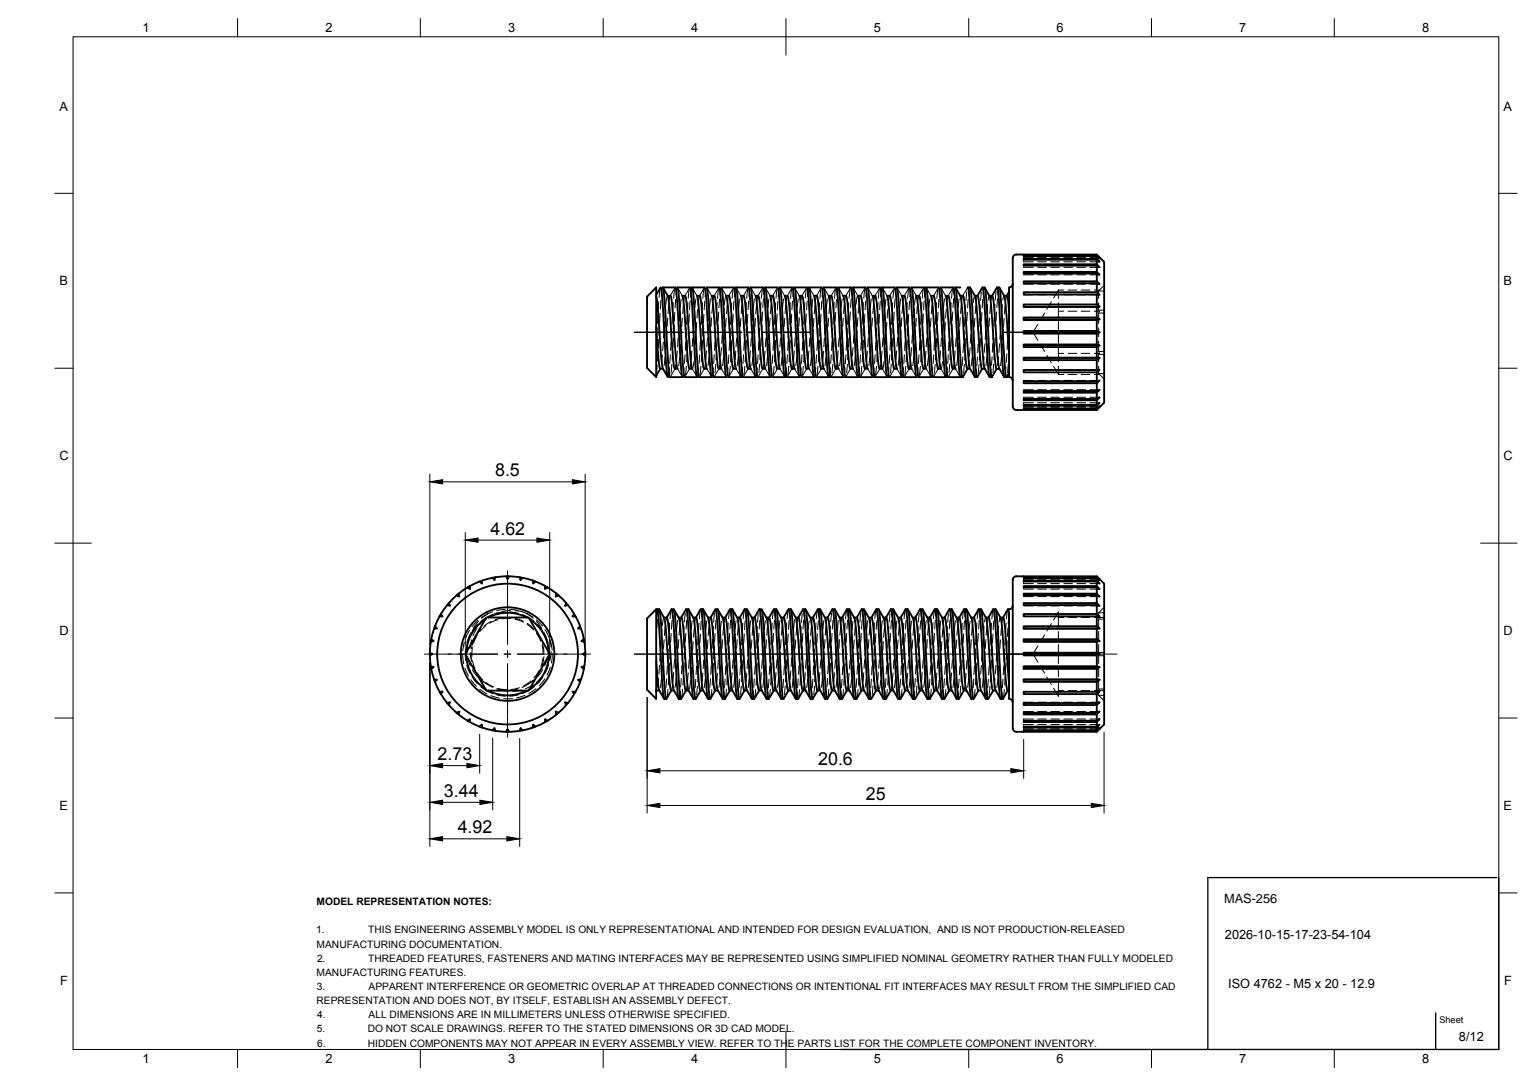
ISO-10303-21;
HEADER;
/* Generated by software containing ST-Developer
 * from STEP Tools, Inc. (www.steptools.com) 
 */

FILE_DESCRIPTION(
/* description */ (''),
/* implementation_level */ '2;1');

FILE_NAME(
/* name */ 'ISO 4762 - M5 x 20 - 12.9.step',
/* time_stamp */ '2026-10-14T18:40:07-07:00',
/* author */ (''),
/* organization */ (''),
/* preprocessor_version */ 'ST-DEVELOPER v20.2',
/* originating_system */ 'Autodesk Translation Framework v15.15.0.0',
/* authorisation */ '');

FILE_SCHEMA (('AUTOMOTIVE_DESIGN { 1 0 10303 214 3 1 1 }'));
ENDSEC;

DATA;
#10=MECHANICAL_DESIGN_GEOMETRIC_PRESENTATION_REPRESENTATION('',(#837),#81040);
#260=(
BOUNDED_CURVE()
B_SPLINE_CURVE(2,(#42262,#42263,#42264),.UNSPECIFIED.,.F.,.F.)
B_SPLINE_CURVE_WITH_KNOTS((3,3),(0.,0.0216285523885327),.UNSPECIFIED.)
CURVE()
GEOMETRIC_REPRESENTATION_ITEM()
RATIONAL_B_SPLINE_CURVE((1.,1.000549833114,1.00070303138813))
REPRESENTATION_ITEM('')
);
#261=(
BOUNDED_CURVE()
B_SPLINE_CURVE(2,(#42268,#42269,#42270),.UNSPECIFIED.,.F.,.F.)
B_SPLINE_CURVE_WITH_KNOTS((3,3),(0.0383363983196538,0.0599649507081082),
 .UNSPECIFIED.)
CURVE()
GEOMETRIC_REPRESENTATION_ITEM()
RATIONAL_B_SPLINE_CURVE((1.00070303139789,1.00054983312164,1.))
REPRESENTATION_ITEM('')
);
#262=(
BOUNDED_CURVE()
B_SPLINE_CURVE(2,(#42563,#42564,#42565),.UNSPECIFIED.,.F.,.F.)
B_SPLINE_CURVE_WITH_KNOTS((3,3),(0.,0.0216285523885616),.UNSPECIFIED.)
CURVE()
GEOMETRIC_REPRESENTATION_ITEM()
RATIONAL_B_SPLINE_CURVE((1.,1.00054983311705,1.00070303139203))
REPRESENTATION_ITEM('')
);
#263=(
BOUNDED_CURVE()
B_SPLINE_CURVE(2,(#42567,#42568,#42569),.UNSPECIFIED.,.F.,.F.)
B_SPLINE_CURVE_WITH_KNOTS((3,3),(0.0383363983195465,0.0599649507081086),
 .UNSPECIFIED.)
CURVE()
GEOMETRIC_REPRESENTATION_ITEM()
RATIONAL_B_SPLINE_CURVE((1.00070303139079,1.00054983311608,1.))
REPRESENTATION_ITEM('')
);
#264=(
BOUNDED_CURVE()
B_SPLINE_CURVE(2,(#42574,#42575,#42576),.UNSPECIFIED.,.F.,.F.)
B_SPLINE_CURVE_WITH_KNOTS((3,3),(0.0383363983195738,0.0599649507081061),
 .UNSPECIFIED.)
CURVE()
GEOMETRIC_REPRESENTATION_ITEM()
RATIONAL_B_SPLINE_CURVE((1.00070303139411,1.00054983311868,1.))
REPRESENTATION_ITEM('')
);
#265=(
BOUNDED_CURVE()
B_SPLINE_CURVE(2,(#42578,#42579,#42580),.UNSPECIFIED.,.F.,.F.)
B_SPLINE_CURVE_WITH_KNOTS((3,3),(0.,0.0216285523884906),.UNSPECIFIED.)
CURVE()
GEOMETRIC_REPRESENTATION_ITEM()
RATIONAL_B_SPLINE_CURVE((1.,1.00054983311838,1.00070303139373))
REPRESENTATION_ITEM('')
);
#266=(
BOUNDED_CURVE()
B_SPLINE_CURVE(2,(#42581,#42582,#42583),.UNSPECIFIED.,.F.,.F.)
B_SPLINE_CURVE_WITH_KNOTS((3,3),(0.0383363983195406,0.0599649507081063),
 .UNSPECIFIED.)
CURVE()
GEOMETRIC_REPRESENTATION_ITEM()
RATIONAL_B_SPLINE_CURVE((1.00070303138964,1.00054983311518,1.))
REPRESENTATION_ITEM('')
);
#267=(
BOUNDED_CURVE()
B_SPLINE_CURVE(2,(#42585,#42586,#42587),.UNSPECIFIED.,.F.,.F.)
B_SPLINE_CURVE_WITH_KNOTS((3,3),(0.,0.0216285523884772),.UNSPECIFIED.)
CURVE()
GEOMETRIC_REPRESENTATION_ITEM()
RATIONAL_B_SPLINE_CURVE((1.,1.00054983312122,1.00070303139736))
REPRESENTATION_ITEM('')
);
#268=(
BOUNDED_CURVE()
B_SPLINE_CURVE(2,(#42588,#42589,#42590),.UNSPECIFIED.,.F.,.F.)
B_SPLINE_CURVE_WITH_KNOTS((3,3),(0.0383363983195954,0.0599649507081057),
 .UNSPECIFIED.)
CURVE()
GEOMETRIC_REPRESENTATION_ITEM()
RATIONAL_B_SPLINE_CURVE((1.00070303139538,1.00054983311967,1.))
REPRESENTATION_ITEM('')
);
#269=(
BOUNDED_CURVE()
B_SPLINE_CURVE(2,(#42592,#42593,#42594),.UNSPECIFIED.,.F.,.F.)
B_SPLINE_CURVE_WITH_KNOTS((3,3),(0.,0.0216285523885691),.UNSPECIFIED.)
CURVE()
GEOMETRIC_REPRESENTATION_ITEM()
RATIONAL_B_SPLINE_CURVE((1.,1.00054983311357,1.00070303138758))
REPRESENTATION_ITEM('')
);
#270=(
BOUNDED_CURVE()
B_SPLINE_CURVE(2,(#42595,#42596,#42597),.UNSPECIFIED.,.F.,.F.)
B_SPLINE_CURVE_WITH_KNOTS((3,3),(0.0383363983195734,0.0599649507081057),
 .UNSPECIFIED.)
CURVE()
GEOMETRIC_REPRESENTATION_ITEM()
RATIONAL_B_SPLINE_CURVE((1.00070303138924,1.00054983311487,1.))
REPRESENTATION_ITEM('')
);
#271=(
BOUNDED_CURVE()
B_SPLINE_CURVE(2,(#42599,#42600,#42601),.UNSPECIFIED.,.F.,.F.)
B_SPLINE_CURVE_WITH_KNOTS((3,3),(0.,0.021628552388544),.UNSPECIFIED.)
CURVE()
GEOMETRIC_REPRESENTATION_ITEM()
RATIONAL_B_SPLINE_CURVE((1.,1.00054983311579,1.00070303139042))
REPRESENTATION_ITEM('')
);
#272=(
BOUNDED_CURVE()
B_SPLINE_CURVE(2,(#42602,#42603,#42604),.UNSPECIFIED.,.F.,.F.)
B_SPLINE_CURVE_WITH_KNOTS((3,3),(0.0383363983195219,0.0599649507081056),
 .UNSPECIFIED.)
CURVE()
GEOMETRIC_REPRESENTATION_ITEM()
RATIONAL_B_SPLINE_CURVE((1.00070303138672,1.0005498331129,1.))
REPRESENTATION_ITEM('')
);
#273=(
BOUNDED_CURVE()
B_SPLINE_CURVE(2,(#42606,#42607,#42608),.UNSPECIFIED.,.F.,.F.)
B_SPLINE_CURVE_WITH_KNOTS((3,3),(0.,0.0216285523886276),.UNSPECIFIED.)
CURVE()
GEOMETRIC_REPRESENTATION_ITEM()
RATIONAL_B_SPLINE_CURVE((1.,1.00054983311002,1.00070303138303))
REPRESENTATION_ITEM('')
);
#274=(
BOUNDED_CURVE()
B_SPLINE_CURVE(2,(#42609,#42610,#42611),.UNSPECIFIED.,.F.,.F.)
B_SPLINE_CURVE_WITH_KNOTS((3,3),(0.0383363983195948,0.0599649507081057),
 .UNSPECIFIED.)
CURVE()
GEOMETRIC_REPRESENTATION_ITEM()
RATIONAL_B_SPLINE_CURVE((1.00070303139332,1.00054983311806,1.))
REPRESENTATION_ITEM('')
);
#275=(
BOUNDED_CURVE()
B_SPLINE_CURVE(2,(#42613,#42614,#42615),.UNSPECIFIED.,.F.,.F.)
B_SPLINE_CURVE_WITH_KNOTS((3,3),(0.,0.0216285523885387),.UNSPECIFIED.)
CURVE()
GEOMETRIC_REPRESENTATION_ITEM()
RATIONAL_B_SPLINE_CURVE((1.,1.00054983311459,1.00070303138888))
REPRESENTATION_ITEM('')
);
#276=(
BOUNDED_CURVE()
B_SPLINE_CURVE(2,(#42616,#42617,#42618),.UNSPECIFIED.,.F.,.F.)
B_SPLINE_CURVE_WITH_KNOTS((3,3),(0.0383363983195453,0.0599649507081048),
 .UNSPECIFIED.)
CURVE()
GEOMETRIC_REPRESENTATION_ITEM()
RATIONAL_B_SPLINE_CURVE((1.00070303138923,1.00054983311486,1.))
REPRESENTATION_ITEM('')
);
#277=(
BOUNDED_CURVE()
B_SPLINE_CURVE(2,(#42620,#42621,#42622),.UNSPECIFIED.,.F.,.F.)
B_SPLINE_CURVE_WITH_KNOTS((3,3),(0.,0.0216285523885327),.UNSPECIFIED.)
CURVE()
GEOMETRIC_REPRESENTATION_ITEM()
RATIONAL_B_SPLINE_CURVE((1.,1.000549833118,1.00070303139324))
REPRESENTATION_ITEM('')
);
#278=(
BOUNDED_CURVE()
B_SPLINE_CURVE(2,(#42623,#42624,#42625),.UNSPECIFIED.,.F.,.F.)
B_SPLINE_CURVE_WITH_KNOTS((3,3),(0.038336398319501,0.0599649507081059),
 .UNSPECIFIED.)
CURVE()
GEOMETRIC_REPRESENTATION_ITEM()
RATIONAL_B_SPLINE_CURVE((1.00070303138577,1.00054983311216,1.))
REPRESENTATION_ITEM('')
);
#279=(
BOUNDED_CURVE()
B_SPLINE_CURVE(2,(#42627,#42628,#42629),.UNSPECIFIED.,.F.,.F.)
B_SPLINE_CURVE_WITH_KNOTS((3,3),(0.,0.0216285523885216),.UNSPECIFIED.)
CURVE()
GEOMETRIC_REPRESENTATION_ITEM()
RATIONAL_B_SPLINE_CURVE((1.,1.0005498331148,1.00070303138915))
REPRESENTATION_ITEM('')
);
#280=(
BOUNDED_CURVE()
B_SPLINE_CURVE(2,(#42630,#42631,#42632),.UNSPECIFIED.,.F.,.F.)
B_SPLINE_CURVE_WITH_KNOTS((3,3),(0.0383363983195421,0.0599649507081054),
 .UNSPECIFIED.)
CURVE()
GEOMETRIC_REPRESENTATION_ITEM()
RATIONAL_B_SPLINE_CURVE((1.00070303139029,1.00054983311569,1.))
REPRESENTATION_ITEM('')
);
#281=(
BOUNDED_CURVE()
B_SPLINE_CURVE(2,(#42634,#42635,#42636),.UNSPECIFIED.,.F.,.F.)
B_SPLINE_CURVE_WITH_KNOTS((3,3),(0.,0.0216285523885795),.UNSPECIFIED.)
CURVE()
GEOMETRIC_REPRESENTATION_ITEM()
RATIONAL_B_SPLINE_CURVE((1.,1.0005498331127,1.00070303138646))
REPRESENTATION_ITEM('')
);
#282=(
BOUNDED_CURVE()
B_SPLINE_CURVE(2,(#42637,#42638,#42639),.UNSPECIFIED.,.F.,.F.)
B_SPLINE_CURVE_WITH_KNOTS((3,3),(0.0383363983195796,0.0599649507081049),
 .UNSPECIFIED.)
CURVE()
GEOMETRIC_REPRESENTATION_ITEM()
RATIONAL_B_SPLINE_CURVE((1.00070303139298,1.00054983311779,1.))
REPRESENTATION_ITEM('')
);
#283=(
BOUNDED_CURVE()
B_SPLINE_CURVE(2,(#42641,#42642,#42643),.UNSPECIFIED.,.F.,.F.)
B_SPLINE_CURVE_WITH_KNOTS((3,3),(0.,0.0216285523885516),.UNSPECIFIED.)
CURVE()
GEOMETRIC_REPRESENTATION_ITEM()
RATIONAL_B_SPLINE_CURVE((1.,1.00054983311626,1.00070303139102))
REPRESENTATION_ITEM('')
);
#284=(
BOUNDED_CURVE()
B_SPLINE_CURVE(2,(#42644,#42645,#42646),.UNSPECIFIED.,.F.,.F.)
B_SPLINE_CURVE_WITH_KNOTS((3,3),(0.0383363983195596,0.059964950708105),
 .UNSPECIFIED.)
CURVE()
GEOMETRIC_REPRESENTATION_ITEM()
RATIONAL_B_SPLINE_CURVE((1.00070303138868,1.00054983311444,1.))
REPRESENTATION_ITEM('')
);
#285=(
BOUNDED_CURVE()
B_SPLINE_CURVE(2,(#42648,#42649,#42650),.UNSPECIFIED.,.F.,.F.)
B_SPLINE_CURVE_WITH_KNOTS((3,3),(0.,0.0216285523885783),.UNSPECIFIED.)
CURVE()
GEOMETRIC_REPRESENTATION_ITEM()
RATIONAL_B_SPLINE_CURVE((1.,1.00054983311312,1.000703031387))
REPRESENTATION_ITEM('')
);
#286=(
BOUNDED_CURVE()
B_SPLINE_CURVE(2,(#42651,#42652,#42653),.UNSPECIFIED.,.F.,.F.)
B_SPLINE_CURVE_WITH_KNOTS((3,3),(0.0383363983195159,0.0599649507081054),
 .UNSPECIFIED.)
CURVE()
GEOMETRIC_REPRESENTATION_ITEM()
RATIONAL_B_SPLINE_CURVE((1.00070303138659,1.0005498331128,1.))
REPRESENTATION_ITEM('')
);
#287=(
BOUNDED_CURVE()
B_SPLINE_CURVE(2,(#42655,#42656,#42657),.UNSPECIFIED.,.F.,.F.)
B_SPLINE_CURVE_WITH_KNOTS((3,3),(0.,0.0216285523885604),.UNSPECIFIED.)
CURVE()
GEOMETRIC_REPRESENTATION_ITEM()
RATIONAL_B_SPLINE_CURVE((1.,1.00054983311293,1.00070303138676))
REPRESENTATION_ITEM('')
);
#288=(
BOUNDED_CURVE()
B_SPLINE_CURVE(2,(#42658,#42659,#42660),.UNSPECIFIED.,.F.,.F.)
B_SPLINE_CURVE_WITH_KNOTS((3,3),(0.0383363983195082,0.0599649507081046),
 .UNSPECIFIED.)
CURVE()
GEOMETRIC_REPRESENTATION_ITEM()
RATIONAL_B_SPLINE_CURVE((1.00070303138548,1.00054983311193,1.))
REPRESENTATION_ITEM('')
);
#289=(
BOUNDED_CURVE()
B_SPLINE_CURVE(2,(#42662,#42663,#42664),.UNSPECIFIED.,.F.,.F.)
B_SPLINE_CURVE_WITH_KNOTS((3,3),(0.,0.0216285523886338),.UNSPECIFIED.)
CURVE()
GEOMETRIC_REPRESENTATION_ITEM()
RATIONAL_B_SPLINE_CURVE((1.,1.00054983310968,1.00070303138259))
REPRESENTATION_ITEM('')
);
#290=(
BOUNDED_CURVE()
B_SPLINE_CURVE(2,(#42665,#42666,#42667),.UNSPECIFIED.,.F.,.F.)
B_SPLINE_CURVE_WITH_KNOTS((3,3),(0.0383363983196053,0.0599649507081053),
 .UNSPECIFIED.)
CURVE()
GEOMETRIC_REPRESENTATION_ITEM()
RATIONAL_B_SPLINE_CURVE((1.00070303139687,1.00054983312084,1.))
REPRESENTATION_ITEM('')
);
#291=(
BOUNDED_CURVE()
B_SPLINE_CURVE(2,(#42669,#42670,#42671),.UNSPECIFIED.,.F.,.F.)
B_SPLINE_CURVE_WITH_KNOTS((3,3),(0.,0.0216285523885115),.UNSPECIFIED.)
CURVE()
GEOMETRIC_REPRESENTATION_ITEM()
RATIONAL_B_SPLINE_CURVE((1.,1.00054983312007,1.00070303139589))
REPRESENTATION_ITEM('')
);
#292=(
BOUNDED_CURVE()
B_SPLINE_CURVE(2,(#42672,#42673,#42674),.UNSPECIFIED.,.F.,.F.)
B_SPLINE_CURVE_WITH_KNOTS((3,3),(0.0383363983195966,0.0599649507081041),
 .UNSPECIFIED.)
CURVE()
GEOMETRIC_REPRESENTATION_ITEM()
RATIONAL_B_SPLINE_CURVE((1.00070303139314,1.00054983311792,1.))
REPRESENTATION_ITEM('')
);
#293=(
BOUNDED_CURVE()
B_SPLINE_CURVE(2,(#42676,#42677,#42678),.UNSPECIFIED.,.F.,.F.)
B_SPLINE_CURVE_WITH_KNOTS((3,3),(0.,0.0216285523885745),.UNSPECIFIED.)
CURVE()
GEOMETRIC_REPRESENTATION_ITEM()
RATIONAL_B_SPLINE_CURVE((1.,1.00054983311169,1.00070303138517))
REPRESENTATION_ITEM('')
);
#294=(
BOUNDED_CURVE()
B_SPLINE_CURVE(2,(#42679,#42680,#42681),.UNSPECIFIED.,.F.,.F.)
B_SPLINE_CURVE_WITH_KNOTS((3,3),(0.0383363983195842,0.0599649507081042),
 .UNSPECIFIED.)
CURVE()
GEOMETRIC_REPRESENTATION_ITEM()
RATIONAL_B_SPLINE_CURVE((1.00070303139113,1.00054983311635,1.))
REPRESENTATION_ITEM('')
);
#295=(
BOUNDED_CURVE()
B_SPLINE_CURVE(2,(#42683,#42684,#42685),.UNSPECIFIED.,.F.,.F.)
B_SPLINE_CURVE_WITH_KNOTS((3,3),(0.,0.0216285523885027),.UNSPECIFIED.)
CURVE()
GEOMETRIC_REPRESENTATION_ITEM()
RATIONAL_B_SPLINE_CURVE((1.,1.00054983311917,1.00070303139474))
REPRESENTATION_ITEM('')
);
#296=(
BOUNDED_CURVE()
B_SPLINE_CURVE(2,(#42686,#42687,#42688),.UNSPECIFIED.,.F.,.F.)
B_SPLINE_CURVE_WITH_KNOTS((3,3),(0.0383363983195908,0.0599649507081052),
 .UNSPECIFIED.)
CURVE()
GEOMETRIC_REPRESENTATION_ITEM()
RATIONAL_B_SPLINE_CURVE((1.00070303139353,1.00054983311823,1.))
REPRESENTATION_ITEM('')
);
#297=(
BOUNDED_CURVE()
B_SPLINE_CURVE(2,(#42690,#42691,#42692),.UNSPECIFIED.,.F.,.F.)
B_SPLINE_CURVE_WITH_KNOTS((3,3),(0.,0.0216285523885997),.UNSPECIFIED.)
CURVE()
GEOMETRIC_REPRESENTATION_ITEM()
RATIONAL_B_SPLINE_CURVE((1.,1.00054983311374,1.00070303138779))
REPRESENTATION_ITEM('')
);
#298=(
BOUNDED_CURVE()
B_SPLINE_CURVE(2,(#42693,#42694,#42695),.UNSPECIFIED.,.F.,.F.)
B_SPLINE_CURVE_WITH_KNOTS((3,3),(0.0383363983195373,0.0599649507081046),
 .UNSPECIFIED.)
CURVE()
GEOMETRIC_REPRESENTATION_ITEM()
RATIONAL_B_SPLINE_CURVE((1.00070303138796,1.00054983311387,1.))
REPRESENTATION_ITEM('')
);
#299=(
BOUNDED_CURVE()
B_SPLINE_CURVE(2,(#42697,#42698,#42699),.UNSPECIFIED.,.F.,.F.)
B_SPLINE_CURVE_WITH_KNOTS((3,3),(0.,0.0216285523885614),.UNSPECIFIED.)
CURVE()
GEOMETRIC_REPRESENTATION_ITEM()
RATIONAL_B_SPLINE_CURVE((1.,1.00054983311414,1.00070303138831))
REPRESENTATION_ITEM('')
);
#300=(
BOUNDED_CURVE()
B_SPLINE_CURVE(2,(#42700,#42701,#42702),.UNSPECIFIED.,.F.,.F.)
B_SPLINE_CURVE_WITH_KNOTS((3,3),(0.0383363983195286,0.0599649507081044),
 .UNSPECIFIED.)
CURVE()
GEOMETRIC_REPRESENTATION_ITEM()
RATIONAL_B_SPLINE_CURVE((1.00070303139035,1.00054983311574,1.))
REPRESENTATION_ITEM('')
);
#301=(
BOUNDED_CURVE()
B_SPLINE_CURVE(2,(#42704,#42705,#42706),.UNSPECIFIED.,.F.,.F.)
B_SPLINE_CURVE_WITH_KNOTS((3,3),(0.,0.0216285523885108),.UNSPECIFIED.)
CURVE()
GEOMETRIC_REPRESENTATION_ITEM()
RATIONAL_B_SPLINE_CURVE((1.,1.00054983311702,1.00070303139198))
REPRESENTATION_ITEM('')
);
#302=(
BOUNDED_CURVE()
B_SPLINE_CURVE(2,(#42707,#42708,#42709),.UNSPECIFIED.,.F.,.F.)
B_SPLINE_CURVE_WITH_KNOTS((3,3),(0.0383363983195893,0.0599649507081084),
 .UNSPECIFIED.)
CURVE()
GEOMETRIC_REPRESENTATION_ITEM()
RATIONAL_B_SPLINE_CURVE((1.00070303139496,1.00054983311935,1.))
REPRESENTATION_ITEM('')
);
#303=(
BOUNDED_CURVE()
B_SPLINE_CURVE(2,(#42711,#42712,#42713),.UNSPECIFIED.,.F.,.F.)
B_SPLINE_CURVE_WITH_KNOTS((3,3),(0.,0.021628552388581),.UNSPECIFIED.)
CURVE()
GEOMETRIC_REPRESENTATION_ITEM()
RATIONAL_B_SPLINE_CURVE((1.,1.00054983311652,1.00070303139135))
REPRESENTATION_ITEM('')
);
#304=(
BOUNDED_CURVE()
B_SPLINE_CURVE(2,(#42714,#42715,#42716),.UNSPECIFIED.,.F.,.F.)
B_SPLINE_CURVE_WITH_KNOTS((3,3),(0.0383363983195303,0.059964950708108),
 .UNSPECIFIED.)
CURVE()
GEOMETRIC_REPRESENTATION_ITEM()
RATIONAL_B_SPLINE_CURVE((1.00070303138822,1.00054983311407,1.))
REPRESENTATION_ITEM('')
);
#305=(
BOUNDED_CURVE()
B_SPLINE_CURVE(2,(#42718,#42719,#42720),.UNSPECIFIED.,.F.,.F.)
B_SPLINE_CURVE_WITH_KNOTS((3,3),(0.,0.0216285523886002),.UNSPECIFIED.)
CURVE()
GEOMETRIC_REPRESENTATION_ITEM()
RATIONAL_B_SPLINE_CURVE((1.,1.00054983311286,1.00070303138666))
REPRESENTATION_ITEM('')
);
#306=(
BOUNDED_CURVE()
B_SPLINE_CURVE(2,(#42721,#42722,#42723),.UNSPECIFIED.,.F.,.F.)
B_SPLINE_CURVE_WITH_KNOTS((3,3),(0.0383363983195208,0.059964950708108),
 .UNSPECIFIED.)
CURVE()
GEOMETRIC_REPRESENTATION_ITEM()
RATIONAL_B_SPLINE_CURVE((1.00070303138903,1.00054983311471,1.))
REPRESENTATION_ITEM('')
);
#307=(
BOUNDED_CURVE()
B_SPLINE_CURVE(2,(#42725,#42726,#42727),.UNSPECIFIED.,.F.,.F.)
B_SPLINE_CURVE_WITH_KNOTS((3,3),(0.,0.0216285523885397),.UNSPECIFIED.)
CURVE()
GEOMETRIC_REPRESENTATION_ITEM()
RATIONAL_B_SPLINE_CURVE((1.,1.00054983311497,1.00070303138936))
REPRESENTATION_ITEM('')
);
#308=(
BOUNDED_CURVE()
B_SPLINE_CURVE(2,(#42728,#42729,#42730),.UNSPECIFIED.,.F.,.F.)
B_SPLINE_CURVE_WITH_KNOTS((3,3),(0.0383363983195002,0.0599649507081073),
 .UNSPECIFIED.)
CURVE()
GEOMETRIC_REPRESENTATION_ITEM()
RATIONAL_B_SPLINE_CURVE((1.00070303138446,1.00054983311114,1.))
REPRESENTATION_ITEM('')
);
#309=(
BOUNDED_CURVE()
B_SPLINE_CURVE(2,(#42732,#42733,#42734),.UNSPECIFIED.,.F.,.F.)
B_SPLINE_CURVE_WITH_KNOTS((3,3),(0.,0.0216285523885717),.UNSPECIFIED.)
CURVE()
GEOMETRIC_REPRESENTATION_ITEM()
RATIONAL_B_SPLINE_CURVE((1.,1.00054983311286,1.00070303138667))
REPRESENTATION_ITEM('')
);
#310=(
BOUNDED_CURVE()
B_SPLINE_CURVE(2,(#42735,#42736,#42737),.UNSPECIFIED.,.F.,.F.)
B_SPLINE_CURVE_WITH_KNOTS((3,3),(0.0383363983195212,0.0599649507081082),
 .UNSPECIFIED.)
CURVE()
GEOMETRIC_REPRESENTATION_ITEM()
RATIONAL_B_SPLINE_CURVE((1.00070303138591,1.00054983311226,1.))
REPRESENTATION_ITEM('')
);
#311=(
BOUNDED_CURVE()
B_SPLINE_CURVE(2,(#42739,#42740,#42741),.UNSPECIFIED.,.F.,.F.)
B_SPLINE_CURVE_WITH_KNOTS((3,3),(0.,0.0216285523885764),.UNSPECIFIED.)
CURVE()
GEOMETRIC_REPRESENTATION_ITEM()
RATIONAL_B_SPLINE_CURVE((1.,1.0005498331135,1.00070303138749))
REPRESENTATION_ITEM('')
);
#312=(
BOUNDED_CURVE()
B_SPLINE_CURVE(2,(#42742,#42743,#42744),.UNSPECIFIED.,.F.,.F.)
B_SPLINE_CURVE_WITH_KNOTS((3,3),(0.0383363983195505,0.059964950708108),
 .UNSPECIFIED.)
CURVE()
GEOMETRIC_REPRESENTATION_ITEM()
RATIONAL_B_SPLINE_CURVE((1.00070303138856,1.00054983311434,1.))
REPRESENTATION_ITEM('')
);
#313=(
BOUNDED_CURVE()
B_SPLINE_CURVE(2,(#42746,#42747,#42748),.UNSPECIFIED.,.F.,.F.)
B_SPLINE_CURVE_WITH_KNOTS((3,3),(0.,0.0216285523885379),.UNSPECIFIED.)
CURVE()
GEOMETRIC_REPRESENTATION_ITEM()
RATIONAL_B_SPLINE_CURVE((1.,1.00054983311513,1.00070303138957))
REPRESENTATION_ITEM('')
);
#314=(
BOUNDED_CURVE()
B_SPLINE_CURVE(2,(#42749,#42750,#42751),.UNSPECIFIED.,.F.,.F.)
B_SPLINE_CURVE_WITH_KNOTS((3,3),(0.0383363983195525,0.0599649507081075),
 .UNSPECIFIED.)
CURVE()
GEOMETRIC_REPRESENTATION_ITEM()
RATIONAL_B_SPLINE_CURVE((1.00070303138821,1.00054983311407,1.))
REPRESENTATION_ITEM('')
);
#315=(
BOUNDED_CURVE()
B_SPLINE_CURVE(2,(#42753,#42754,#42755),.UNSPECIFIED.,.F.,.F.)
B_SPLINE_CURVE_WITH_KNOTS((3,3),(0.,0.0216285523885421),.UNSPECIFIED.)
CURVE()
GEOMETRIC_REPRESENTATION_ITEM()
RATIONAL_B_SPLINE_CURVE((1.,1.00054983311399,1.00070303138812))
REPRESENTATION_ITEM('')
);
#316=(
BOUNDED_CURVE()
B_SPLINE_CURVE(2,(#42756,#42757,#42758),.UNSPECIFIED.,.F.,.F.)
B_SPLINE_CURVE_WITH_KNOTS((3,3),(0.0383363983195263,0.0599649507081077),
 .UNSPECIFIED.)
CURVE()
GEOMETRIC_REPRESENTATION_ITEM()
RATIONAL_B_SPLINE_CURVE((1.00070303138823,1.00054983311409,1.))
REPRESENTATION_ITEM('')
);
#317=(
BOUNDED_CURVE()
B_SPLINE_CURVE(2,(#42760,#42761,#42762),.UNSPECIFIED.,.F.,.F.)
B_SPLINE_CURVE_WITH_KNOTS((3,3),(0.,0.0216285523886281),.UNSPECIFIED.)
CURVE()
GEOMETRIC_REPRESENTATION_ITEM()
RATIONAL_B_SPLINE_CURVE((1.,1.00054983311262,1.00070303138635))
REPRESENTATION_ITEM('')
);
#318=(
BOUNDED_CURVE()
B_SPLINE_CURVE(2,(#42763,#42764,#42765),.UNSPECIFIED.,.F.,.F.)
B_SPLINE_CURVE_WITH_KNOTS((3,3),(0.0383363983195607,0.0599649507081075),
 .UNSPECIFIED.)
CURVE()
GEOMETRIC_REPRESENTATION_ITEM()
RATIONAL_B_SPLINE_CURVE((1.00070303139002,1.00054983311548,1.))
REPRESENTATION_ITEM('')
);
#319=(
BOUNDED_CURVE()
B_SPLINE_CURVE(2,(#42767,#42768,#42769),.UNSPECIFIED.,.F.,.F.)
B_SPLINE_CURVE_WITH_KNOTS((3,3),(0.,0.0216285523885411),.UNSPECIFIED.)
CURVE()
GEOMETRIC_REPRESENTATION_ITEM()
RATIONAL_B_SPLINE_CURVE((1.,1.00054983311589,1.00070303139054))
REPRESENTATION_ITEM('')
);
#320=(
BOUNDED_CURVE()
B_SPLINE_CURVE(2,(#42770,#42771,#42772),.UNSPECIFIED.,.F.,.F.)
B_SPLINE_CURVE_WITH_KNOTS((3,3),(0.0383363983195253,0.0599649507081071),
 .UNSPECIFIED.)
CURVE()
GEOMETRIC_REPRESENTATION_ITEM()
RATIONAL_B_SPLINE_CURVE((1.0007030313902,1.00054983311562,1.))
REPRESENTATION_ITEM('')
);
#321=(
BOUNDED_CURVE()
B_SPLINE_CURVE(2,(#42774,#42775,#42776),.UNSPECIFIED.,.F.,.F.)
B_SPLINE_CURVE_WITH_KNOTS((3,3),(0.,0.0216285523886145),.UNSPECIFIED.)
CURVE()
GEOMETRIC_REPRESENTATION_ITEM()
RATIONAL_B_SPLINE_CURVE((1.,1.00054983311291,1.00070303138673))
REPRESENTATION_ITEM('')
);
#322=(
BOUNDED_CURVE()
B_SPLINE_CURVE(2,(#42777,#42778,#42779),.UNSPECIFIED.,.F.,.F.)
B_SPLINE_CURVE_WITH_KNOTS((3,3),(0.0383363983195111,0.0599649507081069),
 .UNSPECIFIED.)
CURVE()
GEOMETRIC_REPRESENTATION_ITEM()
RATIONAL_B_SPLINE_CURVE((1.00070303138553,1.00054983311197,1.))
REPRESENTATION_ITEM('')
);
#323=(
BOUNDED_CURVE()
B_SPLINE_CURVE(2,(#42781,#42782,#42783),.UNSPECIFIED.,.F.,.F.)
B_SPLINE_CURVE_WITH_KNOTS((3,3),(0.,0.0216285523885865),.UNSPECIFIED.)
CURVE()
GEOMETRIC_REPRESENTATION_ITEM()
RATIONAL_B_SPLINE_CURVE((1.,1.00054983311348,1.00070303138746))
REPRESENTATION_ITEM('')
);
#324=(
BOUNDED_CURVE()
B_SPLINE_CURVE(2,(#42784,#42785,#42786),.UNSPECIFIED.,.F.,.F.)
B_SPLINE_CURVE_WITH_KNOTS((3,3),(0.0383363983194927,0.0599649507081069),
 .UNSPECIFIED.)
CURVE()
GEOMETRIC_REPRESENTATION_ITEM()
RATIONAL_B_SPLINE_CURVE((1.00070303138451,1.00054983311118,1.))
REPRESENTATION_ITEM('')
);
#325=(
BOUNDED_CURVE()
B_SPLINE_CURVE(2,(#42788,#42789,#42790),.UNSPECIFIED.,.F.,.F.)
B_SPLINE_CURVE_WITH_KNOTS((3,3),(0.,0.0216285523884905),.UNSPECIFIED.)
CURVE()
GEOMETRIC_REPRESENTATION_ITEM()
RATIONAL_B_SPLINE_CURVE((1.,1.00054983311838,1.00070303139373))
REPRESENTATION_ITEM('')
);
#326=(
BOUNDED_CURVE()
B_SPLINE_CURVE(2,(#42791,#42792,#42793),.UNSPECIFIED.,.F.,.F.)
B_SPLINE_CURVE_WITH_KNOTS((3,3),(0.0383363983196131,0.0599649507081062),
 .UNSPECIFIED.)
CURVE()
GEOMETRIC_REPRESENTATION_ITEM()
RATIONAL_B_SPLINE_CURVE((1.00070303139756,1.00054983312138,1.))
REPRESENTATION_ITEM('')
);
#327=(
BOUNDED_CURVE()
B_SPLINE_CURVE(2,(#42795,#42796,#42797),.UNSPECIFIED.,.F.,.F.)
B_SPLINE_CURVE_WITH_KNOTS((3,3),(0.,0.0216285523886255),.UNSPECIFIED.)
CURVE()
GEOMETRIC_REPRESENTATION_ITEM()
RATIONAL_B_SPLINE_CURVE((1.,1.00054983311094,1.00070303138421))
REPRESENTATION_ITEM('')
);
#328=(
BOUNDED_CURVE()
B_SPLINE_CURVE(2,(#42798,#42799,#42800),.UNSPECIFIED.,.F.,.F.)
B_SPLINE_CURVE_WITH_KNOTS((3,3),(0.0383363983195603,0.0599649507081068),
 .UNSPECIFIED.)
CURVE()
GEOMETRIC_REPRESENTATION_ITEM()
RATIONAL_B_SPLINE_CURVE((1.0007030313936,1.00054983311828,1.))
REPRESENTATION_ITEM('')
);
#329=(
BOUNDED_CURVE()
B_SPLINE_CURVE(2,(#42802,#42803,#42804),.UNSPECIFIED.,.F.,.F.)
B_SPLINE_CURVE_WITH_KNOTS((3,3),(0.,0.021628552388625),.UNSPECIFIED.)
CURVE()
GEOMETRIC_REPRESENTATION_ITEM()
RATIONAL_B_SPLINE_CURVE((1.,1.00054983311264,1.00070303138639))
REPRESENTATION_ITEM('')
);
#330=(
BOUNDED_CURVE()
B_SPLINE_CURVE(2,(#42805,#42806,#42807),.UNSPECIFIED.,.F.,.F.)
B_SPLINE_CURVE_WITH_KNOTS((3,3),(0.0383363983195806,0.059964950708106),
 .UNSPECIFIED.)
CURVE()
GEOMETRIC_REPRESENTATION_ITEM()
RATIONAL_B_SPLINE_CURVE((1.00070303139255,1.00054983311746,1.))
REPRESENTATION_ITEM('')
);
#331=(
BOUNDED_CURVE()
B_SPLINE_CURVE(2,(#42808,#42809,#42810),.UNSPECIFIED.,.F.,.F.)
B_SPLINE_CURVE_WITH_KNOTS((3,3),(0.,0.0216285523884755),.UNSPECIFIED.)
CURVE()
GEOMETRIC_REPRESENTATION_ITEM()
RATIONAL_B_SPLINE_CURVE((1.,1.00054983312103,1.00070303139712))
REPRESENTATION_ITEM('')
);
#332=(
BOUNDED_CURVE()
B_SPLINE_CURVE(2,(#43060,#43061,#43062),.UNSPECIFIED.,.F.,.F.)
B_SPLINE_CURVE_WITH_KNOTS((3,3),(0.,0.0124050518656677),.UNSPECIFIED.)
CURVE()
GEOMETRIC_REPRESENTATION_ITEM()
RATIONAL_B_SPLINE_CURVE((1.,1.00128973373368,1.00206600698525))
REPRESENTATION_ITEM('')
);
#333=(
BOUNDED_CURVE()
B_SPLINE_CURVE(2,(#43066,#43067,#43068),.UNSPECIFIED.,.F.,.F.)
B_SPLINE_CURVE_WITH_KNOTS((3,3),(0.0499141116010052,0.0623191634666637),
 .UNSPECIFIED.)
CURVE()
GEOMETRIC_REPRESENTATION_ITEM()
RATIONAL_B_SPLINE_CURVE((1.00206600698578,1.00128973373401,1.))
REPRESENTATION_ITEM('')
);
#334=(
BOUNDED_CURVE()
B_SPLINE_CURVE(2,(#43070,#43071,#43072),.UNSPECIFIED.,.F.,.F.)
B_SPLINE_CURVE_WITH_KNOTS((3,3),(0.,0.0124050518656597),.UNSPECIFIED.)
CURVE()
GEOMETRIC_REPRESENTATION_ITEM()
RATIONAL_B_SPLINE_CURVE((1.,1.00128973373396,1.00206600698569))
REPRESENTATION_ITEM('')
);
#335=(
BOUNDED_CURVE()
B_SPLINE_CURVE(2,(#43076,#43077,#43078),.UNSPECIFIED.,.F.,.F.)
B_SPLINE_CURVE_WITH_KNOTS((3,3),(0.049914111601003,0.0623191634666626),
 .UNSPECIFIED.)
CURVE()
GEOMETRIC_REPRESENTATION_ITEM()
RATIONAL_B_SPLINE_CURVE((1.00206600698569,1.00128973373396,1.))
REPRESENTATION_ITEM('')
);
#336=(
BOUNDED_CURVE()
B_SPLINE_CURVE(2,(#43080,#43081,#43082),.UNSPECIFIED.,.F.,.F.)
B_SPLINE_CURVE_WITH_KNOTS((3,3),(0.,0.0124050518656559),.UNSPECIFIED.)
CURVE()
GEOMETRIC_REPRESENTATION_ITEM()
RATIONAL_B_SPLINE_CURVE((1.,1.00128973373402,1.0020660069858))
REPRESENTATION_ITEM('')
);
#337=(
BOUNDED_CURVE()
B_SPLINE_CURVE(2,(#43086,#43087,#43088),.UNSPECIFIED.,.F.,.F.)
B_SPLINE_CURVE_WITH_KNOTS((3,3),(0.0499141116009975,0.062319163466664),
 .UNSPECIFIED.)
CURVE()
GEOMETRIC_REPRESENTATION_ITEM()
RATIONAL_B_SPLINE_CURVE((1.00206600698527,1.0012897337337,1.))
REPRESENTATION_ITEM('')
);
#338=(
BOUNDED_CURVE()
B_SPLINE_CURVE(2,(#43090,#43091,#43092),.UNSPECIFIED.,.F.,.F.)
B_SPLINE_CURVE_WITH_KNOTS((3,3),(0.,0.0124050518656685),.UNSPECIFIED.)
CURVE()
GEOMETRIC_REPRESENTATION_ITEM()
RATIONAL_B_SPLINE_CURVE((1.,1.00128973373364,1.00206600698518))
REPRESENTATION_ITEM('')
);
#339=(
BOUNDED_CURVE()
B_SPLINE_CURVE(2,(#43096,#43097,#43098),.UNSPECIFIED.,.F.,.F.)
B_SPLINE_CURVE_WITH_KNOTS((3,3),(0.049914111600997,0.0623191634666649),
 .UNSPECIFIED.)
CURVE()
GEOMETRIC_REPRESENTATION_ITEM()
RATIONAL_B_SPLINE_CURVE((1.00206600698519,1.00128973373364,1.))
REPRESENTATION_ITEM('')
);
#340=(
BOUNDED_CURVE()
B_SPLINE_CURVE(2,(#43100,#43101,#43102),.UNSPECIFIED.,.F.,.F.)
B_SPLINE_CURVE_WITH_KNOTS((3,3),(0.,0.0124050518656616),.UNSPECIFIED.)
CURVE()
GEOMETRIC_REPRESENTATION_ITEM()
RATIONAL_B_SPLINE_CURVE((1.,1.0012897337338,1.00206600698545))
REPRESENTATION_ITEM('')
);
#341=(
BOUNDED_CURVE()
B_SPLINE_CURVE(2,(#43106,#43107,#43108),.UNSPECIFIED.,.F.,.F.)
B_SPLINE_CURVE_WITH_KNOTS((3,3),(0.049914111601002,0.0623191634666634),
 .UNSPECIFIED.)
CURVE()
GEOMETRIC_REPRESENTATION_ITEM()
RATIONAL_B_SPLINE_CURVE((1.00206600698545,1.0012897337338,1.))
REPRESENTATION_ITEM('')
);
#342=(
BOUNDED_CURVE()
B_SPLINE_CURVE(2,(#43110,#43111,#43112),.UNSPECIFIED.,.F.,.F.)
B_SPLINE_CURVE_WITH_KNOTS((3,3),(0.,0.0124050518656481),.UNSPECIFIED.)
CURVE()
GEOMETRIC_REPRESENTATION_ITEM()
RATIONAL_B_SPLINE_CURVE((1.,1.00128973373427,1.0020660069862))
REPRESENTATION_ITEM('')
);
#343=(
BOUNDED_CURVE()
B_SPLINE_CURVE(2,(#43115,#43116,#43117),.UNSPECIFIED.,.F.,.F.)
B_SPLINE_CURVE_WITH_KNOTS((3,3),(0.0499141116009961,0.0623191634666644),
 .UNSPECIFIED.)
CURVE()
GEOMETRIC_REPRESENTATION_ITEM()
RATIONAL_B_SPLINE_CURVE((1.0020660069852,1.00128973373365,1.))
REPRESENTATION_ITEM('')
);
#360=TOROIDAL_SURFACE('',#16122,2.6505,0.2);
#361=TOROIDAL_SURFACE('',#16315,4.05,0.2);
#364=B_SPLINE_SURFACE_WITH_KNOTS('',3,3,((#40791,#40792,#40793,#40794,#40795,
#40796,#40797,#40798,#40799,#40800,#40801,#40802,#40803,#40804,#40805,#40806,
#40807,#40808,#40809,#40810,#40811,#40812,#40813,#40814,#40815,#40816,#40817,
#40818,#40819,#40820,#40821,#40822,#40823,#40824,#40825,#40826,#40827,#40828,
#40829,#40830,#40831,#40832,#40833,#40834,#40835,#40836,#40837,#40838,#40839,
#40840,#40841,#40842,#40843,#40844,#40845,#40846,#40847,#40848,#40849,#40850,
#40851,#40852,#40853,#40854,#40855,#40856,#40857,#40858,#40859,#40860,#40861,
#40862,#40863,#40864,#40865,#40866,#40867,#40868,#40869,#40870,#40871,#40872,
#40873,#40874,#40875,#40876,#40877,#40878,#40879,#40880,#40881,#40882,#40883,
#40884,#40885,#40886,#40887,#40888,#40889,#40890,#40891,#40892,#40893,#40894,
#40895,#40896,#40897,#40898,#40899,#40900,#40901,#40902,#40903,#40904,#40905,
#40906,#40907,#40908,#40909,#40910,#40911,#40912,#40913,#40914,#40915,#40916,
#40917,#40918,#40919,#40920,#40921,#40922,#40923,#40924,#40925,#40926,#40927,
#40928,#40929,#40930,#40931,#40932,#40933,#40934,#40935,#40936,#40937,#40938,
#40939,#40940,#40941,#40942,#40943,#40944,#40945,#40946,#40947),(#40948,
#40949,#40950,#40951,#40952,#40953,#40954,#40955,#40956,#40957,#40958,#40959,
#40960,#40961,#40962,#40963,#40964,#40965,#40966,#40967,#40968,#40969,#40970,
#40971,#40972,#40973,#40974,#40975,#40976,#40977,#40978,#40979,#40980,#40981,
#40982,#40983,#40984,#40985,#40986,#40987,#40988,#40989,#40990,#40991,#40992,
#40993,#40994,#40995,#40996,#40997,#40998,#40999,#41000,#41001,#41002,#41003,
#41004,#41005,#41006,#41007,#41008,#41009,#41010,#41011,#41012,#41013,#41014,
#41015,#41016,#41017,#41018,#41019,#41020,#41021,#41022,#41023,#41024,#41025,
#41026,#41027,#41028,#41029,#41030,#41031,#41032,#41033,#41034,#41035,#41036,
#41037,#41038,#41039,#41040,#41041,#41042,#41043,#41044,#41045,#41046,#41047,
#41048,#41049,#41050,#41051,#41052,#41053,#41054,#41055,#41056,#41057,#41058,
#41059,#41060,#41061,#41062,#41063,#41064,#41065,#41066,#41067,#41068,#41069,
#41070,#41071,#41072,#41073,#41074,#41075,#41076,#41077,#41078,#41079,#41080,
#41081,#41082,#41083,#41084,#41085,#41086,#41087,#41088,#41089,#41090,#41091,
#41092,#41093,#41094,#41095,#41096,#41097,#41098,#41099,#41100,#41101,#41102,
#41103,#41104),(#41105,#41106,#41107,#41108,#41109,#41110,#41111,#41112,
#41113,#41114,#41115,#41116,#41117,#41118,#41119,#41120,#41121,#41122,#41123,
#41124,#41125,#41126,#41127,#41128,#41129,#41130,#41131,#41132,#41133,#41134,
#41135,#41136,#41137,#41138,#41139,#41140,#41141,#41142,#41143,#41144,#41145,
#41146,#41147,#41148,#41149,#41150,#41151,#41152,#41153,#41154,#41155,#41156,
#41157,#41158,#41159,#41160,#41161,#41162,#41163,#41164,#41165,#41166,#41167,
#41168,#41169,#41170,#41171,#41172,#41173,#41174,#41175,#41176,#41177,#41178,
#41179,#41180,#41181,#41182,#41183,#41184,#41185,#41186,#41187,#41188,#41189,
#41190,#41191,#41192,#41193,#41194,#41195,#41196,#41197,#41198,#41199,#41200,
#41201,#41202,#41203,#41204,#41205,#41206,#41207,#41208,#41209,#41210,#41211,
#41212,#41213,#41214,#41215,#41216,#41217,#41218,#41219,#41220,#41221,#41222,
#41223,#41224,#41225,#41226,#41227,#41228,#41229,#41230,#41231,#41232,#41233,
#41234,#41235,#41236,#41237,#41238,#41239,#41240,#41241,#41242,#41243,#41244,
#41245,#41246,#41247,#41248,#41249,#41250,#41251,#41252,#41253,#41254,#41255,
#41256,#41257,#41258,#41259,#41260,#41261),(#41262,#41263,#41264,#41265,
#41266,#41267,#41268,#41269,#41270,#41271,#41272,#41273,#41274,#41275,#41276,
#41277,#41278,#41279,#41280,#41281,#41282,#41283,#41284,#41285,#41286,#41287,
#41288,#41289,#41290,#41291,#41292,#41293,#41294,#41295,#41296,#41297,#41298,
#41299,#41300,#41301,#41302,#41303,#41304,#41305,#41306,#41307,#41308,#41309,
#41310,#41311,#41312,#41313,#41314,#41315,#41316,#41317,#41318,#41319,#41320,
#41321,#41322,#41323,#41324,#41325,#41326,#41327,#41328,#41329,#41330,#41331,
#41332,#41333,#41334,#41335,#41336,#41337,#41338,#41339,#41340,#41341,#41342,
#41343,#41344,#41345,#41346,#41347,#41348,#41349,#41350,#41351,#41352,#41353,
#41354,#41355,#41356,#41357,#41358,#41359,#41360,#41361,#41362,#41363,#41364,
#41365,#41366,#41367,#41368,#41369,#41370,#41371,#41372,#41373,#41374,#41375,
#41376,#41377,#41378,#41379,#41380,#41381,#41382,#41383,#41384,#41385,#41386,
#41387,#41388,#41389,#41390,#41391,#41392,#41393,#41394,#41395,#41396,#41397,
#41398,#41399,#41400,#41401,#41402,#41403,#41404,#41405,#41406,#41407,#41408,
#41409,#41410,#41411,#41412,#41413,#41414,#41415,#41416,#41417,#41418)),
 .UNSPECIFIED.,.F.,.F.,.F.,(4,4),(4,1,1,1,1,1,1,1,1,1,1,1,1,1,1,1,1,1,1,
1,1,1,1,1,1,1,1,1,1,1,1,1,1,1,1,1,1,1,1,1,1,1,1,1,1,1,1,1,1,1,1,1,1,1,1,
1,1,1,1,1,1,1,1,1,1,1,1,1,1,1,1,1,1,1,1,1,1,1,1,1,1,1,1,1,1,1,1,1,1,1,1,
1,1,1,1,1,1,1,1,1,1,1,1,1,1,1,1,1,1,1,1,1,1,1,1,1,1,1,1,1,1,1,1,1,1,1,1,
1,1,1,1,1,1,1,1,1,1,1,1,1,1,1,1,1,1,1,1,1,1,1,1,1,1,1,4),(-0.000414828532079457,
0.0529939397069977),(8.30815772716272,9.30587489071033,10.3035920542579,
11.3013092178055,12.2990263813532,13.2967435449008,14.2944607084484,15.292177871996,
16.2898950355436,17.2876121990912,18.2853293626388,19.2830465261864,20.280763689734,
21.2784808532816,22.2761980168293,23.2739151803769,24.2716323439245,25.2693495074721,
26.2670666710197,27.2647838345673,28.2625009981149,29.2602181616625,30.2579353252101,
31.2556524887577,32.2533696523054,33.251086815853,34.2488039794006,35.2465211429482,
36.2442383064958,37.2419554700434,38.239672633591,39.2373897971386,40.2351069606862,
41.2328241242338,42.2305412877814,43.2282584513291,44.2259756148767,45.2236927784243,
46.2214099419719,47.2191271055195,48.2168442690671,49.2145614326147,50.2122785961623,
51.2099957597099,52.2077129232575,53.2054300868052,54.2031472503528,55.2008644139004,
56.198581577448,57.1962987409956,58.1940159045432,59.1917330680908,60.1894502316384,
61.187167395186,62.1848845587336,63.1826017222812,64.1803188858289,65.1780360493765,
66.1757532129241,67.1734703764717,68.1711875400193,69.1689047035669,70.1666218671145,
71.1643390306621,72.1620561942097,73.1597733577573,74.157490521305,75.1552076848526,
76.1529248484002,77.1506420119478,78.1483591754954,79.146076339043,80.1437935025906,
81.1415106661382,82.1392278296858,83.1369449932334,84.1346621567811,85.1323793203287,
86.1300964838763,87.1278136474239,88.1255308109715,89.1232479745191,90.1209651380667,
91.1186823016143,92.1163994651619,93.1141166287095,94.1118337922572,95.1095509558048,
96.1072681193524,97.1049852829,98.1027024464476,99.1004196099952,100.098136773543,
101.09585393709,102.093571100638,103.091288264186,104.089005427733,105.086722591281,
106.084439754828,107.082156918376,108.079874081924,109.077591245471,110.075308409019,
111.073025572567,112.070742736114,113.068459899662,114.066177063209,115.063894226757,
116.061611390305,117.059328553852,118.0570457174,119.054762880947,120.052480044495,
121.050197208043,122.04791437159,123.045631535138,124.043348698685,125.041065862233,
126.038783025781,127.036500189328,128.034217352876,129.031934516423,130.029651679971,
131.027368843519,132.025086007066,133.022803170614,134.020520334162,135.018237497709,
136.015954661257,137.013671824804,138.011388988352,139.0091061519,140.006823315447,
141.004540478995,142.002257642542,142.99997480609,143.997691969638,144.995409133185,
145.993126296733,146.99084346028,147.988560623828,148.986277787376,149.983994950923,
150.981712114471,151.979429278019,152.977146441566,153.974863605114,154.972580768661,
155.970297932209,156.968015095757,157.965732259304,158.963449422852,159.961166586399,
160.958883749947,161.957015742027),.UNSPECIFIED.);
#365=B_SPLINE_SURFACE_WITH_KNOTS('',3,3,((#41606,#41607,#41608,#41609,#41610,
#41611,#41612,#41613,#41614,#41615,#41616,#41617,#41618,#41619,#41620,#41621,
#41622,#41623,#41624,#41625,#41626,#41627,#41628,#41629,#41630,#41631,#41632,
#41633,#41634,#41635,#41636,#41637,#41638,#41639,#41640,#41641,#41642,#41643,
#41644,#41645,#41646,#41647,#41648,#41649,#41650,#41651,#41652,#41653,#41654,
#41655,#41656,#41657,#41658,#41659,#41660,#41661,#41662,#41663,#41664,#41665,
#41666,#41667,#41668,#41669,#41670,#41671,#41672,#41673,#41674,#41675,#41676,
#41677,#41678,#41679,#41680,#41681,#41682,#41683,#41684,#41685,#41686,#41687,
#41688,#41689,#41690,#41691,#41692,#41693,#41694,#41695,#41696,#41697,#41698,
#41699,#41700,#41701,#41702,#41703,#41704,#41705,#41706,#41707,#41708,#41709,
#41710,#41711,#41712,#41713,#41714,#41715,#41716,#41717,#41718,#41719,#41720,
#41721,#41722,#41723,#41724,#41725,#41726,#41727,#41728,#41729,#41730,#41731,
#41732,#41733,#41734,#41735,#41736,#41737,#41738,#41739,#41740,#41741,#41742,
#41743,#41744,#41745,#41746,#41747,#41748,#41749,#41750,#41751,#41752,#41753,
#41754,#41755,#41756,#41757,#41758,#41759,#41760,#41761,#41762),(#41763,
#41764,#41765,#41766,#41767,#41768,#41769,#41770,#41771,#41772,#41773,#41774,
#41775,#41776,#41777,#41778,#41779,#41780,#41781,#41782,#41783,#41784,#41785,
#41786,#41787,#41788,#41789,#41790,#41791,#41792,#41793,#41794,#41795,#41796,
#41797,#41798,#41799,#41800,#41801,#41802,#41803,#41804,#41805,#41806,#41807,
#41808,#41809,#41810,#41811,#41812,#41813,#41814,#41815,#41816,#41817,#41818,
#41819,#41820,#41821,#41822,#41823,#41824,#41825,#41826,#41827,#41828,#41829,
#41830,#41831,#41832,#41833,#41834,#41835,#41836,#41837,#41838,#41839,#41840,
#41841,#41842,#41843,#41844,#41845,#41846,#41847,#41848,#41849,#41850,#41851,
#41852,#41853,#41854,#41855,#41856,#41857,#41858,#41859,#41860,#41861,#41862,
#41863,#41864,#41865,#41866,#41867,#41868,#41869,#41870,#41871,#41872,#41873,
#41874,#41875,#41876,#41877,#41878,#41879,#41880,#41881,#41882,#41883,#41884,
#41885,#41886,#41887,#41888,#41889,#41890,#41891,#41892,#41893,#41894,#41895,
#41896,#41897,#41898,#41899,#41900,#41901,#41902,#41903,#41904,#41905,#41906,
#41907,#41908,#41909,#41910,#41911,#41912,#41913,#41914,#41915,#41916,#41917,
#41918,#41919),(#41920,#41921,#41922,#41923,#41924,#41925,#41926,#41927,
#41928,#41929,#41930,#41931,#41932,#41933,#41934,#41935,#41936,#41937,#41938,
#41939,#41940,#41941,#41942,#41943,#41944,#41945,#41946,#41947,#41948,#41949,
#41950,#41951,#41952,#41953,#41954,#41955,#41956,#41957,#41958,#41959,#41960,
#41961,#41962,#41963,#41964,#41965,#41966,#41967,#41968,#41969,#41970,#41971,
#41972,#41973,#41974,#41975,#41976,#41977,#41978,#41979,#41980,#41981,#41982,
#41983,#41984,#41985,#41986,#41987,#41988,#41989,#41990,#41991,#41992,#41993,
#41994,#41995,#41996,#41997,#41998,#41999,#42000,#42001,#42002,#42003,#42004,
#42005,#42006,#42007,#42008,#42009,#42010,#42011,#42012,#42013,#42014,#42015,
#42016,#42017,#42018,#42019,#42020,#42021,#42022,#42023,#42024,#42025,#42026,
#42027,#42028,#42029,#42030,#42031,#42032,#42033,#42034,#42035,#42036,#42037,
#42038,#42039,#42040,#42041,#42042,#42043,#42044,#42045,#42046,#42047,#42048,
#42049,#42050,#42051,#42052,#42053,#42054,#42055,#42056,#42057,#42058,#42059,
#42060,#42061,#42062,#42063,#42064,#42065,#42066,#42067,#42068,#42069,#42070,
#42071,#42072,#42073,#42074,#42075,#42076),(#42077,#42078,#42079,#42080,
#42081,#42082,#42083,#42084,#42085,#42086,#42087,#42088,#42089,#42090,#42091,
#42092,#42093,#42094,#42095,#42096,#42097,#42098,#42099,#42100,#42101,#42102,
#42103,#42104,#42105,#42106,#42107,#42108,#42109,#42110,#42111,#42112,#42113,
#42114,#42115,#42116,#42117,#42118,#42119,#42120,#42121,#42122,#42123,#42124,
#42125,#42126,#42127,#42128,#42129,#42130,#42131,#42132,#42133,#42134,#42135,
#42136,#42137,#42138,#42139,#42140,#42141,#42142,#42143,#42144,#42145,#42146,
#42147,#42148,#42149,#42150,#42151,#42152,#42153,#42154,#42155,#42156,#42157,
#42158,#42159,#42160,#42161,#42162,#42163,#42164,#42165,#42166,#42167,#42168,
#42169,#42170,#42171,#42172,#42173,#42174,#42175,#42176,#42177,#42178,#42179,
#42180,#42181,#42182,#42183,#42184,#42185,#42186,#42187,#42188,#42189,#42190,
#42191,#42192,#42193,#42194,#42195,#42196,#42197,#42198,#42199,#42200,#42201,
#42202,#42203,#42204,#42205,#42206,#42207,#42208,#42209,#42210,#42211,#42212,
#42213,#42214,#42215,#42216,#42217,#42218,#42219,#42220,#42221,#42222,#42223,
#42224,#42225,#42226,#42227,#42228,#42229,#42230,#42231,#42232,#42233)),
 .UNSPECIFIED.,.F.,.F.,.F.,(4,4),(4,1,1,1,1,1,1,1,1,1,1,1,1,1,1,1,1,1,1,
1,1,1,1,1,1,1,1,1,1,1,1,1,1,1,1,1,1,1,1,1,1,1,1,1,1,1,1,1,1,1,1,1,1,1,1,
1,1,1,1,1,1,1,1,1,1,1,1,1,1,1,1,1,1,1,1,1,1,1,1,1,1,1,1,1,1,1,1,1,1,1,1,
1,1,1,1,1,1,1,1,1,1,1,1,1,1,1,1,1,1,1,1,1,1,1,1,1,1,1,1,1,1,1,1,1,1,1,1,
1,1,1,1,1,1,1,1,1,1,1,1,1,1,1,1,1,1,1,1,1,1,1,1,1,1,1,4),(-0.000352467397055627,
0.053040310820889),(11.6159783635572,12.6141103608891,13.6118275244367,
14.6095446879844,15.607261851532,16.6049790150796,17.6026961786272,18.6004133421748,
19.5981305057224,20.59584766927,21.5935648328176,22.5912819963652,23.5889991599128,
24.5867163234605,25.5844334870081,26.5821506505557,27.5798678141033,28.5775849776509,
29.5753021411985,30.5730193047461,31.5707364682937,32.5684536318413,33.5661707953889,
34.5638879589366,35.5616051224842,36.5593222860318,37.5570394495794,38.554756613127,
39.5524737766746,40.5501909402222,41.5479081037698,42.5456252673174,43.543342430865,
44.5410595944127,45.5387767579603,46.5364939215079,47.5342110850555,48.5319282486031,
49.5296454121507,50.5273625756983,51.5250797392459,52.5227969027935,53.5205140663411,
54.5182312298887,55.5159483934364,56.513665556984,57.5113827205316,58.5090998840792,
59.5068170476268,60.5045342111744,61.502251374722,62.4999685382696,63.4976857018172,
64.4954028653649,65.4931200289125,66.4908371924601,67.4885543560077,68.4862715195553,
69.4839886831029,70.4817058466505,71.4794230101981,72.4771401737457,73.4748573372933,
74.4725745008409,75.4702916643886,76.4680088279362,77.4657259914838,78.4634431550314,
79.461160318579,80.4588774821266,81.4565946456742,82.4543118092218,83.4520289727694,
84.449746136317,85.4474632998647,86.4451804634123,87.4428976269599,88.4406147905075,
89.4383319540551,90.4360491176027,91.4337662811503,92.4314834446979,93.4292006082455,
94.4269177717931,95.4246349353407,96.4223520988884,97.420069262436,98.4177864259836,
99.4155035895312,100.413220753079,101.410937916626,102.408655080174,103.406372243722,
104.404089407269,105.401806570817,106.399523734364,107.397240897912,108.39495806146,
109.392675225007,110.390392388555,111.388109552103,112.38582671565,113.383543879198,
114.381261042745,115.378978206293,116.376695369841,117.374412533388,118.372129696936,
119.369846860483,120.367564024031,121.365281187579,122.362998351126,123.360715514674,
124.358432678221,125.356149841769,126.353867005317,127.351584168864,128.349301332412,
129.34701849596,130.344735659507,131.342452823055,132.340169986602,133.33788715015,
134.335604313698,135.333321477245,136.331038640793,137.32875580434,138.326472967888,
139.324190131436,140.321907294983,141.319624458531,142.317341622078,143.315058785626,
144.312775949174,145.310493112721,146.308210276269,147.305927439816,148.303644603364,
149.301361766912,150.299078930459,151.296796094007,152.294513257555,153.292230421102,
154.28994758465,155.287664748197,156.285381911745,157.283099075293,158.28081623884,
159.278533402388,160.276250565935,161.273967729483,162.271684893031,163.269402056578,
164.267119220126,165.264836383673),.UNSPECIFIED.);
#408=B_SPLINE_CURVE_WITH_KNOTS('',3,(#23040,#23041,#23042,#23043,#23044,
#23045,#23046,#23047,#23048,#23049,#23050,#23051,#23052,#23053,#23054,#23055,
#23056,#23057,#23058,#23059,#23060,#23061,#23062,#23063,#23064,#23065,#23066,
#23067,#23068,#23069,#23070,#23071,#23072,#23073,#23074,#23075,#23076,#23077,
#23078,#23079,#23080,#23081,#23082,#23083,#23084,#23085,#23086,#23087,#23088,
#23089,#23090,#23091,#23092,#23093,#23094,#23095,#23096,#23097,#23098,#23099,
#23100,#23101,#23102,#23103,#23104,#23105,#23106,#23107,#23108,#23109,#23110,
#23111,#23112,#23113,#23114,#23115,#23116,#23117,#23118,#23119,#23120,#23121,
#23122,#23123,#23124,#23125,#23126,#23127,#23128,#23129,#23130,#23131,#23132,
#23133,#23134,#23135,#23136,#23137,#23138,#23139,#23140,#23141,#23142,#23143,
#23144,#23145,#23146,#23147,#23148,#23149,#23150,#23151,#23152,#23153,#23154,
#23155,#23156,#23157,#23158,#23159,#23160,#23161,#23162,#23163,#23164,#23165,
#23166,#23167,#23168,#23169,#23170,#23171,#23172,#23173,#23174,#23175,#23176,
#23177,#23178,#23179,#23180,#23181,#23182,#23183,#23184,#23185,#23186,#23187,
#23188,#23189,#23190,#23191,#23192,#23193,#23194,#23195,#23196,#23197),
 .UNSPECIFIED.,.F.,.F.,(4,2,2,2,2,2,2,2,2,2,2,2,2,2,2,2,2,2,2,2,2,2,2,2,
2,2,2,2,2,2,2,2,2,2,2,2,2,2,2,2,2,2,2,2,2,2,2,2,2,2,2,2,2,2,2,2,2,2,2,2,
2,2,2,2,2,2,2,2,2,2,2,2,2,2,2,2,2,2,4),(-0.736675210638058,-0.733821596808743,
-0.694292033914328,-0.689636306082269,-0.686738441869285,-0.684478224512377,
-0.68197459732431,-0.677843159020972,-0.662315926433236,-0.609673816667036,
-0.60542480610492,-0.590249017300808,-0.587646734993429,-0.58603249381003,
-0.584775927897407,-0.583320803513858,-0.580700810859027,-0.567619048230907,
-0.498749414458695,-0.490687875993121,-0.487355526501576,-0.485269466399629,
-0.482983111861107,-0.47981466001079,-0.472190340759041,-0.461503343415649,
-0.402687458406344,-0.390008334220899,-0.387544858158691,-0.385977168728162,
-0.38472244088543,-0.383223865036566,-0.380442637090082,-0.364403892819621,
-0.310894446169308,-0.293090695693202,-0.288631625129639,-0.286024966281755,
-0.283770737027648,-0.281009047858853,-0.27569948623136,-0.268986738050613,
-0.253669224173961,-0.215639415702403,-0.191097914207698,-0.187984675517241,
-0.186403617887784,-0.185150735660367,-0.185140371720751,-0.185130377235419,
-0.185120735762252,-0.185111431649632,-0.185102450266112,-0.185093777770031,
-0.185085401014474,-0.185077307521438,-0.185069485549634,-0.185061923946848,
-0.185054612044751,-0.185047539936342,-0.1850406980958,-0.185032579111707,
-0.185024517471098,-0.185016512188063,-0.185008562278368,-0.185000666664865,
-0.184992824418986,-0.183459446820892,-0.180515474988828,-0.161220776772221,
-0.119046916699663,-0.0967044542819805,-0.0923424843568188,-0.0895154180428306,
-0.087237298885081,-0.0846349927311359,-0.0801453807302738,-0.0602832274206637,
-0.00330615950253142),.UNSPECIFIED.);
#409=B_SPLINE_CURVE_WITH_KNOTS('',3,(#23200,#23201,#23202,#23203,#23204,
#23205,#23206,#23207,#23208,#23209,#23210,#23211,#23212,#23213,#23214,#23215,
#23216,#23217,#23218,#23219,#23220,#23221,#23222,#23223,#23224,#23225,#23226,
#23227,#23228,#23229,#23230,#23231,#23232,#23233,#23234,#23235,#23236,#23237,
#23238,#23239,#23240,#23241,#23242,#23243,#23244,#23245,#23246,#23247,#23248,
#23249,#23250,#23251,#23252,#23253,#23254,#23255,#23256,#23257,#23258,#23259,
#23260,#23261,#23262,#23263,#23264,#23265,#23266,#23267,#23268,#23269,#23270,
#23271,#23272,#23273,#23274,#23275),.UNSPECIFIED.,.F.,.F.,(4,3,3,3,3,3,
3,3,3,3,3,3,3,3,3,3,3,3,3,3,3,3,3,3,3,4),(11.6163931973415,11.7237492295633,
11.835044370979,11.9423196466468,12.049596139851,12.156902775469,12.2642685060456,
12.371800331433,12.4794284226994,12.5872559860832,12.6141103608891,12.7180831030621,
12.8218829433769,12.9255411761381,13.0291226045906,13.1326641607794,13.2362027194087,
13.3398462288228,13.4435459699825,13.5474312704339,13.6118275244367,13.7169098947458,
13.8218092643123,13.9266035018259,14.0313222763496,14.054777935193),
 .UNSPECIFIED.);
#410=B_SPLINE_CURVE_WITH_KNOTS('',3,(#23280,#23281,#23282,#23283,#23284,
#23285,#23286,#23287,#23288,#23289,#23290,#23291,#23292,#23293,#23294,#23295,
#23296,#23297,#23298,#23299,#23300,#23301,#23302,#23303,#23304,#23305,#23306,
#23307,#23308,#23309,#23310,#23311,#23312,#23313,#23314,#23315,#23316,#23317,
#23318,#23319,#23320,#23321,#23322,#23323,#23324,#23325,#23326,#23327,#23328,
#23329,#23330,#23331,#23332,#23333,#23334,#23335,#23336,#23337,#23338,#23339,
#23340,#23341,#23342,#23343,#23344,#23345,#23346,#23347,#23348,#23349,#23350,
#23351,#23352,#23353,#23354,#23355,#23356,#23357,#23358,#23359,#23360,#23361,
#23362,#23363,#23364,#23365,#23366,#23367,#23368,#23369,#23370,#23371,#23372,
#23373,#23374,#23375,#23376,#23377,#23378,#23379,#23380,#23381,#23382,#23383,
#23384,#23385,#23386,#23387,#23388,#23389,#23390,#23391,#23392,#23393,#23394,
#23395,#23396,#23397,#23398,#23399,#23400,#23401,#23402,#23403,#23404,#23405,
#23406,#23407,#23408,#23409,#23410,#23411,#23412,#23413,#23414,#23415,#23416,
#23417,#23418,#23419,#23420,#23421,#23422,#23423,#23424,#23425,#23426,#23427,
#23428,#23429,#23430,#23431,#23432,#23433,#23434,#23435,#23436,#23437,#23438,
#23439,#23440,#23441,#23442,#23443,#23444,#23445,#23446,#23447,#23448,#23449,
#23450,#23451,#23452,#23453,#23454,#23455,#23456,#23457,#23458,#23459,#23460,
#23461,#23462,#23463,#23464,#23465,#23466,#23467,#23468,#23469,#23470,#23471,
#23472,#23473,#23474,#23475,#23476,#23477,#23478,#23479,#23480,#23481,#23482,
#23483,#23484,#23485,#23486,#23487,#23488,#23489,#23490,#23491,#23492,#23493,
#23494,#23495,#23496,#23497,#23498,#23499,#23500,#23501),.UNSPECIFIED.,
 .F.,.F.,(4,2,2,2,2,2,2,2,2,2,2,2,2,2,2,2,2,2,2,2,2,2,2,2,2,2,2,2,2,2,2,
2,2,2,2,2,2,2,2,2,2,2,2,2,2,2,2,2,2,2,2,2,2,2,2,2,2,2,2,2,2,2,2,2,2,2,2,
2,2,2,2,2,2,2,2,2,2,2,2,2,2,2,2,2,2,2,2,2,2,2,2,2,2,2,2,2,2,2,2,2,2,2,2,
2,2,2,2,2,2,2,4),(-1.99319254965038,-1.98653737002634,-1.98379876219187,
-1.98231127336989,-1.98105390575671,-1.97946774020603,-1.97695764114924,
-1.96358609747753,-1.95947365261895,-1.91009979267965,-1.88997447752518,
-1.8855124399241,-1.88293983892923,-1.88069627497894,-1.87792368335606,
-1.87366964594137,-1.85263256574772,-1.80271668913237,-1.79220829787831,
-1.7878977864728,-1.78462777973597,-1.78303063756752,-1.78177262317214,
-1.78029379898174,-1.77766847778042,-1.76624504842418,-1.72805574524784,
-1.69152579643256,-1.68645760565609,-1.68375522131271,-1.68173376564286,
-1.67918575318431,-1.67483532908617,-1.65877935779111,-1.6037048732393,
-1.58756341620945,-1.5847825791044,-1.583286052845,-1.58202929210908,-1.58045430170204,
-1.57798093406084,-1.56527370394193,-1.55688098194784,-1.50556565384859,
-1.49022978933833,-1.48612066592295,-1.48362540409227,-1.48136947813647,
-1.47847265369504,-1.47380975113612,-1.44015465221223,-1.41430436279017,
-1.3907709908021,-1.38618570486933,-1.38435473181944,-1.383063591166,-1.38186692765178,
-1.38018734647392,-1.37572966665698,-1.33404109191877,-1.29299639046651,
-1.28762830059024,-1.28486300891597,-1.28261920610225,-1.28003953442239,
-1.27566305997605,-1.25870238180554,-1.20068310336964,-1.18819100667183,
-1.18559107374171,-1.18413335063411,-1.18287330707974,-1.18124711843356,
-1.17860182329707,-1.16243375888946,-1.10376929772002,-1.09093020651619,
-1.08691406550062,-1.08444070426442,-1.08218190750236,-1.07924926338534,
-1.07302093646664,-1.03972953816717,-1.0098835930594,-1.00216406863422,
-0.988916655393418,-0.986414427156384,-0.984831290152103,-0.983574602856247,
-0.982085784279071,-0.979340969979418,-0.964033763220833,-0.917227233395081,
-0.892981609427976,-0.888570353940284,-0.885748892048188,-0.883500284903431,
-0.880958973937785,-0.876643557614502,-0.858725039011845,-0.8120316403843,
-0.810317698066935,-0.80146037094138,-0.789266527434246,-0.786821851193486,
-0.785254625932403,-0.783995157677338,-0.782484136198523,-0.779651271266861,
-0.762365581868955,-0.736675210638058),.UNSPECIFIED.);
#411=B_SPLINE_CURVE_WITH_KNOTS('',3,(#23503,#23504,#23505,#23506,#23507,
#23508,#23509,#23510,#23511,#23512,#23513,#23514,#23515,#23516,#23517,#23518,
#23519,#23520,#23521,#23522,#23523,#23524,#23525,#23526,#23527,#23528,#23529,
#23530,#23531,#23532,#23533,#23534,#23535,#23536,#23537,#23538,#23539,#23540,
#23541,#23542,#23543,#23544,#23545,#23546,#23547,#23548,#23549,#23550,#23551,
#23552,#23553,#23554),.UNSPECIFIED.,.F.,.F.,(4,3,3,3,3,3,3,3,3,3,3,3,3,
3,3,3,3,4),(14.054777935193,14.1594700099767,14.2641741224379,14.3689912503651,
14.4738754371146,14.5789317449399,14.6095446879844,14.7146790594763,14.8196597064566,
14.9245217842077,15.0293208169872,15.1340920802013,15.2388708079724,15.3437622025241,
15.4487162544608,15.5538525389373,15.607261851532,15.707963267949),
 .UNSPECIFIED.);
#412=B_SPLINE_CURVE_WITH_KNOTS('',3,(#23555,#23556,#23557,#23558,#23559,
#23560,#23561,#23562,#23563,#23564,#23565,#23566,#23567,#23568,#23569,#23570,
#23571,#23572,#23573,#23574,#23575,#23576,#23577,#23578,#23579,#23580,#23581,
#23582,#23583,#23584,#23585,#23586,#23587,#23588,#23589,#23590,#23591,#23592,
#23593,#23594,#23595,#23596,#23597,#23598,#23599,#23600,#23601,#23602,#23603,
#23604,#23605,#23606,#23607,#23608,#23609,#23610,#23611,#23612,#23613,#23614,
#23615,#23616,#23617,#23618,#23619,#23620,#23621,#23622,#23623,#23624,#23625,
#23626,#23627,#23628,#23629,#23630,#23631,#23632,#23633,#23634,#23635,#23636,
#23637,#23638,#23639,#23640,#23641,#23642,#23643,#23644,#23645,#23646,#23647,
#23648,#23649,#23650,#23651,#23652,#23653,#23654,#23655,#23656,#23657,#23658,
#23659,#23660,#23661,#23662,#23663,#23664,#23665,#23666,#23667,#23668,#23669,
#23670,#23671,#23672,#23673,#23674,#23675,#23676,#23677,#23678,#23679,#23680,
#23681,#23682,#23683,#23684,#23685,#23686,#23687,#23688,#23689,#23690,#23691,
#23692,#23693,#23694,#23695,#23696,#23697,#23698,#23699,#23700,#23701,#23702,
#23703,#23704,#23705,#23706,#23707,#23708,#23709,#23710,#23711,#23712,#23713,
#23714),.UNSPECIFIED.,.F.,.F.,(4,2,2,2,2,2,2,2,2,2,2,2,2,2,2,2,2,2,2,2,
2,2,2,2,2,2,2,2,2,2,2,2,2,2,2,2,2,2,2,2,2,2,2,2,2,2,2,2,2,2,2,2,2,2,2,2,
2,2,2,2,2,2,2,2,2,2,2,2,2,2,2,2,2,2,2,2,2,2,2,4),(-2.51428340140175,-2.5075761767229,
-2.45683770840886,-2.44694558480235,-2.43976138139802,-2.43666717087808,
-2.43439424280313,-2.43229232245576,-2.42942596561606,-2.42222426557208,
-2.37875002873089,-2.35254832993181,-2.34360277058353,-2.33975515706998,
-2.33763316598838,-2.33579391733833,-2.33452171846559,-2.33334371170081,
-2.33142428110962,-2.32662747627728,-2.29536552386702,-2.26894776642379,
-2.24547788033084,-2.23934453969068,-2.23642506127349,-2.23416264487136,
-2.23167141480239,-2.22759445232846,-2.21427158911533,-2.1564453148252,
-2.14010421221288,-2.13730832658454,-2.13580526270536,-2.13454558661861,
-2.13296942338265,-2.12990975131705,-2.10887285789977,-2.05788040819895,
-2.04275310843614,-2.03866156407082,-2.03616971049145,-2.03391216218611,
-2.03100666744326,-2.02631629293022,-1.98971337666585,-1.95395538417286,
-1.94029352616069,-1.93762888225658,-1.93615744135929,-1.93489938813596,
-1.93329387424094,-1.93071738003684,-1.9161173043658,-1.8943178333712,-1.86074202471722,
-1.84349754275835,-1.83923594398317,-1.83670871473161,-1.83446173565513,
-1.83162783997351,-1.82716877083037,-1.8015579920678,-1.76511576577924,
-1.74342876761541,-1.73902692727964,-1.73722685757312,-1.73594237209019,
-1.73457089489806,-1.7323601738389,-1.72554131716868,-1.68365381660965,
-1.66232755257428,-1.64407877699645,-1.63974031220367,-1.63719430830286,
-1.63494695966009,-1.63213425033871,-1.62775052475623,-1.60421127678611,
-1.58825468741526),.UNSPECIFIED.);
#413=B_SPLINE_CURVE_WITH_KNOTS('',3,(#23720,#23721,#23722,#23723,#23724,
#23725,#23726,#23727,#23728,#23729,#23730,#23731,#23732,#23733,#23734,#23735,
#23736,#23737,#23738,#23739,#23740,#23741,#23742,#23743,#23744,#23745,#23746,
#23747,#23748,#23749,#23750,#23751,#23752,#23753,#23754,#23755,#23756,#23757,
#23758,#23759,#23760,#23761,#23762,#23763,#23764,#23765,#23766,#23767,#23768,
#23769,#23770,#23771,#23772,#23773,#23774,#23775,#23776,#23777,#23778,#23779,
#23780,#23781,#23782,#23783,#23784,#23785,#23786,#23787,#23788,#23789,#23790,
#23791,#23792,#23793,#23794,#23795,#23796,#23797,#23798,#23799,#23800,#23801,
#23802,#23803,#23804,#23805,#23806,#23807,#23808,#23809,#23810,#23811,#23812,
#23813,#23814,#23815,#23816,#23817,#23818,#23819,#23820,#23821,#23822,#23823,
#23824,#23825,#23826,#23827,#23828,#23829,#23830,#23831,#23832,#23833,#23834,
#23835,#23836,#23837,#23838,#23839,#23840,#23841,#23842,#23843,#23844,#23845,
#23846,#23847,#23848,#23849,#23850,#23851,#23852,#23853,#23854,#23855,#23856,
#23857,#23858,#23859,#23860,#23861,#23862,#23863,#23864,#23865,#23866,#23867,
#23868,#23869,#23870,#23871,#23872,#23873,#23874,#23875,#23876,#23877,#23878,
#23879),.UNSPECIFIED.,.F.,.F.,(4,2,2,2,2,2,2,2,2,2,2,2,2,2,2,2,2,2,2,2,
2,2,2,2,2,2,2,2,2,2,2,2,2,2,2,2,2,2,2,2,2,2,2,2,2,2,2,2,2,2,2,2,2,2,2,2,
2,2,2,2,2,2,2,2,2,2,2,2,2,2,2,2,2,2,2,2,2,2,2,4),(-0.926471073029744,-0.901398759294761,
-0.863449560271604,-0.8587761697636,-0.856877258545011,-0.85570281277469,
-0.854390777529996,-0.852453661213017,-0.847162662369924,-0.839085288849207,
-0.785971877562881,-0.777057598575648,-0.763193976411606,-0.75906279309083,
-0.75656269366143,-0.75430788109391,-0.751420113184561,-0.745434473064014,
-0.701439480574167,-0.663919966451118,-0.65922739160026,-0.657325276204849,
-0.656150248169787,-0.654838926037188,-0.652905234628083,-0.647638216958983,
-0.639610055216725,-0.58732950151616,-0.578277266020182,-0.563770046930224,
-0.559571489157056,-0.557056546905337,-0.555029930440796,-0.552279559627591,
-0.546982047577972,-0.540281886959943,-0.524985634153146,-0.487492707266087,
-0.462041993179969,-0.458914167666053,-0.45732445647121,-0.456066807200957,
-0.45458193471129,-0.451855905147516,-0.436961198923767,-0.393353239812336,
-0.365760600957839,-0.361234075326173,-0.358378298953241,-0.356127120693537,
-0.353608895514417,-0.349395326665183,-0.332804041632327,-0.269379222595975,
-0.261094679575136,-0.258714976427778,-0.257305711512071,-0.256034303932594,
-0.254320957608614,-0.250434290240936,-0.245054712240226,-0.230482217332864,
-0.180040824463748,-0.164788409045415,-0.160515653588025,-0.157984118036114,
-0.155959670457389,-0.153814290875608,-0.149684335246355,-0.132747892627418,
-0.104663709423388,-0.0651145466777724,-0.0605245248097448,-0.0586393776065246,
-0.0573507265026836,-0.0560085391993869,-0.0539314083632888,-0.0514996293803942,
-0.046843274153505,-0.000589973186885262),.UNSPECIFIED.);
#414=B_SPLINE_CURVE_WITH_KNOTS('',3,(#23880,#23881,#23882,#23883,#23884,
#23885,#23886,#23887,#23888,#23889,#23890,#23891,#23892,#23893,#23894,#23895,
#23896,#23897,#23898,#23899,#23900,#23901,#23902,#23903,#23904,#23905,#23906,
#23907,#23908,#23909,#23910,#23911,#23912,#23913,#23914,#23915,#23916,#23917,
#23918,#23919,#23920,#23921,#23922,#23923,#23924,#23925,#23926,#23927,#23928,
#23929,#23930,#23931,#23932,#23933,#23934,#23935,#23936,#23937,#23938,#23939),
 .UNSPECIFIED.,.F.,.F.,(4,2,2,2,2,2,2,2,2,2,2,2,2,2,2,2,2,2,2,2,2,2,2,2,
2,2,2,2,2,4),(-2.32386902743845,-2.30024041246414,-2.28982706294607,-2.28626771725673,
-2.28379755546917,-2.28169323369155,-2.27944215589424,-2.27658444578319,
-2.27205069880471,-2.24420995510776,-2.22185146770358,-2.20084557525772,
-2.18598778828631,-2.18325338576836,-2.18176690229588,-2.18050966000605,
-2.17892272561299,-2.17580707699489,-2.15134499037956,-2.1195743325545,
-2.1000265239033,-2.08816509482076,-2.0844248315671,-2.08231862587725,-2.0800700710637,
-2.07723710407267,-2.07278513444405,-2.04741796436327,-2.00170747490439,
-1.99319254965038),.UNSPECIFIED.);
#415=B_SPLINE_CURVE_WITH_KNOTS('',3,(#23940,#23941,#23942,#23943,#23944,
#23945,#23946,#23947,#23948,#23949,#23950,#23951,#23952,#23953,#23954,#23955,
#23956,#23957,#23958,#23959,#23960,#23961,#23962,#23963,#23964,#23965,#23966,
#23967,#23968,#23969,#23970,#23971,#23972,#23973,#23974,#23975,#23976,#23977,
#23978,#23979,#23980,#23981,#23982,#23983,#23984,#23985,#23986,#23987,#23988,
#23989,#23990,#23991,#23992,#23993,#23994,#23995,#23996,#23997,#23998,#23999,
#24000,#24001,#24002,#24003,#24004,#24005,#24006,#24007,#24008,#24009,#24010,
#24011,#24012,#24013,#24014,#24015,#24016,#24017,#24018,#24019,#24020,#24021,
#24022,#24023,#24024,#24025,#24026,#24027,#24028,#24029,#24030,#24031,#24032,
#24033,#24034,#24035,#24036,#24037,#24038,#24039,#24040,#24041,#24042,#24043,
#24044,#24045,#24046,#24047,#24048,#24049,#24050,#24051,#24052,#24053,#24054,
#24055,#24056,#24057,#24058,#24059,#24060,#24061,#24062,#24063,#24064,#24065,
#24066,#24067,#24068,#24069,#24070,#24071,#24072,#24073,#24074,#24075,#24076,
#24077,#24078,#24079,#24080,#24081,#24082,#24083,#24084,#24085,#24086,#24087,
#24088,#24089,#24090,#24091,#24092,#24093,#24094,#24095,#24096,#24097,#24098,
#24099,#24100,#24101,#24102,#24103,#24104,#24105,#24106,#24107,#24108,#24109,
#24110,#24111,#24112,#24113,#24114,#24115,#24116,#24117,#24118,#24119,#24120,
#24121,#24122,#24123,#24124,#24125,#24126,#24127,#24128,#24129,#24130,#24131,
#24132,#24133,#24134,#24135,#24136,#24137,#24138,#24139,#24140,#24141,#24142,
#24143,#24144,#24145,#24146,#24147,#24148,#24149,#24150,#24151),
 .UNSPECIFIED.,.F.,.F.,(4,2,2,2,2,2,2,2,2,2,2,2,2,2,2,2,2,2,2,2,2,2,2,2,
2,2,2,2,2,2,2,2,2,2,2,2,2,2,2,2,2,2,2,2,2,2,2,2,2,2,2,2,2,2,2,2,2,2,2,2,
2,2,2,2,2,2,2,2,2,2,2,2,2,2,2,2,2,2,2,2,2,2,2,2,2,2,2,2,2,2,2,2,2,2,2,2,
2,2,2,2,2,2,2,2,2,4),(-1.58825468741526,-1.55677506762686,-1.54139479875759,
-1.53864569877202,-1.53715547627514,-1.53589789844193,-1.53431399719557,
-1.53181158703341,-1.51858553333341,-1.46036439035829,-1.44421639674659,
-1.44003904369588,-1.43752901255672,-1.4352766705218,-1.43240780443973,
-1.42783719397291,-1.39873623119091,-1.35645497139845,-1.34174254908841,
-1.33902537677097,-1.33754258912259,-1.33628509220085,-1.33469355133465,
-1.33155601228223,-1.30476527817291,-1.25760534437154,-1.24442306199696,
-1.24036672110512,-1.23788355567592,-1.23562557886839,-1.23270783868223,
-1.22656355135345,-1.2029636011212,-1.17666026239359,-1.1454594412336,-1.14066498106173,
-1.13874619950042,-1.13756839240883,-1.13626106863574,-1.13434584666061,
-1.12920515949249,-1.099335148626,-1.04964048219559,-1.04338318364314,-1.04003650932242,
-1.03793804377308,-1.03563519696388,-1.0324382829047,-1.02471587082062,
-1.01386799284532,-0.952496209407458,-0.942316435553413,-0.939786839112411,
-0.938329715197559,-0.937080962753366,-0.935459307712926,-0.932064270962055,
-0.902850075623865,-0.851083944835811,-0.843539045504256,-0.840604468987905,
-0.838475751765444,-0.836195552509475,-0.833129397117509,-0.826177351757518,
-0.796164195035236,-0.765251952016309,-0.743697803607661,-0.740614769775796,
-0.739034717233685,-0.737777777429725,-0.736285594195263,-0.733524951392105,
-0.717856561959718,-0.667803722517626,-0.646912657506546,-0.642668709759187,
-0.639899310754679,-0.63765612011023,-0.63508152058239,-0.630609816994546,
-0.610327666667982,-0.559925052734969,-0.543811958200507,-0.541167496046246,
-0.539540907412971,-0.53828042250701,-0.536822407231302,-0.534220187814012,
-0.521681642425395,-0.462957025843696,-0.446684494953387,-0.442359922472271,
-0.439792878570727,-0.437548984029459,-0.434769297797808,-0.429327067146504,
-0.39206335072283,-0.3510844558689,-0.343160369793844,-0.340819935367345,
-0.339419677534822,-0.3381459957407,-0.33641512250523,-0.332427443485893,
-0.331363008767816),.UNSPECIFIED.);
#416=B_SPLINE_CURVE_WITH_KNOTS('',3,(#24156,#24157,#24158,#24159,#24160,
#24161,#24162,#24163,#24164,#24165,#24166,#24167,#24168,#24169,#24170,#24171,
#24172,#24173,#24174,#24175,#24176,#24177,#24178,#24179,#24180,#24181,#24182,
#24183,#24184,#24185,#24186,#24187,#24188,#24189,#24190,#24191,#24192,#24193,
#24194,#24195,#24196,#24197,#24198,#24199,#24200,#24201,#24202,#24203,#24204,
#24205,#24206,#24207,#24208,#24209,#24210,#24211,#24212,#24213,#24214,#24215,
#24216,#24217,#24218,#24219,#24220,#24221,#24222,#24223,#24224,#24225,#24226,
#24227,#24228,#24229,#24230,#24231,#24232,#24233,#24234,#24235,#24236,#24237,
#24238,#24239,#24240,#24241,#24242,#24243,#24244,#24245,#24246,#24247,#24248,
#24249,#24250,#24251,#24252,#24253,#24254,#24255,#24256,#24257,#24258,#24259,
#24260,#24261,#24262,#24263,#24264,#24265,#24266,#24267,#24268,#24269,#24270,
#24271,#24272,#24273,#24274,#24275,#24276,#24277,#24278,#24279,#24280,#24281,
#24282,#24283,#24284,#24285,#24286,#24287,#24288,#24289,#24290,#24291,#24292,
#24293,#24294,#24295,#24296,#24297,#24298,#24299,#24300,#24301,#24302,#24303,
#24304,#24305,#24306,#24307,#24308,#24309,#24310,#24311,#24312,#24313,#24314,
#24315,#24316,#24317,#24318,#24319,#24320,#24321,#24322,#24323,#24324,#24325,
#24326,#24327,#24328,#24329,#24330,#24331,#24332,#24333,#24334,#24335,#24336,
#24337,#24338,#24339,#24340,#24341,#24342,#24343,#24344,#24345,#24346,#24347,
#24348,#24349,#24350,#24351,#24352,#24353,#24354,#24355,#24356,#24357,#24358,
#24359,#24360,#24361,#24362,#24363,#24364,#24365,#24366,#24367,#24368,#24369,
#24370,#24371),.UNSPECIFIED.,.F.,.F.,(4,2,2,2,2,2,2,2,2,2,2,2,2,2,2,2,2,
2,2,2,2,2,2,2,2,2,2,2,2,2,2,2,2,2,2,2,2,2,2,2,2,2,2,2,2,2,2,2,2,2,2,2,2,
2,2,2,2,2,2,2,2,2,2,2,2,2,2,2,2,2,2,2,2,2,2,2,2,2,2,2,2,2,2,2,2,2,2,2,2,
2,2,2,2,2,2,2,2,2,2,2,2,2,2,2,2,2,2,4),(-2.18288930522275,-2.17834301383946,
-2.16020040172271,-2.15587072988079,-2.15332731439035,-2.1510806879597,
-2.14826681747001,-2.14387730153829,-2.1201523076371,-2.07288484499641,
-2.05752614137735,-2.05477918087068,-2.05328996736556,-2.05203287237048,
-2.05044923516515,-2.04794710130817,-2.03471863569996,-1.97652329525705,
-1.96038039200939,-1.95620379391468,-1.95369409432431,-1.9514419666657,
-1.94857325213857,-1.94400261283041,-1.91487487853451,-1.87265683400618,
-1.85795633725304,-1.85523983324506,-1.85375720853212,-1.85249967531851,
-1.85090784074904,-1.84776905670891,-1.82053844454068,-1.80702176300512,
-1.762770457098,-1.75754620130744,-1.75481133108086,-1.75278677223426,-1.75026235437542,
-1.74601912725718,-1.73107638943766,-1.72277035561684,-1.67406462991704,
-1.6585415000374,-1.65578724851468,-1.65429647179162,-1.65303948404066,
-1.65145778811473,-1.64836688534275,-1.61499255657007,-1.6073174439316,
-1.56316058746397,-1.55800618092379,-1.55528573064452,-1.55326253842361,
-1.55072773351432,-1.54643765807058,-1.53099284876732,-1.52359312990677,
-1.47079345239254,-1.46273356700672,-1.45745170533687,-1.4555160347539,
-1.45420441800844,-1.45302991697515,-1.45113012579219,-1.44645060936936,
-1.40879652980982,-1.37789096259205,-1.36733124129625,-1.35976588672558,
-1.35659469999181,-1.35429635296919,-1.35219233198252,-1.34935546633975,
-1.34239240660485,-1.29454086604358,-1.26039285948415,-1.25710430676926,
-1.25550345953941,-1.2542450605592,-1.2527686867682,-1.25008208414243,-1.23599879538802,
-1.20020177073284,-1.16420873192039,-1.15953052808974,-1.15662915048781,
-1.15437271942564,-1.15187998748226,-1.14778215559761,-1.13257488419503,
-1.08167177164236,-1.06058446385204,-1.05751334261323,-1.055935687434,-1.05467867073207,
-1.05318402170262,-1.05041255344463,-1.03449880251862,-0.981965032847736,
-0.963518796284954,-0.959029969321492,-0.956424982584346,-0.954183684597177,
-0.951452370623684,-0.946247010678033,-0.926471073029744),.UNSPECIFIED.);
#417=B_SPLINE_CURVE_WITH_KNOTS('',3,(#24373,#24374,#24375,#24376,#24377,
#24378,#24379,#24380,#24381,#24382,#24383,#24384,#24385,#24386,#24387,#24388,
#24389,#24390,#24391,#24392,#24393,#24394,#24395,#24396,#24397,#24398,#24399,
#24400,#24401,#24402,#24403,#24404,#24405,#24406,#24407,#24408,#24409,#24410,
#24411,#24412,#24413,#24414,#24415,#24416,#24417,#24418,#24419,#24420,#24421,
#24422,#24423,#24424,#24425,#24426,#24427,#24428,#24429,#24430,#24431,#24432),
 .UNSPECIFIED.,.F.,.F.,(4,2,2,2,2,2,2,2,2,2,2,2,2,2,2,2,2,2,2,2,2,2,2,2,
2,2,2,2,2,4),(-0.331363008767816,-0.314613325869936,-0.263867340288622,
-0.247176462282809,-0.242822084074471,-0.240248181884976,-0.238004959710724,
-0.235289894837674,-0.230105687478555,-0.223506425722653,-0.208541152356611,
-0.174691666715924,-0.145069412420928,-0.141929844389683,-0.140337806477531,
-0.139080220156367,-0.137597676101777,-0.13488172883738,-0.120193948897179,
-0.102666300485983,-0.0745907170427717,-0.0667114523857546,-0.0479811673334748,
-0.0434728312697193,-0.0408636002469527,-0.0386228621979387,-0.0364783822061139,
-0.0338123195932177,-0.0297771153707352,-0.000589579587611316),
 .UNSPECIFIED.);
#418=B_SPLINE_CURVE_WITH_KNOTS('',3,(#24433,#24434,#24435,#24436,#24437,
#24438,#24439,#24440,#24441,#24442,#24443,#24444,#24445,#24446,#24447,#24448,
#24449,#24450,#24451,#24452,#24453,#24454,#24455,#24456,#24457,#24458,#24459,
#24460,#24461,#24462,#24463,#24464,#24465,#24466,#24467,#24468,#24469,#24470,
#24471,#24472,#24473,#24474,#24475,#24476,#24477,#24478,#24479,#24480,#24481,
#24482,#24483,#24484,#24485,#24486,#24487,#24488,#24489,#24490,#24491,#24492,
#24493,#24494,#24495,#24496,#24497,#24498,#24499,#24500,#24501,#24502,#24503,
#24504,#24505,#24506,#24507,#24508,#24509,#24510,#24511,#24512,#24513,#24514,
#24515,#24516,#24517,#24518,#24519,#24520,#24521,#24522,#24523,#24524,#24525,
#24526,#24527,#24528,#24529,#24530,#24531,#24532,#24533,#24534,#24535,#24536,
#24537,#24538,#24539,#24540,#24541,#24542,#24543,#24544,#24545,#24546,#24547,
#24548,#24549,#24550,#24551,#24552,#24553,#24554,#24555,#24556,#24557,#24558,
#24559,#24560,#24561,#24562,#24563,#24564,#24565,#24566,#24567,#24568,#24569,
#24570,#24571,#24572,#24573,#24574,#24575,#24576,#24577,#24578,#24579,#24580,
#24581,#24582,#24583,#24584,#24585,#24586,#24587,#24588,#24589,#24590,#24591,
#24592),.UNSPECIFIED.,.F.,.F.,(4,2,2,2,2,2,2,2,2,2,2,2,2,2,2,2,2,2,2,2,
2,2,2,2,2,2,2,2,2,2,2,2,2,2,2,2,2,2,2,2,2,2,2,2,2,2,2,2,2,2,2,2,2,2,2,2,
2,2,2,2,2,2,2,2,2,2,2,2,2,2,2,2,2,2,2,2,2,2,2,4),(-2.51358401917516,-2.46703860870495,
-2.46051812019456,-2.45601462776875,-2.45419725742886,-2.45290914450858,
-2.45171041740422,-2.45002073159288,-2.44548318021959,-2.40464700529405,
-2.37779981793696,-2.36090169562812,-2.35677388468954,-2.35462965872032,
-2.35238935779344,-2.3497816367392,-2.34527840742169,-2.32661282921734,
-2.29323509950433,-2.26204653145543,-2.25680265662964,-2.25487274654001,
-2.25356258071575,-2.25238753313668,-2.25048344397783,-2.24577632722571,
-2.20858866072298,-2.17736326057625,-2.16674123678549,-2.15914203105175,
-2.15596576186363,-2.15366699020086,-2.15156482532594,-2.14873385523847,
-2.14180236408896,-2.09357101040751,-2.06252505115547,-2.05729207703341,
-2.05536366441566,-2.05405375605734,-2.05287836137734,-2.05097263444841,
-2.04625610368035,-2.00958269215844,-2.00827377236082,-1.96357062935181,
-1.95836210175496,-1.95563066737396,-1.95360665753113,-1.95108035445126,
-1.94682777536967,-1.93178326394824,-1.92412774371613,-1.87492927438097,
-1.85935091895692,-1.85659442034959,-1.85510325700639,-1.85384644525813,
-1.85226563405835,-1.84917842462162,-1.82743592732228,-1.7933232899625,
-1.7734818379219,-1.76145754600471,-1.75767679399282,-1.75525400601117,
-1.75297560363687,-1.74997200248425,-1.74318546755197,-1.69190450788205,
-1.66983204042916,-1.66282779437516,-1.65807321130845,-1.65621599499858,
-1.65492022064735,-1.65373063107379,-1.65174984896922,-1.64657571147666,
-1.60316397744653,-1.58790776972358),.UNSPECIFIED.);
#419=B_SPLINE_CURVE_WITH_KNOTS('',3,(#24598,#24599,#24600,#24601,#24602,
#24603,#24604,#24605,#24606,#24607,#24608,#24609,#24610,#24611,#24612,#24613,
#24614,#24615,#24616,#24617,#24618,#24619,#24620,#24621,#24622,#24623,#24624,
#24625,#24626,#24627,#24628,#24629,#24630,#24631,#24632,#24633,#24634,#24635,
#24636,#24637,#24638,#24639,#24640,#24641,#24642,#24643,#24644,#24645,#24646,
#24647,#24648,#24649,#24650,#24651,#24652,#24653,#24654,#24655,#24656,#24657,
#24658,#24659,#24660,#24661,#24662,#24663,#24664,#24665,#24666,#24667,#24668,
#24669,#24670,#24671,#24672,#24673,#24674,#24675,#24676,#24677,#24678,#24679,
#24680,#24681,#24682,#24683,#24684,#24685,#24686,#24687,#24688,#24689,#24690,
#24691,#24692,#24693,#24694,#24695,#24696,#24697,#24698,#24699,#24700,#24701,
#24702,#24703,#24704,#24705,#24706,#24707,#24708,#24709,#24710,#24711,#24712,
#24713,#24714,#24715,#24716,#24717,#24718,#24719,#24720,#24721,#24722,#24723,
#24724,#24725,#24726,#24727,#24728,#24729,#24730,#24731,#24732,#24733,#24734,
#24735,#24736,#24737,#24738,#24739,#24740,#24741,#24742,#24743,#24744,#24745,
#24746,#24747,#24748,#24749,#24750,#24751,#24752,#24753,#24754,#24755,#24756,
#24757,#24758,#24759,#24760,#24761,#24762,#24763,#24764,#24765,#24766,#24767,
#24768,#24769,#24770,#24771,#24772,#24773,#24774,#24775,#24776,#24777,#24778,
#24779,#24780,#24781,#24782,#24783,#24784,#24785,#24786,#24787,#24788,#24789,
#24790,#24791,#24792,#24793,#24794,#24795,#24796,#24797,#24798,#24799),
 .UNSPECIFIED.,.F.,.F.,(4,2,2,2,2,2,2,2,2,2,2,2,2,2,2,2,2,2,2,2,2,2,2,2,
2,2,2,2,2,2,2,2,2,2,2,2,2,2,2,2,2,2,2,2,2,2,2,2,2,2,2,2,2,2,2,2,2,2,2,2,
2,2,2,2,2,2,2,2,2,2,2,2,2,2,2,2,2,2,2,2,2,2,2,2,2,2,2,2,2,2,2,2,2,2,2,2,
2,2,2,2,4),(-0.926590849584021,-0.895705628617206,-0.849097035878392,-0.84205238580067,
-0.839201487858656,-0.837093933251416,-0.834798394542621,-0.831643261401205,
-0.824174518738562,-0.813788802669523,-0.7837535010908,-0.777232071165272,
-0.774946725784697,-0.756916936181162,-0.742064214596665,-0.739479374222173,
-0.737870647314892,-0.736611704772934,-0.735141235364103,-0.732481715790049,
-0.718919058633716,-0.685782092130831,-0.646498652233088,-0.641855846977377,
-0.638965158103643,-0.636710135130437,-0.634211917532468,-0.630088762293131,
-0.614588451309749,-0.562036459205467,-0.557273586525968,-0.542536259699213,
-0.539956820168759,-0.53834966162718,-0.537090765311508,-0.535618981590008,
-0.532953677846819,-0.519284180896549,-0.483463864555616,-0.479834864333695,
-0.447003099826601,-0.442349011651426,-0.43945481891684,-0.437199219675766,
-0.434702563613216,-0.430587084483246,-0.415178318239458,-0.363324761820432,
-0.356756312954078,-0.342930448248988,-0.340396089552481,-0.338802484965043,
-0.337544493127627,-0.336062417776771,-0.333349724848171,-0.318740074634343,
-0.287948673622923,-0.247447086897912,-0.242803199030523,-0.239911966447855,
-0.237656599298613,-0.2376061950838,-0.237560501009073,-0.237519066148853,
-0.237481482031868,-0.237447381287586,-0.237416432763583,-0.237388337869124,
-0.237362827247346,-0.237339657852027,-0.237318610250785,-0.237299486247105,
-0.237272793681814,-0.237246662466461,-0.237221077810542,-0.237196025360201,
-0.237171491207558,-0.237147461813345,-0.237123924063153,-0.234481204273956,
-0.229639135778107,-0.223576755855529,-0.172049741676069,-0.143982609666729,
-0.140842202158548,-0.139249695289737,-0.137991710515435,-0.136508637639563,
-0.13379154507168,-0.1190922253451,-0.0836875128642156,-0.0677007568617229,
-0.0578862961661651,-0.045709236361506,-0.0417684314047173,-0.0393099850987222,
-0.0370436444585214,-0.0348306661534586,-0.0319439022230871,-0.0273777962145406,
-0.000589178997369609),.UNSPECIFIED.);
#420=B_SPLINE_CURVE_WITH_KNOTS('',3,(#24800,#24801,#24802,#24803,#24804,
#24805,#24806,#24807,#24808,#24809,#24810,#24811,#24812,#24813,#24814,#24815,
#24816,#24817,#24818,#24819,#24820,#24821,#24822,#24823,#24824,#24825,#24826,
#24827,#24828,#24829,#24830,#24831,#24832,#24833,#24834,#24835,#24836,#24837,
#24838,#24839,#24840,#24841,#24842,#24843,#24844,#24845,#24846,#24847,#24848,
#24849,#24850,#24851,#24852,#24853),.UNSPECIFIED.,.F.,.F.,(4,2,2,2,2,2,
2,2,2,2,2,2,2,2,2,2,2,2,2,2,2,2,2,2,2,2,4),(-2.51327171715581,-2.48216238508032,
-2.45919088034406,-2.45466062409862,-2.45283886646618,-2.4515498705018,
-2.45035209269732,-2.44866616191491,-2.44415559962663,-2.40283336804128,
-2.37572130933742,-2.35946289330924,-2.35538592518744,-2.35324585131935,
-2.35102717896767,-2.34841220047479,-2.34387768404516,-2.32476294411026,
-2.27290024661368,-2.25704996916575,-2.25428163299295,-2.25278787855367,
-2.25153113879486,-2.24995323829489,-2.24687991493532,-2.22570759015456,
-2.18288930522275),.UNSPECIFIED.);
#421=B_SPLINE_CURVE_WITH_KNOTS('',3,(#24854,#24855,#24856,#24857,#24858,
#24859,#24860,#24861,#24862,#24863,#24864,#24865,#24866,#24867,#24868,#24869,
#24870,#24871,#24872,#24873,#24874,#24875,#24876,#24877,#24878,#24879,#24880,
#24881,#24882,#24883,#24884,#24885,#24886,#24887,#24888,#24889,#24890,#24891,
#24892,#24893,#24894,#24895,#24896,#24897,#24898,#24899,#24900,#24901,#24902,
#24903,#24904,#24905,#24906,#24907,#24908,#24909,#24910,#24911,#24912,#24913,
#24914,#24915,#24916,#24917,#24918,#24919,#24920,#24921,#24922,#24923,#24924,
#24925,#24926,#24927,#24928,#24929,#24930,#24931,#24932,#24933,#24934,#24935,
#24936,#24937,#24938,#24939,#24940,#24941,#24942,#24943,#24944,#24945,#24946,
#24947,#24948,#24949,#24950,#24951,#24952,#24953,#24954,#24955,#24956,#24957,
#24958,#24959,#24960,#24961,#24962,#24963,#24964,#24965,#24966,#24967,#24968,
#24969,#24970,#24971,#24972,#24973,#24974,#24975,#24976,#24977,#24978,#24979,
#24980,#24981,#24982,#24983,#24984,#24985,#24986,#24987,#24988,#24989,#24990,
#24991,#24992,#24993,#24994,#24995,#24996,#24997,#24998,#24999,#25000,#25001,
#25002,#25003,#25004,#25005,#25006,#25007,#25008,#25009,#25010,#25011,#25012,
#25013,#25014,#25015,#25016,#25017,#25018,#25019,#25020,#25021,#25022,#25023,
#25024,#25025,#25026,#25027,#25028,#25029,#25030,#25031,#25032,#25033,#25034,
#25035,#25036,#25037,#25038,#25039,#25040,#25041,#25042,#25043,#25044,#25045,
#25046,#25047,#25048,#25049,#25050,#25051,#25052,#25053,#25054,#25055,#25056,
#25057,#25058,#25059,#25060,#25061,#25062,#25063,#25064,#25065,#25066,#25067,
#25068,#25069,#25070,#25071,#25072,#25073,#25074,#25075),.UNSPECIFIED.,
 .F.,.F.,(4,2,2,2,2,2,2,2,2,2,2,2,2,2,2,2,2,2,2,2,2,2,2,2,2,2,2,2,2,2,2,
2,2,2,2,2,2,2,2,2,2,2,2,2,2,2,2,2,2,2,2,2,2,2,2,2,2,2,2,2,2,2,2,2,2,2,2,
2,2,2,2,2,2,2,2,2,2,2,2,2,2,2,2,2,2,2,2,2,2,2,2,2,2,2,2,2,2,2,2,2,2,2,2,
2,2,2,2,2,2,2,4),(-1.58790776972358,-1.56433038537726,-1.55922552834473,
-1.55651550855986,-1.55429663836922,-1.55168292212814,-1.54715436724346,
-1.52813037922064,-1.47614614877465,-1.46028109451036,-1.45751195575631,
-1.45601797405431,-1.45476117260214,-1.45318338617889,-1.4501108637531,
-1.42896988838759,-1.37803958926502,-1.36805226866343,-1.36080496724478,
-1.3576876652133,-1.35539902472085,-1.35328333181485,-1.35039917994523,
-1.34315648021733,-1.30169838395921,-1.27269464144579,-1.26449670339422,
-1.25914786400453,-1.25720279984552,-1.25601998818139,-1.25471780634858,
-1.25282809331194,-1.24786016457302,-1.24043607544603,-1.21609426764117,
-1.16831833072192,-1.16135110661376,-1.15851372473321,-1.15640974861023,
-1.15411187187234,-1.15094212745578,-1.14338416094597,-1.13283645927949,
-1.10199248833042,-1.06418610726124,-1.05951055055522,-1.05761151373998,
-1.05643722499709,-1.05512561058081,-1.05318956827674,-1.04790434174775,
-1.03983840816093,-0.986921597734203,-0.979849263367743,-0.96424914910678,
-0.959944356115374,-0.957406397205592,-0.955383753702977,-0.952667993201792,
-0.947535709764712,-0.906442000049919,-0.864311606286453,-0.859854417102353,
-0.858175525700282,-0.856979535409336,-0.855688908569718,-0.853859037279309,
-0.849278918784948,-0.825798522273947,-0.799834300346273,-0.766250011593278,
-0.761588242008963,-0.758691938877223,-0.756436334221659,-0.753941347516222,
-0.74983251145566,-0.73449664720544,-0.683187480161499,-0.674762776190746,
-0.662035645267422,-0.659561113628769,-0.657985800836894,-0.656729035787356,
-0.655232800303313,-0.652453434985366,-0.636347181587834,-0.581669316826979,
-0.565263035664434,-0.560927233560201,-0.558357533134028,-0.556113792558436,
-0.553337497964581,-0.547912321027593,-0.504863377490104,-0.465348547109447,
-0.460756767152621,-0.458871617368697,-0.457583207893888,-0.456241511823363,
-0.454165620251658,-0.447820358056242,-0.437464068155186,-0.389527692327158,
-0.366507039381414,-0.362143755338416,-0.35933772025724,-0.357091582241529,
-0.354542529520285,-0.35018792614072,-0.331697579609663,-0.331164696783045),
 .UNSPECIFIED.);
#422=B_SPLINE_CURVE_WITH_KNOTS('',3,(#25080,#25081,#25082,#25083,#25084,
#25085,#25086,#25087,#25088,#25089,#25090,#25091,#25092,#25093,#25094,#25095,
#25096,#25097,#25098,#25099,#25100,#25101,#25102,#25103,#25104,#25105,#25106,
#25107,#25108,#25109,#25110,#25111,#25112,#25113,#25114,#25115,#25116,#25117,
#25118,#25119,#25120,#25121,#25122,#25123,#25124,#25125,#25126,#25127,#25128,
#25129,#25130,#25131,#25132,#25133,#25134,#25135,#25136,#25137,#25138,#25139,
#25140,#25141,#25142,#25143,#25144,#25145,#25146,#25147,#25148,#25149,#25150,
#25151,#25152,#25153,#25154,#25155,#25156,#25157,#25158,#25159,#25160,#25161,
#25162,#25163,#25164,#25165,#25166,#25167,#25168,#25169,#25170,#25171,#25172,
#25173,#25174,#25175,#25176,#25177,#25178,#25179,#25180,#25181,#25182,#25183,
#25184,#25185,#25186,#25187,#25188,#25189,#25190,#25191,#25192,#25193,#25194,
#25195,#25196,#25197,#25198,#25199,#25200,#25201,#25202,#25203,#25204,#25205,
#25206,#25207,#25208,#25209,#25210,#25211,#25212,#25213,#25214,#25215,#25216,
#25217,#25218,#25219,#25220,#25221,#25222,#25223,#25224,#25225,#25226,#25227,
#25228,#25229,#25230,#25231,#25232,#25233,#25234,#25235,#25236,#25237,#25238,
#25239,#25240,#25241,#25242,#25243,#25244,#25245,#25246,#25247,#25248,#25249,
#25250,#25251,#25252,#25253,#25254,#25255,#25256,#25257,#25258,#25259,#25260,
#25261,#25262,#25263,#25264,#25265,#25266,#25267,#25268,#25269,#25270,#25271,
#25272,#25273,#25274,#25275,#25276,#25277,#25278,#25279,#25280,#25281,#25282,
#25283,#25284,#25285,#25286,#25287,#25288,#25289,#25290,#25291,#25292,#25293),
 .UNSPECIFIED.,.F.,.F.,(4,2,2,2,2,2,2,2,2,2,2,2,2,2,2,2,2,2,2,2,2,2,2,2,
2,2,2,2,2,2,2,2,2,2,2,2,2,2,2,2,2,2,2,2,2,2,2,2,2,2,2,2,2,2,2,2,2,2,2,2,
2,2,2,2,2,2,2,2,2,2,2,2,2,2,2,2,2,2,2,2,2,2,2,2,2,2,2,2,2,2,2,2,2,2,2,2,
2,2,2,2,2,2,2,2,2,2,4),(-2.18303470285366,-2.15323070742354,-2.13838275441974,
-2.13565920080161,-2.13417502276345,-2.13291756089068,-2.13132758505621,
-2.12819774145529,-2.09732430128089,-2.05947037596656,-2.04158971387745,
-2.03727871475553,-2.03473931492364,-2.03249198606179,-2.02967158806749,
-2.02526089969832,-2.00098170680169,-1.95423868863094,-1.9389419007886,
-1.93619761165177,-1.93470892585,-1.93345172481894,-1.93186725469224,-1.92936251419912,
-1.91608774371415,-1.8579349067261,-1.84179569422143,-1.83761925732135,
-1.83510951416174,-1.83285725855118,-1.8299882590998,-1.82541692029795,
-1.79627084060417,-1.75406610782806,-1.73936708878227,-1.73665055484494,
-1.73516787905997,-1.73391028142891,-1.73231833842737,-1.72917926022242,
-1.70187761255867,-1.68842486591373,-1.65811051600642,-1.64766888773947,
-1.64016876818698,-1.63700858717922,-1.6347123316985,-1.6326061581937,-1.62976022503272,
-1.62274365673674,-1.57566490710204,-1.54073000057352,-1.5375055302525,
-1.53591745204772,-1.53465999739472,-1.53317406646495,-1.5305178873319,
-1.51865850714293,-1.45907989559261,-1.44280473715374,-1.43861714468706,
-1.43610491853278,-1.4338530992537,-1.43098830552653,-1.42643100233579,
-1.39778419182389,-1.35512210007525,-1.34035792101552,-1.33763825993884,
-1.33615489535833,-1.33489733058598,-1.33330621547456,-1.33017111859939,
-1.30379552089089,-1.25734096698368,-1.24325615154456,-1.23910203776784,
-1.23659716011384,-1.23434383637724,-1.23146598879311,-1.22552999347426,
-1.18770298528498,-1.14331160636109,-1.13908645869486,-1.13744080414567,
-1.13625357555316,-1.13495547125603,-1.13308668699463,-1.12825750268597,
-1.12110796042993,-1.09826765738807,-1.04825527587019,-1.04134067265296,
-1.03858686777589,-1.03629453433488,-1.03393894020954,-1.0304741371515,
-1.0209779822248,-1.0067028198717,-0.950036471996001,-0.940858628873664,
-0.938389628295971,-0.936960772696591,-0.935821787841959,-0.934218751633752,
-0.930919155436449,-0.926590849584021),.UNSPECIFIED.);
#423=B_SPLINE_CURVE_WITH_KNOTS('',3,(#25295,#25296,#25297,#25298,#25299,
#25300,#25301,#25302,#25303,#25304,#25305,#25306,#25307,#25308,#25309,#25310,
#25311,#25312,#25313,#25314,#25315,#25316,#25317,#25318,#25319,#25320,#25321,
#25322,#25323,#25324,#25325,#25326,#25327,#25328,#25329,#25330,#25331,#25332,
#25333,#25334,#25335,#25336,#25337,#25338,#25339,#25340,#25341,#25342,#25343,
#25344,#25345,#25346),.UNSPECIFIED.,.F.,.F.,(4,2,2,2,2,2,2,2,2,2,2,2,2,
2,2,2,2,2,2,2,2,2,2,2,2,4),(-0.331164696783045,-0.284340024328848,-0.263458405458446,
-0.260394021052475,-0.258817921732811,-0.25756113203129,-0.256065580756608,
-0.253289371421596,-0.237388738728392,-0.184912682781884,-0.166395205030571,
-0.161901670623027,-0.159295798848285,-0.157054846381753,-0.154909335325312,
-0.150771729368069,-0.13373600435653,-0.106159192349091,-0.0661893748728856,
-0.061617829780471,-0.0597360883543101,-0.0584483707546459,-0.0571057808163933,
-0.0550256913502012,-0.0486456322016143,-0.00058995120662514),
 .UNSPECIFIED.);
#424=B_SPLINE_CURVE_WITH_KNOTS('',3,(#25347,#25348,#25349,#25350,#25351,
#25352,#25353,#25354,#25355,#25356,#25357,#25358,#25359,#25360,#25361,#25362,
#25363,#25364,#25365,#25366,#25367,#25368,#25369,#25370,#25371,#25372,#25373,
#25374,#25375,#25376,#25377,#25378,#25379,#25380,#25381,#25382,#25383,#25384,
#25385,#25386,#25387,#25388,#25389,#25390,#25391,#25392,#25393,#25394,#25395,
#25396,#25397,#25398,#25399,#25400,#25401,#25402,#25403,#25404,#25405,#25406,
#25407,#25408,#25409,#25410,#25411,#25412,#25413,#25414,#25415,#25416,#25417,
#25418,#25419,#25420,#25421,#25422,#25423,#25424,#25425,#25426,#25427,#25428,
#25429,#25430,#25431,#25432,#25433,#25434,#25435,#25436,#25437,#25438,#25439,
#25440,#25441,#25442,#25443,#25444,#25445,#25446,#25447,#25448,#25449,#25450,
#25451,#25452,#25453,#25454,#25455,#25456,#25457,#25458,#25459,#25460,#25461,
#25462,#25463,#25464,#25465,#25466,#25467,#25468,#25469,#25470,#25471,#25472,
#25473,#25474,#25475,#25476,#25477,#25478,#25479,#25480,#25481,#25482,#25483,
#25484,#25485,#25486,#25487,#25488,#25489,#25490,#25491,#25492,#25493,#25494,
#25495,#25496,#25497,#25498,#25499,#25500,#25501,#25502,#25503,#25504,#25505,
#25506),.UNSPECIFIED.,.F.,.F.,(4,2,2,2,2,2,2,2,2,2,2,2,2,2,2,2,2,2,2,2,
2,2,2,2,2,2,2,2,2,2,2,2,2,2,2,2,2,2,2,2,2,2,2,2,2,2,2,2,2,2,2,2,2,2,2,2,
2,2,2,2,2,2,2,2,2,2,2,2,2,2,2,2,2,2,2,2,2,2,2,4),(-2.51410445116209,-2.48115962050804,
-2.4775909854511,-2.47511710807547,-2.47301244678002,-2.47076222930669,
-2.46791145153916,-2.46340035413433,-2.43629515448796,-2.41345917543091,
-2.3918711866273,-2.37725269550936,-2.37452995355423,-2.37304602537111,
-2.37178866658817,-2.37019871104166,-2.36706860085179,-2.34130238490027,
-2.28778461265617,-2.28158674873041,-2.27666077349263,-2.27399903801622,
-2.27197657063979,-2.26943915158629,-2.26513604710984,-2.24955080300122,
-2.2424050734882,-2.20341756298698,-2.18046744818344,-2.17593920896639,
-2.1741178163007,-2.17282892763191,-2.17163114411436,-2.16994507729867,
-2.16543325549935,-2.12410635948414,-2.08265470442655,-2.07733252077868,
-2.07457767069645,-2.07255116461594,-2.07004071453089,-2.06585997657549,
-2.05151614598836,-2.04212252185987,-1.99373447131584,-1.98334167469653,
-1.97698131906251,-1.97490385701313,-1.97356201090889,-1.97227418791932,
-1.97039103713779,-1.96580976647041,-1.92614628363177,-1.88300627035365,
-1.87775431228586,-1.87501386675412,-1.87298888623818,-1.87046871175628,
-1.86624407825216,-1.85147730278375,-1.84284309777178,-1.79042690555159,
-1.78238945657257,-1.7771186455345,-1.77518472927491,-1.77387361724298,
-1.77269906382288,-1.77079827600718,-1.76611178981052,-1.72855070920642,
-1.6844844865033,-1.67858935215021,-1.67571960484346,-1.67346737213277,
-1.67095829089961,-1.66678447810119,-1.652509791412,-1.64298838599048,-1.59084016524227,
-1.58799807313078),.UNSPECIFIED.);
#425=B_SPLINE_CURVE_WITH_KNOTS('',3,(#25512,#25513,#25514,#25515,#25516,
#25517,#25518,#25519,#25520),.UNSPECIFIED.,.F.,.F.,(4,1,1,1,1,1,4),(47.1238898038469,
47.2191271055195,48.2168442690671,49.2145614326147,50.2122785961623,51.2099957597099,
51.753505798748),.UNSPECIFIED.);
#426=B_SPLINE_CURVE_WITH_KNOTS('',3,(#25521,#25522,#25523,#25524,#25525,
#25526,#25527,#25528,#25529,#25530,#25531,#25532,#25533,#25534,#25535,#25536,
#25537,#25538,#25539,#25540,#25541,#25542,#25543,#25544,#25545,#25546,#25547,
#25548,#25549,#25550,#25551,#25552,#25553,#25554,#25555,#25556,#25557,#25558,
#25559,#25560,#25561,#25562,#25563,#25564,#25565,#25566,#25567,#25568,#25569,
#25570,#25571,#25572,#25573,#25574),.UNSPECIFIED.,.F.,.F.,(4,2,2,2,2,2,
2,2,2,2,2,2,2,2,2,2,2,2,2,2,2,2,2,2,2,2,4),(-2.51382926221767,-2.45903949326626,
-2.44068235929343,-2.43633727043439,-2.4337903419711,-2.43154397812033,
-2.42873488528968,-2.42436142953249,-2.40107333404785,-2.35338312683811,
-2.34304546170578,-2.33878344098341,-2.33559364184831,-2.33400554447704,
-2.33278162207138,-2.33133353937978,-2.32884275385845,-2.31910991204386,
-2.25731393916809,-2.24084993657796,-2.23664717385184,-2.23413165225028,
-2.23188053067103,-2.22902160968702,-2.22448363042851,-2.19649575545307,
-2.18303470285366),.UNSPECIFIED.);
#427=B_SPLINE_CURVE_WITH_KNOTS('',3,(#25575,#25576,#25577,#25578,#25579,
#25580,#25581,#25582,#25583,#25584,#25585,#25586,#25587,#25588,#25589,#25590,
#25591,#25592,#25593,#25594,#25595,#25596,#25597,#25598,#25599,#25600,#25601,
#25602,#25603,#25604,#25605,#25606,#25607,#25608,#25609,#25610,#25611,#25612,
#25613,#25614,#25615,#25616,#25617,#25618,#25619,#25620,#25621,#25622,#25623,
#25624,#25625,#25626,#25627,#25628,#25629,#25630,#25631,#25632,#25633,#25634,
#25635,#25636,#25637,#25638,#25639,#25640,#25641,#25642,#25643,#25644,#25645,
#25646,#25647,#25648,#25649,#25650,#25651,#25652,#25653,#25654,#25655,#25656,
#25657,#25658,#25659,#25660,#25661,#25662,#25663,#25664,#25665,#25666,#25667,
#25668,#25669,#25670,#25671,#25672,#25673,#25674,#25675,#25676,#25677,#25678,
#25679,#25680,#25681,#25682,#25683,#25684,#25685,#25686,#25687,#25688,#25689,
#25690,#25691,#25692,#25693,#25694,#25695,#25696,#25697,#25698,#25699,#25700,
#25701,#25702,#25703,#25704,#25705,#25706,#25707,#25708,#25709,#25710,#25711,
#25712,#25713,#25714,#25715,#25716,#25717,#25718,#25719,#25720,#25721,#25722,
#25723,#25724,#25725,#25726,#25727,#25728,#25729,#25730,#25731,#25732,#25733,
#25734,#25735,#25736,#25737,#25738,#25739,#25740,#25741,#25742,#25743,#25744,
#25745,#25746,#25747,#25748,#25749,#25750,#25751,#25752,#25753,#25754,#25755,
#25756,#25757,#25758,#25759,#25760,#25761,#25762,#25763,#25764,#25765,#25766,
#25767,#25768,#25769,#25770,#25771,#25772,#25773,#25774,#25775,#25776,#25777,
#25778,#25779,#25780,#25781,#25782,#25783,#25784,#25785,#25786,#25787,#25788,
#25789,#25790,#25791,#25792,#25793,#25794),.UNSPECIFIED.,.F.,.F.,(4,2,2,
2,2,2,2,2,2,2,2,2,2,2,2,2,2,2,2,2,2,2,2,2,2,2,2,2,2,2,2,2,2,2,2,2,2,2,2,
2,2,2,2,2,2,2,2,2,2,2,2,2,2,2,2,2,2,2,2,2,2,2,2,2,2,2,2,2,2,2,2,2,2,2,2,
2,2,2,2,2,2,2,2,2,2,2,2,2,2,2,2,2,2,2,2,2,2,2,2,2,2,2,2,2,2,2,2,2,2,4),
(-1.58799807313078,-1.58281854779097,-1.57755537961493,-1.5756224874594,
-1.57431153510487,-1.57313671950623,-1.57123475362205,-1.56654160087626,
-1.52906351136109,-1.49802699439358,-1.48199304797864,-1.47782511396363,
-1.47531717555945,-1.47306445112747,-1.47019199152731,-1.46560938630689,
-1.43669924933499,-1.39428106696778,-1.37954944304334,-1.37683123410999,
-1.37534815887241,-1.37409054249698,-1.3724990119409,-1.36936207201397,
-1.34274183254778,-1.28674100229136,-1.27993345901643,-1.27689317464382,
-1.27461735267793,-1.2721882306633,-1.26837862871245,-1.25723710660705,
-1.23894332830876,-1.21377157079921,-1.20269944921508,-1.20183196487044,
-1.1806593824426,-1.17758610323861,-1.17600826057003,-1.174751591428,-1.17325796937191,
-1.17049004405378,-1.15464591426987,-1.10283366266568,-1.08368075910792,
-1.0791439567425,-1.07652848512044,-1.07430988584095,-1.07160236463613,
-1.06650883198453,-1.02845631994496,-0.98703199366014,-0.979653981653059,
-0.977375689492475,-0.975989358952021,-0.974710736414749,-0.972948252382905,
-0.968776938777643,-0.949308591445746,-0.898213513488314,-0.883458187345647,
-0.879234678108117,-0.876714705181225,-0.874689625715152,-0.871948694274047,
-0.866694631378739,-0.823439680357804,-0.783858298084751,-0.779271076918284,
-0.777386865775199,-0.776098786118058,-0.774757126591892,-0.772680757375622,
-0.766329880626308,-0.755960188204414,-0.707840955538581,-0.697561859977648,
-0.683732683711984,-0.679605829781044,-0.677107111653054,-0.674852757496159,
-0.671964490956605,-0.665973890678441,-0.62125639897922,-0.584495431343864,
-0.579779286833981,-0.577873528946357,-0.576698059128757,-0.575388009606254,
-0.57345929734738,-0.568224880184591,-0.537165905962623,-0.488987914889991,
-0.482052090544821,-0.479220220913931,-0.477117698220485,-0.474818838034934,
-0.471643015508458,-0.464047682685806,-0.453431819894759,-0.42224030535768,
-0.384950837732984,-0.380245214903167,-0.378341230681134,-0.377166096588368,
-0.375855686179772,-0.373925163426813,-0.368678008366101,-0.360689937409051,
-0.331376765677369),.UNSPECIFIED.);
#428=B_SPLINE_CURVE_WITH_KNOTS('',3,(#25800,#25801,#25802,#25803,#25804,
#25805,#25806,#25807,#25808,#25809,#25810,#25811,#25812,#25813,#25814,#25815,
#25816,#25817,#25818,#25819,#25820,#25821,#25822,#25823,#25824,#25825,#25826,
#25827,#25828,#25829,#25830,#25831,#25832,#25833,#25834,#25835,#25836,#25837,
#25838,#25839,#25840,#25841,#25842,#25843,#25844,#25845,#25846,#25847,#25848,
#25849,#25850,#25851,#25852,#25853,#25854,#25855,#25856,#25857,#25858,#25859,
#25860,#25861,#25862,#25863,#25864,#25865,#25866,#25867,#25868,#25869,#25870,
#25871,#25872,#25873,#25874,#25875,#25876,#25877,#25878,#25879,#25880,#25881,
#25882,#25883,#25884,#25885,#25886,#25887,#25888,#25889,#25890,#25891,#25892,
#25893,#25894,#25895,#25896,#25897,#25898,#25899,#25900,#25901,#25902,#25903,
#25904,#25905,#25906,#25907,#25908,#25909,#25910,#25911,#25912,#25913,#25914,
#25915,#25916,#25917,#25918,#25919,#25920,#25921,#25922,#25923,#25924,#25925,
#25926,#25927,#25928,#25929,#25930,#25931,#25932,#25933,#25934,#25935,#25936,
#25937,#25938,#25939,#25940,#25941,#25942,#25943,#25944,#25945,#25946,#25947,
#25948,#25949,#25950,#25951,#25952,#25953),.UNSPECIFIED.,.F.,.F.,(4,2,2,
2,2,2,2,2,2,2,2,2,2,2,2,2,2,2,2,2,2,2,2,2,2,2,2,2,2,2,2,2,2,2,2,2,2,2,2,
2,2,2,2,2,2,2,2,2,2,2,2,2,2,2,2,2,2,2,2,2,2,2,2,2,2,2,2,2,2,2,2,2,2,2,2,
2,4),(-0.926782221294469,-0.896569100631809,-0.867447118673057,-0.862876094611461,
-0.860006951553309,-0.857754387215146,-0.855244096965053,-0.851066274682072,
-0.834916065147125,-0.776686390209619,-0.763443585714247,-0.760940167704961,
-0.759355947067707,-0.758098536432829,-0.756609114835076,-0.753862217391411,
-0.738514391918759,-0.691339421288076,-0.667534478572589,-0.663141365188601,
-0.660325983629374,-0.658078676370874,-0.655535052155691,-0.651206417428453,
-0.6330909157989,-0.585626792600053,-0.564456624116818,-0.561382686323562,
-0.559804384165768,-0.558547278484847,-0.557053027733001,-0.554283624801016,
-0.53842083286486,-0.486429462491141,-0.467451549432601,-0.46292553704893,
-0.460311979787076,-0.458092471214793,-0.455380709575718,-0.450269616839376,
-0.411074460894452,-0.366679149602077,-0.362463768482037,-0.360819511930875,
-0.359632481435553,-0.358333666825421,-0.356462303850262,-0.351617877119955,
-0.344438872658291,-0.32144410179083,-0.271648037273247,-0.264711303041573,
-0.261953609145812,-0.25965992714859,-0.257304879895282,-0.253844487590635,
-0.244586799371763,-0.23069623817164,-0.182930715482505,-0.179584128800173,
-0.164918984744038,-0.162342767911905,-0.160736473467934,-0.159477499261556,
-0.158004749467612,-0.155523551248057,-0.143761124602971,-0.116923019618865,
-0.0726531924634352,-0.0654919159067642,-0.0626209873586662,-0.0605082243338179,
-0.0582162528217251,-0.0550827265177684,-0.0516124903134288,-0.0403488636777721,
-0.000589815695671829),.UNSPECIFIED.);
#429=B_SPLINE_CURVE_WITH_KNOTS('',3,(#25954,#25955,#25956,#25957,#25958,
#25959),.UNSPECIFIED.,.F.,.F.,(4,1,1,4),(51.753505798748,52.2077129232575,
53.2054300868052,53.4070751110265),.UNSPECIFIED.);
#430=B_SPLINE_CURVE_WITH_KNOTS('',3,(#25961,#25962,#25963,#25964,#25965,
#25966,#25967,#25968,#25969,#25970,#25971,#25972,#25973,#25974,#25975,#25976,
#25977,#25978,#25979,#25980,#25981,#25982,#25983,#25984,#25985,#25986,#25987,
#25988,#25989,#25990,#25991,#25992,#25993,#25994,#25995,#25996,#25997,#25998,
#25999,#26000,#26001,#26002,#26003,#26004,#26005,#26006,#26007,#26008,#26009,
#26010,#26011,#26012,#26013,#26014,#26015,#26016,#26017,#26018,#26019,#26020,
#26021,#26022,#26023,#26024,#26025,#26026,#26027,#26028,#26029,#26030,#26031,
#26032),.UNSPECIFIED.,.F.,.F.,(4,2,2,2,2,2,2,2,2,2,2,2,2,2,2,2,2,2,2,2,
2,2,2,2,2,2,2,2,2,2,2,2,2,2,2,4),(-0.331376765677369,-0.309063892239683,
-0.285958208367855,-0.281592278087566,-0.278785677343909,-0.276539819396871,
-0.273991872497997,-0.269641116675965,-0.251198764775781,-0.210921638042901,
-0.183051994460163,-0.179916331687803,-0.178325200630787,-0.177067771202634,
-0.177060482826282,-0.177053263815713,-0.177046112922922,-0.177039028893918,
-0.177032010767957,-0.177025057373861,-0.177018167626151,-0.177011340628512,
-0.175534301229271,-0.172876503285918,-0.169474827828848,-0.16198886748036,
-0.137296419888448,-0.0900392263524134,-0.0830363294569277,-0.0801930047857767,
-0.0780877085930016,-0.0757913910703241,-0.0726292855006604,-0.0651159049661456,
-0.0546487482589572,-0.000590208984640202),.UNSPECIFIED.);
#431=B_SPLINE_CURVE_WITH_KNOTS('',3,(#26033,#26034,#26035,#26036,#26037,
#26038,#26039,#26040,#26041,#26042,#26043,#26044,#26045,#26046,#26047,#26048,
#26049,#26050,#26051,#26052,#26053,#26054,#26055,#26056,#26057,#26058,#26059,
#26060,#26061,#26062,#26063,#26064,#26065,#26066,#26067,#26068,#26069,#26070,
#26071,#26072,#26073,#26074,#26075,#26076,#26077,#26078,#26079,#26080,#26081,
#26082,#26083,#26084,#26085,#26086,#26087,#26088,#26089,#26090,#26091,#26092,
#26093,#26094,#26095,#26096,#26097,#26098,#26099,#26100,#26101,#26102,#26103,
#26104,#26105,#26106,#26107,#26108,#26109,#26110,#26111,#26112,#26113,#26114,
#26115,#26116,#26117,#26118,#26119,#26120,#26121,#26122,#26123,#26124,#26125,
#26126,#26127,#26128,#26129,#26130,#26131,#26132,#26133,#26134,#26135,#26136,
#26137,#26138,#26139,#26140,#26141,#26142,#26143,#26144,#26145,#26146,#26147,
#26148,#26149,#26150,#26151,#26152,#26153,#26154,#26155,#26156,#26157,#26158,
#26159,#26160,#26161,#26162,#26163,#26164,#26165,#26166,#26167,#26168,#26169,
#26170,#26171,#26172,#26173,#26174,#26175,#26176,#26177,#26178,#26179,#26180,
#26181,#26182,#26183,#26184,#26185,#26186,#26187,#26188,#26189,#26190,#26191,
#26192,#26193,#26194,#26195,#26196,#26197,#26198,#26199,#26200,#26201,#26202,
#26203,#26204,#26205,#26206,#26207,#26208,#26209,#26210,#26211,#26212,#26213,
#26214,#26215,#26216,#26217,#26218,#26219,#26220,#26221,#26222,#26223,#26224,
#26225,#26226,#26227,#26228,#26229,#26230,#26231,#26232,#26233,#26234,#26235,
#26236,#26237,#26238,#26239,#26240,#26241,#26242,#26243,#26244,#26245,#26246,
#26247,#26248,#26249,#26250,#26251,#26252,#26253,#26254,#26255,#26256,#26257,
#26258,#26259,#26260,#26261,#26262),.UNSPECIFIED.,.F.,.F.,(4,2,2,2,2,2,
2,2,2,2,2,2,2,2,2,2,2,2,2,2,2,2,2,2,2,2,2,2,2,2,2,2,2,2,2,2,2,2,2,2,2,2,
2,2,2,2,2,2,2,2,2,2,2,2,2,2,2,2,2,2,2,2,2,2,2,2,2,2,2,2,2,2,2,2,2,2,2,2,
2,2,2,2,2,2,2,2,2,2,2,2,2,2,2,2,2,2,2,2,2,2,2,2,2,2,2,2,2,2,2,2,2,2,2,2,
4),(-2.51346753526968,-2.49656179228236,-2.49424723594855,-2.49273616890078,
-2.49153253300303,-2.4904003041141,-2.48891890748557,-2.48628092833495,
-2.47467461223247,-2.46438953224031,-2.41344210935815,-2.40349461615151,
-2.39627032435406,-2.39315773071129,-2.39087061291293,-2.38875496529178,
-2.38586876956187,-2.37860980224731,-2.34044838303393,-2.30883856078443,
-2.3002571234992,-2.29651339291565,-2.29361521200013,-2.29210067622909,
-2.29209676840992,-2.29209284763182,-2.29208891390529,-2.29208496724888,
-2.292081007472,-2.29207703453806,-2.29207304832167,-2.29206904876174,-2.2920650358846,
-2.29206100947057,-2.29205696947747,-2.29205291583333,-2.29204884855905,
-2.29204476735244,-2.29204067231708,-2.29203656334953,-2.29203244024959,
-2.29202830317416,-2.29202415190499,-2.29201998627501,-2.2920158061623,
-2.29201161171023,-2.29200735585989,-2.29200303220012,-2.29199863949181,
-2.29199417644603,-2.29198964205109,-2.29198503500484,-2.29198035405605,
-2.29072396623304,-2.28914406122872,-2.28605971234948,-2.25313701549437,
-2.22819669415689,-2.20033728864931,-2.19550277604362,-2.19285044322371,
-2.19083341211432,-2.18824620332314,-2.18383126039513,-2.16634169349974,
-2.11751650752112,-2.10362146207841,-2.09841081189956,-2.0946197886711,
-2.09292436995261,-2.09165624682317,-2.09023965806498,-2.08782411721593,
-2.07918227157483,-2.06467469556245,-2.03652651853766,-2.00123953520626,
-1.99619631574526,-1.99349966870737,-1.99128187958603,-1.98865784365498,
-1.98408208799893,-1.9643599454585,-1.9131083739074,-1.89731800110081,-1.89455263350775,
-1.89305970821891,-1.89180321516825,-1.89022508306611,-1.88714975356278,
-1.86590431340644,-1.81848083834169,-1.8004494510167,-1.79612832339647,
-1.79358712837836,-1.7913407632741,-1.78852497205372,-1.78412811281269,
-1.7601943684581,-1.71311724953864,-1.69778110606826,-1.69503556125834,
-1.69354684698124,-1.69229002049101,-1.69070655582423,-1.68760642285652,
-1.66434293455431,-1.62354861643047,-1.60893761960786,-1.60244718966934,
-1.59728205236897,-1.59455970113808,-1.59231958379201,-1.58970895658841,
-1.58797213626332),.UNSPECIFIED.);
#432=B_SPLINE_CURVE_WITH_KNOTS('',3,(#26267,#26268,#26269,#26270,#26271,
#26272,#26273,#26274,#26275,#26276,#26277,#26278,#26279,#26280,#26281,#26282,
#26283,#26284,#26285,#26286,#26287,#26288,#26289,#26290,#26291,#26292,#26293,
#26294,#26295,#26296,#26297,#26298,#26299,#26300,#26301,#26302,#26303,#26304,
#26305,#26306,#26307,#26308,#26309,#26310,#26311,#26312,#26313,#26314,#26315,
#26316,#26317,#26318,#26319,#26320,#26321,#26322,#26323,#26324,#26325,#26326,
#26327,#26328,#26329,#26330,#26331,#26332,#26333,#26334,#26335,#26336,#26337,
#26338,#26339,#26340,#26341,#26342,#26343,#26344,#26345,#26346,#26347,#26348,
#26349,#26350,#26351,#26352,#26353,#26354,#26355,#26356,#26357,#26358,#26359,
#26360,#26361,#26362,#26363,#26364,#26365,#26366,#26367,#26368,#26369,#26370,
#26371,#26372,#26373,#26374,#26375,#26376,#26377,#26378,#26379,#26380,#26381,
#26382,#26383,#26384,#26385,#26386,#26387,#26388,#26389,#26390,#26391,#26392,
#26393,#26394,#26395,#26396,#26397,#26398,#26399,#26400,#26401,#26402,#26403,
#26404,#26405,#26406,#26407,#26408,#26409,#26410,#26411,#26412,#26413,#26414,
#26415,#26416,#26417,#26418,#26419,#26420,#26421,#26422,#26423,#26424,#26425,
#26426,#26427,#26428,#26429,#26430,#26431,#26432,#26433,#26434,#26435,#26436,
#26437,#26438,#26439,#26440,#26441,#26442,#26443,#26444,#26445,#26446,#26447,
#26448,#26449,#26450,#26451,#26452,#26453,#26454,#26455,#26456,#26457,#26458,
#26459,#26460,#26461,#26462,#26463,#26464,#26465,#26466,#26467,#26468,#26469,
#26470,#26471,#26472,#26473,#26474,#26475,#26476,#26477,#26478,#26479,#26480,
#26481,#26482,#26483,#26484,#26485,#26486),.UNSPECIFIED.,.F.,.F.,(4,2,2,
2,2,2,2,2,2,2,2,2,2,2,2,2,2,2,2,2,2,2,2,2,2,2,2,2,2,2,2,2,2,2,2,2,2,2,2,
2,2,2,2,2,2,2,2,2,2,2,2,2,2,2,2,2,2,2,2,2,2,2,2,2,2,2,2,2,2,2,2,2,2,2,2,
2,2,2,2,2,2,2,2,2,2,2,2,2,2,2,2,2,2,2,2,2,2,2,2,2,2,2,2,2,2,2,2,2,2,4),
(-2.18319200174337,-2.16359838216707,-2.1584116001934,-2.15648969410656,
-2.15518100271013,-2.15400424566726,-2.15209168910771,-2.14733515781527,
-2.1117026065375,-2.06598685646796,-2.05998912749124,-2.05709937449685,
-2.05484471035047,-2.05234651101395,-2.04822250514987,-2.03442145243029,
-2.02543629577283,-1.97610993079422,-1.96051859735302,-1.95776130709681,
-1.95626985859612,-1.95501288431121,-1.95343193894711,-1.95093872828567,
-1.93786949853894,-1.93007531197245,-1.87860936625802,-1.86846603671781,
-1.86113158605661,-1.85799942688707,-1.85570820926452,-1.85359596284519,
-1.85072546270073,-1.84356386857095,-1.79931583588026,-1.76201427868664,
-1.75863540324206,-1.75701699140117,-1.75575730520372,-1.75429383070465,
-1.75173592666085,-1.74120938965973,-1.68599124027133,-1.67182058774856,
-1.66237510029339,-1.65891752477938,-1.65656353706547,-1.65427022678671,
-1.65151217240877,-1.64457021923226,-1.59480995628112,-1.56498014999898,
-1.55984312005975,-1.55792842001342,-1.55662118878533,-1.55544310789001,
-1.55352343947155,-1.54872459774506,-1.51607767614575,-1.48675320837772,
-1.47243778484153,-1.4629208941717,-1.45945320627041,-1.45709700459764,
-1.45480511416044,-1.45205307667352,-1.44514971648253,-1.39499021934369,
-1.37221643280129,-1.36507931473656,-1.36025683228186,-1.35838905648669,
-1.35709114121835,-1.35590368006945,-1.35425717660693,-1.35002685272821,
-1.3057114569128,-1.27140333647857,-1.26302142366455,-1.25971968882476,
-1.25739687609636,-1.25504560822842,-1.25160198491647,-1.24225736039381,
-1.22828929603157,-1.17569161707384,-1.16249594593501,-1.1599952910368,
-1.1584119989668,-1.15715476730923,-1.15566490053829,-1.15291547138757,
-1.13750586590118,-1.08979268683339,-1.06655946222934,-1.06218820417152,
-1.05937965125502,-1.05713317268694,-1.05458552700571,-1.05023776279689,
-1.03184699280381,-0.991802722515877,-0.963657384518453,-0.96051761509897,
-0.958925407794182,-0.957667647150966,-0.956184823873192,-0.953468151099108,
-0.938770136960093,-0.926782221294469),.UNSPECIFIED.);
#433=B_SPLINE_CURVE_WITH_KNOTS('',3,(#26487,#26488,#26489,#26490,#26491,
#26492,#26493,#26494,#26495,#26496,#26497,#26498,#26499,#26500,#26501,#26502,
#26503,#26504,#26505,#26506,#26507,#26508,#26509,#26510,#26511,#26512,#26513,
#26514,#26515,#26516,#26517,#26518,#26519,#26520,#26521,#26522,#26523,#26524,
#26525,#26526,#26527,#26528,#26529,#26530,#26531,#26532,#26533,#26534,#26535,
#26536,#26537,#26538,#26539,#26540,#26541,#26542,#26543,#26544,#26545,#26546,
#26547,#26548,#26549,#26550,#26551,#26552,#26553,#26554,#26555,#26556,#26557,
#26558,#26559,#26560,#26561,#26562,#26563,#26564,#26565,#26566,#26567,#26568,
#26569,#26570,#26571,#26572,#26573,#26574,#26575,#26576,#26577,#26578,#26579,
#26580,#26581,#26582,#26583,#26584,#26585,#26586,#26587,#26588,#26589,#26590,
#26591,#26592,#26593,#26594,#26595,#26596,#26597,#26598,#26599,#26600,#26601,
#26602,#26603,#26604,#26605,#26606,#26607,#26608,#26609,#26610,#26611,#26612,
#26613,#26614,#26615,#26616,#26617,#26618,#26619,#26620,#26621,#26622,#26623,
#26624,#26625,#26626,#26627,#26628,#26629,#26630,#26631,#26632,#26633,#26634,
#26635,#26636,#26637,#26638,#26639,#26640,#26641,#26642,#26643,#26644,#26645,
#26646,#26647,#26648,#26649,#26650,#26651,#26652,#26653,#26654,#26655,#26656,
#26657,#26658,#26659,#26660,#26661,#26662,#26663,#26664,#26665,#26666,#26667,
#26668,#26669,#26670,#26671,#26672,#26673,#26674,#26675,#26676,#26677,#26678,
#26679,#26680,#26681,#26682,#26683,#26684,#26685,#26686,#26687,#26688,#26689,
#26690,#26691,#26692,#26693,#26694,#26695,#26696),.UNSPECIFIED.,.F.,.F.,
(4,2,2,2,2,2,2,2,2,2,2,2,2,2,2,2,2,2,2,2,2,2,2,2,2,2,2,2,2,2,2,2,2,2,2,
2,2,2,2,2,2,2,2,2,2,2,2,2,2,2,2,2,2,2,2,2,2,2,2,2,2,2,2,2,2,2,2,2,2,2,2,
2,2,2,2,2,2,2,2,2,2,2,2,2,2,2,2,2,2,2,2,2,2,2,2,2,2,2,2,2,2,2,2,2,4),(-1.58797213626332,
-1.5851929007491,-1.5663422844173,-1.51419113504517,-1.49831169608799,-1.49554225745563,
-1.49404834616904,-1.49279174156747,-1.49121437593086,-1.48814317787937,
-1.46703177656211,-1.41614769494923,-1.40097955905269,-1.39688603160707,
-1.39439474632506,-1.39213887207933,-1.38923716471809,-1.38455625656101,
-1.34767100094664,-1.31220497116264,-1.29859999805051,-1.2959386080392,
-1.29446795206325,-1.29320937908204,-1.29160184711831,-1.28902033922292,
-1.27422728704706,-1.2704075810326,-1.25750066205839,-1.20583112652477,
-1.19976368995687,-1.19646809061598,-1.19417002883725,-1.19182259665336,
-1.18839578697113,-1.17916635650738,-1.12562321929112,-1.09988575134419,
-1.09675565798519,-1.09516571459432,-1.09390836805184,-1.09242444874957,
-1.08970172541419,-1.07486675030426,-1.03169035384809,-1.00362467498763,
-0.999084627258315,-0.996225166722573,-0.993974121173912,-0.991459211339525,
-0.98725874516619,-0.970822265571422,-0.909425777807314,-0.899269227848342,
-0.896741808908697,-0.895285306637434,-0.894036620311793,-0.892414479487631,
-0.889016543084278,-0.859688219414146,-0.806342908280219,-0.79989390930073,
-0.796904624741144,-0.794628474582261,-0.792199789842373,-0.788392523505356,
-0.776131794161726,-0.755719113906674,-0.723641362493661,-0.717161664297247,
-0.710306326389501,-0.699775968838783,-0.697217776842032,-0.695754280985651,
-0.694494670686153,-0.692876520728066,-0.689498760586868,-0.65523219478018,
-0.607696342518147,-0.600711970852484,-0.597871687747316,-0.595767030877307,
-0.59346984196221,-0.590303667014539,-0.582766833567633,-0.572257412688759,
-0.5416056563801,-0.52126461190133,-0.514076782525264,-0.500608793142929,
-0.498093774263695,-0.496506300997038,-0.495249084389736,-0.493763178101448,
-0.491031291730914,-0.476000215818838,-0.431365170330414,-0.404886988352848,
-0.400388542027565,-0.397541633132385,-0.395291889687219,-0.39276946027005,
-0.388534951295831,-0.371669015387297,-0.331262636501411),.UNSPECIFIED.);
#434=B_SPLINE_CURVE_WITH_KNOTS('',3,(#26702,#26703,#26704,#26705,#26706,
#26707,#26708,#26709,#26710),.UNSPECIFIED.,.F.,.F.,(4,1,1,1,1,1,4),(65.9734457253857,
66.1757532129241,67.1734703764717,68.1711875400193,69.1689047035669,70.1666218671145,
70.6036277493768),.UNSPECIFIED.);
#435=B_SPLINE_CURVE_WITH_KNOTS('',3,(#26711,#26712,#26713,#26714,#26715,
#26716,#26717,#26718,#26719,#26720,#26721,#26722,#26723,#26724,#26725,#26726,
#26727,#26728,#26729,#26730,#26731,#26732,#26733,#26734,#26735,#26736,#26737,
#26738,#26739,#26740,#26741,#26742,#26743,#26744,#26745,#26746,#26747,#26748,
#26749,#26750,#26751,#26752,#26753,#26754,#26755,#26756,#26757,#26758,#26759,
#26760,#26761,#26762,#26763,#26764,#26765,#26766),.UNSPECIFIED.,.F.,.F.,
(4,2,2,2,2,2,2,2,2,2,2,2,2,2,2,2,2,2,2,2,2,2,2,2,2,2,2,4),(-2.51394155306699,
-2.466637600994,-2.4617427397929,-2.45762045848769,-2.45512266136964,-2.45286794636516,
-2.44997755319159,-2.44533497805284,-2.40601539242209,-2.38392710713627,
-2.36049431156025,-2.35724775535317,-2.35593199396106,-2.3546288135796,
-2.35344713167725,-2.35150779911278,-2.34659141335136,-2.30853132004468,
-2.27817622236129,-2.26772679171622,-2.2602956332158,-2.25710544234426,
-2.25480391126825,-2.25270422506788,-2.24988409942968,-2.2430165150615,
-2.19405343286759,-2.18319200174337),.UNSPECIFIED.);
#436=B_SPLINE_CURVE_WITH_KNOTS('',3,(#26768,#26769,#26770,#26771,#26772,
#26773,#26774,#26775,#26776,#26777,#26778,#26779,#26780,#26781,#26782,#26783,
#26784,#26785,#26786,#26787,#26788,#26789,#26790,#26791,#26792,#26793,#26794,
#26795,#26796,#26797,#26798,#26799,#26800,#26801,#26802,#26803,#26804,#26805,
#26806,#26807,#26808,#26809,#26810,#26811,#26812,#26813,#26814,#26815,#26816,
#26817,#26818,#26819,#26820,#26821,#26822,#26823,#26824,#26825,#26826,#26827,
#26828,#26829,#26830,#26831,#26832,#26833,#26834,#26835,#26836,#26837,#26838,
#26839,#26840,#26841,#26842,#26843,#26844,#26845,#26846,#26847,#26848,#26849,
#26850,#26851,#26852,#26853,#26854,#26855,#26856,#26857,#26858,#26859),
 .UNSPECIFIED.,.F.,.F.,(4,2,2,2,2,2,2,2,2,2,2,2,2,2,2,2,2,2,2,2,2,2,2,2,
2,2,2,2,2,2,2,2,2,2,2,2,2,2,2,2,2,2,2,2,2,4),(-0.331262636501411,-0.312537078033625,
-0.300832996363419,-0.298187411773189,-0.296703916745071,-0.295446313583396,
-0.293855270118835,-0.290615749906918,-0.286356679162698,-0.276030209491528,
-0.228465125088051,-0.205056141648706,-0.200292075512775,-0.197657880779281,
-0.195582052980325,-0.195490067650667,-0.195407293701803,-0.195331674364844,
-0.195261724972701,-0.195196335329914,-0.195134650617439,-0.195075995992206,
-0.195019826822999,-0.194965694784247,-0.194913223937621,-0.194862093538244,
-0.194812025352817,-0.194762774111738,-0.19471412011704,-0.194665863532038,
-0.191834663234259,-0.185628295894901,-0.161570327181278,-0.120953101159568,
-0.116450037651974,-0.101616979484438,-0.099033135339379,-0.0974247572295934,
-0.096165915090873,-0.0946953889985359,-0.0920353584835478,-0.0784614972025078,
-0.0467598687421659,-0.00940609176814624,-0.00362882690152282,-0.000621359024833994),
 .UNSPECIFIED.);
#437=B_SPLINE_CURVE_WITH_KNOTS('',3,(#26860,#26861,#26862,#26863,#26864,
#26865,#26866,#26867,#26868),.UNSPECIFIED.,.F.,.F.,(4,1,1,1,1,1,4),(65.9734457253857,
66.4908371924601,67.4885543560077,68.4862715195553,69.4839886831029,70.4817058466505,
70.6039745846252),.UNSPECIFIED.);
#438=B_SPLINE_CURVE_WITH_KNOTS('',3,(#26874,#26875,#26876,#26877,#26878,
#26879,#26880,#26881,#26882,#26883,#26884,#26885,#26886,#26887,#26888,#26889,
#26890,#26891,#26892,#26893,#26894,#26895,#26896,#26897,#26898,#26899,#26900,
#26901,#26902,#26903,#26904,#26905,#26906,#26907,#26908,#26909,#26910,#26911,
#26912,#26913,#26914,#26915,#26916,#26917,#26918,#26919,#26920,#26921,#26922,
#26923,#26924,#26925,#26926,#26927,#26928,#26929,#26930,#26931,#26932,#26933,
#26934,#26935,#26936,#26937,#26938,#26939,#26940,#26941,#26942,#26943,#26944,
#26945,#26946,#26947,#26948,#26949,#26950,#26951,#26952,#26953,#26954,#26955,
#26956,#26957,#26958,#26959,#26960,#26961,#26962,#26963,#26964,#26965,#26966,
#26967,#26968,#26969,#26970,#26971,#26972,#26973,#26974,#26975,#26976,#26977,
#26978,#26979,#26980,#26981,#26982,#26983,#26984,#26985,#26986,#26987,#26988,
#26989,#26990,#26991,#26992,#26993,#26994,#26995,#26996,#26997,#26998,#26999,
#27000,#27001,#27002,#27003,#27004,#27005,#27006,#27007,#27008,#27009,#27010,
#27011,#27012),.UNSPECIFIED.,.F.,.F.,(4,3,3,3,3,3,3,3,3,3,3,3,3,3,3,3,3,
3,3,3,3,3,3,3,3,3,3,3,3,3,3,3,3,3,3,3,3,3,3,3,3,3,3,3,3,3,4),(72.2566313142932,
72.3602645627545,72.4637412961988,72.567131952733,72.670473758299,72.7738038687084,
72.8772298862312,72.9807049395385,73.0843641198611,73.1597733577573,73.2647320310558,
73.3695332432659,73.474211236588,73.5788234142111,73.6834053394952,73.7879925318276,
73.8926903737461,73.9974494450646,74.1023905972613,74.157490521305,74.2624491946034,
74.3672504068134,74.4719284001355,74.5765405777585,74.6811225030425,74.7857096953747,
74.8904075372932,74.9951666086117,75.1001077608083,75.1552076848526,75.2601663581511,
75.3649675703609,75.469645563683,75.5742577413061,75.6788396665902,75.783426858922,
75.8881247008404,75.9928837721588,76.0978249243555,76.1529248484002,76.2578569199746,
76.3626439379309,76.4673216974341,76.5719713509118,76.6765579426452,76.7812391269951,
76.8859203113449),.UNSPECIFIED.);
#439=B_SPLINE_CURVE_WITH_KNOTS('',3,(#27013,#27014,#27015,#27016,#27017,
#27018),.UNSPECIFIED.,.F.,.F.,(4,1,1,4),(70.6036277493768,71.1643390306621,
72.1620561942097,72.2566310325653),.UNSPECIFIED.);
#440=B_SPLINE_CURVE_WITH_KNOTS('',3,(#27020,#27021,#27022,#27023,#27024),
 .UNSPECIFIED.,.F.,.F.,(4,1,4),(70.6039745846252,71.4794230101981,72.2566298138773),
 .UNSPECIFIED.);
#441=B_SPLINE_CURVE_WITH_KNOTS('',3,(#27025,#27026,#27027,#27028,#27029,
#27030,#27031,#27032,#27033,#27034,#27035,#27036,#27037,#27038,#27039,#27040,
#27041,#27042,#27043,#27044,#27045,#27046,#27047,#27048,#27049,#27050,#27051,
#27052,#27053,#27054,#27055,#27056,#27057,#27058,#27059,#27060,#27061,#27062,
#27063,#27064,#27065,#27066,#27067,#27068,#27069,#27070,#27071,#27072,#27073,
#27074,#27075,#27076,#27077,#27078,#27079,#27080,#27081,#27082,#27083,#27084,
#27085,#27086,#27087,#27088,#27089,#27090,#27091,#27092,#27093,#27094,#27095,
#27096,#27097,#27098,#27099,#27100,#27101,#27102,#27103,#27104,#27105,#27106,
#27107,#27108,#27109,#27110,#27111,#27112,#27113,#27114,#27115,#27116,#27117,
#27118,#27119,#27120,#27121,#27122,#27123,#27124,#27125,#27126,#27127,#27128,
#27129,#27130,#27131,#27132,#27133,#27134,#27135,#27136,#27137,#27138,#27139,
#27140,#27141,#27142,#27143,#27144,#27145,#27146,#27147,#27148,#27149,#27150,
#27151,#27152,#27153,#27154,#27155,#27156,#27157,#27158,#27159,#27160,#27161,
#27162,#27163,#27164,#27165,#27166,#27167,#27168,#27169,#27170,#27171,#27172,
#27173,#27174,#27175,#27176,#27177,#27178,#27179,#27180,#27181,#27182,#27183,
#27184,#27185,#27186,#27187,#27188,#27189,#27190),.UNSPECIFIED.,.F.,.F.,
(4,2,2,2,2,2,2,2,2,2,2,2,2,2,2,2,2,2,2,2,2,2,2,2,2,2,2,2,2,2,2,2,2,2,2,
2,2,2,2,2,2,2,2,2,2,2,2,2,2,2,2,2,2,2,2,2,2,2,2,2,2,2,2,2,2,2,2,2,2,2,2,
2,2,2,2,2,2,2,2,2,2,2,4),(-2.51330016705752,-2.47991256274182,-2.47529421864695,
-2.4728770419069,-2.47132370811844,-2.4698596046738,-2.46860064517186,-2.4669848530403,
-2.46437511981821,-2.44905909909445,-2.43145075979571,-2.40980862070163,
-2.38441020802264,-2.37554419845501,-2.37294406094825,-2.37043126395865,
-2.36818048880956,-2.36531915807952,-2.36077166539362,-2.33242979206749,
-2.29028115258029,-2.27985543836915,-2.27556886743201,-2.27238212011941,
-2.27076428981524,-2.26951646673672,-2.26805808971772,-2.26552097690678,
-2.25524029574819,-2.19403330477267,-2.18319928172661,-2.17548453064293,
-2.17228976555339,-2.16998810430565,-2.16789046670598,-2.16454458651877,
-2.15828727472907,-2.10862815690352,-2.07872439634806,-2.07358234294318,
-2.07166740114468,-2.07036050990824,-2.06918313579971,-2.06726539847066,
-2.0624752654823,-2.03120494517,-2.00474676260167,-1.98139779817127,-1.97528812501293,
-1.97237746645103,-1.97012089964132,-1.96763517933785,-1.96356529556603,
-1.95025468714898,-1.94074376402126,-1.89135754142829,-1.87576111808876,
-1.8730042864536,-1.87151325004914,-1.87025672840254,-1.86867651365306,
-1.86559114622134,-1.84390124485284,-1.80799875526818,-1.78930432285737,
-1.78162123549416,-1.77571718100365,-1.77284603762069,-1.77059403159059,
-1.76808656862234,-1.76391866536552,-1.74969554545172,-1.74008836109247,
-1.69176924791012,-1.68138250321778,-1.67502498943512,-1.67294800552402,
-1.67160635405697,-1.67031862047412,-1.66843544979252,-1.66385338009683,
-1.62422138514652,-1.58784062522319),.UNSPECIFIED.);
#442=B_SPLINE_CURVE_WITH_KNOTS('',3,(#27196,#27197,#27198,#27199,#27200,
#27201,#27202,#27203,#27204,#27205,#27206,#27207,#27208,#27209,#27210,#27211,
#27212,#27213,#27214,#27215,#27216,#27217,#27218,#27219,#27220,#27221,#27222,
#27223,#27224,#27225,#27226,#27227,#27228,#27229,#27230,#27231,#27232,#27233,
#27234,#27235,#27236,#27237,#27238,#27239,#27240,#27241,#27242,#27243,#27244,
#27245,#27246,#27247,#27248,#27249,#27250,#27251,#27252,#27253,#27254,#27255,
#27256,#27257,#27258,#27259,#27260,#27261,#27262,#27263,#27264,#27265,#27266,
#27267,#27268,#27269,#27270,#27271,#27272,#27273,#27274,#27275,#27276,#27277,
#27278,#27279,#27280,#27281,#27282,#27283,#27284,#27285,#27286,#27287,#27288,
#27289,#27290,#27291,#27292,#27293,#27294,#27295,#27296,#27297,#27298,#27299,
#27300,#27301,#27302,#27303,#27304,#27305,#27306,#27307,#27308,#27309,#27310,
#27311,#27312,#27313,#27314,#27315,#27316,#27317,#27318,#27319,#27320,#27321,
#27322,#27323,#27324,#27325,#27326,#27327,#27328,#27329,#27330,#27331,#27332,
#27333,#27334,#27335,#27336,#27337,#27338,#27339,#27340,#27341,#27342,#27343,
#27344,#27345,#27346,#27347,#27348,#27349,#27350,#27351,#27352,#27353,#27354,
#27355,#27356,#27357,#27358,#27359,#27360,#27361,#27362,#27363,#27364,#27365,
#27366,#27367),.UNSPECIFIED.,.F.,.F.,(4,2,2,2,2,2,2,2,2,2,2,2,2,2,2,2,2,
2,2,2,2,2,2,2,2,2,2,2,2,2,2,2,2,2,2,2,2,2,2,2,2,2,2,2,2,2,2,2,2,2,2,2,2,
2,2,2,2,2,2,2,2,2,2,2,2,2,2,2,2,2,2,2,2,2,2,2,2,2,2,2,2,2,2,2,2,4),(-0.926807318156856,
-0.925373376894712,-0.922713571027084,-0.921082197429211,-0.919820983452259,
-0.918365503869921,-0.915775850211289,-0.90345491509868,-0.874298322310961,
-0.833079534301998,-0.825834080675445,-0.822948939119945,-0.820832544766051,
-0.818543164258394,-0.815424891538882,-0.80817547098942,-0.798184089328335,
-0.747211001922924,-0.726077872881513,-0.723004874505717,-0.721426667831066,
-0.720169431854571,-0.718674782275535,-0.715903998226448,-0.700014398287469,
-0.647755460227258,-0.6290304993301,-0.624521689505782,-0.621911878994728,
-0.619670455078301,-0.61694400867495,-0.611763386103654,-0.566763233892935,
-0.528911052604525,-0.524235744475249,-0.522336329847796,-0.521161656910474,
-0.519849451286753,-0.517912226725937,-0.512621818685951,-0.504546114369096,
-0.451475453742175,-0.443037867787702,-0.428727097014748,-0.424548478078506,
-0.422037670582143,-0.419784616041472,-0.416914813247638,-0.41102309633798,
-0.369520376990956,-0.329162402132365,-0.324603233221116,-0.322909765846531,
-0.32170959020882,-0.320421249380948,-0.318605707999499,-0.314117460590152,
-0.291589075693152,-0.282497019545978,-0.233799987062063,-0.226907837373905,
-0.22408277986961,-0.221981296203417,-0.219725598053063,-0.21664096372067,
-0.213179056558184,-0.207203429930074,-0.1942258004651,-0.147710486661316,
-0.139797729375172,-0.126759667223844,-0.124267477631899,-0.122686546961463,
-0.121429143446021,-0.119936657983165,-0.117176084710195,-0.101525116676944,
-0.0480775700168125,-0.0330517577391862,-0.0268002465373971,-0.0238929708442883,
-0.0216289297483238,-0.019528173283468,-0.0171074106056456,-0.0136712472908266,
-0.000589101730667486),.UNSPECIFIED.);
#443=B_SPLINE_CURVE_WITH_KNOTS('',3,(#27368,#27369,#27370,#27371,#27372,
#27373,#27374,#27375,#27376,#27377,#27378,#27379,#27380,#27381,#27382,#27383,
#27384,#27385,#27386,#27387,#27388,#27389,#27390,#27391,#27392,#27393,#27394,
#27395,#27396,#27397,#27398,#27399,#27400,#27401,#27402,#27403,#27404,#27405,
#27406,#27407,#27408,#27409,#27410,#27411,#27412,#27413,#27414,#27415,#27416,
#27417,#27418,#27419),.UNSPECIFIED.,.F.,.F.,(4,3,3,3,3,3,3,3,3,3,3,3,3,
3,3,3,3,4),(76.8859203113449,76.9906794404996,77.095620626684,77.1506420119478,
77.2556006852461,77.3604018974561,77.4650798907783,77.5696920684015,77.6742739936856,
77.7788611860176,77.8835590279362,77.9883180992548,78.0932592514514,78.1483591754954,
78.2655869204099,78.382405937241,78.4985506711647,78.5398163393789),
 .UNSPECIFIED.);
#444=B_SPLINE_CURVE_WITH_KNOTS('',3,(#27420,#27421,#27422,#27423,#27424,
#27425,#27426,#27427,#27428,#27429,#27430,#27431,#27432,#27433,#27434,#27435,
#27436,#27437,#27438,#27439,#27440,#27441,#27442,#27443,#27444,#27445,#27446,
#27447,#27448,#27449,#27450,#27451,#27452,#27453,#27454,#27455,#27456,#27457,
#27458,#27459,#27460,#27461,#27462,#27463,#27464,#27465,#27466,#27467,#27468,
#27469,#27470,#27471,#27472,#27473,#27474,#27475,#27476,#27477,#27478,#27479,
#27480,#27481,#27482,#27483,#27484,#27485,#27486,#27487,#27488,#27489,#27490,
#27491,#27492,#27493,#27494,#27495,#27496,#27497,#27498,#27499,#27500,#27501,
#27502,#27503,#27504,#27505,#27506,#27507,#27508,#27509,#27510,#27511,#27512,
#27513,#27514,#27515,#27516,#27517,#27518,#27519,#27520,#27521,#27522,#27523,
#27524,#27525,#27526,#27527,#27528,#27529,#27530,#27531,#27532,#27533,#27534,
#27535,#27536,#27537,#27538,#27539,#27540,#27541,#27542,#27543,#27544,#27545,
#27546,#27547,#27548,#27549,#27550,#27551,#27552,#27553,#27554,#27555,#27556,
#27557,#27558,#27559,#27560,#27561,#27562,#27563,#27564,#27565,#27566,#27567,
#27568,#27569,#27570,#27571,#27572,#27573,#27574,#27575,#27576,#27577,#27578,
#27579,#27580,#27581,#27582,#27583,#27584,#27585,#27586,#27587,#27588,#27589,
#27590,#27591,#27592,#27593,#27594,#27595,#27596,#27597,#27598,#27599,#27600,
#27601,#27602,#27603,#27604,#27605,#27606,#27607,#27608,#27609,#27610,#27611,
#27612,#27613,#27614,#27615,#27616,#27617,#27618,#27619,#27620,#27621,#27622,
#27623,#27624,#27625,#27626,#27627,#27628,#27629,#27630,#27631,#27632,#27633,
#27634,#27635,#27636,#27637,#27638,#27639,#27640,#27641,#27642,#27643),
 .UNSPECIFIED.,.F.,.F.,(4,2,2,2,2,2,2,2,2,2,2,2,2,2,2,2,2,2,2,2,2,2,2,2,
2,2,2,2,2,2,2,2,2,2,2,2,2,2,2,2,2,2,2,2,2,2,2,2,2,2,2,2,2,2,2,2,2,2,2,2,
2,2,2,2,2,2,2,2,2,2,2,2,2,2,2,2,2,2,2,2,2,2,2,2,2,2,2,2,2,2,2,2,2,2,2,2,
2,2,2,2,2,2,2,2,2,2,2,2,2,2,2,4),(-1.58784062522319,-1.58221103954342,-1.57624379253658,
-1.57336030004944,-1.57110678889273,-1.5686060511992,-1.56446898299355,
-1.55054031333842,-1.5403996123742,-1.48844940522033,-1.48044057016584,
-1.47518385362657,-1.47325207147764,-1.47194149333888,-1.47076672597767,
-1.4688643037845,-1.46416735823224,-1.42685748453031,-1.39571037012948,
-1.3796441492217,-1.37547399866116,-1.37296582418165,-1.3707135833922,-1.36784269676348,
-1.36326452976911,-1.3338661568848,-1.28269358222039,-1.27823077797614,
-1.27487063935757,-1.2732559658949,-1.27199671755082,-1.27053092911233,
-1.26796255187546,-1.25730409551706,-1.23402934605179,-1.18466678326279,
-1.17768802828592,-1.17492424917217,-1.1726295664007,-1.17027763960127,
-1.16682955455234,-1.15745100760379,-1.14341407555502,-1.09000305083113,
-1.07762655782137,-1.07517309973763,-1.07360431720513,-1.07234799098609,
-1.07084660405032,-1.06804254251476,-1.05131907054971,-1.02219495066418,
-0.9823059764507,-0.977656020347348,-0.974763331421145,-0.972508259456574,
-0.970011535578737,-0.965894451670222,-0.950461926067842,-0.898434063152091,
-0.892358085407629,-0.878254646857698,-0.875706396014921,-0.874108733593552,
-0.872850670815167,-0.871372190868561,-0.868675453697037,-0.854386645095842,
-0.83379807270375,-0.785706357108745,-0.77876249055942,-0.775929036702919,
-0.773825952992545,-0.771527079904415,-0.768352342853144,-0.760764958496427,
-0.750163951228377,-0.71905093550358,-0.681637270713771,-0.676937307973491,
-0.67503413336087,-0.673859046308614,-0.672548249224625,-0.670616392034461,
-0.665360920851439,-0.657356160705935,-0.605467264792169,-0.595107241660825,
-0.581320178577621,-0.577197514745334,-0.574699536054711,-0.572444695775254,
-0.569554203330038,-0.563553117135836,-0.519029241755175,-0.482077028959812,
-0.477362993831511,-0.475457459290951,-0.474281934789479,-0.472971637895728,
-0.471042237212878,-0.465803971318245,-0.434699629213652,-0.386567694011509,
-0.379627406296936,-0.376794578242346,-0.374691656841344,-0.372392666182983,
-0.369217224770673,-0.361625527917048,-0.351016654667816,-0.331163854026367),
 .UNSPECIFIED.);
#445=B_SPLINE_CURVE_WITH_KNOTS('',3,(#27648,#27649,#27650,#27651,#27652,
#27653,#27654,#27655,#27656,#27657,#27658,#27659,#27660,#27661,#27662,#27663,
#27664,#27665,#27666,#27667,#27668,#27669,#27670,#27671,#27672,#27673,#27674,
#27675,#27676,#27677,#27678,#27679,#27680,#27681,#27682,#27683,#27684,#27685,
#27686,#27687,#27688,#27689,#27690,#27691,#27692,#27693,#27694,#27695,#27696,
#27697,#27698,#27699,#27700,#27701,#27702,#27703,#27704,#27705,#27706,#27707,
#27708,#27709,#27710,#27711,#27712,#27713,#27714,#27715,#27716,#27717,#27718,
#27719,#27720,#27721,#27722,#27723,#27724,#27725,#27726,#27727,#27728,#27729,
#27730,#27731,#27732,#27733,#27734,#27735,#27736,#27737,#27738,#27739,#27740,
#27741,#27742,#27743,#27744,#27745,#27746,#27747,#27748,#27749,#27750,#27751,
#27752,#27753,#27754,#27755,#27756,#27757,#27758,#27759,#27760,#27761,#27762,
#27763,#27764,#27765,#27766,#27767,#27768,#27769,#27770,#27771,#27772,#27773,
#27774,#27775,#27776,#27777,#27778,#27779,#27780,#27781,#27782,#27783,#27784,
#27785,#27786,#27787,#27788,#27789,#27790,#27791,#27792,#27793,#27794,#27795,
#27796,#27797,#27798,#27799,#27800,#27801,#27802,#27803,#27804,#27805,#27806,
#27807,#27808,#27809,#27810,#27811,#27812,#27813,#27814,#27815,#27816,#27817,
#27818,#27819,#27820,#27821,#27822,#27823,#27824,#27825,#27826,#27827,#27828,
#27829,#27830,#27831,#27832,#27833,#27834,#27835,#27836,#27837,#27838,#27839,
#27840,#27841,#27842,#27843,#27844,#27845,#27846,#27847,#27848,#27849,#27850,
#27851),.UNSPECIFIED.,.F.,.F.,(4,2,2,2,2,2,2,2,2,2,2,2,2,2,2,2,2,2,2,2,
2,2,2,2,2,2,2,2,2,2,2,2,2,2,2,2,2,2,2,2,2,2,2,2,2,2,2,2,2,2,2,2,2,2,2,2,
2,2,2,2,2,2,2,2,2,2,2,2,2,2,2,2,2,2,2,2,2,2,2,2,2,2,2,2,2,2,2,2,2,2,2,2,
2,2,2,2,2,2,2,2,2,4),(-2.18351281682041,-2.18101681610237,-2.1372290852562,
-2.12230855412162,-2.11958131522797,-2.11809621566542,-2.11683862965526,
-2.11524933235074,-2.11212331065142,-2.08108951867406,-2.04334702308628,
-2.02549204063445,-2.02118247014029,-2.01864315334134,-2.01639543379035,
-2.01357392767378,-2.00916030230868,-1.98481735473266,-1.94652470527624,
-1.92531954767722,-1.9209651494158,-1.91917173531293,-1.91788759929618,
-1.91668201002598,-1.9146197520273,-1.90890717017128,-1.86602816708059,
-1.82738618997019,-1.82228356652633,-1.81957374242647,-1.81735452457443,
-1.81473979965965,-1.81020797347806,-1.79114276621091,-1.73921311664175,
-1.723353900045,-1.720584705783,-1.7190905623037,-1.7178335390829,-1.71625533803371,
-1.71318159035454,-1.69201279303018,-1.64100155323564,-1.63108288676515,
-1.62387392809614,-1.62076290641904,-1.61847505178503,-1.61635738373742,
-1.61290670811308,-1.6042227764439,-1.54679198967744,-1.5313036791489,-1.52570400233818,
-1.5216955570262,-1.51996082054256,-1.51868632399239,-1.51728732222685,
-1.51495338261783,-1.5070907376698,-1.44322790731788,-1.42660968236939,
-1.42239416762734,-1.41987559198117,-1.41762460781561,-1.41476976814698,
-1.41024606415742,-1.38274738846111,-1.33902026916804,-1.32410781823506,
-1.32138092997059,-1.31989589425515,-1.31863828554251,-1.3170488618652,
-1.31452805404872,-1.30095653388421,-1.294006931938,-1.25769731442286,-1.22865277151619,
-1.22408373627076,-1.22121511994126,-1.2189625206458,-1.21645172735011,
-1.21227197191485,-1.19609988066308,-1.13765288145582,-1.12462434190597,
-1.12213286299651,-1.12055223188168,-1.11929496323575,-1.11780251585233,
-1.1150416935152,-1.0993801385356,-1.04939480462388,-1.02844500712769,-1.02419649919778,
-1.02142533428652,-1.0191815040607,-1.016607034876,-1.0121377570243,-0.991906648634121,
-0.941860362376527,-0.926807318156856),.UNSPECIFIED.);
#446=B_SPLINE_CURVE_WITH_KNOTS('',3,(#27853,#27854,#27855,#27856,#27857,
#27858,#27859,#27860,#27861,#27862,#27863,#27864,#27865,#27866,#27867,#27868,
#27869,#27870,#27871,#27872,#27873,#27874,#27875,#27876,#27877,#27878,#27879,
#27880,#27881,#27882,#27883,#27884,#27885,#27886,#27887,#27888,#27889,#27890,
#27891,#27892,#27893,#27894,#27895,#27896,#27897,#27898,#27899,#27900,#27901,
#27902,#27903,#27904,#27905,#27906,#27907,#27908,#27909,#27910),
 .UNSPECIFIED.,.F.,.F.,(4,2,2,2,2,2,2,2,2,2,2,2,2,2,2,2,2,2,2,2,2,2,2,2,
2,2,2,2,4),(-0.331163854026367,-0.319863441156325,-0.282506835646621,-0.277805204671239,
-0.275901757877679,-0.274726626002702,-0.273415898471444,-0.271484352001104,
-0.26623100329555,-0.258230573221689,-0.206412150061396,-0.183470942609572,
-0.179123961518021,-0.176322980558378,-0.174077374758578,-0.171620148404089,
-0.167481878800948,-0.162478015590372,-0.152386304442785,-0.125059925231917,
-0.0825698578329224,-0.0781441494796792,-0.0764693740893651,-0.0752744619194422,
-0.0739829355785006,-0.0721483906077727,-0.0675390301218784,-0.0437529782176269,
-0.000590121595483474),.UNSPECIFIED.);
#447=B_SPLINE_CURVE_WITH_KNOTS('',3,(#27911,#27912,#27913,#27914,#27915,
#27916,#27917,#27918,#27919,#27920,#27921,#27922,#27923,#27924,#27925,#27926,
#27927,#27928,#27929,#27930,#27931,#27932,#27933,#27934,#27935,#27936,#27937,
#27938,#27939,#27940,#27941,#27942,#27943,#27944,#27945,#27946,#27947,#27948,
#27949,#27950,#27951,#27952,#27953,#27954,#27955,#27956,#27957,#27958,#27959,
#27960,#27961,#27962,#27963,#27964,#27965,#27966,#27967,#27968,#27969,#27970,
#27971,#27972,#27973,#27974,#27975,#27976,#27977,#27978,#27979,#27980,#27981,
#27982,#27983,#27984,#27985,#27986,#27987,#27988,#27989,#27990,#27991,#27992,
#27993,#27994,#27995,#27996,#27997,#27998,#27999,#28000,#28001,#28002,#28003,
#28004,#28005,#28006,#28007,#28008,#28009,#28010,#28011,#28012,#28013,#28014,
#28015,#28016,#28017,#28018,#28019,#28020,#28021,#28022,#28023,#28024,#28025,
#28026,#28027,#28028,#28029,#28030,#28031,#28032,#28033,#28034,#28035,#28036,
#28037,#28038,#28039,#28040,#28041,#28042,#28043,#28044,#28045,#28046,#28047,
#28048,#28049,#28050,#28051,#28052,#28053,#28054,#28055,#28056,#28057,#28058,
#28059,#28060,#28061,#28062,#28063,#28064,#28065,#28066,#28067,#28068,#28069,
#28070,#28071,#28072,#28073,#28074,#28075,#28076,#28077,#28078,#28079,#28080,
#28081,#28082,#28083,#28084,#28085,#28086,#28087,#28088,#28089,#28090,#28091,
#28092),.UNSPECIFIED.,.F.,.F.,(4,2,2,2,2,2,2,2,2,2,2,2,2,2,2,2,2,2,2,2,
2,2,2,2,2,2,2,2,2,2,2,2,2,2,2,2,2,2,2,2,2,2,2,2,2,2,2,2,2,2,2,2,2,2,2,2,
2,2,2,2,2,2,2,2,2,2,2,2,2,2,2,2,2,2,2,2,2,2,2,2,2,2,2,2,2,2,2,2,2,2,4),
(-2.51353945094856,-2.50220186507432,-2.49527542065432,-2.4923592038255,
-2.4901372269883,-2.48799464166275,-2.48587512033717,-2.48240866365923,
-2.47361280374915,-2.45880492184982,-2.40618900205649,-2.39313758226095,
-2.3905069447287,-2.38904325567487,-2.38778433848214,-2.38616819344917,
-2.38355710255715,-2.36822767398951,-2.31716309211462,-2.30372540991668,
-2.2976034428148,-2.29271602857679,-2.29006856305797,-2.29004487329658,
-2.2900206881505,-2.28999599511909,-2.28997078131414,-2.28994503347818,
-2.28991873800238,-2.28789976666376,-2.28529951635349,-2.28082673225287,
-2.26259338861597,-2.20983409160828,-2.1939004978952,-2.19112940705993,
-2.18963541990004,-2.18837923418689,-2.18680300330163,-2.1837357838108,
-2.16272443384726,-2.11187846482913,-2.09661162278341,-2.09251027500257,
-2.0900177539398,-2.08776303461586,-2.08486599196874,-2.08019913913287,
-2.04067387747045,-2.00775269183138,-1.99423646712642,-1.99158039115654,
-1.99011116142325,-1.98885286758129,-1.98724447781428,-1.98465927006454,
-1.96977723397764,-1.9657112920977,-1.92484159572174,-1.90074633741755,
-1.89453602685366,-1.89160633467944,-1.88934741998761,-1.88687152921894,
-1.88284584064097,-1.86992814297236,-1.86106762445878,-1.81066778903153,
-1.79496500775627,-1.7922036682246,-1.79071171582063,-1.78945532751888,
-1.78787642461829,-1.78538884343792,-1.77240851787872,-1.7644681380549,
-1.71798280984101,-1.69832496422443,-1.6938938206752,-1.69132871223749,
-1.68908556850196,-1.68630559324293,-1.68202529533571,-1.66054121399684,
-1.61108208154023,-1.59547781481612,-1.59272064160989,-1.59122953241725,
-1.58997301610867,-1.58839289240738,-1.58779384257567),.UNSPECIFIED.);
#448=B_SPLINE_CURVE_WITH_KNOTS('',3,(#28098,#28099,#28100,#28101,#28102,
#28103,#28104,#28105,#28106,#28107,#28108,#28109,#28110,#28111,#28112,#28113,
#28114,#28115,#28116,#28117,#28118,#28119,#28120,#28121,#28122,#28123,#28124,
#28125,#28126,#28127,#28128,#28129,#28130,#28131,#28132,#28133,#28134,#28135,
#28136,#28137,#28138,#28139,#28140,#28141,#28142,#28143,#28144,#28145,#28146,
#28147,#28148,#28149,#28150,#28151,#28152,#28153,#28154,#28155,#28156,#28157,
#28158,#28159,#28160,#28161,#28162,#28163,#28164,#28165,#28166,#28167,#28168,
#28169,#28170,#28171,#28172,#28173,#28174,#28175,#28176,#28177,#28178,#28179,
#28180,#28181,#28182,#28183,#28184,#28185,#28186,#28187,#28188,#28189,#28190,
#28191,#28192,#28193,#28194,#28195,#28196,#28197,#28198,#28199,#28200,#28201,
#28202,#28203,#28204,#28205,#28206,#28207,#28208,#28209,#28210,#28211,#28212,
#28213,#28214,#28215,#28216,#28217,#28218,#28219,#28220,#28221,#28222,#28223,
#28224,#28225,#28226,#28227,#28228,#28229,#28230,#28231,#28232,#28233,#28234,
#28235,#28236,#28237,#28238,#28239,#28240,#28241,#28242,#28243,#28244,#28245,
#28246,#28247,#28248,#28249,#28250,#28251,#28252,#28253,#28254,#28255,#28256,
#28257,#28258,#28259,#28260,#28261,#28262,#28263,#28264,#28265,#28266,#28267),
 .UNSPECIFIED.,.F.,.F.,(4,2,2,2,2,2,2,2,2,2,2,2,2,2,2,2,2,2,2,2,2,2,2,2,
2,2,2,2,2,2,2,2,2,2,2,2,2,2,2,2,2,2,2,2,2,2,2,2,2,2,2,2,2,2,2,2,2,2,2,2,
2,2,2,2,2,2,2,2,2,2,2,2,2,2,2,2,2,2,2,2,2,2,2,2,4),(-0.926452780362809,
-0.909637390829123,-0.905229033347337,-0.902409538782332,-0.900162569554983,
-0.897623191808063,-0.893311291056809,-0.875413314360576,-0.828683561839237,
-0.826602189992789,-0.819658396293833,-0.806054498526084,-0.803532363268601,
-0.801942752075319,-0.800685424975685,-0.799201217319981,-0.796477140805644,
-0.781612357380261,-0.738205760173885,-0.71041582483058,-0.705884297560961,
-0.703027417811861,-0.700776653718294,-0.698260229705421,-0.69405286355535,
-0.67752947311056,-0.614988949722869,-0.605919794125388,-0.603461365362065,
-0.602034923473083,-0.600895576046197,-0.599289021167143,-0.595971085594238,
-0.562732826372065,-0.513945411207184,-0.507061002043918,-0.504237813121291,
-0.502137243919294,-0.499836115548513,-0.496649028056098,-0.488986935526028,
-0.478249535149239,-0.418807071527379,-0.4067760496548,-0.404108058120974,
-0.402619354801629,-0.401361957695237,-0.399777010521043,-0.396568755446391,
-0.392362061495167,-0.382219182975904,-0.336833320660837,-0.311146559031905,
-0.306682433989072,-0.303845509941163,-0.301596223973575,-0.29906647174904,
-0.294800719127599,-0.277538402984045,-0.243906241970156,-0.210539914062049,
-0.205761662800579,-0.203876827853335,-0.202607846560628,-0.20131699883905,
-0.199985948362352,-0.198115467943968,-0.185932207224183,-0.157374934046016,
-0.11539442927958,-0.108162898220615,-0.105280301336457,-0.103164725556191,
-0.100875228828571,-0.0977550038494009,-0.0904928011869399,-0.0804782340822814,
-0.0295372784663833,-0.0132637756828869,-0.00675812967874559,-0.00463040526874976,
-0.00325817851213518,-0.00205816246604583,-0.00108891780732919,-0.000589454289888855),
 .UNSPECIFIED.);
#449=B_SPLINE_CURVE_WITH_KNOTS('',3,(#28268,#28269,#28270,#28271,#28272,
#28273,#28274,#28275,#28276,#28277,#28278,#28279,#28280,#28281,#28282,#28283,
#28284,#28285,#28286,#28287,#28288,#28289,#28290,#28291,#28292,#28293,#28294,
#28295,#28296,#28297,#28298,#28299,#28300,#28301,#28302,#28303,#28304,#28305,
#28306,#28307,#28308,#28309,#28310,#28311,#28312,#28313,#28314,#28315,#28316,
#28317,#28318,#28319,#28320,#28321,#28322,#28323,#28324,#28325),
 .UNSPECIFIED.,.F.,.F.,(4,2,2,2,2,2,2,2,2,2,2,2,2,2,2,2,2,2,2,2,2,2,2,2,
2,2,2,2,4),(-2.51424347129331,-2.51298909616975,-2.50974297696382,-2.49086577269954,
-2.43953947552916,-2.42420230201702,-2.42009286305575,-2.41759741122848,
-2.41534131430693,-2.41244427175551,-2.40778102725624,-2.36861356833193,
-2.34088994770667,-2.32822021179079,-2.32332203447788,-2.31970836324781,
-2.3180661535042,-2.31684531340443,-2.31546990813453,-2.31321238005377,
-2.30562425205202,-2.24145067854674,-2.22481168872888,-2.22059456534028,
-2.21807565631282,-2.21582476734007,-2.21297058292729,-2.2084489828068,
-2.18351281682041),.UNSPECIFIED.);
#450=B_SPLINE_CURVE_WITH_KNOTS('',3,(#28326,#28327,#28328,#28329,#28330,
#28331,#28332,#28333,#28334,#28335,#28336,#28337,#28338,#28339,#28340,#28341,
#28342,#28343,#28344,#28345,#28346,#28347,#28348,#28349,#28350,#28351,#28352,
#28353,#28354,#28355,#28356,#28357,#28358,#28359,#28360,#28361,#28362,#28363,
#28364,#28365,#28366,#28367,#28368,#28369,#28370,#28371,#28372,#28373,#28374,
#28375,#28376,#28377,#28378,#28379,#28380,#28381,#28382,#28383,#28384,#28385,
#28386,#28387,#28388,#28389,#28390,#28391,#28392,#28393,#28394,#28395,#28396,
#28397,#28398,#28399,#28400,#28401,#28402,#28403,#28404,#28405,#28406,#28407,
#28408,#28409,#28410,#28411,#28412,#28413,#28414,#28415,#28416,#28417,#28418,
#28419,#28420,#28421,#28422,#28423,#28424,#28425,#28426,#28427,#28428,#28429,
#28430,#28431,#28432,#28433,#28434,#28435,#28436,#28437,#28438,#28439,#28440,
#28441,#28442,#28443,#28444,#28445,#28446,#28447,#28448,#28449,#28450,#28451,
#28452,#28453,#28454,#28455,#28456,#28457,#28458,#28459,#28460,#28461,#28462,
#28463,#28464,#28465,#28466,#28467,#28468,#28469,#28470,#28471,#28472,#28473,
#28474,#28475,#28476,#28477,#28478,#28479,#28480,#28481,#28482,#28483,#28484,
#28485,#28486,#28487,#28488,#28489,#28490,#28491,#28492,#28493,#28494,#28495,
#28496,#28497,#28498,#28499,#28500,#28501,#28502,#28503,#28504,#28505,#28506,
#28507,#28508,#28509,#28510,#28511,#28512,#28513,#28514,#28515,#28516,#28517,
#28518,#28519,#28520,#28521,#28522,#28523,#28524,#28525,#28526,#28527),
 .UNSPECIFIED.,.F.,.F.,(4,2,2,2,2,2,2,2,2,2,2,2,2,2,2,2,2,2,2,2,2,2,2,2,
2,2,2,2,2,2,2,2,2,2,2,2,2,2,2,2,2,2,2,2,2,2,2,2,2,2,2,2,2,2,2,2,2,2,2,2,
2,2,2,2,2,2,2,2,2,2,2,2,2,2,2,2,2,2,2,2,2,2,2,2,2,2,2,2,2,2,2,2,2,2,2,2,
2,2,2,2,4),(-1.58779384257567,-1.58530794947241,-1.56363531377009,-1.5277173334975,
-1.502108239085,-1.4956983741498,-1.49273101241254,-1.49046665410613,-1.48800798875912,
-1.48406165264793,-1.47182624559535,-1.42947772403734,-1.39953940009233,
-1.39439420386491,-1.39247864574392,-1.39117150395504,-1.38999403421244,
-1.38807638593596,-1.38328768519082,-1.35003123001768,-1.3163578787736,
-1.2990850221524,-1.29481979239473,-1.29229086757762,-1.2900426420838,-1.28720749980552,
-1.28274703433158,-1.25712946427265,-1.2309016158967,-1.19974792762863,
-1.19495386378932,-1.19303530967686,-1.19185766863045,-1.19055070335237,
-1.18863604401668,-1.1834970163045,-1.15363841567152,-1.10395251088246,
-1.0976974001608,-1.09435182250629,-1.09225401353284,-1.08995186341681,
-1.08675587422493,-1.07903550863753,-1.06819045349403,-1.00684065986656,
-0.996653163768813,-0.994123460804956,-0.992666602774408,-0.991418250122011,
-0.989797372338245,-0.986404993373701,-0.957262671062231,-0.905738153423709,
-0.897985897829439,-0.894690400011276,-0.892392346577639,-0.890044870833402,
-0.886617901687495,-0.87738745063311,-0.823843874675645,-0.798107568135285,
-0.794977466447497,-0.793387515135325,-0.792130160400013,-0.790646229167718,
-0.787923478132749,-0.773088200049362,-0.729910036825996,-0.70184577967035,
-0.69730574949192,-0.694446284358185,-0.692195225413299,-0.689680290444027,
-0.685479758113578,-0.669042693550401,-0.607639976093929,-0.597488851031956,
-0.594961878846494,-0.593505473381675,-0.592256763100708,-0.590634452145934,
-0.587235670757584,-0.557876756830801,-0.504570747755453,-0.498116529623879,
-0.495126226002401,-0.49284989523288,-0.490421592138919,-0.486616126413661,
-0.474371876822789,-0.453999217792585,-0.422879830155066,-0.398939084188236,
-0.395825093693884,-0.394238486223362,-0.392981235825957,-0.391494444456293,
-0.388758746054412,-0.373647931397671,-0.331223639443211),.UNSPECIFIED.);
#451=B_SPLINE_CURVE_WITH_KNOTS('',3,(#28532,#28533,#28534,#28535,#28536,
#28537,#28538,#28539,#28540,#28541,#28542,#28543,#28544,#28545,#28546,#28547,
#28548,#28549,#28550,#28551,#28552,#28553,#28554,#28555,#28556,#28557,#28558,
#28559,#28560,#28561,#28562,#28563,#28564,#28565,#28566,#28567,#28568,#28569,
#28570,#28571,#28572,#28573,#28574,#28575,#28576,#28577,#28578,#28579,#28580,
#28581,#28582,#28583,#28584,#28585,#28586,#28587,#28588,#28589,#28590,#28591,
#28592,#28593,#28594,#28595,#28596,#28597,#28598,#28599,#28600,#28601,#28602,
#28603,#28604,#28605,#28606,#28607,#28608,#28609,#28610,#28611,#28612,#28613,
#28614,#28615,#28616,#28617,#28618,#28619,#28620,#28621,#28622,#28623,#28624,
#28625,#28626,#28627,#28628,#28629,#28630,#28631,#28632,#28633,#28634,#28635,
#28636,#28637,#28638,#28639,#28640,#28641,#28642,#28643,#28644,#28645,#28646,
#28647,#28648,#28649,#28650,#28651,#28652,#28653,#28654,#28655,#28656,#28657,
#28658,#28659,#28660,#28661,#28662,#28663,#28664,#28665,#28666,#28667,#28668,
#28669,#28670,#28671,#28672,#28673,#28674,#28675,#28676,#28677,#28678,#28679,
#28680,#28681,#28682,#28683,#28684,#28685,#28686,#28687,#28688,#28689,#28690,
#28691,#28692,#28693,#28694,#28695,#28696,#28697,#28698,#28699,#28700,#28701,
#28702,#28703,#28704,#28705,#28706,#28707,#28708,#28709,#28710,#28711,#28712,
#28713,#28714,#28715,#28716,#28717,#28718,#28719,#28720,#28721,#28722,#28723,
#28724,#28725,#28726,#28727,#28728,#28729,#28730,#28731,#28732,#28733),
 .UNSPECIFIED.,.F.,.F.,(4,2,2,2,2,2,2,2,2,2,2,2,2,2,2,2,2,2,2,2,2,2,2,2,
2,2,2,2,2,2,2,2,2,2,2,2,2,2,2,2,2,2,2,2,2,2,2,2,2,2,2,2,2,2,2,2,2,2,2,2,
2,2,2,2,2,2,2,2,2,2,2,2,2,2,2,2,2,2,2,2,2,2,2,2,2,2,2,2,2,2,2,2,2,2,2,2,
2,2,2,2,4),(-2.18264003139251,-2.14598451708076,-2.10816324425232,-2.10222939614988,
-2.0993523865971,-2.09709962472545,-2.09459527428191,-2.09044181082173,
-2.07635722326331,-2.06768237234159,-2.01458815009102,-2.00651223311199,
-2.00122290088457,-1.99928645620989,-1.9979749021351,-1.99680090168871,
-1.99490274494027,-1.99023136912594,-1.95231774782686,-1.90753000941557,
-1.90231067993299,-1.89957704643358,-1.89733637115704,-1.8947349626996,
-1.89025938272062,-1.87198742392528,-1.81926721632703,-1.8033360604423,
-1.80056442705413,-1.79907002736022,-1.797813416199,-1.79623652430868,-1.79316762776359,
-1.7721257845726,-1.72130604146506,-1.70604383032626,-1.70194202418997,
-1.69944887860977,-1.69719336477275,-1.69429497280168,-1.68962524999063,
-1.65465448426018,-1.62954044403999,-1.60654603379918,-1.60201364758044,
-1.60019159491186,-1.59890258516541,-1.59770495083073,-1.59601943672233,
-1.59151154759564,-1.55015084884505,-1.50844831044497,-1.50331178188857,
-1.50059537565022,-1.49857291477652,-1.49603605541585,-1.49173523329185,
-1.47617214165339,-1.42057980179783,-1.40439869897935,-1.40161658903259,
-1.40011994170544,-1.39886344698385,-1.39728922798726,-1.39423284770309,
-1.37359207520142,-1.32240919203572,-1.30709484263055,-1.30298844807667,
-1.30049427226178,-1.29823895994862,-1.29534240983719,-1.29067890181161,
-1.25678765109242,-1.2202430768001,-1.20510121321782,-1.20250176290395,
-1.20088882445463,-1.19962978186435,-1.19816288368014,-1.19551894024778,
-1.18223748360061,-1.15043463924379,-1.10948361271134,-1.10486482500918,
-1.10198167533799,-1.09972796941844,-1.09722653510611,-1.09308717663254,
-1.07738987906207,-1.04744044205406,-1.00837454542915,-1.00375780977525,
-1.00186871928028,-1.00057971673414,-0.99923944727864,-0.997169282320156,
-0.990868671238765,-0.980612478789826,-0.933876250565931,-0.926452780362809),
 .UNSPECIFIED.);
#452=B_SPLINE_CURVE_WITH_KNOTS('',3,(#28735,#28736,#28737,#28738,#28739,
#28740,#28741,#28742,#28743,#28744,#28745,#28746,#28747,#28748,#28749,#28750,
#28751,#28752,#28753,#28754,#28755,#28756,#28757,#28758,#28759,#28760,#28761,
#28762,#28763,#28764,#28765,#28766,#28767,#28768,#28769,#28770,#28771,#28772,
#28773,#28774,#28775,#28776,#28777,#28778,#28779,#28780,#28781,#28782,#28783,
#28784,#28785,#28786,#28787,#28788,#28789,#28790,#28791,#28792,#28793,#28794,
#28795,#28796,#28797,#28798,#28799,#28800,#28801,#28802,#28803,#28804,#28805,
#28806,#28807,#28808,#28809,#28810,#28811,#28812,#28813,#28814,#28815,#28816,
#28817,#28818),.UNSPECIFIED.,.F.,.F.,(4,2,2,2,2,2,2,2,2,2,2,2,2,2,2,2,2,
2,2,2,2,2,2,2,2,2,2,2,2,2,2,2,2,2,2,2,2,2,2,2,2,4),(-0.331223639443211,
-0.328400283237573,-0.318230345971041,-0.301571799019314,-0.297219577159239,
-0.294646191467861,-0.29240295333943,-0.289632073593904,-0.284232991031098,
-0.277370440987669,-0.261533147621455,-0.221660235473837,-0.19938299995667,
-0.196293789654357,-0.194712475032134,-0.193490616217635,-0.193482886691718,
-0.193475217914417,-0.193467608531236,-0.1934600574321,-0.193452563300397,
-0.193445124781644,-0.19343774067915,-0.193430409979487,-0.19342313169482,
-0.193415904542959,-0.193408727497731,-0.1919276918568,-0.190320685315479,
-0.187773706910874,-0.18280122812995,-0.169845147164471,-0.128787708133948,
-0.103050212938598,-0.0985848410198022,-0.0957478779548156,-0.0934990459870276,
-0.0909703220249327,-0.0867075750181842,-0.0694766656570718,-0.0373212317703668,
-0.000589895100449732),.UNSPECIFIED.);
#453=B_SPLINE_CURVE_WITH_KNOTS('',3,(#28819,#28820,#28821,#28822,#28823,
#28824,#28825,#28826,#28827,#28828,#28829,#28830,#28831,#28832,#28833,#28834,
#28835,#28836,#28837,#28838,#28839,#28840,#28841,#28842,#28843,#28844,#28845,
#28846,#28847,#28848,#28849,#28850,#28851,#28852,#28853,#28854,#28855,#28856,
#28857,#28858,#28859,#28860,#28861,#28862,#28863,#28864,#28865,#28866,#28867,
#28868,#28869,#28870,#28871,#28872,#28873,#28874,#28875,#28876,#28877,#28878,
#28879,#28880,#28881,#28882,#28883,#28884,#28885,#28886,#28887,#28888,#28889,
#28890,#28891,#28892,#28893,#28894,#28895,#28896,#28897,#28898,#28899,#28900,
#28901,#28902,#28903,#28904,#28905,#28906,#28907,#28908,#28909,#28910,#28911,
#28912,#28913,#28914,#28915,#28916,#28917,#28918,#28919,#28920,#28921,#28922,
#28923,#28924,#28925,#28926,#28927,#28928,#28929,#28930,#28931,#28932,#28933,
#28934,#28935,#28936,#28937,#28938,#28939,#28940,#28941,#28942,#28943,#28944,
#28945,#28946,#28947,#28948,#28949,#28950,#28951,#28952,#28953,#28954,#28955,
#28956,#28957,#28958,#28959,#28960,#28961,#28962,#28963,#28964,#28965,#28966,
#28967,#28968,#28969,#28970,#28971,#28972,#28973,#28974,#28975,#28976,#28977,
#28978,#28979,#28980,#28981,#28982,#28983,#28984,#28985,#28986),
 .UNSPECIFIED.,.F.,.F.,(4,2,2,2,2,2,2,2,2,2,2,2,2,2,2,2,2,2,2,2,2,2,2,2,
2,2,2,2,2,2,2,2,2,2,2,2,2,2,2,2,2,2,2,2,2,2,2,2,2,2,2,2,2,2,2,2,2,2,2,2,
2,2,2,2,2,2,2,2,2,2,2,2,2,2,2,2,2,2,2,2,2,2,2,4),(-2.51455855929107,-2.51267182880103,
-2.51070992938911,-2.50944404317543,-2.50824341760209,-2.50686998312504,
-2.5046508170838,-2.49776268037399,-2.48328141238618,-2.43134975919785,
-2.41592979517343,-2.41181344669691,-2.40931665937358,-2.40706120102442,
-2.40416755859932,-2.399515090484,-2.35967307239754,-2.33087137330689,-2.31934138430718,
-2.31474724717373,-2.31233861907934,-2.31078850070573,-2.30934995365382,
-2.30813825193173,-2.3065556437761,-2.30346104587939,-2.27105233106817,
-2.23432188999498,-2.21671480519106,-2.212423325102,-2.20988796821129,-2.20763964562131,
-2.20481190507332,-2.20037783686281,-2.17550534314661,-2.12929179002068,
-2.11907402644167,-2.11279029264204,-2.1107217758433,-2.10938159027269,
-2.1080918321381,-2.10620037573726,-2.10157158395456,-2.06272787620119,
-2.01882008688869,-2.01355659330931,-2.01081321545647,-2.0087873446844,
-2.00626769959418,-2.00204787052256,-1.9873360563847,-1.93617665552517,
-1.9166595416907,-1.91248251071885,-1.91071870976273,-1.90943955011861,
-1.9080530718869,-1.90577541100855,-1.89840660830998,-1.85698225723775,
-1.83578842024898,-1.81760633237194,-1.81327287723171,-1.81072815510037,
-1.80848093849328,-1.80566708304984,-1.80127907173016,-1.77762856658772,
-1.73981116668979,-1.71684754745087,-1.71284628666751,-1.71111281516262,
-1.70983852640525,-1.7084390022998,-1.70610267362239,-1.6982184297288,-1.63435668719908,
-1.61773550055021,-1.61351972240989,-1.61100110385319,-1.60875015954643,
-1.60589548422185,-1.60137228783183,-1.58839498599662),.UNSPECIFIED.);
#454=B_SPLINE_CURVE_WITH_KNOTS('',3,(#28992,#28993,#28994,#28995,#28996,
#28997,#28998,#28999,#29000,#29001,#29002,#29003,#29004,#29005,#29006,#29007,
#29008,#29009,#29010,#29011,#29012,#29013,#29014,#29015,#29016,#29017,#29018,
#29019,#29020,#29021,#29022,#29023,#29024,#29025,#29026,#29027,#29028,#29029,
#29030,#29031,#29032,#29033,#29034,#29035,#29036,#29037,#29038,#29039,#29040,
#29041,#29042,#29043,#29044,#29045,#29046,#29047,#29048,#29049,#29050,#29051,
#29052,#29053,#29054,#29055,#29056,#29057,#29058,#29059,#29060,#29061,#29062,
#29063,#29064,#29065,#29066,#29067,#29068,#29069,#29070,#29071,#29072,#29073,
#29074,#29075,#29076,#29077,#29078,#29079,#29080,#29081,#29082,#29083,#29084,
#29085,#29086,#29087,#29088,#29089,#29090,#29091,#29092,#29093,#29094,#29095,
#29096,#29097,#29098,#29099,#29100,#29101,#29102,#29103,#29104,#29105,#29106,
#29107,#29108,#29109,#29110,#29111,#29112,#29113,#29114,#29115,#29116,#29117,
#29118,#29119,#29120,#29121,#29122,#29123,#29124,#29125,#29126,#29127,#29128,
#29129,#29130,#29131,#29132,#29133,#29134,#29135,#29136,#29137,#29138,#29139,
#29140,#29141,#29142,#29143,#29144,#29145,#29146,#29147,#29148,#29149,#29150,
#29151,#29152,#29153,#29154,#29155),.UNSPECIFIED.,.F.,.F.,(4,2,2,2,2,2,
2,2,2,2,2,2,2,2,2,2,2,2,2,2,2,2,2,2,2,2,2,2,2,2,2,2,2,2,2,2,2,2,2,2,2,2,
2,2,2,2,2,2,2,2,2,2,2,2,2,2,2,2,2,2,2,2,2,2,2,2,2,2,2,2,2,2,2,2,2,2,2,2,
2,2,2,4),(-0.92677959358465,-0.913956461130793,-0.887738891672986,-0.88460392692942,
-0.883012622282303,-0.88175477462299,-0.880270911707597,-0.877549931281789,
-0.862766394361419,-0.819969429023721,-0.79148963880891,-0.786936396563254,
-0.784072428199227,-0.78182019700041,-0.779306410335309,-0.775113611790413,
-0.758784126405556,-0.698657199786042,-0.687281807858335,-0.684659282558548,
-0.683180723310601,-0.681922185656012,-0.680323380708066,-0.67704636708009,
-0.672724771099001,-0.62415063732743,-0.592032702904539,-0.587387979671654,
-0.584496297058608,-0.582240621835037,-0.579741807221744,-0.575617958157782,
-0.560118639868694,-0.507592837897413,-0.502745404443118,-0.488037317593654,
-0.485458757510819,-0.48385163229742,-0.482592422724597,-0.481119879474698,
-0.478452219407395,-0.464748199372748,-0.428746998202478,-0.392514894443486,
-0.387837323526096,-0.384935697135191,-0.38267868134251,-0.380184906170556,
-0.37608444400125,-0.360856403997985,-0.30994950409805,-0.288863758069141,
-0.285791990872181,-0.284213929083897,-0.282956548399099,-0.281461419176586,
-0.278688936006906,-0.262765672654064,-0.210164493371885,-0.191771762761121,
-0.187280697736259,-0.184674739580836,-0.182516231652231,-0.182476324449123,
-0.182438033032951,-0.182401247586332,-0.182365867957033,-0.18233180268593,
-0.182298968078676,-0.179559949958377,-0.176588839186943,-0.171819231333473,
-0.162389840194946,-0.115810719314727,-0.089364706251363,-0.0862274145327824,
-0.0846353913761449,-0.0833772170991153,-0.081893251484031,-0.0791728076642042,
-0.0644110085413288,-0.000590038431533063),.UNSPECIFIED.);
#455=B_SPLINE_CURVE_WITH_KNOTS('',3,(#29156,#29157,#29158,#29159,#29160,
#29161,#29162,#29163,#29164,#29165,#29166,#29167,#29168,#29169,#29170,#29171,
#29172,#29173,#29174,#29175,#29176,#29177,#29178,#29179,#29180,#29181,#29182,
#29183,#29184,#29185,#29186,#29187,#29188,#29189,#29190,#29191,#29192,#29193,
#29194,#29195,#29196,#29197,#29198,#29199,#29200,#29201,#29202,#29203,#29204,
#29205,#29206,#29207,#29208,#29209,#29210,#29211,#29212,#29213,#29214,#29215,
#29216,#29217,#29218,#29219,#29220,#29221,#29222,#29223,#29224,#29225),
 .UNSPECIFIED.,.F.,.F.,(4,2,2,2,2,2,2,2,2,2,2,2,2,2,2,2,2,2,2,2,2,2,2,2,
2,2,2,2,2,2,2,2,2,2,4),(-2.51322710726194,-2.50306881125958,-2.500318325518,
-2.49815032271898,-2.4959489582546,-2.49342563129446,-2.48918475967013,
-2.47519140971142,-2.41681275051123,-2.40166680893969,-2.3989300207045,
-2.39744323970873,-2.39618634741625,-2.39460061606263,-2.39148957656057,
-2.36733357237162,-2.32989726596998,-2.31379660224984,-2.30685603765565,
-2.30301464286754,-2.29965910347358,-2.29735087919383,-2.29505941343393,
-2.29230722082498,-2.28539985991157,-2.23532504570624,-2.21251159976598,
-2.20536789146102,-2.20054240368459,-2.1986744984044,-2.19737683100111,
-2.19618986191896,-2.19454439272652,-2.1903186976033,-2.18264003139251),
 .UNSPECIFIED.);
#456=B_SPLINE_CURVE_WITH_KNOTS('',3,(#29226,#29227,#29228,#29229,#29230,
#29231,#29232,#29233,#29234,#29235,#29236,#29237,#29238,#29239,#29240,#29241,
#29242,#29243,#29244,#29245,#29246,#29247,#29248,#29249,#29250,#29251,#29252,
#29253,#29254,#29255,#29256,#29257,#29258,#29259,#29260,#29261,#29262,#29263,
#29264,#29265,#29266,#29267,#29268,#29269,#29270,#29271,#29272,#29273,#29274,
#29275,#29276,#29277,#29278,#29279,#29280,#29281,#29282,#29283,#29284,#29285,
#29286,#29287,#29288,#29289,#29290,#29291,#29292,#29293,#29294,#29295,#29296,
#29297,#29298,#29299,#29300,#29301,#29302,#29303,#29304,#29305,#29306,#29307,
#29308,#29309,#29310,#29311,#29312,#29313,#29314,#29315,#29316,#29317,#29318,
#29319,#29320,#29321,#29322,#29323,#29324,#29325,#29326,#29327,#29328,#29329,
#29330,#29331,#29332,#29333,#29334,#29335,#29336,#29337,#29338,#29339,#29340,
#29341,#29342,#29343,#29344,#29345,#29346,#29347,#29348,#29349,#29350,#29351,
#29352,#29353,#29354,#29355,#29356,#29357,#29358,#29359,#29360,#29361,#29362,
#29363,#29364,#29365,#29366,#29367,#29368,#29369,#29370,#29371,#29372,#29373,
#29374,#29375,#29376,#29377,#29378,#29379,#29380,#29381,#29382,#29383,#29384,
#29385,#29386,#29387,#29388,#29389,#29390,#29391,#29392,#29393,#29394,#29395,
#29396,#29397,#29398,#29399,#29400,#29401,#29402,#29403,#29404,#29405,#29406,
#29407,#29408,#29409,#29410,#29411,#29412,#29413,#29414,#29415,#29416,#29417,
#29418,#29419,#29420,#29421,#29422,#29423,#29424,#29425,#29426,#29427,#29428,
#29429,#29430,#29431),.UNSPECIFIED.,.F.,.F.,(4,2,2,2,2,2,2,2,2,2,2,2,2,
2,2,2,2,2,2,2,2,2,2,2,2,2,2,2,2,2,2,2,2,2,2,2,2,2,2,2,2,2,2,2,2,2,2,2,2,
2,2,2,2,2,2,2,2,2,2,2,2,2,2,2,2,2,2,2,2,2,2,2,2,2,2,2,2,2,2,2,2,2,2,2,2,
2,2,2,2,2,2,2,2,2,2,2,2,2,2,2,2,2,4),(-1.58839498599662,-1.57389679594943,
-1.53012524666282,-1.51520503035608,-1.51247775967064,-1.51099264995324,
-1.50973506747913,-1.50814581829002,-1.50562556430176,-1.49206516637976,
-1.48508584688019,-1.43335240337203,-1.42318373105345,-1.41583489023955,
-1.41270008424995,-1.41040822700298,-1.40829630140824,-1.40542764008709,
-1.39827798178308,-1.35366871659575,-1.31743508525211,-1.3135487905047,
-1.31183575689162,-1.31056465268956,-1.30915580048413,-1.30677702832592,
-1.29849796658949,-1.25782231538263,-1.25419345451046,-1.22028973431126,
-1.21562517441884,-1.21272792532229,-1.21047206546839,-1.20797728645389,
-1.20386992457662,-1.18855331909787,-1.13738865577281,-1.11664590076547,
-1.11358558436978,-1.11201027469046,-1.11075341699938,-1.10925695855602,
-1.10647688108613,-1.0903574930049,-1.03553479667585,-1.01925934847971,
-1.01493416233628,-1.01236678209581,-1.01012261103052,-1.00734260511122,
-1.00189982430362,-0.964635404703312,-0.923660173673593,-0.915723316973921,
-0.913381301371229,-0.911980585637987,-0.910706838537789,-0.908976374686079,
-0.904991790424494,-0.88720698795585,-0.844130026595071,-0.820569568567948,
-0.816185610615111,-0.813373101539888,-0.811126170030985,-0.808580924010213,
-0.804244487974513,-0.786017809540127,-0.764732584541424,-0.723010575005474,
-0.715967458056545,-0.713728838222886,-0.712351086200415,-0.711068255573755,
-0.709282598561758,-0.704975328454701,-0.68423109950062,-0.624017932979638,
-0.617203246173567,-0.614465329367151,-0.612176940933543,-0.609815841503152,
-0.606324959288843,-0.596640907909793,-0.581981948412719,-0.551236680492311,
-0.520479501240534,-0.515690744058459,-0.513772684182183,-0.512594840768582,
-0.511287165012195,-0.5093706262964,-0.504221547627114,-0.474249737280712,
-0.424678480154916,-0.417717637722567,-0.414956446843606,-0.412662192114699,
-0.410308947906355,-0.406855666865491,-0.397442401063055,-0.3833359825281,
-0.331428972207689),.UNSPECIFIED.);
#457=B_SPLINE_CURVE_WITH_KNOTS('',3,(#29436,#29437,#29438,#29439,#29440,
#29441,#29442,#29443,#29444,#29445,#29446,#29447,#29448,#29449,#29450,#29451,
#29452,#29453,#29454,#29455,#29456,#29457,#29458,#29459,#29460,#29461,#29462,
#29463,#29464,#29465,#29466,#29467,#29468,#29469,#29470,#29471,#29472,#29473,
#29474,#29475,#29476,#29477,#29478,#29479,#29480,#29481,#29482,#29483,#29484,
#29485,#29486,#29487,#29488,#29489,#29490,#29491,#29492,#29493,#29494,#29495,
#29496,#29497,#29498,#29499,#29500,#29501,#29502,#29503,#29504,#29505,#29506,
#29507,#29508,#29509,#29510,#29511,#29512,#29513,#29514,#29515,#29516,#29517,
#29518,#29519,#29520,#29521,#29522,#29523,#29524,#29525,#29526,#29527,#29528,
#29529,#29530,#29531,#29532,#29533,#29534,#29535,#29536,#29537,#29538,#29539,
#29540,#29541,#29542,#29543,#29544,#29545,#29546,#29547,#29548,#29549,#29550,
#29551,#29552,#29553,#29554,#29555,#29556,#29557,#29558,#29559,#29560,#29561,
#29562,#29563,#29564,#29565,#29566,#29567,#29568,#29569,#29570,#29571,#29572,
#29573,#29574,#29575,#29576,#29577,#29578,#29579,#29580,#29581,#29582,#29583,
#29584,#29585,#29586,#29587,#29588,#29589,#29590,#29591,#29592,#29593,#29594,
#29595,#29596,#29597,#29598,#29599,#29600,#29601,#29602,#29603,#29604,#29605,
#29606,#29607,#29608,#29609,#29610,#29611,#29612,#29613,#29614,#29615,#29616,
#29617,#29618,#29619,#29620,#29621,#29622,#29623,#29624,#29625,#29626,#29627,
#29628,#29629,#29630,#29631,#29632,#29633,#29634,#29635,#29636,#29637,#29638,
#29639,#29640,#29641,#29642,#29643,#29644,#29645,#29646,#29647,#29648,#29649,
#29650,#29651),.UNSPECIFIED.,.F.,.F.,(4,2,2,2,2,2,2,2,2,2,2,2,2,2,2,2,2,
2,2,2,2,2,2,2,2,2,2,2,2,2,2,2,2,2,2,2,2,2,2,2,2,2,2,2,2,2,2,2,2,2,2,2,2,
2,2,2,2,2,2,2,2,2,2,2,2,2,2,2,2,2,2,2,2,2,2,2,2,2,2,2,2,2,2,2,2,2,2,2,2,
2,2,2,2,2,2,2,2,2,2,2,2,2,2,2,2,2,2,4),(-2.18327158177654,-2.18237473463362,
-2.1798643145631,-2.17761231538485,-2.17474482746901,-2.1701782813769,-2.14119715670792,
-2.09884498927307,-2.08412528277437,-2.08140785580374,-2.07992502811304,
-2.07866750515955,-2.07707591611306,-2.07393831137517,-2.04707624538335,
-2.01093049290248,-1.99572431302921,-1.98905151351183,-1.9837710798474,
-1.9810245526589,-1.97899869223382,-1.97648204385171,-1.97227433396359,
-1.957673757243,-1.94954653254484,-1.89650001839176,-1.88842577944554,-1.88313696289202,
-1.88120032976807,-1.87988853525725,-1.87871423424549,-1.87681543313071,
-1.87214168097356,-1.83434134530135,-1.78938220949677,-1.78418661432689,
-1.78145753919213,-1.77921661409665,-1.77661040136295,-1.7721153282108,
-1.75357539473028,-1.70111512496838,-1.68520588740849,-1.68243472274365,
-1.68094022540139,-1.67968332464732,-1.67810580755332,-1.6750349335161,
-1.65394829732468,-1.60305970955705,-1.58787946106536,-1.58378424760483,
-1.58129220698214,-1.57903581742817,-1.57613367572018,-1.57145251493047,
-1.53446495148284,-1.49946601313129,-1.48553350804964,-1.48285462501969,
-1.48137997219493,-1.4801214786333,-1.47851851655293,-1.47595282504375,
-1.46149580455587,-1.45617430555503,-1.40387978146931,-1.388414579538,-1.38429462681168,
-1.38179719136077,-1.37954212907725,-1.37665035336343,-1.37200364225382,
-1.33262458000192,-1.2995395597515,-1.28598744316519,-1.28332849442826,
-1.28185818415954,-1.2805992736605,-1.27899046539558,-1.27640527788,-1.26154228164339,
-1.2576224943358,-1.2187346028497,-1.19060414772441,-1.18606172708297,-1.18320127153122,
-1.18094974656275,-1.17843461100669,-1.1742344872179,-1.15780836471621,
-1.0965292632248,-1.08627150875081,-1.08373530750034,-1.08227662295387,
-1.08102796737465,-1.07940830558278,-1.07602408042783,-1.04721034938435,
-0.996823319807449,-0.9879960720525,-0.984523368248433,-0.982401526806259,
-0.980116372271241,-0.977021824067564,-0.969908843914664,-0.960159636101433,
-0.92677959358465),.UNSPECIFIED.);
#458=B_SPLINE_CURVE_WITH_KNOTS('',3,(#29653,#29654,#29655,#29656,#29657,
#29658,#29659,#29660,#29661,#29662,#29663,#29664,#29665,#29666,#29667,#29668,
#29669,#29670,#29671,#29672,#29673,#29674,#29675,#29676,#29677,#29678,#29679,
#29680,#29681,#29682,#29683,#29684,#29685,#29686,#29687,#29688,#29689,#29690,
#29691,#29692,#29693,#29694,#29695,#29696,#29697,#29698,#29699,#29700,#29701,
#29702,#29703,#29704,#29705,#29706,#29707,#29708,#29709,#29710,#29711,#29712,
#29713,#29714,#29715,#29716,#29717,#29718,#29719,#29720),.UNSPECIFIED.,
 .F.,.F.,(4,2,2,2,2,2,2,2,2,2,2,2,2,2,2,2,2,2,2,2,2,2,2,2,2,2,2,2,2,2,2,
2,2,4),(-0.331428972207689,-0.329069592277333,-0.31754448082226,-0.314911286889619,
-0.313430515309816,-0.312172530874924,-0.310577569749016,-0.307318810788601,
-0.272108301779798,-0.225394121966846,-0.218355992557429,-0.215506219692164,
-0.213398962200356,-0.21114907560631,-0.208088514010398,-0.20466469999614,
-0.198783566725625,-0.160678346912252,-0.12099775587246,-0.116413804600362,
-0.114529870692238,-0.113241624547243,-0.111899440938968,-0.10982164988372,
-0.103461667375636,-0.0930722481795077,-0.0320180274467594,-0.0203029537165471,
-0.0164251417768983,-0.0139809767253367,-0.011820034564099,-0.00961711351532164,
-0.00560281701044909,-0.000589238754991204),.UNSPECIFIED.);
#459=B_SPLINE_CURVE_WITH_KNOTS('',3,(#29721,#29722,#29723,#29724,#29725,
#29726,#29727,#29728,#29729,#29730,#29731,#29732,#29733,#29734,#29735,#29736,
#29737,#29738,#29739,#29740,#29741,#29742,#29743,#29744,#29745,#29746,#29747,
#29748,#29749,#29750,#29751,#29752,#29753,#29754,#29755,#29756,#29757,#29758,
#29759,#29760,#29761,#29762,#29763,#29764,#29765,#29766,#29767,#29768,#29769,
#29770,#29771,#29772,#29773,#29774,#29775,#29776,#29777,#29778,#29779,#29780,
#29781,#29782,#29783,#29784,#29785,#29786,#29787,#29788,#29789,#29790,#29791,
#29792,#29793,#29794,#29795,#29796,#29797,#29798,#29799,#29800,#29801,#29802,
#29803,#29804,#29805,#29806,#29807,#29808,#29809,#29810,#29811,#29812,#29813,
#29814,#29815,#29816,#29817,#29818,#29819,#29820,#29821,#29822,#29823,#29824,
#29825,#29826,#29827,#29828,#29829,#29830,#29831,#29832,#29833,#29834,#29835,
#29836,#29837,#29838,#29839,#29840,#29841,#29842,#29843,#29844,#29845,#29846,
#29847,#29848,#29849,#29850,#29851,#29852,#29853,#29854,#29855,#29856,#29857,
#29858,#29859,#29860,#29861,#29862,#29863,#29864,#29865,#29866,#29867,#29868,
#29869,#29870,#29871,#29872,#29873,#29874,#29875,#29876,#29877,#29878,#29879,
#29880,#29881,#29882,#29883,#29884,#29885,#29886,#29887,#29888,#29889,#29890,
#29891,#29892,#29893,#29894,#29895,#29896,#29897,#29898,#29899,#29900,#29901,
#29902,#29903,#29904,#29905,#29906,#29907,#29908,#29909,#29910),
 .UNSPECIFIED.,.F.,.F.,(4,2,2,2,2,2,2,2,2,2,2,2,2,2,2,2,2,2,2,2,2,2,2,2,
2,2,2,2,2,2,2,2,2,2,2,2,2,2,2,2,2,2,2,2,2,2,2,2,2,2,2,2,2,2,2,2,2,2,2,2,
2,2,2,2,2,2,2,2,2,2,2,2,2,2,2,2,2,2,2,2,2,2,2,2,2,2,2,2,2,2,2,2,2,2,4),
(-2.51385800421912,-2.44636517931643,-2.431612280618,-2.42889332475062,
-2.42741020504889,-2.42615277103915,-2.42456175169058,-2.42142665686335,
-2.39504305790227,-2.34861391700199,-2.33910351988365,-2.33430548895331,
-2.33132315755465,-2.32857636760943,-2.32854220446278,-2.32850690336214,
-2.32847038404083,-2.32843255880197,-2.32839333146543,-2.32835259642427,
-2.32831023743384,-2.3282661261745,-2.32822012052279,-2.32817206277085,
-2.32812177731026,-2.32809325676061,-2.32805762578005,-2.32801285630427,
-2.32795619200621,-2.32788379186356,-2.32779013116768,-2.32559208321247,
-2.32272021037873,-2.3181389885118,-2.28886693672711,-2.24676880078385,
-2.23208397823921,-2.22936822641916,-2.22788578304132,-2.22662827238712,
-2.22503632728358,-2.22189693076285,-2.19439071927247,-2.15792878071183,
-2.14329755799621,-2.1368005931387,-2.13163115886668,-2.12890766716624,
-2.12666718396756,-2.12405678205579,-2.1195427478348,-2.10072813596257,
-2.09399861600692,-2.05216146011603,-2.03454642543843,-2.03058191621004,
-2.02885519540958,-2.0275822319552,-2.02635660388504,-2.02419252284182,
-2.01773514987145,-1.95224143081994,-1.94120671222611,-1.9333823437529,
-1.93016920728132,-1.92786370886945,-1.92576895023238,-1.92244140505524,
-1.91625461428461,-1.86576513105235,-1.83362518615939,-1.83050911421993,
-1.82894304034653,-1.82780852984964,-1.82635534807342,-1.8238416015201,
-1.81384137755083,-1.75232256766172,-1.73588031383969,-1.73167986356789,
-1.72916519412771,-1.72691450722465,-1.7240556984035,-1.71951703761676,
-1.69148772476889,-1.64825210442742,-1.63340831816123,-1.63068535834978,
-1.62920150167953,-1.627944318572,-1.62635473168511,-1.62383237486457,-1.61021973740491,
-1.60334132476312,-1.58784363167967),.UNSPECIFIED.);
#460=B_SPLINE_CURVE_WITH_KNOTS('',3,(#29916,#29917,#29918,#29919,#29920,
#29921,#29922,#29923,#29924,#29925,#29926,#29927,#29928,#29929,#29930,#29931,
#29932,#29933,#29934,#29935,#29936,#29937,#29938,#29939,#29940,#29941,#29942,
#29943,#29944,#29945,#29946,#29947,#29948,#29949,#29950,#29951,#29952,#29953,
#29954,#29955,#29956,#29957,#29958,#29959,#29960,#29961,#29962,#29963,#29964,
#29965,#29966,#29967,#29968,#29969,#29970,#29971,#29972,#29973,#29974,#29975,
#29976,#29977,#29978,#29979,#29980,#29981,#29982,#29983,#29984,#29985,#29986,
#29987,#29988,#29989,#29990,#29991,#29992,#29993,#29994,#29995,#29996,#29997,
#29998,#29999,#30000,#30001,#30002,#30003,#30004,#30005,#30006,#30007,#30008,
#30009,#30010,#30011,#30012,#30013,#30014,#30015,#30016,#30017,#30018,#30019,
#30020,#30021,#30022,#30023,#30024,#30025,#30026,#30027,#30028,#30029,#30030,
#30031,#30032,#30033,#30034,#30035,#30036,#30037,#30038,#30039,#30040,#30041,
#30042,#30043,#30044,#30045,#30046,#30047,#30048,#30049,#30050,#30051,#30052,
#30053,#30054,#30055,#30056,#30057,#30058,#30059,#30060,#30061,#30062,#30063,
#30064,#30065,#30066,#30067,#30068,#30069,#30070,#30071,#30072,#30073),
 .UNSPECIFIED.,.F.,.F.,(4,2,2,2,2,2,2,2,2,2,2,2,2,2,2,2,2,2,2,2,2,2,2,2,
2,2,2,2,2,2,2,2,2,2,2,2,2,2,2,2,2,2,2,2,2,2,2,2,2,2,2,2,2,2,2,2,2,2,2,2,
2,2,2,2,2,2,2,2,2,2,2,2,2,2,2,2,2,2,4),(-0.926655402496498,-0.923325713363623,
-0.875292521762498,-0.868346533299104,-0.865512679640234,-0.863409460980203,
-0.861110593662156,-0.857936137348705,-0.850350669588792,-0.839753052092,
-0.80865427827618,-0.771245861527511,-0.766547068349882,-0.764644066482668,
-0.763468989606336,-0.76215809480017,-0.760225876991041,-0.754968056358794,
-0.74695836949584,-0.694972907930171,-0.684978571269381,-0.670996910459284,
-0.666853556032092,-0.664350981166793,-0.662097059452066,-0.659214757552757,
-0.653256188746563,-0.612550460754442,-0.571486359006606,-0.56695796555454,
-0.565269281098544,-0.564070607723434,-0.562781806314694,-0.560962224650154,
-0.556446943285244,-0.533636464436129,-0.510487308828706,-0.473380312573813,
-0.468700165707988,-0.465798253733345,-0.463541815998277,-0.461049491659218,
-0.456953285347575,-0.441763515642257,-0.390850431239601,-0.36975580306435,
-0.366684518508422,-0.365106856799941,-0.363849876085606,-0.362355318467321,
-0.359584148064584,-0.343675898136389,-0.291197077674096,-0.272699618055052,
-0.268207304685064,-0.265601569733216,-0.263360387709269,-0.260630165087058,
-0.255429819582491,-0.248883755018148,-0.23409264982936,-0.182540404821751,
-0.169618780281208,-0.167133463660783,-0.165554781913349,-0.16429772163908,
-0.163102679175141,-0.160860067986025,-0.152482104862663,-0.13694380760027,
-0.115306868483614,-0.0741973780390122,-0.0695757179166427,-0.0666911871463561,
-0.0644366553561687,-0.0619345645218826,-0.0577947266259297,-0.0528738525793985,
-0.000589974190451465),.UNSPECIFIED.);
#461=B_SPLINE_CURVE_WITH_KNOTS('',3,(#30074,#30075,#30076,#30077,#30078,
#30079,#30080,#30081,#30082,#30083,#30084,#30085,#30086,#30087,#30088,#30089,
#30090,#30091,#30092,#30093,#30094,#30095,#30096,#30097,#30098,#30099,#30100,
#30101,#30102,#30103,#30104,#30105,#30106,#30107,#30108,#30109,#30110,#30111,
#30112,#30113,#30114,#30115,#30116,#30117,#30118,#30119,#30120,#30121,#30122,
#30123,#30124,#30125,#30126,#30127,#30128,#30129,#30130,#30131,#30132,#30133,
#30134,#30135,#30136,#30137,#30138,#30139,#30140,#30141,#30142,#30143,#30144,
#30145,#30146,#30147,#30148,#30149,#30150,#30151,#30152,#30153,#30154,#30155,
#30156,#30157,#30158,#30159,#30160,#30161,#30162,#30163,#30164,#30165,#30166,
#30167,#30168,#30169,#30170,#30171,#30172,#30173,#30174,#30175,#30176,#30177,
#30178,#30179,#30180,#30181,#30182,#30183,#30184,#30185,#30186,#30187),
 .UNSPECIFIED.,.F.,.F.,(4,2,2,2,2,2,2,2,2,2,2,2,2,2,2,2,2,2,2,2,2,2,2,2,
2,2,2,2,2,2,2,2,2,2,2,2,2,2,2,2,2,2,2,2,2,2,2,2,2,2,2,2,2,2,2,2,4),(-2.5136943146703,
-2.48380750396871,-2.48159185501007,-2.48012132498352,-2.47892808420488,
-2.47767089825701,-2.47608450433997,-2.47297130089924,-2.44869524354049,
-2.43335605149126,-2.39114991208164,-2.38382693609609,-2.38069679813858,
-2.37840599846826,-2.37629339513071,-2.37342127026519,-2.36624967973667,
-2.32226479000931,-2.28769438669882,-2.28397482608036,-2.28110157668122,
-2.27958653808802,-2.27958267230492,-2.27957879377167,-2.27957490225234,
-2.27957099774637,-2.27956708041037,-2.27956315007698,-2.27955920645746,
-2.27955524962164,-2.2795512794122,-2.27954729589535,-2.2795432988887,-2.27953928829381,
-2.27953526406274,-2.2795312261854,-2.27952717450785,-2.2795231090035,-2.27951902952133,
-2.27951493603563,-2.27951082802332,-2.2795067058843,-2.27950256948525,
-2.27949841863929,-2.27949425329322,-2.27949007323984,-2.27948587865382,
-2.27948160529282,-2.27947726300606,-2.27947285048055,-2.27821609677091,
-2.27663886446651,-2.27415779496651,-2.261334242407,-2.2027368319213,-2.18655457165281,
-2.18327158177654),.UNSPECIFIED.);
#462=B_SPLINE_CURVE_WITH_KNOTS('',3,(#30188,#30189,#30190,#30191,#30192,
#30193,#30194,#30195,#30196,#30197,#30198,#30199,#30200,#30201,#30202,#30203,
#30204,#30205,#30206,#30207,#30208,#30209,#30210,#30211,#30212,#30213,#30214,
#30215,#30216,#30217,#30218,#30219,#30220,#30221,#30222,#30223,#30224,#30225,
#30226,#30227,#30228,#30229,#30230,#30231,#30232,#30233,#30234,#30235,#30236,
#30237,#30238,#30239,#30240,#30241,#30242,#30243,#30244,#30245,#30246,#30247,
#30248,#30249,#30250,#30251,#30252,#30253,#30254,#30255,#30256,#30257,#30258,
#30259,#30260,#30261,#30262,#30263,#30264,#30265,#30266,#30267,#30268,#30269,
#30270,#30271,#30272,#30273,#30274,#30275,#30276,#30277,#30278,#30279,#30280,
#30281,#30282,#30283,#30284,#30285,#30286,#30287,#30288,#30289,#30290,#30291,
#30292,#30293,#30294,#30295,#30296,#30297,#30298,#30299,#30300,#30301,#30302,
#30303,#30304,#30305,#30306,#30307,#30308,#30309,#30310,#30311,#30312,#30313,
#30314,#30315,#30316,#30317,#30318,#30319,#30320,#30321,#30322,#30323,#30324,
#30325,#30326,#30327,#30328,#30329,#30330,#30331,#30332,#30333,#30334,#30335,
#30336,#30337,#30338,#30339,#30340,#30341,#30342,#30343,#30344,#30345,#30346,
#30347,#30348,#30349,#30350,#30351,#30352,#30353,#30354,#30355,#30356,#30357,
#30358,#30359,#30360,#30361,#30362,#30363,#30364,#30365,#30366,#30367,#30368,
#30369,#30370,#30371,#30372,#30373,#30374,#30375,#30376,#30377,#30378,#30379,
#30380,#30381,#30382,#30383,#30384,#30385,#30386,#30387,#30388,#30389,#30390,
#30391,#30392,#30393,#30394,#30395),.UNSPECIFIED.,.F.,.F.,(4,2,2,2,2,2,
2,2,2,2,2,2,2,2,2,2,2,2,2,2,2,2,2,2,2,2,2,2,2,2,2,2,2,2,2,2,2,2,2,2,2,2,
2,2,2,2,2,2,2,2,2,2,2,2,2,2,2,2,2,2,2,2,2,2,2,2,2,2,2,2,2,2,2,2,2,2,2,2,
2,2,2,2,2,2,2,2,2,2,2,2,2,2,2,2,2,2,2,2,2,2,2,2,2,4),(-1.58784363167967,
-1.55653980649131,-1.53682627591046,-1.53239112152884,-1.52982491184867,
-1.52758152976368,-1.52480219787095,-1.5205246686636,-1.4991362545965,-1.4495755190104,
-1.43395890214868,-1.43120089727338,-1.42970948290601,-1.42845279554363,
-1.4268725656368,-1.42378773388125,-1.40213419884548,-1.36619124270863,
-1.34057587306419,-1.33416475951176,-1.33119691501943,-1.32893222794554,
-1.32647324435256,-1.32252648248045,-1.31029044259186,-1.25706652143903,
-1.25621897288139,-1.2350281280096,-1.23195418944306,-1.2303761830444,-1.22911947666921,
-1.22762592046895,-1.22485840672266,-1.2090251233432,-1.15732730437855,
-1.13806118812672,-1.1335162372456,-1.13089886856031,-1.12868029723667,
-1.12597482324312,-1.12089126147169,-1.08347584283976,-1.04337702507936,
-1.03435336219944,-1.0318995445329,-1.03047424955446,-1.02920787039768,
-1.02752769853864,-1.02382166632852,-0.992139621717132,-0.942218023775984,
-0.935292937536694,-0.932537678671096,-0.930245188132086,-0.927890516315309,
-0.924429104431877,-0.914955356384526,-0.900725485187351,-0.84475086213516,
-0.834904872657207,-0.832404181503658,-0.830953864441757,-0.829818732357317,
-0.828248138572338,-0.825110504955073,-0.821021047967029,-0.77728167038638,
-0.739952702858024,-0.735273637980358,-0.73237221966898,-0.730116066076078,
-0.727623960439035,-0.723527910733295,-0.708336824255992,-0.657429690776177,
-0.636313026745115,-0.633241211270951,-0.631663541276157,-0.630406700922518,
-0.628912510370345,-0.626142571117113,-0.610258665634811,-0.558049427505137,
-0.539273879825064,-0.534762426406683,-0.532152499129624,-0.529911820416523,
-0.527187340481007,-0.52201373775495,-0.47680791018961,-0.439162346565744,
-0.434478173968208,-0.432577618931206,-0.431402995563107,-0.430091594735694,
-0.428156892725011,-0.422881651416646,-0.41483641160278,-0.362276266293727,
-0.354099082601777,-0.339103189566385,-0.334854231083463,-0.332328427301319,
-0.331109356375104),.UNSPECIFIED.);
#463=B_SPLINE_CURVE_WITH_KNOTS('',3,(#30400,#30401,#30402,#30403,#30404,
#30405,#30406,#30407,#30408,#30409,#30410,#30411,#30412,#30413,#30414,#30415,
#30416,#30417,#30418,#30419,#30420,#30421,#30422,#30423,#30424,#30425,#30426,
#30427,#30428,#30429,#30430,#30431,#30432,#30433,#30434,#30435,#30436,#30437,
#30438,#30439,#30440,#30441,#30442,#30443,#30444,#30445,#30446,#30447,#30448,
#30449,#30450,#30451,#30452,#30453,#30454,#30455,#30456,#30457,#30458,#30459,
#30460,#30461,#30462,#30463,#30464,#30465,#30466,#30467,#30468,#30469,#30470,
#30471,#30472,#30473,#30474,#30475,#30476,#30477,#30478,#30479,#30480,#30481,
#30482,#30483,#30484,#30485,#30486,#30487,#30488,#30489,#30490,#30491,#30492,
#30493,#30494,#30495,#30496,#30497,#30498,#30499,#30500,#30501,#30502,#30503,
#30504,#30505,#30506,#30507,#30508,#30509,#30510,#30511,#30512,#30513,#30514,
#30515,#30516,#30517,#30518,#30519,#30520,#30521,#30522,#30523,#30524,#30525,
#30526,#30527,#30528,#30529,#30530,#30531,#30532,#30533,#30534,#30535,#30536,
#30537,#30538,#30539,#30540,#30541,#30542,#30543,#30544,#30545,#30546,#30547,
#30548,#30549,#30550,#30551,#30552,#30553,#30554,#30555,#30556,#30557,#30558,
#30559,#30560,#30561,#30562,#30563,#30564,#30565,#30566,#30567,#30568,#30569,
#30570,#30571,#30572,#30573,#30574,#30575,#30576,#30577,#30578,#30579,#30580,
#30581,#30582,#30583,#30584,#30585,#30586,#30587,#30588,#30589,#30590,#30591,
#30592,#30593,#30594,#30595,#30596,#30597,#30598,#30599,#30600,#30601,#30602,
#30603,#30604,#30605,#30606,#30607,#30608,#30609,#30610,#30611,#30612,#30613,
#30614,#30615,#30616,#30617,#30618,#30619,#30620,#30621),.UNSPECIFIED.,
 .F.,.F.,(4,2,2,2,2,2,2,2,2,2,2,2,2,2,2,2,2,2,2,2,2,2,2,2,2,2,2,2,2,2,2,
2,2,2,2,2,2,2,2,2,2,2,2,2,2,2,2,2,2,2,2,2,2,2,2,2,2,2,2,2,2,2,2,2,2,2,2,
2,2,2,2,2,2,2,2,2,2,2,2,2,2,2,2,2,2,2,2,2,2,2,2,2,2,2,2,2,2,2,2,2,2,2,2,
2,2,2,2,2,2,2,4),(-2.18313823310106,-2.17650014074798,-2.16849956335008,
-2.16324663360991,-2.16131510569996,-2.16000435347047,-2.1588291534518,
-2.15692548973529,-2.15222274298792,-2.11487023056838,-2.08376576596208,
-2.0731669056622,-2.06558003609966,-2.06240529074588,-2.06010631427114,
-2.05800305845717,-2.05516924953659,-2.04822388216365,-2.00013839462087,
-1.96898236395335,-1.96374033751326,-1.96181030409453,-1.96049980788447,
-1.95932426178314,-1.957418964536,-1.9527068278182,-1.91570222526175,-1.87000896481567,
-1.86480345652993,-1.86207220397753,-1.85983102407378,-1.85722625106635,
-1.85273798025903,-1.83429862184862,-1.78172974525158,-1.76580949915184,
-1.76303771422548,-1.76154301824036,-1.7602860308786,-1.75870850659651,
-1.75563791355718,-1.73456528107433,-1.68369541475719,-1.66848094942072,
-1.66438252302699,-1.66188965770112,-1.65963325176594,-1.6567321110341,
-1.65205466644138,-1.61615542557009,-1.58024314816059,-1.56613753979821,
-1.5634497122733,-1.56197306179936,-1.56071466483217,-1.55911413597651,
-1.55655670877066,-1.54227070067467,-1.49018592542974,-1.46967833143249,
-1.46519267704807,-1.46261485308224,-1.46037166749937,-1.45760587903819,
-1.45337417161085,-1.43267580750312,-1.38240894350438,-1.37187447011469,
-1.36755647697839,-1.36428196163704,-1.36268385445326,-1.36142561557265,
-1.35994710565132,-1.35732397881196,-1.34593489590491,-1.29158172521746,
-1.27747394335548,-1.26805908156956,-1.26460544793684,-1.26225200778468,
-1.25995758854654,-1.25719621503331,-1.25023503729521,-1.22014279652187,
-1.18744383121592,-1.18147278862045,-1.16731804592522,-1.16476720102792,
-1.16316872289635,-1.16191055240079,-1.16043254288782,-1.15773815192072,
-1.14349749066547,-1.1230353616999,-1.07476600581412,-1.06783840326462,
-1.06500769531284,-1.06290523220257,-1.06060564806382,-1.05742736527376,
-1.04981897316048,-1.03917966466301,-1.00786834948704,-0.970762749794328,
-0.966051433093671,-0.964146324132916,-0.962970851662352,-0.961660393374075,
-0.959730346751497,-0.954487792326,-0.926655402496498),.UNSPECIFIED.);
#464=B_SPLINE_CURVE_WITH_KNOTS('',3,(#30623,#30624,#30625,#30626,#30627,
#30628,#30629,#30630,#30631,#30632,#30633,#30634,#30635,#30636,#30637,#30638,
#30639,#30640,#30641,#30642,#30643,#30644,#30645,#30646,#30647,#30648,#30649,
#30650,#30651,#30652,#30653,#30654,#30655,#30656,#30657,#30658,#30659,#30660,
#30661,#30662,#30663,#30664,#30665,#30666,#30667,#30668,#30669,#30670,#30671,
#30672,#30673,#30674,#30675,#30676,#30677,#30678,#30679,#30680,#30681,#30682,
#30683,#30684,#30685,#30686,#30687,#30688),.UNSPECIFIED.,.F.,.F.,(4,2,2,
2,2,2,2,2,2,2,2,2,2,2,2,2,2,2,2,2,2,2,2,2,2,2,2,2,2,2,2,2,4),(-0.331109356375104,
-0.330303897401218,-0.327570551246305,-0.322354305808374,-0.278470603079092,
-0.23948808912336,-0.23486645263933,-0.232976334313686,-0.231686962383251,
-0.230512412367563,-0.228725244679188,-0.224022011686405,-0.217062588272462,
-0.195224533200124,-0.14360464029413,-0.136858870570049,-0.133862335986385,
-0.131584959885326,-0.129159100344137,-0.125364891990015,-0.113222369558161,
-0.0848579885321056,-0.0607828913531212,-0.0560868797785358,-0.0521097054833987,
-0.037208406203165,-0.0346213853586508,-0.0330120986818491,-0.0317532478928443,
-0.0305638137843062,-0.0291095057448026,-0.026933433543985,-0.000589134625819604),
 .UNSPECIFIED.);
#465=B_SPLINE_CURVE_WITH_KNOTS('',3,(#30689,#30690,#30691,#30692,#30693,
#30694,#30695,#30696,#30697,#30698,#30699,#30700,#30701,#30702,#30703,#30704,
#30705,#30706,#30707,#30708,#30709,#30710,#30711,#30712,#30713,#30714,#30715,
#30716,#30717,#30718,#30719,#30720,#30721,#30722,#30723,#30724,#30725,#30726,
#30727,#30728,#30729,#30730,#30731,#30732,#30733,#30734,#30735,#30736,#30737,
#30738,#30739,#30740,#30741,#30742,#30743,#30744,#30745,#30746,#30747,#30748,
#30749,#30750,#30751,#30752,#30753,#30754,#30755,#30756,#30757,#30758,#30759,
#30760,#30761,#30762,#30763,#30764,#30765,#30766,#30767,#30768,#30769,#30770,
#30771,#30772,#30773,#30774,#30775,#30776,#30777,#30778,#30779,#30780,#30781,
#30782,#30783,#30784,#30785,#30786,#30787,#30788,#30789,#30790,#30791,#30792,
#30793,#30794,#30795,#30796,#30797,#30798,#30799,#30800,#30801,#30802,#30803,
#30804,#30805,#30806,#30807,#30808,#30809,#30810,#30811,#30812,#30813,#30814,
#30815,#30816,#30817,#30818,#30819,#30820,#30821,#30822,#30823,#30824,#30825,
#30826,#30827,#30828,#30829,#30830,#30831,#30832,#30833,#30834,#30835,#30836,
#30837,#30838,#30839,#30840,#30841,#30842),.UNSPECIFIED.,.F.,.F.,(4,2,2,
2,2,2,2,2,2,2,2,2,2,2,2,2,2,2,2,2,2,2,2,2,2,2,2,2,2,2,2,2,2,2,2,2,2,2,2,
2,2,2,2,2,2,2,2,2,2,2,2,2,2,2,2,2,2,2,2,2,2,2,2,2,2,2,2,2,2,2,2,2,2,2,2,
2,4),(-2.51375681360086,-2.45794213146706,-2.45071965764826,-2.44760757250335,
-2.44532072587026,-2.44320525687753,-2.44031919318414,-2.43305996673879,
-2.39470503687006,-2.37296163661332,-2.35801217863793,-2.34984917919882,
-2.34760362946983,-2.34641337301195,-2.34515585191424,-2.34355624402572,
-2.34099993793383,-2.32671139850862,-2.32106395787574,-2.27386825927659,
-2.25409208787252,-2.24965391941919,-2.24708754296824,-2.24484495058458,
-2.24206780788502,-2.23779593935463,-2.21649416166766,-2.16305184237234,
-2.15495619772662,-2.14965759124721,-2.14772017971664,-2.14640869992296,
-2.14523533076961,-2.14333926789419,-2.13867843596651,-2.10024950972278,
-2.05591925371147,-2.05072604681632,-2.04799832590834,-2.04597526168391,
-2.04344780178337,-2.03918762058278,-2.02404691056754,-2.01609730897087,
-1.96348548779911,-1.95543802649353,-1.95016278811696,-1.94822863453562,
-1.9469177773227,-1.94574376699351,-1.94384444309316,-1.939164485079,-1.90154490452413,
-1.856382454607,-1.85121484610332,-1.84849235200069,-1.84625270765591,-1.84364330378483,
-1.83913104721527,-1.82032471937217,-1.76814426432835,-1.75226448396576,
-1.74949550249777,-1.74800189206388,-1.74674557266302,-1.74516860558605,
-1.74209830147497,-1.72099784261568,-1.67013420248603,-1.65495626934021,
-1.65086249948869,-1.64837151860129,-1.64611621211735,-1.64321564406959,
-1.63853741526135,-1.60240793685852,-1.58789531626404),.UNSPECIFIED.);
#466=B_SPLINE_CURVE_WITH_KNOTS('',3,(#30848,#30849,#30850,#30851,#30852,
#30853,#30854,#30855,#30856,#30857,#30858,#30859,#30860,#30861,#30862,#30863,
#30864,#30865,#30866,#30867,#30868,#30869,#30870,#30871,#30872,#30873,#30874,
#30875,#30876,#30877,#30878,#30879,#30880,#30881,#30882,#30883,#30884,#30885,
#30886,#30887,#30888,#30889,#30890,#30891,#30892,#30893,#30894,#30895,#30896,
#30897,#30898,#30899,#30900,#30901,#30902,#30903,#30904,#30905,#30906,#30907,
#30908,#30909,#30910,#30911,#30912,#30913,#30914,#30915,#30916,#30917,#30918,
#30919,#30920,#30921,#30922,#30923,#30924,#30925,#30926,#30927,#30928,#30929,
#30930,#30931,#30932,#30933,#30934,#30935,#30936,#30937,#30938,#30939,#30940,
#30941,#30942,#30943,#30944,#30945,#30946,#30947,#30948,#30949,#30950,#30951,
#30952,#30953,#30954,#30955,#30956,#30957,#30958,#30959,#30960,#30961,#30962,
#30963,#30964,#30965,#30966,#30967,#30968,#30969,#30970,#30971,#30972,#30973,
#30974,#30975,#30976,#30977,#30978,#30979,#30980,#30981,#30982,#30983,#30984,
#30985,#30986,#30987,#30988,#30989,#30990,#30991,#30992,#30993,#30994,#30995,
#30996,#30997,#30998,#30999,#31000,#31001,#31002,#31003,#31004,#31005,#31006,
#31007),.UNSPECIFIED.,.F.,.F.,(4,2,2,2,2,2,2,2,2,2,2,2,2,2,2,2,2,2,2,2,
2,2,2,2,2,2,2,2,2,2,2,2,2,2,2,2,2,2,2,2,2,2,2,2,2,2,2,2,2,2,2,2,2,2,2,2,
2,2,2,2,2,2,2,2,2,2,2,2,2,2,2,2,2,2,2,2,2,2,2,4),(-0.926487082041935,-0.919519046294147,
-0.853132654091859,-0.850806128732264,-0.846777685742755,-0.845165205788428,
-0.843986415478232,-0.842679504961684,-0.840767190191302,-0.835647875483367,
-0.806046589922917,-0.756015259050599,-0.749101116906417,-0.746347187231973,
-0.744054631341706,-0.74169868715226,-0.738233142163533,-0.728733503487495,
-0.714451857078804,-0.685274123450052,-0.652362504504582,-0.647567338036432,
-0.64564813668675,-0.644470029801406,-0.643162466602563,-0.641246764996082,
-0.63610391052732,-0.606208788186661,-0.556561968077072,-0.550301752083055,
-0.546954121900428,-0.544855314483211,-0.542552296799797,-0.53935551746919,
-0.531635214359003,-0.520791476422158,-0.459490915981134,-0.449250893738567,
-0.446716110709871,-0.445257718833719,-0.444008966874389,-0.442388729902252,
-0.439001728829059,-0.410091087056446,-0.359401712627847,-0.350866874655805,
-0.347441217530255,-0.345328037532181,-0.343036517516631,-0.339905236346695,
-0.332578883096989,-0.322449737284953,-0.271172416483522,-0.262655587733686,
-0.249991584963173,-0.247518200743472,-0.245943073796501,-0.244686075622419,
-0.243189084274288,-0.240573585903472,-0.226724147250775,-0.189797330148935,
-0.154670677974332,-0.149998640334782,-0.147098871138603,-0.144842338239581,
-0.142348119410802,-0.139775265701751,-0.131246496577364,-0.106109691571056,
-0.0845309477201506,-0.0511203434290437,-0.0480282735500214,-0.0464460638951027,
-0.0451887123291273,-0.0436975490125595,-0.0421061898407145,-0.0395976931801813,
-0.0347318331322307,-0.000589557231629116),.UNSPECIFIED.);
#467=B_SPLINE_CURVE_WITH_KNOTS('',3,(#31008,#31009,#31010,#31011,#31012,
#31013,#31014,#31015,#31016,#31017,#31018,#31019,#31020,#31021,#31022,#31023,
#31024,#31025,#31026,#31027,#31028,#31029,#31030,#31031,#31032,#31033,#31034,
#31035,#31036,#31037,#31038,#31039,#31040,#31041,#31042,#31043,#31044,#31045,
#31046,#31047,#31048,#31049,#31050,#31051,#31052,#31053,#31054,#31055,#31056,
#31057,#31058,#31059,#31060,#31061),.UNSPECIFIED.,.F.,.F.,(4,2,2,2,2,2,
2,2,2,2,2,2,2,2,2,2,2,2,2,2,2,2,2,2,2,2,4),(-2.51392997756644,-2.47925034003837,
-2.46787561577195,-2.46443006814493,-2.46131418039933,-2.45902571130518,
-2.45690956220446,-2.45402383239197,-2.44677206785488,-2.40623254515391,
-2.37652497658567,-2.36409290225745,-2.36161581258405,-2.3601212717904,
-2.35886448832694,-2.35728731252615,-2.35421766679582,-2.33316258505554,
-2.28232116150033,-2.26711255886796,-2.2632077429606,-2.2606581810041,-2.25841224411778,
-2.25560730943267,-2.25124731827107,-2.22831283676925,-2.18313823310106),
 .UNSPECIFIED.);
#468=B_SPLINE_CURVE_WITH_KNOTS('',3,(#31062,#31063,#31064,#31065,#31066,
#31067,#31068,#31069,#31070,#31071,#31072,#31073,#31074,#31075,#31076,#31077,
#31078,#31079,#31080,#31081,#31082,#31083,#31084,#31085,#31086,#31087,#31088,
#31089,#31090,#31091,#31092,#31093,#31094,#31095,#31096,#31097,#31098,#31099,
#31100,#31101,#31102,#31103,#31104,#31105,#31106,#31107,#31108,#31109,#31110,
#31111,#31112,#31113,#31114,#31115,#31116,#31117,#31118,#31119,#31120,#31121,
#31122,#31123,#31124,#31125,#31126,#31127,#31128,#31129,#31130,#31131,#31132,
#31133,#31134,#31135,#31136,#31137,#31138,#31139,#31140,#31141,#31142,#31143,
#31144,#31145,#31146,#31147,#31148,#31149,#31150,#31151,#31152,#31153,#31154,
#31155,#31156,#31157,#31158,#31159,#31160,#31161,#31162,#31163,#31164,#31165,
#31166,#31167,#31168,#31169,#31170,#31171,#31172,#31173,#31174,#31175,#31176,
#31177,#31178,#31179,#31180,#31181,#31182,#31183,#31184,#31185,#31186,#31187,
#31188,#31189,#31190,#31191,#31192,#31193,#31194,#31195,#31196,#31197,#31198,
#31199,#31200,#31201,#31202,#31203,#31204,#31205,#31206,#31207,#31208,#31209,
#31210,#31211,#31212,#31213,#31214,#31215,#31216,#31217,#31218,#31219,#31220,
#31221,#31222,#31223,#31224,#31225,#31226,#31227,#31228,#31229,#31230,#31231,
#31232,#31233,#31234,#31235,#31236,#31237,#31238,#31239,#31240,#31241,#31242,
#31243,#31244,#31245,#31246,#31247,#31248,#31249,#31250,#31251,#31252,#31253,
#31254,#31255,#31256,#31257,#31258,#31259,#31260,#31261,#31262,#31263,#31264,
#31265,#31266,#31267,#31268,#31269,#31270,#31271,#31272,#31273,#31274,#31275,
#31276,#31277,#31278,#31279,#31280,#31281,#31282,#31283,#31284,#31285,#31286,
#31287,#31288,#31289),.UNSPECIFIED.,.F.,.F.,(4,2,2,2,2,2,2,2,2,2,2,2,2,
2,2,2,2,2,2,2,2,2,2,2,2,2,2,2,2,2,2,2,2,2,2,2,2,2,2,2,2,2,2,2,2,2,2,2,2,
2,2,2,2,2,2,2,2,2,2,2,2,2,2,2,2,2,2,2,2,2,2,2,2,2,2,2,2,2,2,2,2,2,2,2,2,
2,2,2,2,2,2,2,2,2,2,2,2,2,2,2,2,2,2,2,2,2,2,2,2,2,2,2,2,4),(-1.58789531626404,
-1.56632330799281,-1.55260822009488,-1.54994147171121,-1.5484698572259,
-1.54721170767095,-1.54560631769368,-1.54303130214716,-1.52836487517108,
-1.52461519682311,-1.5203290012024,-1.48046128243722,-1.46465960933695,
-1.45780804058913,-1.4524158361625,-1.44964691631573,-1.44740449457976,
-1.44483119678367,-1.44047708513609,-1.42375988623407,-1.419731981072,-1.36904200254157,
-1.35330846543775,-1.35054560027695,-1.34905323578783,-1.34779674539953,
-1.3462180236831,-1.34313981633201,-1.32173579179229,-1.28557433526854,
-1.25741014251873,-1.25304727454674,-1.25024182370792,-1.24799635770079,
-1.24544828740429,-1.24109590882473,-1.22262385693901,-1.17719385718619,
-1.17046508857678,-1.15414199680576,-1.15148964436731,-1.14986095769563,
-1.14860062026286,-1.14714480680467,-1.14455135921006,-1.13215052476846,
-1.10262864288724,-1.06189124980245,-1.05464303971722,-1.05175835511275,
-1.04964284529301,-1.04735495072256,-1.04423965684726,-1.0370016077036,
-1.02702903140207,-0.976068121315767,-0.954911323489691,-0.951838779759563,
-0.950261178635078,-0.949004629329425,-0.947511063962971,-0.94474301817856,
-0.928891577303083,-0.876993434721977,-0.857931354426813,-0.853400809660581,
-0.850786910127888,-0.848568451621496,-0.845859632614358,-0.840759179004347,
-0.802211488329657,-0.75959716218359,-0.758246928981988,-0.753248326244628,
-0.751295777078435,-0.750111692639656,-0.748811193966249,-0.746929145356903,
-0.742010928837825,-0.734685218248878,-0.710887218221637,-0.662321753614042,
-0.655418454892473,-0.652592377943891,-0.650491434511711,-0.648191638506678,
-0.645009619039459,-0.637375560064032,-0.626688763387258,-0.56806706677885,
-0.555215516452342,-0.552734240137113,-0.551157005829997,-0.549900336856127,
-0.548406142281509,-0.545635648562147,-0.529732423329915,-0.47730445538788,
-0.458750750228605,-0.454255168907759,-0.45164906871098,-0.44940849042876,
-0.446680157024712,-0.441486998095788,-0.396751603873804,-0.394935613176538,
-0.358755424237927,-0.354020532344979,-0.352111656716646,-0.350935627155792,
-0.349626272018241,-0.347700870858144,-0.342489365087485,-0.331435948914524),
 .UNSPECIFIED.);
#469=B_SPLINE_CURVE_WITH_KNOTS('',3,(#31294,#31295,#31296,#31297,#31298,
#31299,#31300,#31301,#31302,#31303,#31304,#31305,#31306,#31307,#31308,#31309,
#31310,#31311,#31312,#31313,#31314,#31315,#31316,#31317,#31318,#31319,#31320,
#31321,#31322,#31323,#31324,#31325,#31326,#31327,#31328,#31329,#31330,#31331,
#31332,#31333,#31334,#31335,#31336,#31337,#31338,#31339,#31340,#31341,#31342,
#31343,#31344,#31345,#31346,#31347,#31348,#31349,#31350,#31351,#31352,#31353,
#31354,#31355,#31356,#31357,#31358,#31359,#31360,#31361,#31362,#31363,#31364,
#31365,#31366,#31367,#31368,#31369,#31370,#31371,#31372,#31373,#31374,#31375,
#31376,#31377,#31378,#31379,#31380,#31381,#31382,#31383,#31384,#31385,#31386,
#31387,#31388,#31389,#31390,#31391,#31392,#31393,#31394,#31395,#31396,#31397,
#31398,#31399,#31400,#31401,#31402,#31403,#31404,#31405,#31406,#31407,#31408,
#31409,#31410,#31411,#31412,#31413,#31414,#31415,#31416,#31417,#31418,#31419,
#31420,#31421,#31422,#31423,#31424,#31425,#31426,#31427,#31428,#31429,#31430,
#31431,#31432,#31433,#31434,#31435,#31436,#31437,#31438,#31439,#31440,#31441,
#31442,#31443,#31444,#31445,#31446,#31447,#31448,#31449,#31450,#31451,#31452,
#31453,#31454,#31455,#31456,#31457,#31458,#31459,#31460,#31461,#31462,#31463,
#31464,#31465,#31466,#31467,#31468,#31469,#31470,#31471,#31472,#31473,#31474,
#31475,#31476,#31477,#31478,#31479,#31480,#31481,#31482,#31483,#31484,#31485,
#31486,#31487,#31488,#31489,#31490,#31491,#31492,#31493,#31494,#31495,#31496,
#31497,#31498,#31499,#31500,#31501,#31502,#31503,#31504,#31505,#31506,#31507,
#31508,#31509),.UNSPECIFIED.,.F.,.F.,(4,2,2,2,2,2,2,2,2,2,2,2,2,2,2,2,2,
2,2,2,2,2,2,2,2,2,2,2,2,2,2,2,2,2,2,2,2,2,2,2,2,2,2,2,2,2,2,2,2,2,2,2,2,
2,2,2,2,2,2,2,2,2,2,2,2,2,2,2,2,2,2,2,2,2,2,2,2,2,2,2,2,2,2,2,2,2,2,2,2,
2,2,2,2,2,2,2,2,2,2,2,2,2,2,2,2,2,2,4),(-2.18248318461725,-2.16336349765169,
-2.14775642214826,-2.14362542823053,-2.14112620280769,-2.13887266462903,
-2.13598720331341,-2.13135952756185,-2.09101285713337,-2.05871537336153,
-2.04532988201391,-2.04268065038738,-2.04121280606555,-2.03995418937083,
-2.03834340879016,-2.03575055044026,-2.02071709027729,-2.00365287757137,
-1.96641619692546,-1.9486888150696,-1.94438995119981,-1.94185372330336,
-1.9396067640389,-1.93678358100428,-1.93236219595033,-1.90777381868706,
-1.86134716771145,-1.84609173769782,-1.84334996726934,-1.84186210921606,
-1.84060528429423,-1.8390208785363,-1.83651548318221,-1.82321810605045,
-1.76511054911628,-1.74897914314285,-1.74480425872534,-1.74229536573777,
-1.74004382070738,-1.73717565454415,-1.73260549874066,-1.70345877118439,
-1.66127661793546,-1.64658360086218,-1.64386799739637,-1.64238580896394,
-1.64112861226076,-1.63953716091862,-1.636399004779,-1.60850569889185,-1.56832060422808,
-1.54990317304396,-1.54555492678409,-1.54300786036086,-1.54076241299782,
-1.53795583626916,-1.53358894387216,-1.51044337442874,-1.46264124661311,
-1.45229689633146,-1.44595822958394,-1.44388358670144,-1.44254247171398,
-1.4412544048148,-1.43936940494194,-1.43477616295435,-1.3953936444425,-1.36569265540894,
-1.35007293617909,-1.34594054339681,-1.34344082785594,-1.34118707567517,
-1.33830165647755,-1.33367469206995,-1.30235639717736,-1.25699012620154,
-1.24737099945124,-1.24489073699183,-1.24344531414065,-1.24230973545728,
-1.24073297319326,-1.23756375875274,-1.2334216389086,-1.22350116828241,
-1.18051471624533,-1.15227357639197,-1.1477288737738,-1.14486812041644,
-1.14261707205833,-1.1401032078919,-1.13590696259556,-1.11951961510119,
-1.05866957790602,-1.04802214982316,-1.04545456805297,-1.04398892211783,
-1.04272957398718,-1.04111446922409,-1.03775234990613,-1.00610343628861,
-0.955550692319651,-0.949374314961531,-0.946049295718204,-0.943954770855837,
-0.941648411420969,-0.938431986650012,-0.930589042675148,-0.926487082041935),
 .UNSPECIFIED.);
#470=B_SPLINE_CURVE_WITH_KNOTS('',3,(#31511,#31512,#31513,#31514,#31515,
#31516,#31517,#31518,#31519,#31520,#31521,#31522,#31523,#31524,#31525,#31526,
#31527,#31528,#31529,#31530,#31531,#31532,#31533,#31534,#31535,#31536,#31537,
#31538,#31539,#31540,#31541,#31542,#31543,#31544,#31545,#31546,#31547,#31548,
#31549,#31550,#31551,#31552,#31553,#31554,#31555,#31556,#31557,#31558,#31559,
#31560,#31561,#31562,#31563,#31564,#31565,#31566,#31567,#31568),
 .UNSPECIFIED.,.F.,.F.,(4,2,2,2,2,2,2,2,2,2,2,2,2,2,2,2,2,2,2,2,2,2,2,2,
2,2,2,2,4),(-0.331435948914524,-0.31172364526831,-0.263170569126268,-0.256269729644499,
-0.253443923322989,-0.25134291324687,-0.24904278206988,-0.245923315505089,
-0.23861127550794,-0.228414704350684,-0.176361379217015,-0.170372043346642,
-0.156223267255245,-0.153672912463893,-0.152074692451328,-0.150816698445778,
-0.149338891153073,-0.147766329218671,-0.141813366022237,-0.117459937775749,
-0.0948122256869664,-0.0607635253584692,-0.0560985289222733,-0.0532013378053364,
-0.0509457242613279,-0.0484514222973981,-0.0458781266326321,-0.0420670449395709,
-0.000589526463412705),.UNSPECIFIED.);
#471=B_SPLINE_CURVE_WITH_KNOTS('',3,(#31569,#31570,#31571,#31572,#31573,
#31574,#31575,#31576,#31577,#31578,#31579,#31580,#31581,#31582,#31583,#31584,
#31585,#31586,#31587,#31588,#31589,#31590,#31591,#31592,#31593,#31594,#31595,
#31596,#31597,#31598,#31599,#31600,#31601,#31602,#31603,#31604,#31605,#31606,
#31607,#31608,#31609,#31610,#31611,#31612,#31613,#31614,#31615,#31616,#31617,
#31618,#31619,#31620,#31621,#31622,#31623,#31624,#31625,#31626,#31627,#31628,
#31629,#31630,#31631,#31632,#31633,#31634,#31635,#31636,#31637,#31638,#31639,
#31640,#31641,#31642,#31643,#31644,#31645,#31646,#31647,#31648,#31649,#31650,
#31651,#31652,#31653,#31654,#31655,#31656,#31657,#31658,#31659,#31660,#31661,
#31662,#31663,#31664,#31665,#31666,#31667,#31668,#31669,#31670,#31671,#31672,
#31673,#31674,#31675,#31676,#31677,#31678,#31679,#31680,#31681,#31682,#31683,
#31684,#31685,#31686,#31687,#31688,#31689,#31690,#31691,#31692,#31693,#31694,
#31695,#31696,#31697,#31698,#31699,#31700,#31701,#31702,#31703,#31704,#31705,
#31706,#31707,#31708,#31709,#31710,#31711,#31712,#31713,#31714,#31715,#31716,
#31717,#31718,#31719,#31720,#31721,#31722),.UNSPECIFIED.,.F.,.F.,(4,2,2,
2,2,2,2,2,2,2,2,2,2,2,2,2,2,2,2,2,2,2,2,2,2,2,2,2,2,2,2,2,2,2,2,2,2,2,2,
2,2,2,2,2,2,2,2,2,2,2,2,2,2,2,2,2,2,2,2,2,2,2,2,2,2,2,2,2,2,2,2,2,2,2,2,
2,4),(-2.51402502574908,-2.47470167861683,-2.47062003550392,-2.46840356552127,
-2.46647396139582,-2.4651635116513,-2.46398783485779,-2.46208203007919,
-2.45736719978629,-2.42049621463849,-2.3890193225746,-2.37287541922573,
-2.36881096309099,-2.36626570081076,-2.36401867980291,-2.36120595955095,
-2.3568214433753,-2.33325996579091,-2.2888407998375,-2.27102594699721,-2.26798103580416,
-2.26639170069939,-2.26513400598461,-2.26364870331146,-2.26099585330683,
-2.24918990129547,-2.18952280113643,-2.17323531011668,-2.16904625267641,
-2.1665334770377,-2.16428137949127,-2.16141653246269,-2.15685976884375,
-2.12825919325423,-2.08552135832312,-2.07074349462449,-2.06802285906055,
-2.06653915626993,-2.06528142973848,-2.06369029740298,-2.06055574746516,
-2.03435014487387,-1.9882078129375,-1.97842959654965,-1.97129968270036,
-1.96820233117608,-1.96591683556777,-1.96379590253879,-1.96089194998257,
-1.95353338018007,-1.90152884560886,-1.87224016666654,-1.86884281858144,
-1.86722065633448,-1.86597182032097,-1.86451497458452,-1.86198660769655,
-1.85182126508958,-1.79045289250787,-1.77960610294204,-1.77188340450194,
-1.76868628535712,-1.76638325732925,-1.76428459859174,-1.76093757618218,
-1.75467941971044,-1.70494593862386,-1.67506476043248,-1.66992302203681,
-1.66800749053168,-1.66669997964575,-1.66552188110591,-1.6636026509022,
-1.6588072438466,-1.62596585191893,-1.59196095806438,-1.5879525852104),
 .UNSPECIFIED.);
#472=B_SPLINE_CURVE_WITH_KNOTS('',3,(#31728,#31729,#31730,#31731,#31732,
#31733,#31734,#31735,#31736,#31737,#31738,#31739,#31740,#31741,#31742,#31743,
#31744,#31745,#31746,#31747,#31748,#31749,#31750,#31751,#31752,#31753,#31754,
#31755,#31756,#31757,#31758,#31759,#31760,#31761,#31762,#31763,#31764,#31765,
#31766,#31767,#31768,#31769,#31770,#31771,#31772,#31773,#31774,#31775,#31776,
#31777,#31778,#31779,#31780,#31781,#31782,#31783,#31784,#31785,#31786,#31787,
#31788,#31789,#31790,#31791,#31792,#31793,#31794,#31795,#31796,#31797,#31798,
#31799,#31800,#31801,#31802,#31803,#31804,#31805,#31806,#31807,#31808,#31809,
#31810,#31811,#31812,#31813,#31814,#31815,#31816,#31817,#31818,#31819,#31820,
#31821,#31822,#31823,#31824,#31825,#31826,#31827,#31828,#31829,#31830,#31831,
#31832,#31833,#31834,#31835,#31836,#31837,#31838,#31839,#31840,#31841,#31842,
#31843,#31844,#31845,#31846,#31847,#31848,#31849,#31850,#31851,#31852,#31853,
#31854,#31855,#31856,#31857,#31858,#31859,#31860,#31861,#31862,#31863,#31864,
#31865,#31866,#31867,#31868,#31869,#31870,#31871,#31872,#31873,#31874,#31875,
#31876,#31877,#31878,#31879,#31880,#31881,#31882,#31883,#31884,#31885,#31886,
#31887,#31888,#31889,#31890,#31891,#31892,#31893,#31894,#31895,#31896,#31897,
#31898,#31899,#31900,#31901,#31902,#31903,#31904,#31905,#31906,#31907,#31908,
#31909,#31910,#31911,#31912,#31913,#31914,#31915,#31916,#31917,#31918,#31919,
#31920,#31921,#31922,#31923,#31924,#31925,#31926,#31927,#31928,#31929,#31930,
#31931,#31932,#31933),.UNSPECIFIED.,.F.,.F.,(4,2,2,2,2,2,2,2,2,2,2,2,2,
2,2,2,2,2,2,2,2,2,2,2,2,2,2,2,2,2,2,2,2,2,2,2,2,2,2,2,2,2,2,2,2,2,2,2,2,
2,2,2,2,2,2,2,2,2,2,2,2,2,2,2,2,2,2,2,2,2,2,2,2,2,2,2,2,2,2,2,2,2,2,2,2,
2,2,2,2,2,2,2,2,2,2,2,2,2,2,2,2,2,4),(-0.926835277835367,-0.925873954986695,
-0.924616719560883,-0.923122054168583,-0.920351198881222,-0.904459961791444,
-0.85218402580426,-0.833475406670089,-0.828967731157254,-0.826358178249558,
-0.824116738700649,-0.821389978043216,-0.816207851056626,-0.770588219191198,
-0.733406653481095,-0.728695513022017,-0.726790111156261,-0.725614346494368,
-0.724303452166689,-0.722372575413242,-0.717126617220737,-0.685931186638188,
-0.637914418002453,-0.630964077153999,-0.628128997746839,-0.626025068300671,
-0.623725618163677,-0.62055071342649,-0.612965900694323,-0.602370404817436,
-0.571289038902266,-0.533831200997893,-0.5291332070713,-0.527230013076427,
-0.52605466001535,-0.52474330552582,-0.522810143482474,-0.517548115017041,
-0.509530608633596,-0.457439357740223,-0.447738933322376,-0.433588926130673,
-0.429427092553468,-0.426919987581367,-0.424666203224915,-0.421789894136978,
-0.41586475120717,-0.379738571169095,-0.339499260650803,-0.330648600981391,
-0.328211072449628,-0.326788996218543,-0.325521122392203,-0.323833035129925,
-0.320086179787175,-0.290444882365525,-0.238142037225003,-0.231476457226726,
-0.228493681253355,-0.226218043360304,-0.226090576380072,-0.226019531974051,
-0.225975147795664,-0.225924403061927,-0.22587830618997,-0.225836428431162,
-0.225798378662318,-0.225763802883822,-0.225732380059235,-0.225703819142697,
-0.2256778562844,-0.225654252329823,-0.225632790482336,-0.225613274183203,
-0.225595525137274,-0.225569083041879,-0.225543190903403,-0.22551783493928,
-0.225493001826754,-0.225468678521816,-0.225444852352635,-0.222797620932892,
-0.2179184717921,-0.211809510273456,-0.198416180491977,-0.147913974553709,
-0.131910990608478,-0.129270577017266,-0.127644936627505,-0.126384195817458,
-0.124924731411772,-0.12231708124785,-0.109694986464427,-0.0577111029791184,
-0.0429217872131351,-0.0332814200974314,-0.029681477805666,-0.0275353780005982,
-0.0253744016189034,-0.0231701734708456,-0.0203093949989657,-0.0130520156989647,
-0.000589121680142322),.UNSPECIFIED.);
#473=B_SPLINE_CURVE_WITH_KNOTS('',3,(#31934,#31935,#31936,#31937,#31938,
#31939,#31940,#31941,#31942,#31943,#31944,#31945,#31946,#31947,#31948,#31949,
#31950,#31951,#31952,#31953,#31954,#31955,#31956,#31957,#31958,#31959,#31960,
#31961,#31962,#31963,#31964,#31965,#31966,#31967,#31968,#31969,#31970,#31971,
#31972,#31973,#31974,#31975,#31976,#31977,#31978,#31979,#31980,#31981,#31982,
#31983,#31984,#31985,#31986,#31987,#31988,#31989,#31990,#31991,#31992,#31993,
#31994,#31995,#31996,#31997,#31998,#31999,#32000,#32001,#32002,#32003,#32004,
#32005,#32006,#32007,#32008,#32009,#32010,#32011,#32012,#32013,#32014,#32015,
#32016,#32017),.UNSPECIFIED.,.F.,.F.,(4,2,2,2,2,2,2,2,2,2,2,2,2,2,2,2,2,
2,2,2,2,2,2,2,2,2,2,2,2,2,2,2,2,2,2,2,2,2,2,2,2,4),(-2.51280355570323,-2.45942325427332,
-2.44426263417454,-2.44152553787292,-2.44003884905819,-2.43878219077984,
-2.43719695276756,-2.43408746645967,-2.41001272855345,-2.37137025137207,
-2.35597755753649,-2.34924913535989,-2.34398785574709,-2.34125531572185,
-2.3412229317397,-2.34118921587799,-2.34115408029595,-2.34111742920532,
-2.3410791580746,-2.34103915256707,-2.34099728740793,-2.34095342507851,
-2.34090741430289,-2.34085908829961,-2.34080826280075,-2.34077591693697,
-2.34073458978196,-2.3406815253674,-2.33843678314745,-2.33563570741767,
-2.33128627055838,-2.30827056865735,-2.26033131742769,-2.24997680995143,
-2.24363387596532,-2.24155886128455,-2.24021776650185,-2.23892994151421,
-2.23704564013059,-2.23245581633457,-2.19302657914985,-2.18248318461725),
 .UNSPECIFIED.);
#474=B_SPLINE_CURVE_WITH_KNOTS('',3,(#32018,#32019,#32020,#32021,#32022,
#32023,#32024,#32025,#32026,#32027,#32028,#32029,#32030,#32031,#32032,#32033,
#32034,#32035,#32036,#32037,#32038,#32039,#32040,#32041,#32042,#32043,#32044,
#32045,#32046,#32047,#32048,#32049,#32050,#32051,#32052,#32053,#32054,#32055,
#32056,#32057,#32058,#32059,#32060,#32061,#32062,#32063,#32064,#32065,#32066,
#32067,#32068,#32069,#32070,#32071,#32072,#32073,#32074,#32075,#32076,#32077,
#32078,#32079,#32080,#32081,#32082,#32083,#32084,#32085,#32086,#32087,#32088,
#32089,#32090,#32091,#32092,#32093,#32094,#32095,#32096,#32097,#32098,#32099,
#32100,#32101,#32102,#32103,#32104,#32105,#32106,#32107,#32108,#32109,#32110,
#32111,#32112,#32113,#32114,#32115,#32116,#32117,#32118,#32119,#32120,#32121,
#32122,#32123,#32124,#32125,#32126,#32127,#32128,#32129,#32130,#32131,#32132,
#32133,#32134,#32135,#32136,#32137,#32138,#32139,#32140,#32141,#32142,#32143,
#32144,#32145,#32146,#32147,#32148,#32149,#32150,#32151,#32152,#32153,#32154,
#32155,#32156,#32157,#32158,#32159,#32160,#32161,#32162,#32163,#32164,#32165,
#32166,#32167,#32168,#32169,#32170,#32171,#32172,#32173,#32174,#32175,#32176,
#32177,#32178,#32179,#32180,#32181,#32182,#32183,#32184,#32185,#32186,#32187,
#32188,#32189,#32190,#32191,#32192,#32193,#32194,#32195,#32196,#32197,#32198,
#32199,#32200,#32201,#32202,#32203,#32204,#32205,#32206,#32207,#32208,#32209,
#32210,#32211,#32212,#32213,#32214,#32215,#32216,#32217,#32218,#32219,#32220,
#32221,#32222,#32223,#32224,#32225,#32226,#32227,#32228,#32229,#32230,#32231,
#32232,#32233,#32234,#32235,#32236,#32237,#32238,#32239),.UNSPECIFIED.,
 .F.,.F.,(4,2,2,2,2,2,2,2,2,2,2,2,2,2,2,2,2,2,2,2,2,2,2,2,2,2,2,2,2,2,2,
2,2,2,2,2,2,2,2,2,2,2,2,2,2,2,2,2,2,2,2,2,2,2,2,2,2,2,2,2,2,2,2,2,2,2,2,
2,2,2,2,2,2,2,2,2,2,2,2,2,2,2,2,2,2,2,2,2,2,2,2,2,2,2,2,2,2,2,2,2,2,2,2,
2,2,2,2,2,2,2,4),(-1.5879525852104,-1.57458975846264,-1.57031589714921,
-1.56778442442157,-1.56553552113557,-1.56270165497985,-1.55824738786618,
-1.53283690906585,-1.48713337491167,-1.47695949055901,-1.47069522210094,
-1.46862911772098,-1.4672894683517,-1.46599934335257,-1.46410597685683,
-1.45946567791737,-1.42081262487195,-1.3905755159231,-1.37478462430487,
-1.37063640389922,-1.36813248210081,-1.36587836901618,-1.36299724250785,
-1.35838683962124,-1.32784152922721,-1.32046832379782,-1.29791034683781,
-1.27511800236025,-1.27060440611576,-1.26878500556775,-1.26749616821184,
-1.26613064332966,-1.26394701480732,-1.25734176148359,-1.20613204574239,
-1.17688360054628,-1.17230876636834,-1.1694384613991,-1.16718575653382,
-1.16467611364536,-1.16050128245191,-1.14438835909185,-1.11308895462519,
-1.07593598975129,-1.07122413184009,-1.06931887704709,-1.06814334149643,
-1.06683285438391,-1.06490286406299,-1.0596611051626,-1.02851446561567,
-0.980429497837874,-0.973484364673308,-0.970650578686587,-0.968547315311905,
-0.966248311079458,-0.96307351276614,-0.955486563056699,-0.944886569682506,
-0.913780305458279,-0.876351126063622,-0.87165146342062,-0.869748261097883,
-0.868573111342117,-0.867262200115879,-0.865330097651549,-0.860073486389425,
-0.852066583450143,-0.800148059178257,-0.789871417493344,-0.776037280291282,
-0.771909406682415,-0.76941016981365,-0.767155410872964,-0.764266713540674,
-0.758275540828574,-0.71361597576308,-0.67677955776591,-0.672063761634389,
-0.670157855106759,-0.668982205056979,-0.667671868691615,-0.665742584942656,
-0.66050570585247,-0.629421761550526,-0.581258922383746,-0.574319923965814,
-0.571487204135684,-0.569384211666245,-0.567084995480548,-0.563908970881281,
-0.556314561231851,-0.545700973670453,-0.514525319663746,-0.477193503629126,
-0.47249153165773,-0.470587950222745,-0.469412736280955,-0.46810191850319,
-0.466170240828056,-0.460916546151231,-0.452915598598613,-0.401094191418584,
-0.378171405590259,-0.373813392885962,-0.371008939127249,-0.368762898642373,
-0.366212698859851,-0.361853005045509,-0.343290147407682,-0.331151912909351),
 .UNSPECIFIED.);
#475=B_SPLINE_CURVE_WITH_KNOTS('',3,(#32244,#32245,#32246,#32247,#32248,
#32249,#32250,#32251,#32252,#32253,#32254,#32255,#32256,#32257,#32258,#32259,
#32260,#32261,#32262,#32263,#32264,#32265,#32266,#32267,#32268,#32269,#32270,
#32271,#32272,#32273,#32274,#32275,#32276,#32277,#32278,#32279,#32280,#32281,
#32282,#32283,#32284,#32285,#32286,#32287,#32288,#32289,#32290,#32291,#32292,
#32293,#32294,#32295,#32296,#32297,#32298,#32299,#32300,#32301,#32302,#32303,
#32304,#32305,#32306,#32307,#32308,#32309,#32310,#32311,#32312,#32313,#32314,
#32315,#32316,#32317,#32318,#32319,#32320,#32321,#32322,#32323,#32324,#32325,
#32326,#32327,#32328,#32329,#32330,#32331,#32332,#32333,#32334,#32335,#32336,
#32337,#32338,#32339,#32340,#32341,#32342,#32343,#32344,#32345,#32346,#32347,
#32348,#32349,#32350,#32351,#32352,#32353,#32354,#32355,#32356,#32357,#32358,
#32359,#32360,#32361,#32362,#32363,#32364,#32365,#32366,#32367,#32368,#32369,
#32370,#32371,#32372,#32373,#32374,#32375,#32376,#32377,#32378,#32379,#32380,
#32381,#32382,#32383,#32384,#32385,#32386,#32387,#32388,#32389,#32390,#32391,
#32392,#32393,#32394,#32395,#32396,#32397,#32398,#32399,#32400,#32401,#32402,
#32403,#32404,#32405,#32406,#32407,#32408,#32409,#32410,#32411,#32412,#32413,
#32414,#32415,#32416,#32417,#32418,#32419,#32420,#32421,#32422,#32423,#32424,
#32425,#32426,#32427,#32428,#32429,#32430,#32431,#32432,#32433,#32434,#32435,
#32436,#32437,#32438,#32439,#32440,#32441,#32442,#32443,#32444,#32445,#32446,
#32447,#32448,#32449,#32450,#32451,#32452,#32453,#32454,#32455,#32456,#32457,
#32458,#32459,#32460,#32461),.UNSPECIFIED.,.F.,.F.,(4,2,2,2,2,2,2,2,2,2,
2,2,2,2,2,2,2,2,2,2,2,2,2,2,2,2,2,2,2,2,2,2,2,2,2,2,2,2,2,2,2,2,2,2,2,2,
2,2,2,2,2,2,2,2,2,2,2,2,2,2,2,2,2,2,2,2,2,2,2,2,2,2,2,2,2,2,2,2,2,2,2,2,
2,2,2,2,2,2,2,2,2,2,2,2,2,2,2,2,2,2,2,2,2,2,2,2,2,2,4),(-2.18338867985252,
-2.17304102988321,-2.14381756447417,-2.1271921983873,-2.12439157541843,
-2.12289076920439,-2.12163422263203,-2.12006425966396,-2.11702845541298,
-2.09720648249968,-2.0452628747484,-2.02984328028683,-2.0257272289343,-2.02323064208988,
-2.02097537416667,-2.01808198470289,-2.01342992921446,-1.97361130766299,
-1.9449569257605,-1.92769844533424,-1.92487370296174,-1.92336787825266,
-1.92211158462659,-1.9205475312516,-1.91811005656014,-1.90600388047791,
-1.85236702256448,-1.83831538914147,-1.82892820216747,-1.82547838001922,
-1.82312566603208,-1.82083051271919,-1.81806650850368,-1.81108909052652,
-1.76168820128402,-1.73157398844635,-1.72641370241309,-1.72449536261635,
-1.72318718926321,-1.72200949545005,-1.7200926604049,-1.71531175522481,
-1.68116104507842,-1.64814376354915,-1.63106079131407,-1.62680882216696,
-1.62428212525191,-1.62203237841302,-1.61919059209525,-1.61471032533007,
-1.58857937680316,-1.54357474743067,-1.52849283191948,-1.52575798827675,
-1.52427119393879,-1.52301364856646,-1.5214262796317,-1.51891239275892,
-1.50547285596822,-1.49829187463721,-1.47797313779314,-1.43317493124286,
-1.42799749527775,-1.42527192048741,-1.42303080119901,-1.42042087737265,
-1.41591070050339,-1.39716179654827,-1.34490038017141,-1.32900828147958,
-1.32623749695321,-1.32474293226893,-1.32348580182992,-1.32190778247953,
-1.31942492141555,-1.30654851665753,-1.30464536226076,-1.30116546215753,
-1.28765141072812,-1.25764727507516,-1.23319178199413,-1.22877343820248,
-1.22595018234654,-1.22370189341153,-1.22116281080147,-1.2168557943578,
-1.19904517832619,-1.1614926124188,-1.14636738239161,-1.1298255910023,-1.12716366101996,
-1.12553164279912,-1.1242703544355,-1.12281527533551,-1.12022747617846,
-1.10793741531231,-1.07891704772819,-1.03752382415657,-1.03028082601933,
-1.02739609263648,-1.02527979888145,-1.02299033730041,-1.01987161430627,
-1.01261958760833,-1.00262356482312,-0.951655457150748,-0.930525054975316,
-0.927452143251984,-0.926835277835367),.UNSPECIFIED.);
#476=B_SPLINE_CURVE_WITH_KNOTS('',3,(#32463,#32464,#32465,#32466,#32467,
#32468,#32469,#32470,#32471,#32472,#32473,#32474,#32475,#32476,#32477,#32478,
#32479,#32480,#32481,#32482,#32483,#32484,#32485,#32486,#32487,#32488,#32489,
#32490,#32491,#32492,#32493,#32494,#32495,#32496,#32497,#32498,#32499,#32500,
#32501,#32502,#32503,#32504,#32505,#32506,#32507,#32508,#32509,#32510,#32511,
#32512,#32513,#32514,#32515,#32516,#32517,#32518,#32519,#32520,#32521,#32522,
#32523,#32524,#32525,#32526,#32527,#32528,#32529,#32530,#32531,#32532,#32533,
#32534,#32535,#32536,#32537,#32538,#32539,#32540,#32541,#32542,#32543,#32544,
#32545,#32546,#32547,#32548),.UNSPECIFIED.,.F.,.F.,(4,2,2,2,2,2,2,2,2,2,
2,2,2,2,2,2,2,2,2,2,2,2,2,2,2,2,2,2,2,2,2,2,2,2,2,2,2,2,2,2,2,2,4),(-0.331151912909351,
-0.302471423886003,-0.275268135967566,-0.272128314356745,-0.270536129369491,
-0.269278417518081,-0.267795714444919,-0.265079445863502,-0.250389152885383,
-0.208251852747366,-0.179067406331704,-0.174477397694502,-0.171602589951601,
-0.169349459873731,-0.169264139805164,-0.169198402560599,-0.169147373229639,
-0.169107530917496,-0.169076282320816,-0.169025601796399,-0.16897739650466,
-0.168931486879703,-0.168887710062428,-0.168845918062359,-0.168805976109094,
-0.168767761222614,-0.168731161031078,-0.168696072668769,-0.168662401753735,
-0.168630061519431,-0.165890851613642,-0.160611945406604,-0.153849295199289,
-0.138345925343512,-0.0988768538035574,-0.0756831005859633,-0.072574003326672,
-0.0709883571160977,-0.0697310616221267,-0.0682432680326189,-0.0655032703358452,
-0.0503020257269651,-0.000590129853255855),.UNSPECIFIED.);
#477=B_SPLINE_CURVE_WITH_KNOTS('',3,(#32549,#32550,#32551,#32552,#32553,
#32554,#32555,#32556,#32557,#32558,#32559,#32560,#32561,#32562,#32563,#32564,
#32565,#32566,#32567,#32568,#32569,#32570,#32571,#32572,#32573,#32574,#32575,
#32576,#32577,#32578,#32579,#32580,#32581,#32582,#32583,#32584,#32585,#32586,
#32587,#32588,#32589,#32590,#32591,#32592,#32593,#32594,#32595,#32596,#32597,
#32598,#32599,#32600,#32601,#32602,#32603,#32604,#32605,#32606,#32607,#32608,
#32609,#32610,#32611,#32612,#32613,#32614,#32615,#32616,#32617,#32618,#32619,
#32620,#32621,#32622,#32623,#32624,#32625,#32626,#32627,#32628,#32629,#32630,
#32631,#32632,#32633,#32634,#32635,#32636,#32637,#32638,#32639,#32640,#32641,
#32642,#32643,#32644,#32645,#32646,#32647,#32648,#32649,#32650,#32651,#32652,
#32653,#32654,#32655,#32656,#32657,#32658,#32659,#32660,#32661,#32662,#32663,
#32664,#32665,#32666,#32667,#32668,#32669,#32670,#32671,#32672,#32673,#32674,
#32675,#32676,#32677,#32678,#32679,#32680,#32681,#32682,#32683,#32684,#32685,
#32686,#32687,#32688,#32689,#32690),.UNSPECIFIED.,.F.,.F.,(4,3,3,3,3,3,
3,3,3,3,3,3,3,3,3,3,3,3,3,3,3,3,3,3,3,3,3,3,3,3,3,3,3,3,3,3,3,3,3,3,3,3,
3,3,3,3,3,4),(147.65485471872,147.7596787603,147.864497286824,147.974284115959,
148.079269184167,148.184337191304,148.289587067188,148.303644603364,148.408603236093,
148.513404407742,148.618082360711,148.72269449813,148.82727638342,148.931863536024,
149.036561338889,149.141320371478,149.246261485861,149.301361766912,149.406320459688,
149.51112169103,149.615799702885,149.720411898661,149.824993841696,149.929581051351,
150.034278909835,150.139037997312,150.24397916487,150.299078930459,150.404037717633,
150.508839044419,150.613517152794,150.718129445701,150.822711486324,150.92729879388,
151.031996750053,151.136755935245,151.241697199507,151.296796094007,151.401755143354,
151.506556527578,151.611233913488,151.715845195958,151.820425938971,151.925011662141,
152.029704696172,152.134458843432,152.23938750251,152.284650028018),
 .UNSPECIFIED.);
#478=B_SPLINE_CURVE_WITH_KNOTS('',3,(#32696,#32697,#32698,#32699,#32700,
#32701,#32702,#32703,#32704,#32705,#32706,#32707,#32708,#32709,#32710,#32711,
#32712,#32713,#32714,#32715,#32716,#32717,#32718,#32719,#32720,#32721,#32722,
#32723,#32724,#32725,#32726,#32727,#32728,#32729,#32730,#32731,#32732,#32733,
#32734,#32735,#32736,#32737,#32738,#32739,#32740,#32741,#32742,#32743,#32744,
#32745,#32746,#32747,#32748,#32749,#32750,#32751,#32752,#32753,#32754,#32755,
#32756,#32757,#32758,#32759,#32760,#32761,#32762,#32763,#32764,#32765,#32766,
#32767,#32768,#32769,#32770,#32771,#32772,#32773,#32774,#32775,#32776,#32777,
#32778,#32779,#32780,#32781,#32782,#32783,#32784,#32785,#32786,#32787,#32788,
#32789,#32790,#32791,#32792,#32793,#32794,#32795,#32796,#32797,#32798,#32799,
#32800,#32801,#32802,#32803,#32804,#32805,#32806,#32807,#32808,#32809,#32810,
#32811,#32812,#32813,#32814,#32815,#32816,#32817,#32818,#32819,#32820,#32821,
#32822,#32823,#32824,#32825,#32826,#32827,#32828,#32829,#32830,#32831,#32832,
#32833,#32834,#32835,#32836,#32837),.UNSPECIFIED.,.F.,.F.,(4,3,3,3,3,3,
3,3,3,3,3,3,3,3,3,3,3,3,3,3,3,3,3,3,3,3,3,3,3,3,3,3,3,3,3,3,3,3,3,3,3,3,
3,3,3,3,3,4),(153.9380400259,153.974863605114,154.079804365441,154.184587631212,
154.289247714775,154.393842015211,154.498406122077,154.602975581005,154.707655938966,
154.812397641858,154.917321790079,154.972580768661,155.077561582248,155.182384840127,
155.28708463541,155.391718452278,155.496321823315,155.600930236945,155.705648817651,
155.810428384599,155.915389438099,155.970297932209,156.075278237136,156.180101410843,
156.284801742362,156.389436478036,156.49404114557,156.598651228907,156.703372026609,
156.808154124326,156.913118164361,156.968015095757,157.07284356268,157.177514242715,
157.282061843758,157.386543784192,157.490995815696,157.595453646235,157.700023809841,
157.804655964143,157.909472737595,157.965732259304,158.070872240667,158.175862782332,
158.280733003082,158.385531426381,158.490318442128,158.567664456021),
 .UNSPECIFIED.);
#479=B_SPLINE_CURVE_WITH_KNOTS('',3,(#32838,#32839,#32840,#32841,#32842,
#32843,#32844,#32845,#32846,#32847,#32848,#32849,#32850,#32851,#32852,#32853,
#32854,#32855,#32856,#32857,#32858,#32859,#32860,#32861,#32862,#32863,#32864,
#32865,#32866,#32867,#32868,#32869,#32870,#32871,#32872,#32873,#32874,#32875,
#32876,#32877,#32878,#32879,#32880,#32881,#32882,#32883,#32884,#32885,#32886,
#32887,#32888,#32889,#32890,#32891,#32892,#32893,#32894,#32895,#32896,#32897,
#32898,#32899,#32900,#32901,#32902,#32903,#32904,#32905,#32906,#32907,#32908,
#32909),.UNSPECIFIED.,.F.,.F.,(4,2,2,2,2,2,2,2,2,2,2,2,2,2,2,2,2,2,2,2,
2,2,2,2,2,2,2,2,2,2,2,2,2,2,2,4),(-2.5140779328986,-2.47849070595892,-2.44670937580689,
-2.42920952710399,-2.42492483703576,-2.42239027827562,-2.42014066872104,
-2.41730862047916,-2.41286246276546,-2.38769182458136,-2.34612449882485,
-2.33310382859779,-2.32811400782696,-2.32556025767983,-2.32395001442939,
-2.32246645753187,-2.32245942734251,-2.32245234484813,-2.32244520895705,
-2.32243801850278,-2.32243077248093,-2.32242346972502,-2.32241610902578,
-2.32240868916012,-2.32118643060593,-2.31961822636813,-2.31659184641,-2.29693492462091,
-2.24483702526331,-2.22939701795696,-2.2252787097483,-2.22278132735393,
-2.22052570599751,-2.21763236829677,-2.21298142448337,-2.18338867985252),
 .UNSPECIFIED.);
#480=B_SPLINE_CURVE_WITH_KNOTS('',3,(#32911,#32912,#32913,#32914,#32915,
#32916,#32917,#32918,#32919,#32920,#32921,#32922,#32923,#32924,#32925,#32926,
#32927,#32928,#32929,#32930,#32931,#32932,#32933,#32934,#32935,#32936,#32937,
#32938,#32939,#32940,#32941,#32942,#32943,#32944,#32945,#32946,#32947,#32948,
#32949,#32950,#32951,#32952,#32953,#32954,#32955,#32956,#32957,#32958,#32959,
#32960,#32961,#32962,#32963,#32964,#32965),.UNSPECIFIED.,.F.,.F.,(4,3,3,
3,3,3,3,3,3,3,3,3,3,3,3,3,3,3,4),(152.284650028018,152.294513257555,152.399472165554,
152.504273610123,152.608951831273,152.7135642338,152.818146380757,152.92273379122,
153.027431844461,153.132191123553,153.237132475827,153.292230421102,153.397521479036,
153.502654337752,153.611500759789,153.71641998599,153.821291112116,153.926162314978,
153.9380400259),.UNSPECIFIED.);
#481=B_SPLINE_CURVE_WITH_KNOTS('',3,(#32966,#32967,#32968,#32969,#32970,
#32971,#32972,#32973,#32974),.UNSPECIFIED.,.F.,.F.,(4,1,1,1,1,1,4),(153.938047498774,
154.28994758465,155.287664748197,156.285381911745,157.283099075293,158.28081623884,
158.568767222197),.UNSPECIFIED.);
#482=B_SPLINE_CURVE_WITH_KNOTS('',3,(#32978,#32979,#32980,#32981,#32982,
#32983),.UNSPECIFIED.,.F.,.F.,(4,1,1,4),(-4.09157007060747,-3.99086865419044,
-2.99315149064283,-2.06679288006903),.UNSPECIFIED.);
#483=B_SPLINE_CURVE_WITH_KNOTS('',3,(#32987,#32988,#32989,#32990,#32991),
 .UNSPECIFIED.,.F.,.F.,(4,1,4),(0.,0.997717163547601,1.11662023360664),
 .UNSPECIFIED.);
#484=B_SPLINE_CURVE_WITH_KNOTS('',3,(#32993,#32994,#32995,#32996,#32997,
#32998,#32999,#33000,#33001,#33002,#33003,#33004,#33005,#33006,#33007,#33008,
#33009,#33010,#33011,#33012,#33013,#33014,#33015,#33016,#33017,#33018,#33019,
#33020,#33021,#33022,#33023,#33024,#33025,#33026,#33027,#33028,#33029,#33030,
#33031,#33032,#33033,#33034,#33035,#33036,#33037,#33038,#33039,#33040,#33041,
#33042,#33043,#33044,#33045,#33046,#33047,#33048,#33049,#33050,#33051,#33052,
#33053,#33054,#33055,#33056,#33057,#33058,#33059,#33060,#33061,#33062,#33063,
#33064,#33065,#33066,#33067,#33068,#33069,#33070,#33071,#33072,#33073,#33074,
#33075,#33076,#33077,#33078,#33079,#33080,#33081,#33082,#33083,#33084,#33085,
#33086,#33087,#33088,#33089,#33090,#33091,#33092,#33093,#33094,#33095,#33096,
#33097,#33098,#33099,#33100,#33101,#33102,#33103,#33104,#33105,#33106,#33107,
#33108,#33109,#33110,#33111,#33112,#33113,#33114,#33115,#33116,#33117,#33118,
#33119,#33120,#33121,#33122,#33123,#33124,#33125,#33126,#33127,#33128,#33129,
#33130,#33131,#33132,#33133,#33134,#33135,#33136,#33137,#33138,#33139,#33140,
#33141,#33142,#33143,#33144,#33145,#33146,#33147,#33148,#33149,#33150,#33151,
#33152,#33153,#33154,#33155,#33156,#33157,#33158,#33159,#33160,#33161,#33162,
#33163,#33164,#33165,#33166,#33167,#33168,#33169,#33170,#33171,#33172,#33173,
#33174,#33175,#33176,#33177,#33178,#33179,#33180,#33181,#33182),
 .UNSPECIFIED.,.F.,.F.,(4,3,3,3,3,3,3,3,3,3,3,3,3,3,3,3,3,3,3,3,3,3,3,3,
3,3,3,3,3,3,3,3,3,3,3,3,3,3,3,3,3,3,3,3,3,3,3,3,3,3,3,3,3,3,3,3,3,3,3,3,
3,3,3,4),(1.11662023360664,1.21403017783247,1.31170569649031,1.40889083867501,
1.50602851129987,1.60315132101257,1.70122207253323,1.79846974995715,1.89695203852618,
1.99543432709521,2.09523986473024,2.19490213157771,2.29468330146085,2.39416483461276,
2.49361268276311,2.59305713236532,2.69308072193469,2.79266593261604,2.89290871162943,
2.99315149064282,3.09301416604425,3.19273726352095,3.29250368735464,3.39205463887835,
3.49157499828158,3.5910949646367,3.69103838702513,3.79070576812542,3.89078721115793,
3.99086865419044,4.09044699529707,4.18988074033137,4.2897188750072,4.38897039473104,
4.48818819271083,4.58740287522122,4.68769861085042,4.78705712910369,4.88782147342087,
4.98858581773805,5.08830325928589,5.18787780272281,5.28768095004317,5.38707637536471,
5.48643893157123,5.58579903228547,5.68592501953552,5.78542910701009,5.88586604414787,
5.98630298128566,6.08601752413451,6.18558951336581,6.28539334229924,6.38478707876317,
6.48414827749628,6.58350735551845,6.68363555284716,6.78313945746615,6.88357980114971,
6.98402014483327,7.09349031126651,7.2026554514492,7.31130400709731,7.39980554040953),
 .UNSPECIFIED.);
#485=B_SPLINE_CURVE_WITH_KNOTS('',3,(#33184,#33185,#33186,#33187,#33188,
#33189,#33190,#33191,#33192,#33193,#33194,#33195,#33196,#33197,#33198,#33199,
#33200,#33201,#33202,#33203,#33204,#33205,#33206,#33207,#33208,#33209,#33210,
#33211,#33212,#33213,#33214,#33215,#33216,#33217,#33218,#33219,#33220,#33221,
#33222,#33223,#33224,#33225,#33226,#33227,#33228,#33229,#33230,#33231,#33232,
#33233,#33234,#33235,#33236,#33237,#33238,#33239,#33240,#33241,#33242,#33243,
#33244,#33245,#33246,#33247,#33248,#33249,#33250,#33251,#33252,#33253,#33254,
#33255,#33256,#33257,#33258,#33259,#33260,#33261,#33262,#33263,#33264,#33265,
#33266,#33267,#33268,#33269,#33270,#33271,#33272,#33273,#33274,#33275,#33276,
#33277,#33278,#33279,#33280,#33281,#33282,#33283,#33284,#33285,#33286,#33287,
#33288,#33289,#33290,#33291,#33292,#33293,#33294,#33295,#33296,#33297,#33298,
#33299,#33300,#33301,#33302,#33303,#33304,#33305,#33306,#33307,#33308,#33309,
#33310,#33311,#33312,#33313,#33314,#33315,#33316,#33317,#33318,#33319,#33320,
#33321,#33322,#33323,#33324,#33325,#33326,#33327,#33328,#33329,#33330,#33331,
#33332,#33333,#33334,#33335,#33336,#33337,#33338,#33339,#33340,#33341,#33342,
#33343,#33344,#33345,#33346,#33347,#33348,#33349,#33350,#33351,#33352,#33353,
#33354,#33355,#33356,#33357,#33358,#33359,#33360,#33361,#33362,#33363,#33364,
#33365,#33366,#33367,#33368,#33369,#33370,#33371,#33372,#33373,#33374,#33375,
#33376),.UNSPECIFIED.,.F.,.F.,(4,3,3,3,3,3,3,3,3,3,3,3,3,3,3,3,3,3,3,3,
3,3,3,3,3,3,3,3,3,3,3,3,3,3,3,3,3,3,3,3,3,3,3,3,3,3,3,3,3,3,3,3,3,3,3,3,
3,3,3,3,3,3,3,3,4),(7.39980554078624,7.50091414539458,7.60207208886389,
7.70338883416616,7.80478910492028,7.90640042005354,7.98173730838088,8.08143708868561,
8.18099393916635,8.28080150576161,8.38017929631084,8.47952428002577,8.57886689516197,
8.6790137893536,8.7785007869756,8.87897762945204,8.97945447192849,9.0791522318597,
9.1787070823736,9.27851515151141,9.37789100753077,9.47723408588057,9.57657482757993,
9.67672402955397,9.77620925214669,9.87669044381139,9.9771716354761,10.0768652714557,
10.1764159173836,10.2762250275886,10.3755965132625,10.474935168476,10.5742714401109,
10.6744257798391,10.7739064621368,10.8743976305802,10.9748887990237,11.0745852497462,
11.1741387497813,11.2739471513801,11.3733215659471,11.4726631716966,11.5720024115391,
11.6721532992972,11.7716369630197,11.8721214627955,11.9726059625713,12.0723019306664,
12.1718549473224,12.2716634696719,12.371037402717,12.4703785287419,12.5697172913276,
12.6698687500254,12.7693519475211,12.86983753682,12.9703231261189,13.0692183781977,
13.1679810507849,13.2666427695192,13.3652350418257,13.463808588127,13.5623731344459,
13.6609891043227,13.6829908479658),.UNSPECIFIED.);
#486=B_SPLINE_CURVE_WITH_KNOTS('',3,(#33378,#33379,#33380,#33381,#33382,
#33383,#33384,#33385,#33386,#33387,#33388,#33389,#33390,#33391,#33392,#33393,
#33394,#33395,#33396,#33397,#33398,#33399,#33400,#33401,#33402,#33403,#33404,
#33405,#33406,#33407,#33408,#33409,#33410,#33411,#33412,#33413,#33414,#33415,
#33416,#33417,#33418,#33419,#33420,#33421,#33422,#33423,#33424,#33425,#33426,
#33427,#33428,#33429,#33430,#33431,#33432,#33433,#33434,#33435,#33436,#33437,
#33438,#33439,#33440,#33441,#33442,#33443,#33444,#33445,#33446,#33447,#33448,
#33449,#33450,#33451,#33452,#33453,#33454,#33455,#33456,#33457,#33458,#33459,
#33460,#33461,#33462,#33463,#33464,#33465,#33466,#33467,#33468,#33469,#33470,
#33471,#33472,#33473,#33474,#33475,#33476,#33477,#33478,#33479,#33480,#33481,
#33482,#33483,#33484,#33485,#33486,#33487,#33488,#33489,#33490,#33491,#33492,
#33493,#33494,#33495,#33496,#33497,#33498,#33499,#33500,#33501,#33502,#33503,
#33504,#33505,#33506,#33507,#33508,#33509,#33510,#33511,#33512,#33513,#33514,
#33515,#33516,#33517,#33518,#33519,#33520,#33521,#33522,#33523,#33524,#33525,
#33526,#33527,#33528,#33529,#33530,#33531,#33532,#33533,#33534,#33535,#33536,
#33537,#33538,#33539,#33540,#33541,#33542,#33543,#33544,#33545,#33546,#33547,
#33548,#33549,#33550,#33551,#33552,#33553,#33554,#33555,#33556,#33557,#33558,
#33559,#33560,#33561,#33562,#33563,#33564,#33565,#33566,#33567,#33568,#33569,
#33570),.UNSPECIFIED.,.F.,.F.,(4,3,3,3,3,3,3,3,3,3,3,3,3,3,3,3,3,3,3,3,
3,3,3,3,3,3,3,3,3,3,3,3,3,3,3,3,3,3,3,3,3,3,3,3,3,3,3,3,3,3,3,3,3,3,3,3,
3,3,3,3,3,3,3,3,4),(13.6829908482444,13.8045870330681,13.9281224185238,
13.9680402896666,14.0677361753039,14.1672891052979,14.2670976487875,14.3664714855134,
14.465812511784,14.5651511713017,14.6653027417798,14.7647858290595,14.8652716411369,
14.9657574532142,15.0654532473382,15.1650060852554,15.2648146516937,15.3641883956647,
15.4635293291348,15.5628678959341,15.663019576141,15.7625025718607,15.8629885943112,
15.9634746167618,16.0631703607544,16.1627231473695,16.262531726487,16.3619054166746,
16.4612462955444,16.5605848069985,16.6607365503262,16.7602194894246,16.860705634867,
16.9611917803094,17.0608875760243,17.1604404151583,17.2602489812456,17.3596227255052,
17.4589636589118,17.5583022252944,17.658453904935,17.7579368993666,17.8584229216118,
17.958908943857,18.0586047239988,18.1581575474241,18.2579661174216,18.35733984576,
18.4566807632012,18.556019313596,18.6561710120482,18.7556539906012,18.8561400490029,
18.9566261074046,19.0563218826592,19.1558747010642,19.2556832723002,19.3550569953302,
19.454397907366,19.5537364522654,19.6538881569371,19.7533711298283,19.8538572003902,
19.9543432709522,19.9661761551454),.UNSPECIFIED.);
#487=B_SPLINE_CURVE_WITH_KNOTS('',3,(#33572,#33573,#33574,#33575,#33576,
#33577,#33578,#33579,#33580,#33581,#33582,#33583,#33584,#33585,#33586,#33587,
#33588,#33589,#33590,#33591,#33592,#33593,#33594,#33595,#33596,#33597,#33598,
#33599,#33600,#33601,#33602,#33603,#33604,#33605,#33606,#33607,#33608,#33609,
#33610,#33611,#33612,#33613,#33614,#33615,#33616,#33617,#33618,#33619,#33620,
#33621,#33622,#33623,#33624,#33625,#33626,#33627,#33628,#33629,#33630,#33631,
#33632,#33633,#33634,#33635,#33636,#33637,#33638,#33639,#33640,#33641,#33642,
#33643,#33644,#33645,#33646,#33647,#33648,#33649,#33650,#33651,#33652,#33653,
#33654,#33655,#33656,#33657,#33658,#33659,#33660,#33661,#33662,#33663,#33664,
#33665,#33666,#33667,#33668,#33669,#33670,#33671,#33672,#33673,#33674,#33675,
#33676,#33677,#33678,#33679,#33680,#33681,#33682,#33683,#33684,#33685,#33686,
#33687,#33688,#33689,#33690,#33691,#33692,#33693,#33694,#33695,#33696,#33697,
#33698,#33699,#33700,#33701,#33702,#33703,#33704,#33705,#33706,#33707,#33708,
#33709,#33710,#33711,#33712,#33713,#33714,#33715,#33716,#33717,#33718,#33719,
#33720,#33721,#33722,#33723,#33724,#33725,#33726,#33727,#33728,#33729,#33730,
#33731,#33732,#33733,#33734,#33735,#33736,#33737,#33738,#33739,#33740,#33741,
#33742,#33743,#33744,#33745,#33746,#33747,#33748,#33749,#33750,#33751,#33752,
#33753,#33754,#33755,#33756,#33757,#33758,#33759,#33760,#33761),
 .UNSPECIFIED.,.F.,.F.,(4,3,3,3,3,3,3,3,3,3,3,3,3,3,3,3,3,3,3,3,3,3,3,3,
3,3,3,3,3,3,3,3,3,3,3,3,3,3,3,3,3,3,3,3,3,3,3,3,3,3,3,3,3,3,3,3,3,3,3,3,
3,3,3,4),(19.9661761554973,20.0656647147026,20.165010707087,20.2642422239616,
20.3634112611229,20.4625485789532,20.5616848984301,20.6609195515273,20.760201924141,
20.8596630799886,20.9520604344998,21.0517562140533,21.1513090368406,21.2511176069915,
21.3504913345749,21.4498322512187,21.5491708007745,21.6493225000927,21.7488054777122,
21.8492915378798,21.9497775980474,22.0494733772045,22.1490261995813,22.248834769833,
22.3482084969741,22.4475494131644,22.5468879622562,22.6470396620909,22.7465226392252,
22.8470087004101,22.947494761595,23.0471905416208,23.1467433648807,23.2465519349134,
23.3459256629671,23.445266580079,23.5446051301003,23.6447568288609,23.7442398069341,
23.8447258660384,23.9452119251426,24.0449077047904,24.1444605276681,24.2442690977958,
24.3436428254591,24.4429837421786,24.5423222918056,24.6424739910267,24.7419569687061,
24.8424430286982,24.9429290886902,25.0426248683205,25.1421776911792,25.2419862613116,
25.3413599889527,25.4407009056489,25.5400394552514,25.640191154498,25.7396741321502,
25.8401601921941,25.9406462522379,26.0607488610849,26.1793890881263,26.2493612672369),
 .UNSPECIFIED.);
#488=B_SPLINE_CURVE_WITH_KNOTS('',3,(#33763,#33764,#33765,#33766,#33767,
#33768,#33769,#33770,#33771,#33772),.UNSPECIFIED.,.F.,.F.,(4,1,1,1,1,1,
1,4),(26.249361462325,26.9383634157855,27.9360805793331,28.9337977428807,
29.9315149064283,30.9292320699759,31.9269492335235,32.5325467695046),
 .UNSPECIFIED.);
#489=B_SPLINE_CURVE_WITH_KNOTS('',3,(#33774,#33775,#33776,#33777,#33778,
#33779,#33780,#33781,#33782,#33783,#33784,#33785,#33786,#33787,#33788,#33789,
#33790,#33791,#33792,#33793,#33794,#33795,#33796,#33797,#33798,#33799,#33800,
#33801,#33802,#33803,#33804,#33805,#33806,#33807,#33808,#33809,#33810,#33811,
#33812,#33813,#33814,#33815,#33816,#33817,#33818,#33819,#33820,#33821,#33822,
#33823,#33824,#33825,#33826,#33827,#33828,#33829,#33830,#33831,#33832,#33833,
#33834,#33835,#33836,#33837,#33838,#33839,#33840,#33841,#33842,#33843,#33844,
#33845,#33846,#33847,#33848,#33849,#33850,#33851,#33852,#33853,#33854,#33855,
#33856,#33857,#33858,#33859,#33860,#33861,#33862,#33863,#33864,#33865,#33866,
#33867,#33868,#33869,#33870,#33871,#33872,#33873,#33874,#33875,#33876,#33877,
#33878,#33879,#33880,#33881,#33882,#33883,#33884,#33885,#33886,#33887,#33888,
#33889,#33890,#33891,#33892,#33893,#33894,#33895,#33896,#33897,#33898,#33899,
#33900,#33901,#33902,#33903,#33904,#33905,#33906,#33907,#33908,#33909,#33910,
#33911,#33912,#33913,#33914,#33915,#33916,#33917,#33918,#33919,#33920,#33921,
#33922,#33923,#33924,#33925,#33926,#33927,#33928,#33929,#33930,#33931,#33932,
#33933,#33934,#33935,#33936,#33937,#33938,#33939,#33940,#33941,#33942,#33943,
#33944,#33945,#33946,#33947,#33948,#33949,#33950,#33951,#33952,#33953,#33954,
#33955,#33956,#33957,#33958,#33959,#33960,#33961,#33962,#33963,#33964,#33965,
#33966),.UNSPECIFIED.,.F.,.F.,(4,3,3,3,3,3,3,3,3,3,3,3,3,3,3,3,3,3,3,3,
3,3,3,3,3,3,3,3,3,3,3,3,3,3,3,3,3,3,3,3,3,3,3,3,3,3,3,3,3,3,3,3,3,3,3,3,
3,3,3,3,3,3,3,3,4),(32.5325469962121,32.6429236413342,32.7537139011972,
32.8650586993773,32.9246663970711,33.0243621767635,33.1239149996856,33.2237235698022,
33.3230972975093,33.4224382142723,33.5217767639425,33.6219284631115,33.7214114408325,
33.8218975007256,33.9223835606187,34.0220793403112,34.1216321632334,34.22144073335,
34.3208144610572,34.4201553778202,34.5194939274904,34.6196456266594,34.7191286043804,
34.8196146642734,34.9201007241663,35.019796503859,35.1193493267814,35.2191578968979,
35.3185316246053,35.4178725413685,35.517211091039,35.6173627902077,35.716845767929,
35.8173318278214,35.9178178877139,36.0175136674065,36.1170664903288,36.2168750604454,
36.3162487881527,36.4155897049157,36.514928254586,36.6150799537549,36.714562931476,
36.8150489913688,36.9155350512616,37.0152308309542,37.1147836538765,37.2145922239931,
37.3139659517004,37.4133068684635,37.5126454181339,37.6127971173027,37.7122800950239,
37.8127661549165,37.9132522148092,38.0117371315798,38.1122364996896,38.2104651268854,
38.3086346576359,38.4067769601568,38.509015739232,38.6072534265365,38.7055475932706,
38.8039800274578,38.8157320764579),.UNSPECIFIED.);
#490=B_SPLINE_CURVE_WITH_KNOTS('',3,(#33968,#33969,#33970,#33971,#33972,
#33973,#33974,#33975,#33976,#33977,#33978,#33979,#33980,#33981,#33982,#33983,
#33984,#33985,#33986,#33987,#33988,#33989,#33990,#33991,#33992,#33993,#33994,
#33995,#33996,#33997,#33998,#33999,#34000,#34001,#34002,#34003,#34004,#34005,
#34006,#34007,#34008,#34009,#34010,#34011,#34012,#34013,#34014,#34015,#34016,
#34017,#34018,#34019,#34020,#34021,#34022,#34023,#34024,#34025,#34026,#34027,
#34028,#34029,#34030,#34031,#34032,#34033,#34034,#34035,#34036,#34037,#34038,
#34039,#34040,#34041,#34042,#34043,#34044,#34045,#34046,#34047,#34048,#34049,
#34050,#34051,#34052,#34053,#34054,#34055,#34056,#34057,#34058,#34059,#34060,
#34061,#34062,#34063,#34064,#34065,#34066,#34067,#34068,#34069,#34070,#34071,
#34072,#34073,#34074,#34075,#34076,#34077,#34078,#34079,#34080,#34081,#34082,
#34083,#34084,#34085,#34086,#34087,#34088,#34089,#34090,#34091,#34092,#34093,
#34094,#34095,#34096,#34097,#34098,#34099,#34100,#34101,#34102,#34103,#34104,
#34105,#34106,#34107,#34108,#34109,#34110,#34111,#34112,#34113,#34114,#34115,
#34116,#34117,#34118,#34119,#34120,#34121,#34122,#34123,#34124,#34125,#34126,
#34127,#34128,#34129,#34130,#34131,#34132,#34133,#34134,#34135,#34136,#34137,
#34138,#34139,#34140,#34141,#34142,#34143,#34144,#34145,#34146,#34147,#34148,
#34149,#34150,#34151,#34152,#34153,#34154,#34155,#34156,#34157),
 .UNSPECIFIED.,.F.,.F.,(4,3,3,3,3,3,3,3,3,3,3,3,3,3,3,3,3,3,3,3,3,3,3,3,
3,3,3,3,3,3,3,3,3,3,3,3,3,3,3,3,3,3,3,3,3,3,3,3,3,3,3,3,3,3,3,3,3,3,3,3,
3,3,3,4),(38.8157320766842,38.9109693783568,39.0106651580491,39.1102179809711,
39.2100265510878,39.3094002787948,39.4087411955576,39.5080797452276,39.6082314443968,
39.7077144221177,39.808200482011,39.9086865419044,40.0083823215971,40.1079351445195,
40.2077437146361,40.3071174423435,40.4064583591067,40.5057969087771,40.6059486079458,
40.7054315856671,40.8059176455595,40.906403705452,41.0060994851446,41.1056523080669,
41.2054608781835,41.3048346058908,41.4041755226539,41.5035140723242,41.6036657714931,
41.7031487492143,41.8036348091069,41.9041208689996,42.0038166486922,42.1033694716144,
42.203178041731,42.3025517694383,42.4018926862013,42.5012312358716,42.6013829350405,
42.7008659127616,42.8013519726544,42.9018380325472,43.0015338122398,43.1010866351621,
43.2008952052787,43.300268932986,43.3996098497491,43.4989483994195,43.5991000985883,
43.6985830763095,43.7990691362021,43.8995551960948,43.9992509757874,44.0988037987097,
44.1986123688262,44.2979860965335,44.3973270132966,44.4966655629669,44.5968172621358,
44.6963002398569,44.7967862997496,44.8972723596424,45.0393109849315,45.0989173838638),
 .UNSPECIFIED.);
#491=B_SPLINE_CURVE_WITH_KNOTS('',3,(#34159,#34160,#34161,#34162,#34163,
#34164,#34165,#34166,#34167,#34168),.UNSPECIFIED.,.F.,.F.,(4,1,1,1,1,1,
1,4),(45.0989204148471,45.89498952319,46.8927066867377,47.8904238502853,
48.8881410138329,49.8858581773805,50.8835753409281,51.3821026672746),
 .UNSPECIFIED.);
#492=B_SPLINE_CURVE_WITH_KNOTS('',3,(#34170,#34171,#34172,#34173,#34174,
#34175,#34176,#34177,#34178,#34179,#34180,#34181,#34182,#34183,#34184,#34185,
#34186,#34187,#34188,#34189,#34190,#34191,#34192,#34193,#34194,#34195,#34196,
#34197,#34198,#34199,#34200,#34201,#34202,#34203,#34204,#34205,#34206,#34207,
#34208,#34209,#34210,#34211,#34212,#34213,#34214,#34215,#34216,#34217,#34218,
#34219,#34220,#34221,#34222,#34223,#34224,#34225,#34226,#34227,#34228,#34229,
#34230,#34231,#34232,#34233,#34234,#34235,#34236,#34237,#34238,#34239,#34240,
#34241,#34242,#34243,#34244,#34245,#34246,#34247,#34248,#34249,#34250,#34251,
#34252,#34253,#34254,#34255,#34256,#34257,#34258,#34259,#34260,#34261,#34262,
#34263,#34264,#34265,#34266,#34267,#34268,#34269,#34270,#34271,#34272,#34273,
#34274,#34275,#34276,#34277,#34278,#34279,#34280,#34281,#34282,#34283,#34284,
#34285,#34286,#34287,#34288,#34289,#34290,#34291,#34292,#34293,#34294,#34295,
#34296,#34297,#34298,#34299,#34300,#34301,#34302,#34303,#34304,#34305,#34306,
#34307,#34308,#34309,#34310,#34311,#34312,#34313,#34314,#34315,#34316,#34317,
#34318,#34319,#34320,#34321,#34322,#34323,#34324,#34325,#34326,#34327,#34328,
#34329,#34330,#34331,#34332,#34333,#34334,#34335,#34336,#34337,#34338,#34339,
#34340,#34341,#34342,#34343,#34344,#34345,#34346,#34347,#34348,#34349,#34350,
#34351,#34352,#34353,#34354,#34355,#34356,#34357,#34358,#34359),
 .UNSPECIFIED.,.F.,.F.,(4,3,3,3,3,3,3,3,3,3,3,3,3,3,3,3,3,3,3,3,3,3,3,3,
3,3,3,3,3,3,3,3,3,3,3,3,3,3,3,3,3,3,3,3,3,3,3,3,3,3,3,3,3,3,3,3,3,3,3,3,
3,3,3,4),(51.3821026910434,51.4861327815925,51.5904454853881,51.6949031312876,
51.7996461633303,51.8812925044757,51.9809882841683,52.0805411070906,52.1803496772072,
52.2797234049145,52.3790643216776,52.4784028713478,52.5785545705166,52.6780375482378,
52.7785236081306,52.8790096680233,52.9787054477158,53.0782582706381,53.1780668407547,
53.2774405684621,53.3767814852251,53.4761200348954,53.5762717340643,53.6757547117854,
53.7762407716782,53.8767268315709,53.9764226112636,54.075975434186,54.1757840043025,
54.2751577320098,54.3744986487728,54.4738371984431,54.573988897612,54.6734718753331,
54.7739579352258,54.8744439951185,54.9741397748111,55.0736925977335,55.1735011678501,
55.2728748955575,55.3722158123206,55.4715543619908,55.5717060611596,55.6711890388808,
55.7716750987734,55.8721611586661,55.9718569383586,56.0714097612811,56.1712183313977,
56.270592059105,56.369932975868,56.4692715255384,56.5694232247072,56.6689062024283,
56.7693922623211,56.8698783222138,56.9693045316758,57.067409750273,57.1654215585788,
57.2633721047655,57.3638510780515,57.4618119537227,57.5635499758161,57.6652879979096),
 .UNSPECIFIED.);
#493=B_SPLINE_CURVE_WITH_KNOTS('',3,(#34361,#34362,#34363,#34364,#34365,
#34366,#34367,#34368,#34369,#34370,#34371,#34372,#34373,#34374,#34375,#34376,
#34377,#34378,#34379,#34380,#34381,#34382,#34383,#34384,#34385,#34386,#34387,
#34388,#34389,#34390,#34391,#34392,#34393,#34394,#34395,#34396,#34397,#34398,
#34399,#34400,#34401,#34402,#34403,#34404,#34405,#34406,#34407,#34408,#34409,
#34410,#34411,#34412,#34413,#34414,#34415,#34416,#34417,#34418,#34419,#34420,
#34421,#34422,#34423,#34424,#34425,#34426,#34427,#34428,#34429,#34430,#34431,
#34432,#34433,#34434,#34435,#34436,#34437,#34438,#34439,#34440,#34441,#34442,
#34443,#34444,#34445,#34446,#34447,#34448,#34449,#34450,#34451,#34452,#34453,
#34454,#34455,#34456,#34457,#34458,#34459,#34460,#34461,#34462,#34463,#34464,
#34465,#34466,#34467,#34468,#34469,#34470,#34471,#34472,#34473,#34474,#34475,
#34476,#34477,#34478,#34479,#34480,#34481,#34482,#34483,#34484,#34485,#34486,
#34487,#34488,#34489,#34490,#34491,#34492,#34493,#34494,#34495,#34496,#34497,
#34498,#34499,#34500,#34501,#34502,#34503,#34504,#34505,#34506,#34507,#34508,
#34509,#34510,#34511,#34512,#34513,#34514,#34515,#34516,#34517,#34518,#34519,
#34520,#34521,#34522,#34523,#34524,#34525,#34526,#34527,#34528,#34529,#34530,
#34531,#34532,#34533,#34534,#34535,#34536,#34537,#34538,#34539,#34540,#34541,
#34542,#34543,#34544,#34545,#34546,#34547,#34548,#34549,#34550),
 .UNSPECIFIED.,.F.,.F.,(4,3,3,3,3,3,3,3,3,3,3,3,3,3,3,3,3,3,3,3,3,3,3,3,
3,3,3,3,3,3,3,3,3,3,3,3,3,3,3,3,3,3,3,3,3,3,3,3,3,3,3,3,3,3,3,3,3,3,3,3,
3,3,3,4),(57.665287998223,57.8070952114157,57.8675954857614,57.967291265454,
58.0668440883763,58.1666526584929,58.2660263862001,58.3653673029632,58.4647058526337,
58.5648575518025,58.6643405295236,58.7648265894163,58.865312649309,58.9650084290015,
59.0645612519237,59.1643698220403,59.2637435497476,59.3630844665106,59.4624230161809,
59.5625747153498,59.6620576930709,59.7625437529638,59.8630298128566,59.9627255925492,
60.0622784154715,60.162086985588,60.2614607132954,60.3608016300585,60.4601401797288,
60.5602918788976,60.6597748566188,60.7602609165115,60.8607469764042,60.9604427560968,
61.0599955790191,61.1598041491357,61.259177876843,61.3585187936061,61.4578573432764,
61.5580090424452,61.6574920201664,61.7579780800591,61.8584641399518,61.9581599196445,
62.0577127425668,62.1575213126834,62.2568950403907,62.3562359571538,62.4555745068242,
62.555726205993,62.6552091837141,62.7556952436068,62.8561813034994,62.955877083192,
63.0554299061143,63.1552384762309,63.2546122039382,63.3539531207012,63.4532916703714,
63.5534433695403,63.6529263472615,63.7534124071542,63.853898467047,63.9484733054025),
 .UNSPECIFIED.);
#494=B_SPLINE_CURVE_WITH_KNOTS('',3,(#34552,#34553,#34554,#34555,#34556,
#34557,#34558,#34559,#34560,#34561,#34562,#34563,#34564,#34565,#34566,#34567,
#34568,#34569,#34570,#34571,#34572,#34573,#34574,#34575,#34576,#34577,#34578,
#34579,#34580,#34581,#34582,#34583,#34584,#34585,#34586,#34587,#34588,#34589,
#34590,#34591,#34592,#34593,#34594,#34595,#34596,#34597,#34598,#34599,#34600,
#34601,#34602,#34603,#34604,#34605,#34606,#34607,#34608,#34609,#34610,#34611,
#34612,#34613,#34614,#34615,#34616,#34617,#34618,#34619,#34620,#34621,#34622,
#34623,#34624,#34625,#34626,#34627,#34628,#34629,#34630,#34631,#34632,#34633,
#34634,#34635,#34636,#34637,#34638,#34639,#34640,#34641,#34642,#34643,#34644,
#34645,#34646,#34647,#34648,#34649,#34650,#34651,#34652,#34653,#34654,#34655,
#34656,#34657,#34658,#34659,#34660,#34661,#34662,#34663,#34664,#34665,#34666,
#34667,#34668,#34669,#34670,#34671,#34672,#34673,#34674,#34675,#34676,#34677,
#34678,#34679,#34680,#34681,#34682,#34683,#34684,#34685,#34686,#34687,#34688,
#34689,#34690,#34691,#34692,#34693,#34694,#34695,#34696,#34697,#34698,#34699,
#34700,#34701,#34702,#34703,#34704,#34705,#34706,#34707,#34708,#34709,#34710,
#34711,#34712,#34713,#34714,#34715,#34716,#34717,#34718,#34719,#34720,#34721,
#34722,#34723,#34724,#34725,#34726,#34727,#34728,#34729,#34730,#34731,#34732,
#34733,#34734,#34735,#34736,#34737,#34738,#34739,#34740,#34741,#34742,#34743,
#34744),.UNSPECIFIED.,.F.,.F.,(4,3,3,3,3,3,3,3,3,3,3,3,3,3,3,3,3,3,3,3,
3,3,3,3,3,3,3,3,3,3,3,3,3,3,3,3,3,3,3,3,3,3,3,3,3,3,3,3,3,3,3,3,3,3,3,3,
3,3,3,3,3,3,3,3,4),(63.9484733056258,64.0469101210583,64.1474983097503,
64.2457098131483,64.3438737786661,64.4420220526341,64.5444204471243,64.6426930224998,
64.7410320253817,64.8395232369876,64.8516156305946,64.9513114102871,65.0508642332093,
65.1506728033259,65.2500465310332,65.3493874477962,65.4487259974665,65.5488776966354,
65.6483606743565,65.7488467342494,65.8493327941422,65.9490285738348,66.0485813967571,
66.1483899668737,66.247763694581,66.347104611344,66.4464431610144,66.5465948601833,
66.6460778379043,66.746563897797,66.8470499576898,66.9467457373824,67.0462985603045,
67.1461071304212,67.2454808581284,67.3448217748916,67.4441603245621,67.5443120237309,
67.6437950014522,67.7442810613448,67.8447671212375,67.9444629009302,68.0440157238524,
68.143824293969,68.2431980216763,68.3425389384395,68.4418774881096,68.5420291872785,
68.6415121649996,68.7419982248924,68.8424842847851,68.9421800644777,69.0417328874002,
69.1415414575167,69.240915185224,69.3402561019872,69.4395946516573,69.5397463508262,
69.6392293285473,69.73971538844,69.8402014483327,69.9515510975534,70.062533144783,
70.1728865793843,70.2316583852461),.UNSPECIFIED.);
#495=B_SPLINE_CURVE_WITH_KNOTS('',3,(#34746,#34747,#34748,#34749,#34750,
#34751,#34752,#34753,#34754,#34755),.UNSPECIFIED.,.F.,.F.,(4,1,1,1,1,1,
1,4),(70.2316586125821,70.8379186118803,71.8356357754279,72.8333529389755,
73.8310701025231,74.8287872660707,75.8265044296183,76.5148439197617),
 .UNSPECIFIED.);
#496=B_SPLINE_CURVE_WITH_KNOTS('',3,(#34757,#34758,#34759,#34760,#34761,
#34762,#34763,#34764,#34765,#34766,#34767,#34768,#34769,#34770,#34771,#34772,
#34773,#34774,#34775,#34776,#34777,#34778,#34779,#34780,#34781,#34782,#34783,
#34784,#34785,#34786,#34787,#34788,#34789,#34790,#34791,#34792,#34793,#34794,
#34795,#34796,#34797,#34798,#34799,#34800,#34801,#34802,#34803,#34804,#34805,
#34806,#34807,#34808,#34809,#34810,#34811,#34812,#34813,#34814,#34815,#34816,
#34817,#34818,#34819,#34820,#34821,#34822,#34823,#34824,#34825,#34826,#34827,
#34828,#34829,#34830,#34831,#34832,#34833,#34834,#34835,#34836,#34837,#34838,
#34839,#34840,#34841,#34842,#34843,#34844,#34845,#34846,#34847,#34848,#34849,
#34850,#34851,#34852,#34853,#34854,#34855,#34856,#34857,#34858,#34859,#34860,
#34861,#34862,#34863,#34864,#34865,#34866,#34867,#34868,#34869,#34870,#34871,
#34872,#34873,#34874,#34875,#34876,#34877,#34878,#34879,#34880,#34881,#34882,
#34883,#34884,#34885,#34886,#34887,#34888,#34889,#34890,#34891,#34892,#34893,
#34894,#34895,#34896,#34897,#34898,#34899,#34900,#34901,#34902,#34903,#34904,
#34905,#34906,#34907,#34908,#34909,#34910,#34911,#34912,#34913,#34914,#34915,
#34916,#34917,#34918,#34919,#34920,#34921,#34922,#34923,#34924,#34925,#34926,
#34927,#34928,#34929,#34930,#34931,#34932,#34933,#34934,#34935,#34936,#34937,
#34938,#34939,#34940,#34941,#34942,#34943,#34944,#34945,#34946),
 .UNSPECIFIED.,.F.,.F.,(4,3,3,3,3,3,3,3,3,3,3,3,3,3,3,3,3,3,3,3,3,3,3,3,
3,3,3,3,3,3,3,3,3,3,3,3,3,3,3,3,3,3,3,3,3,3,3,3,3,3,3,3,3,3,3,3,3,3,3,3,
3,3,3,4),(76.5148441159767,76.6331916616517,76.7530359215634,76.824221593166,
76.9239173728584,77.0234701957806,77.1232787658972,77.2226524936043,77.3219934103671,
77.4213319600372,77.5214836592063,77.6209666369272,77.7214526968204,77.8219387567136,
77.9216345364062,78.0211873593286,78.1209959294452,78.2203696571526,78.3197105739157,
78.4190491235861,78.5192008227549,78.6186838004761,78.7191698603686,78.8196559202612,
78.9193516999539,79.0189045228762,79.1187130929927,79.2180868207001,79.3174277374632,
79.4167662871335,79.5169179863023,79.6164009640235,79.7168870239162,79.8173730838088,
79.9170688635014,80.0166216864236,80.1164302565402,80.2158039842475,80.3151449010106,
80.4144834506808,80.5146351498497,80.6141181275708,80.7146041874636,80.8150902473564,
80.914786027049,81.0143388499712,81.1141474200878,81.2135211477951,81.3128620645582,
81.4122006142286,81.5123523133974,81.6118352911185,81.7123213510113,81.812807410904,
81.9122859939485,82.0116217850278,82.1108427790342,82.2100011139379,82.3091275647997,
82.4082528670978,82.5074761530274,82.6067470602028,82.7061961999099,82.7980292265394),
 .UNSPECIFIED.);
#497=B_SPLINE_CURVE_WITH_KNOTS('',3,(#34948,#34949,#34950,#34951,#34952,
#34953,#34954,#34955,#34956,#34957,#34958,#34959,#34960,#34961,#34962,#34963,
#34964,#34965,#34966,#34967,#34968,#34969,#34970,#34971,#34972,#34973,#34974,
#34975,#34976,#34977,#34978,#34979,#34980,#34981,#34982,#34983,#34984,#34985,
#34986,#34987,#34988,#34989,#34990,#34991,#34992,#34993,#34994,#34995,#34996,
#34997,#34998,#34999,#35000,#35001,#35002,#35003,#35004,#35005,#35006,#35007,
#35008,#35009,#35010,#35011,#35012,#35013,#35014,#35015,#35016,#35017,#35018,
#35019,#35020,#35021,#35022,#35023,#35024,#35025,#35026,#35027,#35028,#35029,
#35030,#35031,#35032,#35033,#35034,#35035,#35036,#35037,#35038,#35039,#35040,
#35041,#35042,#35043,#35044,#35045,#35046,#35047,#35048,#35049,#35050,#35051,
#35052,#35053,#35054,#35055,#35056,#35057,#35058,#35059,#35060,#35061,#35062,
#35063,#35064,#35065,#35066,#35067,#35068,#35069,#35070,#35071,#35072,#35073,
#35074,#35075,#35076,#35077,#35078,#35079,#35080,#35081,#35082,#35083,#35084,
#35085,#35086,#35087,#35088,#35089,#35090,#35091,#35092,#35093,#35094,#35095,
#35096,#35097,#35098,#35099,#35100,#35101,#35102,#35103,#35104,#35105,#35106,
#35107,#35108,#35109,#35110,#35111,#35112,#35113,#35114,#35115,#35116,#35117,
#35118,#35119,#35120,#35121,#35122,#35123,#35124,#35125,#35126,#35127,#35128,
#35129,#35130,#35131,#35132,#35133,#35134,#35135,#35136,#35137,#35138,#35139,
#35140),.UNSPECIFIED.,.F.,.F.,(4,3,3,3,3,3,3,3,3,3,3,3,3,3,3,3,3,3,3,3,
3,3,3,3,3,3,3,3,3,3,3,3,3,3,3,3,3,3,3,3,3,3,3,3,3,3,3,3,3,3,3,3,3,3,3,3,
3,3,3,3,3,3,3,3,4),(82.7980292269413,82.8105245744516,82.9102203541442,
83.0097731770666,83.1095817471832,83.2089554748905,83.3082963916536,83.407634941324,
83.5077866404928,83.6072696182139,83.7077556781066,83.8082417379992,83.9079375176917,
84.007490340614,84.1072989107306,84.2066726384379,84.3060135552009,84.4053521048711,
84.50550380404,84.6049867817612,84.705472841654,84.8059589015468,84.9056546812395,
85.0052075041618,85.1050160742784,85.2043898019857,85.3037307187489,85.4030692684192,
85.5032209675881,85.6027039453093,85.7031900052019,85.8036760650945,85.9033718447871,
86.0029246677094,86.102733237826,86.2021069655333,86.3014478822963,86.4007864319666,
86.5009381311355,86.6004211088566,86.7009071687494,86.8013932286421,86.9010890083347,
87.000641831257,87.1004504013736,87.1998241290809,87.299165045844,87.3985035955144,
87.4986552946832,87.5981382724043,87.698624332297,87.7991103921897,87.8988061718823,
87.9983589948046,88.0981675649212,88.1975412926285,88.2968822093916,88.3962207590619,
88.4963724582308,88.5958554359519,88.6963414958446,88.7968275557373,88.9205993160034,
89.0424478486719,89.0812145338453),.UNSPECIFIED.);
#498=B_SPLINE_CURVE_WITH_KNOTS('',3,(#35142,#35143,#35144,#35145,#35146,
#35147,#35148,#35149,#35150,#35151,#35152,#35153,#35154,#35155,#35156,#35157,
#35158,#35159,#35160,#35161,#35162,#35163,#35164,#35165,#35166,#35167,#35168,
#35169,#35170,#35171,#35172,#35173,#35174,#35175,#35176,#35177,#35178,#35179,
#35180,#35181,#35182,#35183,#35184,#35185,#35186,#35187,#35188,#35189,#35190,
#35191,#35192,#35193,#35194,#35195,#35196,#35197,#35198,#35199,#35200,#35201,
#35202,#35203,#35204,#35205,#35206,#35207,#35208,#35209,#35210,#35211,#35212,
#35213,#35214,#35215,#35216,#35217,#35218,#35219,#35220,#35221,#35222,#35223,
#35224,#35225,#35226,#35227,#35228,#35229,#35230,#35231,#35232,#35233,#35234,
#35235,#35236,#35237,#35238,#35239,#35240,#35241,#35242,#35243,#35244,#35245,
#35246,#35247,#35248,#35249,#35250,#35251,#35252,#35253,#35254,#35255,#35256,
#35257,#35258,#35259,#35260,#35261,#35262,#35263,#35264,#35265,#35266,#35267,
#35268,#35269,#35270,#35271,#35272,#35273,#35274,#35275,#35276,#35277,#35278,
#35279,#35280,#35281,#35282,#35283,#35284,#35285,#35286,#35287,#35288,#35289,
#35290,#35291,#35292,#35293,#35294,#35295,#35296,#35297,#35298,#35299,#35300,
#35301,#35302,#35303,#35304,#35305,#35306,#35307,#35308,#35309,#35310,#35311,
#35312,#35313,#35314,#35315,#35316,#35317,#35318,#35319,#35320,#35321,#35322,
#35323,#35324,#35325,#35326,#35327,#35328,#35329,#35330,#35331,#35332,#35333,
#35334),.UNSPECIFIED.,.F.,.F.,(4,3,3,3,3,3,3,3,3,3,3,3,3,3,3,3,3,3,3,3,
3,3,3,3,3,3,3,3,3,3,3,3,3,3,3,3,3,3,3,3,3,3,3,3,3,3,3,3,3,3,3,3,3,3,3,3,
3,3,3,3,3,3,3,3,4),(89.0812145341209,89.1798277015848,89.2783970373168,
89.3769539358606,89.4755297704361,89.5742162318756,89.6729694918042,89.7718816291792,
89.7945447192849,89.8942404989775,89.9937933218998,90.0936018920164,90.1929756197236,
90.2923165364868,90.3916550861572,90.491806785326,90.5912897630471,90.6917758229398,
90.7922618828325,90.8919576625251,90.9915104854473,91.0913190555639,91.1906927832712,
91.2900337000343,91.3893722497046,91.4895239488735,91.5890069265947,91.6894929864874,
91.7899790463801,91.8896748260726,91.9892276489952,92.0890362191118,92.1884099468192,
92.2877508635822,92.3870894132525,92.4872411124213,92.5867240901425,92.6872101500351,
92.7876962099277,92.8873919896202,92.9869448125427,93.0867533826593,93.1861271103666,
93.2854680271297,93.3848065767998,93.4849582759687,93.5844412536898,93.6849273135825,
93.7854133734753,93.8851091531678,93.9846619760905,94.0844705462071,94.1838442739143,
94.2831851906773,94.3825237403476,94.4826754395165,94.5821584172377,94.6826444771303,
94.7831305370229,94.8847948887262,94.9862963274486,95.0876311352717,95.1888678692207,
95.2900278217262,95.3643998413005),.UNSPECIFIED.);
#499=B_SPLINE_CURVE_WITH_KNOTS('',3,(#35336,#35337,#35338,#35339,#35340,
#35341,#35342,#35343,#35344,#35345,#35346,#35347,#35348,#35349,#35350,#35351,
#35352,#35353,#35354,#35355,#35356,#35357,#35358,#35359,#35360,#35361,#35362,
#35363,#35364,#35365,#35366,#35367,#35368,#35369,#35370,#35371,#35372,#35373,
#35374,#35375,#35376,#35377,#35378,#35379,#35380,#35381,#35382,#35383,#35384,
#35385,#35386,#35387,#35388,#35389,#35390,#35391,#35392,#35393,#35394,#35395,
#35396,#35397,#35398,#35399,#35400,#35401,#35402,#35403,#35404,#35405,#35406,
#35407,#35408,#35409,#35410,#35411,#35412,#35413,#35414,#35415,#35416,#35417,
#35418,#35419,#35420,#35421,#35422,#35423,#35424,#35425,#35426,#35427,#35428,
#35429,#35430,#35431,#35432,#35433,#35434,#35435,#35436,#35437,#35438,#35439,
#35440,#35441,#35442,#35443,#35444,#35445,#35446,#35447,#35448,#35449,#35450,
#35451,#35452,#35453,#35454,#35455,#35456,#35457,#35458,#35459,#35460,#35461,
#35462,#35463,#35464,#35465,#35466,#35467,#35468,#35469,#35470,#35471,#35472,
#35473,#35474,#35475,#35476,#35477,#35478,#35479,#35480,#35481,#35482,#35483,
#35484,#35485,#35486,#35487,#35488,#35489,#35490,#35491,#35492,#35493,#35494,
#35495,#35496,#35497,#35498,#35499,#35500,#35501,#35502,#35503,#35504,#35505,
#35506,#35507,#35508,#35509,#35510,#35511,#35512,#35513,#35514,#35515,#35516,
#35517,#35518,#35519,#35520,#35521,#35522,#35523,#35524,#35525),
 .UNSPECIFIED.,.F.,.F.,(4,3,3,3,3,3,3,3,3,3,3,3,3,3,3,3,3,3,3,3,3,3,3,3,
3,3,3,3,3,3,3,3,3,3,3,3,3,3,3,3,3,3,3,3,3,3,3,3,3,3,3,3,3,3,3,3,3,3,3,3,
3,3,3,4),(95.3643998416745,95.4730572664134,95.5820351393695,95.6915015544521,
95.7808477005705,95.880543480263,95.9800963031853,96.0799048733019,96.1792786010091,
96.2786195177721,96.3779580674424,96.4781097666113,96.5775927443324,96.6780788042252,
96.7785648641181,96.8782606438108,96.9778134667331,97.0776220368497,97.1769957645571,
97.2763366813202,97.3756752309906,97.4758269301594,97.5753099078806,97.6757959677732,
97.7762820276658,97.8759778073584,97.9755306302807,98.0753392003973,98.1747129281046,
98.2740538448677,98.373392394538,98.4735440937068,98.573027071428,98.6735131313206,
98.7739991912133,98.8736949709058,98.9732477938281,99.0730563639447,99.1724300916519,
99.2717710084149,99.3711095580852,99.4712612572542,99.5707442349753,99.6712302948681,
99.771716354761,99.8714121344538,99.9709649573763,100.070773527493,100.1701472552,
100.269488171964,100.368826721634,100.468978420803,100.568461398524,100.668947458417,
100.769433518309,100.867766132118,100.965935563168,101.064013280475,101.162031368816,
101.260021836025,101.358073520992,101.456152065062,101.554380441358,101.64758514848),
 .UNSPECIFIED.);
#500=B_SPLINE_CURVE_WITH_KNOTS('',3,(#35527,#35528,#35529,#35530,#35531,
#35532,#35533,#35534,#35535,#35536,#35537),.UNSPECIFIED.,.F.,.F.,(4,1,1,
1,1,1,1,1,4),(101.64758514848,101.767150681856,102.764867845404,103.762585008951,
104.760302172499,105.758019336047,106.755736499594,107.753453663142,107.93077045566),
 .UNSPECIFIED.);
#501=B_SPLINE_CURVE_WITH_KNOTS('',3,(#35539,#35540,#35541,#35542,#35543,
#35544,#35545,#35546,#35547,#35548,#35549,#35550,#35551,#35552,#35553,#35554,
#35555,#35556,#35557,#35558,#35559,#35560,#35561,#35562,#35563,#35564,#35565,
#35566,#35567,#35568,#35569,#35570,#35571,#35572,#35573,#35574,#35575,#35576,
#35577,#35578,#35579,#35580,#35581,#35582,#35583,#35584,#35585,#35586,#35587,
#35588,#35589,#35590,#35591,#35592,#35593,#35594,#35595,#35596,#35597,#35598,
#35599,#35600,#35601,#35602,#35603,#35604,#35605,#35606,#35607,#35608,#35609,
#35610,#35611,#35612,#35613,#35614,#35615,#35616,#35617,#35618,#35619,#35620,
#35621,#35622,#35623,#35624,#35625,#35626,#35627,#35628,#35629,#35630,#35631,
#35632,#35633,#35634,#35635,#35636,#35637,#35638,#35639,#35640,#35641,#35642,
#35643,#35644,#35645,#35646,#35647,#35648,#35649,#35650,#35651,#35652,#35653,
#35654,#35655,#35656,#35657,#35658,#35659,#35660,#35661,#35662,#35663,#35664,
#35665,#35666,#35667,#35668,#35669,#35670,#35671,#35672,#35673,#35674,#35675,
#35676,#35677,#35678,#35679,#35680,#35681,#35682,#35683,#35684,#35685,#35686,
#35687,#35688,#35689,#35690,#35691,#35692,#35693,#35694,#35695,#35696,#35697,
#35698,#35699,#35700,#35701,#35702,#35703,#35704,#35705,#35706,#35707,#35708,
#35709,#35710,#35711,#35712,#35713,#35714,#35715,#35716,#35717,#35718,#35719,
#35720,#35721,#35722,#35723,#35724,#35725,#35726,#35727,#35728,#35729,#35730,
#35731),.UNSPECIFIED.,.F.,.F.,(4,3,3,3,3,3,3,3,3,3,3,3,3,3,3,3,3,3,3,3,
3,3,3,3,3,3,3,3,3,3,3,3,3,3,3,3,3,3,3,3,3,3,3,3,3,3,3,3,3,3,3,3,3,3,3,3,
3,3,3,3,3,3,3,3,4),(107.93077045566,108.033320502039,108.131274959939,108.229174356975,
108.327050797025,108.424936350185,108.522922660142,108.620968324305,108.719170328587,
108.751170826689,108.850866606382,108.950419429304,109.050227999421,109.149601727128,
109.248942643891,109.348281193561,109.44843289273,109.547915870452,109.648401930344,
109.748887990237,109.84858376993,109.948136592852,110.047945162969,110.147318890677,
110.24665980744,110.34599835711,110.446150056279,110.545633034001,110.646119093893,
110.746605153785,110.846300933477,110.945853756399,111.045662326516,111.145036054223,
111.244376970986,111.343715520656,111.443867219825,111.543350197546,111.643836257439,
111.744322317332,111.844018097025,111.943570919947,112.043379490064,112.142753217771,
112.242094134534,112.341432684205,112.441584383373,112.541067361094,112.641553420987,
112.74203948088,112.841735260573,112.941288083496,113.041096653612,113.14047038132,
113.239811298083,113.339149847754,113.439301546922,113.538784524644,113.639270584536,
113.739756644428,113.845800654927,113.951510358964,114.057014148429,114.162240196533,
114.213955762579),.UNSPECIFIED.);
#502=B_SPLINE_CURVE_WITH_KNOTS('',3,(#35733,#35734,#35735,#35736,#35737,
#35738,#35739,#35740,#35741,#35742,#35743,#35744,#35745,#35746,#35747,#35748,
#35749,#35750,#35751,#35752,#35753,#35754,#35755,#35756,#35757,#35758,#35759,
#35760,#35761,#35762,#35763,#35764,#35765,#35766,#35767,#35768,#35769,#35770,
#35771,#35772,#35773,#35774,#35775,#35776,#35777,#35778,#35779,#35780,#35781,
#35782,#35783,#35784,#35785,#35786,#35787,#35788,#35789,#35790,#35791,#35792,
#35793,#35794,#35795,#35796,#35797,#35798,#35799,#35800,#35801,#35802,#35803,
#35804,#35805,#35806,#35807,#35808,#35809,#35810,#35811,#35812,#35813,#35814,
#35815,#35816,#35817,#35818,#35819,#35820,#35821,#35822,#35823,#35824,#35825,
#35826,#35827,#35828,#35829,#35830,#35831,#35832,#35833,#35834,#35835,#35836,
#35837,#35838,#35839,#35840,#35841,#35842,#35843,#35844,#35845,#35846,#35847,
#35848,#35849,#35850,#35851,#35852,#35853,#35854,#35855,#35856,#35857,#35858,
#35859,#35860,#35861,#35862,#35863,#35864,#35865,#35866,#35867,#35868,#35869,
#35870,#35871,#35872,#35873,#35874,#35875,#35876,#35877,#35878,#35879,#35880,
#35881,#35882,#35883,#35884,#35885,#35886,#35887,#35888,#35889,#35890,#35891,
#35892,#35893,#35894,#35895,#35896,#35897,#35898,#35899,#35900,#35901,#35902,
#35903,#35904,#35905,#35906,#35907,#35908,#35909,#35910,#35911,#35912,#35913,
#35914,#35915,#35916,#35917,#35918,#35919,#35920,#35921,#35922),
 .UNSPECIFIED.,.F.,.F.,(4,3,3,3,3,3,3,3,3,3,3,3,3,3,3,3,3,3,3,3,3,3,3,3,
3,3,3,3,3,3,3,3,3,3,3,3,3,3,3,3,3,3,3,3,3,3,3,3,3,3,3,3,3,3,3,3,3,3,3,3,
3,3,3,4),(114.213955762839,114.317000725158,114.422118995862,114.525515211232,
114.631494509603,114.737473807975,114.837169587668,114.93672241059,115.036530980707,
115.135904708414,115.235245625178,115.334584174848,115.434735874017,115.534218851738,
115.634704911631,115.735190971523,115.834886751215,115.934439574137,116.034248144254,
116.133621871961,116.232962788724,116.332301338394,116.432453037563,116.531936015284,
116.632422075177,116.73290813507,116.832603914763,116.932156737685,117.031965307801,
117.131339035509,117.230679952272,117.330018501942,117.430170201111,117.529653178832,
117.630139238725,117.730625298618,117.830321078311,117.929873901234,118.02968247135,
118.129056199058,118.228397115822,118.327735665493,118.427887364661,118.527370342383,
118.627856402274,118.728342462166,118.828038241858,118.92759106478,119.027399634897,
119.126773362604,119.226114279367,119.325452829037,119.425604528206,119.525087505926,
119.62557356582,119.726059625713,119.824409942825,119.922632846727,120.020760508367,
120.118824976187,120.216892947049,120.314957356844,120.413115312058,120.497141070019),
 .UNSPECIFIED.);
#503=B_SPLINE_CURVE_WITH_KNOTS('',3,(#35924,#35925,#35926,#35927,#35928,
#35929,#35930,#35931,#35932,#35933,#35934),.UNSPECIFIED.,.F.,.F.,(4,1,1,
1,1,1,1,1,4),(120.497141070019,120.723776789261,121.721493952808,122.719211116356,
123.716928279904,124.714645443451,125.712362606999,126.710079770546,126.780326377198),
 .UNSPECIFIED.);
#504=B_SPLINE_CURVE_WITH_KNOTS('',3,(#35936,#35937,#35938,#35939,#35940,
#35941,#35942,#35943,#35944,#35945,#35946,#35947,#35948,#35949,#35950,#35951,
#35952,#35953,#35954,#35955,#35956,#35957,#35958,#35959,#35960,#35961,#35962,
#35963,#35964,#35965,#35966,#35967,#35968,#35969,#35970,#35971,#35972,#35973,
#35974,#35975,#35976,#35977,#35978,#35979,#35980,#35981,#35982,#35983,#35984,
#35985,#35986,#35987,#35988,#35989,#35990,#35991,#35992,#35993,#35994,#35995,
#35996,#35997,#35998,#35999,#36000,#36001,#36002,#36003,#36004,#36005,#36006,
#36007,#36008,#36009,#36010,#36011,#36012,#36013,#36014,#36015,#36016,#36017,
#36018,#36019,#36020,#36021,#36022,#36023,#36024,#36025,#36026,#36027,#36028,
#36029,#36030,#36031,#36032,#36033,#36034,#36035,#36036,#36037,#36038,#36039,
#36040,#36041,#36042,#36043,#36044,#36045,#36046,#36047,#36048,#36049,#36050,
#36051,#36052,#36053,#36054,#36055,#36056,#36057,#36058,#36059,#36060,#36061,
#36062,#36063,#36064,#36065,#36066,#36067,#36068,#36069,#36070,#36071,#36072,
#36073,#36074,#36075,#36076,#36077,#36078,#36079,#36080,#36081,#36082,#36083,
#36084,#36085,#36086,#36087,#36088,#36089,#36090,#36091,#36092,#36093,#36094,
#36095,#36096,#36097,#36098,#36099,#36100,#36101,#36102,#36103,#36104,#36105,
#36106,#36107,#36108,#36109,#36110,#36111,#36112,#36113,#36114,#36115,#36116,
#36117,#36118,#36119,#36120,#36121,#36122,#36123,#36124,#36125,#36126,#36127,
#36128),.UNSPECIFIED.,.F.,.F.,(4,3,3,3,3,3,3,3,3,3,3,3,3,3,3,3,3,3,3,3,
3,3,3,3,3,3,3,3,3,3,3,3,3,3,3,3,3,3,3,3,3,3,3,3,3,3,3,3,3,3,3,3,3,3,3,3,
3,3,3,3,3,3,3,3,4),(126.780326377198,126.879001192006,126.982600659767,
127.08103492238,127.179417182261,127.277779082583,127.376152236855,127.474629094606,
127.57316636921,127.671863081557,127.707796934094,127.807492713718,127.907045536571,
128.006854106705,128.106227834345,128.20556875104,128.304907300644,128.405058999893,
128.50454197755,128.605028037596,128.705514097642,128.805209877294,128.904762700175,
129.004571270302,129.103944997966,129.203285914686,129.302624464312,129.402776163531,
129.502259141207,129.602745201198,129.703231261189,129.802927041231,129.902479864504,
130.002288434533,130.101662162591,130.201003079704,130.300341629723,130.400493328476,
130.499976306539,130.600462365638,130.700948424737,130.800644203842,130.900197026178,
131.000005596442,131.09937932357,131.198720239757,131.298058788856,131.398210488714,
131.497693465881,131.598179527083,131.698665588285,131.798361367887,131.897914190712,
131.997722760852,132.097096488448,132.196437405094,132.295775954643,132.39592765394,
132.495410631529,132.595896691681,132.696382751832,132.809856982766,132.922875421434,
133.035120909341,133.063511684147),.UNSPECIFIED.);
#505=B_SPLINE_CURVE_WITH_KNOTS('',3,(#36130,#36131,#36132,#36133,#36134,
#36135,#36136,#36137,#36138,#36139,#36140,#36141,#36142,#36143,#36144,#36145,
#36146,#36147,#36148,#36149,#36150,#36151,#36152,#36153,#36154,#36155,#36156,
#36157,#36158,#36159,#36160,#36161,#36162,#36163,#36164,#36165,#36166,#36167,
#36168,#36169,#36170,#36171,#36172,#36173,#36174,#36175,#36176,#36177,#36178,
#36179,#36180,#36181,#36182,#36183,#36184,#36185,#36186,#36187,#36188,#36189,
#36190,#36191,#36192,#36193,#36194,#36195,#36196,#36197,#36198,#36199,#36200,
#36201,#36202,#36203,#36204,#36205,#36206,#36207,#36208,#36209,#36210,#36211,
#36212,#36213,#36214,#36215,#36216,#36217,#36218,#36219,#36220,#36221,#36222,
#36223,#36224,#36225,#36226,#36227,#36228,#36229,#36230,#36231,#36232,#36233,
#36234,#36235,#36236,#36237,#36238,#36239,#36240,#36241,#36242,#36243,#36244,
#36245,#36246,#36247,#36248,#36249,#36250,#36251,#36252,#36253,#36254,#36255,
#36256,#36257,#36258,#36259,#36260,#36261,#36262,#36263,#36264,#36265,#36266,
#36267,#36268,#36269,#36270,#36271,#36272,#36273,#36274,#36275,#36276,#36277,
#36278,#36279,#36280,#36281,#36282,#36283,#36284,#36285,#36286,#36287,#36288,
#36289,#36290,#36291,#36292,#36293,#36294,#36295,#36296,#36297,#36298,#36299,
#36300,#36301,#36302,#36303,#36304,#36305,#36306,#36307,#36308,#36309,#36310,
#36311,#36312,#36313,#36314,#36315,#36316,#36317,#36318,#36319,#36320,#36321,
#36322),.UNSPECIFIED.,.F.,.F.,(4,3,3,3,3,3,3,3,3,3,3,3,3,3,3,3,3,3,3,3,
3,3,3,3,3,3,3,3,3,3,3,3,3,3,3,3,3,3,3,3,3,3,3,3,3,3,3,3,3,3,3,3,3,3,3,3,
3,3,3,3,3,3,3,3,4),(133.063511684378,133.163441927701,133.263379444908,
133.363353474979,133.463460668199,133.563646061882,133.664007338062,133.69409991538,
133.793795690245,133.893348508343,133.993157079666,134.092530802596,134.191871714609,
134.291210259562,134.391361964404,134.490844937539,134.591331008233,134.691817078927,
134.791512859528,134.891065683314,134.990874253209,135.090247981665,135.189588899133,
135.288927449464,135.389079147717,135.488562125982,135.589048184229,135.689534242475,
135.789230038708,135.888782878248,135.98859144422,136.087965188613,136.18730612205,
136.28664468836,136.386796367776,136.486279361883,136.586765383953,136.687251406023,
136.786947147162,136.886499931537,136.986308511291,137.085682200745,137.185023079448,
137.284361591303,137.38451333587,137.483996276754,137.584482423162,137.68496856957,
137.784664367767,137.884217208881,137.98402577441,138.083399519428,138.182740453135,
138.282079019362,138.382230697801,138.481713690971,138.582199712044,138.682685733118,
138.782337641651,138.881849707232,138.981252599569,139.080581051976,139.179864432588,
139.279162144185,139.346696991558),.UNSPECIFIED.);
#506=B_SPLINE_CURVE_WITH_KNOTS('',3,(#36324,#36325,#36326,#36327,#36328,
#36329,#36330,#36331,#36332,#36333),.UNSPECIFIED.,.F.,.F.,(4,1,1,1,1,1,
1,4),(139.346704108471,139.680402896665,140.678120060213,141.675837223761,
142.673554387308,143.671271550856,144.668988714403,145.629877388167),
 .UNSPECIFIED.);
#507=B_SPLINE_CURVE_WITH_KNOTS('',3,(#36335,#36336,#36337,#36338,#36339,
#36340,#36341,#36342,#36343,#36344,#36345,#36346,#36347,#36348,#36349,#36350,
#36351,#36352,#36353,#36354,#36355,#36356,#36357,#36358,#36359,#36360,#36361,
#36362,#36363,#36364,#36365,#36366,#36367,#36368,#36369,#36370,#36371,#36372,
#36373,#36374,#36375,#36376,#36377,#36378,#36379,#36380,#36381,#36382,#36383,
#36384,#36385,#36386,#36387,#36388,#36389,#36390,#36391,#36392,#36393,#36394,
#36395,#36396,#36397,#36398,#36399,#36400,#36401,#36402,#36403,#36404,#36405,
#36406,#36407,#36408,#36409,#36410,#36411,#36412,#36413,#36414,#36415,#36416,
#36417,#36418,#36419,#36420,#36421,#36422,#36423,#36424,#36425,#36426,#36427,
#36428,#36429,#36430,#36431,#36432,#36433,#36434,#36435,#36436,#36437,#36438,
#36439,#36440,#36441,#36442,#36443,#36444,#36445,#36446,#36447,#36448,#36449,
#36450,#36451,#36452,#36453,#36454,#36455,#36456,#36457,#36458,#36459,#36460,
#36461,#36462,#36463,#36464,#36465,#36466,#36467,#36468,#36469,#36470,#36471,
#36472,#36473,#36474,#36475,#36476,#36477,#36478,#36479,#36480,#36481,#36482,
#36483,#36484,#36485,#36486,#36487,#36488,#36489,#36490,#36491,#36492,#36493,
#36494,#36495,#36496,#36497,#36498,#36499,#36500,#36501,#36502,#36503,#36504,
#36505,#36506,#36507,#36508,#36509,#36510,#36511,#36512,#36513,#36514,#36515,
#36516,#36517,#36518),.UNSPECIFIED.,.F.,.F.,(4,3,3,3,3,3,3,3,3,3,3,3,3,
3,3,3,3,3,3,3,3,3,3,3,3,3,3,3,3,3,3,3,3,3,3,3,3,3,3,3,3,3,3,3,3,3,3,3,3,
3,3,3,3,3,3,3,3,3,3,3,3,4),(145.629882298737,145.666705877951,145.766384642873,
145.865920420162,145.965733247829,146.065089978344,146.164413953413,146.263735639361,
146.363907489895,146.463373965384,146.563898503442,146.664423041499,146.76413985131,
146.863713619766,146.963516942926,147.062911262015,147.162272592399,147.261631351433,
147.361758564836,147.461261049816,147.561700627431,147.662140205046,147.761856531703,
147.86143020012,147.961233596179,148.060628734971,148.159991226439,148.259351484042,
148.35947795518,148.458982740841,148.559420054718,148.659857368594,148.759429470789,
148.85885831745,148.958697844287,149.057947757569,149.157165188389,149.256380742093,
149.356679189605,149.45604160929,149.556808070715,149.657574532141,149.757455188729,
149.857192392999,149.956954805835,150.056510368982,150.156031757094,150.255549171896,
150.355484802844,150.455140905904,150.555216300796,150.655291695689,150.754023326402,
150.857477251065,150.955955233998,151.054376281426,151.152772005683,151.251173984121,
151.349671802857,151.44822569065,151.546931739433,151.581654723703),
 .UNSPECIFIED.);
#508=B_SPLINE_CURVE_WITH_KNOTS('',3,(#36522,#36523,#36524,#36525,#36526,
#36527,#36528,#36529,#36530),.UNSPECIFIED.,.F.,.F.,(4,1,1,1,1,1,4),(-153.648443186332,
-152.650726022784,-151.653008859237,-150.655291695689,-149.657574532141,
-148.659857368594,-148.604832135738),.UNSPECIFIED.);
#509=B_SPLINE_CURVE_WITH_KNOTS('',3,(#36532,#36533,#36534,#36535,#36536,
#36537,#36538,#36539,#36540,#36541,#36542,#36543,#36544,#36545,#36546,#36547,
#36548,#36549,#36550,#36551,#36552,#36553,#36554,#36555,#36556,#36557,#36558,
#36559,#36560,#36561,#36562,#36563,#36564,#36565,#36566,#36567,#36568,#36569,
#36570,#36571,#36572,#36573,#36574,#36575,#36576,#36577,#36578,#36579,#36580,
#36581,#36582,#36583,#36584,#36585,#36586,#36587,#36588,#36589,#36590,#36591,
#36592,#36593,#36594,#36595,#36596,#36597,#36598,#36599,#36600,#36601,#36602,
#36603,#36604,#36605,#36606,#36607,#36608,#36609,#36610,#36611,#36612,#36613,
#36614,#36615,#36616,#36617,#36618,#36619,#36620,#36621,#36622,#36623,#36624,
#36625,#36626,#36627,#36628,#36629,#36630,#36631,#36632,#36633,#36634,#36635,
#36636,#36637,#36638,#36639,#36640,#36641,#36642,#36643,#36644,#36645,#36646,
#36647,#36648,#36649,#36650,#36651,#36652,#36653,#36654,#36655,#36656,#36657,
#36658,#36659,#36660,#36661,#36662,#36663,#36664,#36665,#36666,#36667,#36668,
#36669,#36670,#36671,#36672,#36673,#36674,#36675,#36676,#36677,#36678,#36679,
#36680,#36681,#36682,#36683,#36684,#36685,#36686,#36687,#36688,#36689,#36690,
#36691,#36692,#36693,#36694,#36695,#36696,#36697,#36698,#36699,#36700,#36701,
#36702,#36703,#36704,#36705,#36706,#36707,#36708,#36709,#36710,#36711,#36712,
#36713,#36714,#36715,#36716,#36717,#36718,#36719,#36720,#36721),
 .UNSPECIFIED.,.F.,.F.,(4,3,3,3,3,3,3,3,3,3,3,3,3,3,3,3,3,3,3,3,3,3,3,3,
3,3,3,3,3,3,3,3,3,3,3,3,3,3,3,3,3,3,3,3,3,3,3,3,3,3,3,3,3,3,3,3,3,3,3,3,
3,3,3,4),(-148.604832135738,-148.505962784877,-148.407231123561,-148.30860605164,
-148.210037628834,-148.111494393919,-148.012944919945,-147.914294538918,
-147.815588589436,-147.716717637151,-147.662140205046,-147.562425664213,
-147.462853677051,-147.363049847607,-147.263656113331,-147.164294916824,
-147.064935841065,-146.964807641174,-146.865303738886,-146.764863390193,
-146.664423041499,-146.564743311022,-146.465206774951,-146.365394162826,
-146.266037180969,-146.166713145758,-146.067391590729,-145.967220162534,
-145.867754284884,-145.767230081417,-145.666705877951,-145.567006099255,
-145.467449250399,-145.3676416834,-145.268263894502,-145.168918912445,-145.069576298971,
-144.969429402829,-144.869942406862,-144.769465560633,-144.668988714403,
-144.569290954782,-144.469736104588,-144.369928035372,-144.270552179694,
-144.171209101692,-144.071868360348,-143.971719157975,-143.872233935751,
-143.771752743304,-143.671271550856,-143.57157791419,-143.472027267565,
-143.372218157532,-143.27284667114,-143.173508015202,-143.074171742837,
-142.974017403955,-142.874536720922,-142.774045554115,-142.673554387308,
-142.558582310432,-142.440114569609,-142.321646828785),.UNSPECIFIED.);
#510=B_SPLINE_CURVE_WITH_KNOTS('',3,(#36723,#36724,#36725,#36726,#36727,
#36728,#36729,#36730,#36731,#36732,#36733,#36734,#36735,#36736,#36737,#36738,
#36739,#36740,#36741,#36742,#36743,#36744,#36745,#36746,#36747,#36748,#36749,
#36750,#36751,#36752,#36753,#36754,#36755,#36756,#36757,#36758,#36759,#36760,
#36761,#36762,#36763,#36764,#36765,#36766,#36767,#36768,#36769,#36770,#36771,
#36772,#36773,#36774,#36775,#36776,#36777,#36778,#36779,#36780,#36781,#36782,
#36783,#36784,#36785,#36786,#36787,#36788,#36789,#36790,#36791,#36792,#36793,
#36794,#36795,#36796,#36797,#36798,#36799,#36800,#36801,#36802,#36803,#36804,
#36805,#36806,#36807,#36808,#36809,#36810,#36811,#36812,#36813,#36814,#36815,
#36816,#36817,#36818,#36819,#36820,#36821,#36822,#36823,#36824,#36825,#36826,
#36827,#36828,#36829,#36830,#36831,#36832,#36833,#36834,#36835,#36836,#36837,
#36838,#36839,#36840,#36841,#36842,#36843,#36844,#36845,#36846,#36847,#36848,
#36849,#36850,#36851,#36852,#36853,#36854,#36855,#36856,#36857,#36858,#36859,
#36860,#36861,#36862,#36863,#36864,#36865,#36866,#36867,#36868,#36869,#36870,
#36871,#36872,#36873,#36874,#36875,#36876,#36877,#36878,#36879,#36880,#36881,
#36882,#36883,#36884,#36885,#36886,#36887,#36888,#36889,#36890,#36891,#36892,
#36893,#36894,#36895,#36896,#36897,#36898,#36899,#36900,#36901,#36902,#36903,
#36904,#36905,#36906,#36907,#36908,#36909,#36910,#36911,#36912,#36913,#36914,
#36915),.UNSPECIFIED.,.F.,.F.,(4,3,3,3,3,3,3,3,3,3,3,3,3,3,3,3,3,3,3,3,
3,3,3,3,3,3,3,3,3,3,3,3,3,3,3,3,3,3,3,3,3,3,3,3,3,3,3,3,3,3,3,3,3,3,3,3,
3,3,3,3,3,3,3,3,4),(-142.321646828558,-142.222022503885,-142.122401901353,
-142.022755196475,-141.922984285233,-141.823143319578,-141.723124900889,
-141.675837223761,-141.576141255699,-141.476588239077,-141.376779716719,
-141.277405783711,-141.178064657725,-141.078725895178,-140.978574436437,
-140.879091238983,-140.778605649598,-140.678120060213,-140.578424560305,
-140.478872021712,-140.379063381081,-140.279689946681,-140.180349325956,
-140.081011074658,-139.98085903016,-139.881376353523,-139.780889625094,
-139.680402896665,-139.580707011083,-139.481154081145,-139.381345537641,
-139.281971700972,-139.182630674759,-139.083292015298,-138.983140444753,
-138.883657357531,-138.783171545324,-138.682685733118,-138.582989938995,
-138.483437101079,-138.383628534641,-138.284254790672,-138.184913857203,
-138.085575290406,-137.985423610197,-137.88594061448,-137.785454592025,
-137.68496856957,-137.58527282556,-137.485720038928,-137.385911459815,-137.286537769609,
-137.187196890722,-137.087858379249,-136.987706635943,-136.888223696826,
-136.787737551424,-136.687251406023,-136.587301790218,-136.48749505883,
-136.387800988718,-136.288189658078,-136.188626947872,-136.089062730842,
-136.038461521379),.UNSPECIFIED.);
#511=B_SPLINE_CURVE_WITH_KNOTS('',3,(#36917,#36918,#36919,#36920,#36921,
#36922,#36923,#36924,#36925,#36926,#36927,#36928,#36929,#36930,#36931,#36932,
#36933,#36934,#36935,#36936,#36937,#36938,#36939,#36940,#36941,#36942,#36943,
#36944,#36945,#36946,#36947,#36948,#36949,#36950,#36951,#36952,#36953,#36954,
#36955,#36956,#36957,#36958,#36959,#36960,#36961,#36962,#36963,#36964,#36965,
#36966,#36967,#36968,#36969,#36970,#36971,#36972,#36973,#36974,#36975,#36976,
#36977,#36978,#36979,#36980,#36981,#36982,#36983,#36984,#36985,#36986,#36987,
#36988,#36989,#36990,#36991,#36992,#36993,#36994,#36995,#36996,#36997,#36998,
#36999,#37000,#37001,#37002,#37003,#37004,#37005,#37006,#37007,#37008,#37009,
#37010,#37011,#37012,#37013,#37014,#37015,#37016,#37017,#37018,#37019,#37020,
#37021,#37022,#37023,#37024,#37025,#37026,#37027,#37028,#37029,#37030,#37031,
#37032,#37033,#37034,#37035,#37036,#37037,#37038,#37039,#37040,#37041,#37042,
#37043,#37044,#37045,#37046,#37047,#37048,#37049,#37050,#37051,#37052,#37053,
#37054,#37055,#37056,#37057,#37058,#37059,#37060,#37061,#37062,#37063,#37064,
#37065,#37066,#37067,#37068,#37069,#37070,#37071,#37072,#37073,#37074,#37075,
#37076,#37077,#37078,#37079,#37080,#37081,#37082,#37083,#37084,#37085,#37086,
#37087,#37088,#37089,#37090,#37091,#37092,#37093,#37094,#37095,#37096,#37097,
#37098,#37099,#37100,#37101,#37102,#37103,#37104,#37105,#37106),
 .UNSPECIFIED.,.F.,.F.,(4,3,3,3,3,3,3,3,3,3,3,3,3,3,3,3,3,3,3,3,3,3,3,3,
3,3,3,3,3,3,3,3,3,3,3,3,3,3,3,3,3,3,3,3,3,3,3,3,3,3,3,3,3,3,3,3,3,3,3,3,
3,3,3,4),(-136.038461521153,-135.924409265068,-135.806971753772,-135.689534242475,
-135.589838462332,-135.490285638907,-135.390477068909,-135.29110334057,
-135.191762423128,-135.092423872733,-134.992272174281,-134.892789195728,
-134.792303137327,-134.691817078927,-134.59212130367,-134.492568485263,
-134.392759914028,-134.293386190995,-134.194045278957,-134.094706734055,
-133.994555029386,-133.895072056493,-133.794585985936,-133.69409991538,
-133.594404133346,-133.494851308051,-133.395042738524,-133.29566900839,
-133.196328089184,-133.096989537059,-132.996837840753,-132.897354860572,
-132.796868806202,-132.696382751832,-132.596686972278,-132.497134149491,
-132.39732557934,-132.297951851756,-132.198610935112,-132.099272385557,
-131.999120686239,-131.899637708619,-131.799151648452,-131.698665588285,
-131.598969809128,-131.499416986751,-131.399608416499,-131.300234689358,
-131.200893773167,-131.101555224075,-131.001403524241,-130.901920547106,
-130.801434485922,-130.700948424737,-130.602038734921,-130.50327125118,
-130.404617056666,-130.30602371374,-130.207459776814,-130.108893838909,
-130.010232689273,-129.911519685389,-129.812645395257,-129.755276214539),
 .UNSPECIFIED.);
#512=B_SPLINE_CURVE_WITH_KNOTS('',3,(#37108,#37109,#37110,#37111,#37112,
#37113,#37114,#37115,#37116,#37117,#37118,#37119,#37120,#37121,#37122,#37123,
#37124,#37125,#37126,#37127,#37128,#37129,#37130,#37131,#37132,#37133,#37134,
#37135,#37136,#37137,#37138,#37139,#37140,#37141,#37142,#37143,#37144,#37145,
#37146,#37147,#37148,#37149,#37150,#37151,#37152,#37153,#37154,#37155,#37156,
#37157,#37158,#37159,#37160,#37161,#37162,#37163,#37164,#37165,#37166,#37167,
#37168,#37169,#37170,#37171,#37172,#37173,#37174,#37175,#37176,#37177,#37178,
#37179,#37180,#37181,#37182,#37183,#37184,#37185,#37186,#37187,#37188,#37189,
#37190,#37191,#37192,#37193,#37194,#37195,#37196,#37197,#37198,#37199,#37200,
#37201,#37202,#37203,#37204,#37205,#37206,#37207,#37208,#37209,#37210,#37211,
#37212,#37213,#37214,#37215,#37216,#37217,#37218,#37219,#37220,#37221,#37222,
#37223,#37224,#37225,#37226,#37227,#37228,#37229,#37230,#37231,#37232,#37233,
#37234,#37235,#37236,#37237,#37238,#37239,#37240,#37241,#37242,#37243,#37244,
#37245,#37246,#37247,#37248,#37249,#37250,#37251,#37252,#37253,#37254,#37255,
#37256,#37257,#37258,#37259,#37260,#37261,#37262,#37263,#37264,#37265,#37266,
#37267,#37268,#37269,#37270,#37271,#37272,#37273,#37274,#37275,#37276,#37277,
#37278,#37279,#37280,#37281,#37282,#37283,#37284,#37285,#37286,#37287,#37288,
#37289,#37290,#37291,#37292,#37293,#37294,#37295,#37296,#37297),
 .UNSPECIFIED.,.F.,.F.,(4,3,3,3,3,3,3,3,3,3,3,3,3,3,3,3,3,3,3,3,3,3,3,3,
3,3,3,3,3,3,3,3,3,3,3,3,3,3,3,3,3,3,3,3,3,3,3,3,3,3,3,3,3,3,3,3,3,3,3,3,
3,3,3,4),(-129.755276214199,-129.703231261189,-129.603535481542,-129.503982658665,
-129.404174088537,-129.304800360874,-129.205459444155,-129.106120894529,
-129.005969195307,-128.906486217628,-128.806000157635,-128.705514097642,
-128.605818318012,-128.506265495153,-128.406456925021,-128.307083197379,
-128.207742280683,-128.108403731081,-128.008252031834,-127.908769054182,
-127.808282994138,-127.707796934094,-127.608101154355,-127.508548331385,
-127.40873976128,-127.309366033524,-127.210025116712,-127.110686566993,
-127.010534867881,-126.911051890111,-126.810565830328,-126.710079770546,
-126.610383990863,-126.510831167951,-126.411022597832,-126.311648870134,
-126.212307953381,-126.11296940372,-126.01281770454,-125.913334726828,-125.812848666914,
-125.712362606999,-125.612666827313,-125.513114004398,-125.413305434279,
-125.313931706579,-125.214590789824,-125.115252240161,-125.015100540983,
-124.91561756327,-124.81513150336,-124.714645443451,-124.614949663752,-124.515396840823,
-124.415588270708,-124.316214542995,-124.216873626225,-124.117535076548,
-124.017383377387,-123.917900399659,-123.817414339782,-123.716928279904,
-123.586846403148,-123.472090978371),.UNSPECIFIED.);
#513=B_SPLINE_CURVE_WITH_KNOTS('',3,(#37299,#37300,#37301,#37302,#37303,
#37304,#37305,#37306,#37307,#37308),.UNSPECIFIED.,.F.,.F.,(4,1,1,1,1,1,
1,4),(-123.47209090702,-122.719211116356,-121.721493952808,-120.723776789261,
-119.726059625713,-118.728342462166,-117.730625298618,-117.18890559984),
 .UNSPECIFIED.);
#514=B_SPLINE_CURVE_WITH_KNOTS('',3,(#37310,#37311,#37312,#37313,#37314,
#37315,#37316,#37317,#37318,#37319,#37320,#37321,#37322,#37323,#37324,#37325,
#37326,#37327,#37328,#37329,#37330,#37331,#37332,#37333,#37334,#37335,#37336,
#37337,#37338,#37339,#37340,#37341,#37342,#37343,#37344,#37345,#37346,#37347,
#37348,#37349,#37350,#37351,#37352,#37353,#37354,#37355,#37356,#37357,#37358,
#37359,#37360,#37361,#37362,#37363,#37364,#37365,#37366,#37367,#37368,#37369,
#37370,#37371,#37372,#37373,#37374,#37375,#37376,#37377,#37378,#37379,#37380,
#37381,#37382,#37383,#37384,#37385,#37386,#37387,#37388,#37389,#37390,#37391,
#37392,#37393,#37394,#37395,#37396,#37397,#37398,#37399,#37400,#37401,#37402,
#37403,#37404,#37405,#37406,#37407,#37408,#37409,#37410,#37411,#37412,#37413,
#37414,#37415,#37416,#37417,#37418,#37419,#37420,#37421,#37422,#37423,#37424,
#37425,#37426,#37427,#37428,#37429,#37430,#37431,#37432,#37433,#37434,#37435,
#37436,#37437,#37438,#37439,#37440,#37441,#37442,#37443,#37444,#37445,#37446,
#37447,#37448,#37449,#37450,#37451,#37452,#37453,#37454,#37455,#37456,#37457,
#37458,#37459,#37460,#37461,#37462,#37463,#37464,#37465,#37466,#37467,#37468,
#37469,#37470,#37471,#37472,#37473,#37474,#37475,#37476,#37477,#37478,#37479,
#37480,#37481,#37482,#37483,#37484,#37485,#37486,#37487,#37488,#37489,#37490,
#37491,#37492,#37493,#37494,#37495,#37496,#37497,#37498,#37499,#37500,#37501,
#37502),.UNSPECIFIED.,.F.,.F.,(4,3,3,3,3,3,3,3,3,3,3,3,3,3,3,3,3,3,3,3,
3,3,3,3,3,3,3,3,3,3,3,3,3,3,3,3,3,3,3,3,3,3,3,3,3,3,3,3,3,3,3,3,3,3,3,3,
3,3,3,3,3,3,3,3,4),(-117.188905373774,-117.082806220657,-116.976309141457,
-116.869598521819,-116.76256993861,-116.73290813507,-116.633212355378,-116.533659532456,
-116.433850962339,-116.334477234632,-116.23513631787,-116.1357977682,-116.035646069031,
-115.93616309131,-115.835677031416,-115.735190971523,-115.63549519183,-115.535942368908,
-115.436133798791,-115.336760071084,-115.23741915432,-115.13808060465,-115.037928905481,
-114.93844592776,-114.837959867867,-114.737473807975,-114.637778028282,
-114.53822520536,-114.438416635244,-114.339042907536,-114.239701990773,
-114.140363441103,-114.040211741934,-113.940728764213,-113.840242704321,
-113.739756644428,-113.640060864735,-113.540508041813,-113.440699471697,
-113.341325743989,-113.241984827226,-113.142646277556,-113.042494578387,
-112.943011600666,-112.842525540773,-112.74203948088,-112.642343701187,
-112.542790878265,-112.442982308148,-112.343608580441,-112.244267663677,
-112.144929114007,-112.044777414838,-111.945294437117,-111.844808377224,
-111.744322317332,-111.646106275261,-111.548054692826,-111.45009534431,
-111.352196038359,-111.254324663627,-111.156401948211,-111.058451996033,
-110.960378173053,-110.905720293008),.UNSPECIFIED.);
#515=B_SPLINE_CURVE_WITH_KNOTS('',3,(#37504,#37505,#37506,#37507,#37508,
#37509,#37510,#37511,#37512,#37513,#37514,#37515,#37516,#37517,#37518,#37519,
#37520,#37521,#37522,#37523,#37524,#37525,#37526,#37527,#37528,#37529,#37530,
#37531,#37532,#37533,#37534,#37535,#37536,#37537,#37538,#37539,#37540,#37541,
#37542,#37543,#37544,#37545,#37546,#37547,#37548,#37549,#37550,#37551,#37552,
#37553,#37554,#37555,#37556,#37557,#37558,#37559,#37560,#37561,#37562,#37563,
#37564,#37565,#37566,#37567,#37568,#37569,#37570,#37571,#37572,#37573,#37574,
#37575,#37576,#37577,#37578,#37579,#37580,#37581,#37582,#37583,#37584,#37585,
#37586,#37587,#37588,#37589,#37590,#37591,#37592,#37593,#37594,#37595,#37596,
#37597,#37598,#37599,#37600,#37601,#37602,#37603,#37604,#37605,#37606,#37607,
#37608,#37609,#37610,#37611,#37612,#37613,#37614,#37615,#37616,#37617,#37618,
#37619,#37620,#37621,#37622,#37623,#37624,#37625,#37626,#37627,#37628,#37629,
#37630,#37631,#37632,#37633,#37634,#37635,#37636,#37637,#37638,#37639,#37640,
#37641,#37642,#37643,#37644,#37645,#37646,#37647,#37648,#37649,#37650,#37651,
#37652,#37653,#37654,#37655,#37656,#37657,#37658,#37659,#37660,#37661,#37662,
#37663,#37664,#37665,#37666,#37667,#37668,#37669,#37670,#37671,#37672,#37673,
#37674,#37675,#37676,#37677,#37678,#37679,#37680,#37681,#37682,#37683,#37684,
#37685,#37686,#37687,#37688,#37689,#37690),.UNSPECIFIED.,.F.,.F.,(4,3,3,
3,3,3,3,3,3,3,3,3,3,3,3,3,3,3,3,3,3,3,3,3,3,3,3,3,3,3,3,3,3,3,3,3,3,3,3,
3,3,3,3,3,3,3,3,3,3,3,3,3,3,3,3,3,3,3,3,3,3,3,4),(-110.90572029266,-110.746605153785,
-110.646909374091,-110.547356551166,-110.44754798105,-110.348174253341,
-110.248833336576,-110.149494786903,-110.049343087737,-109.949860110014,
-109.849374050125,-109.748887990237,-109.649192210544,-109.549639387622,
-109.449830817506,-109.350457089798,-109.251116173035,-109.151777623365,
-109.051625924196,-108.952142946475,-108.851656886582,-108.751170826689,
-108.651475046997,-108.551922224075,-108.452113653958,-108.352739926252,
-108.253399009489,-108.154060459819,-108.05390876065,-107.954425782929,
-107.853939723036,-107.753453663142,-107.653757883449,-107.554205060526,
-107.45439649041,-107.355022762702,-107.255681845939,-107.156343296268,
-107.0561915971,-106.956708619378,-106.856222559486,-106.755736499594,-106.656040719902,
-106.556487896979,-106.456679326863,-106.357305599156,-106.257964682393,
-106.158626132723,-106.058474433554,-105.958991455833,-105.85850539594,
-105.758019336047,-105.658323556354,-105.558770733432,-105.458962163316,
-105.359588435608,-105.260247518845,-105.160908969175,-105.060757270006,
-104.961274292285,-104.860788232392,-104.760302172499,-104.622534985481),
 .UNSPECIFIED.);
#516=B_SPLINE_CURVE_WITH_KNOTS('',3,(#37692,#37693,#37694,#37695,#37696,
#37697,#37698,#37699,#37700,#37701),.UNSPECIFIED.,.F.,.F.,(4,1,1,1,1,1,
1,4),(-104.622526910524,-103.762585008951,-102.764867845404,-101.767150681856,
-100.769433518309,-99.771716354761,-98.7739991912134,-98.3393545396807),
 .UNSPECIFIED.);
#517=B_SPLINE_CURVE_WITH_KNOTS('',3,(#37703,#37704,#37705,#37706,#37707,
#37708,#37709,#37710,#37711,#37712,#37713,#37714,#37715,#37716,#37717,#37718,
#37719,#37720,#37721,#37722,#37723,#37724,#37725,#37726,#37727,#37728,#37729,
#37730,#37731,#37732,#37733,#37734,#37735,#37736,#37737,#37738,#37739,#37740,
#37741,#37742,#37743,#37744,#37745,#37746,#37747,#37748,#37749,#37750,#37751,
#37752,#37753,#37754,#37755,#37756,#37757,#37758,#37759,#37760,#37761,#37762,
#37763,#37764,#37765,#37766,#37767,#37768,#37769,#37770,#37771,#37772,#37773,
#37774,#37775,#37776,#37777,#37778,#37779,#37780,#37781,#37782,#37783,#37784,
#37785,#37786,#37787,#37788,#37789,#37790,#37791,#37792,#37793,#37794,#37795,
#37796,#37797,#37798,#37799,#37800,#37801,#37802,#37803,#37804,#37805,#37806,
#37807,#37808,#37809,#37810,#37811,#37812,#37813,#37814,#37815,#37816,#37817,
#37818,#37819,#37820,#37821,#37822,#37823,#37824,#37825,#37826,#37827,#37828,
#37829,#37830,#37831,#37832,#37833,#37834,#37835,#37836,#37837,#37838,#37839,
#37840,#37841,#37842,#37843,#37844,#37845,#37846,#37847,#37848,#37849,#37850,
#37851,#37852,#37853,#37854,#37855,#37856,#37857,#37858,#37859,#37860,#37861,
#37862,#37863,#37864,#37865,#37866,#37867,#37868,#37869,#37870,#37871,#37872,
#37873,#37874,#37875,#37876,#37877,#37878,#37879,#37880,#37881,#37882,#37883,
#37884,#37885,#37886,#37887,#37888,#37889,#37890,#37891,#37892,#37893,#37894,
#37895),.UNSPECIFIED.,.F.,.F.,(4,3,3,3,3,3,3,3,3,3,3,3,3,3,3,3,3,3,3,3,
3,3,3,3,3,3,3,3,3,3,3,3,3,3,3,3,3,3,3,3,3,3,3,3,3,3,3,3,3,3,3,3,3,3,3,3,
3,3,3,3,3,3,3,3,4),(-98.3393496783013,-98.2376690492644,-98.1359188389092,
-98.0339904197929,-97.9319640594039,-97.8297250457828,-97.7762820276658,
-97.6765862479732,-97.5770334250509,-97.4772248549343,-97.377851127227,
-97.278510210464,-97.1791716607937,-97.0790199616248,-96.9795369839036,
-96.8790509240109,-96.7785648641182,-96.6788690844256,-96.5793162615036,
-96.4795076913869,-96.3801339636796,-96.2807930469166,-96.1814544972463,
-96.0813027980773,-95.9818198203562,-95.8813337604633,-95.7808477005705,
-95.6811519208779,-95.5815990979555,-95.4817905278389,-95.3824168001316,
-95.2830758833684,-95.1837373336981,-95.0835856345293,-94.9841026568082,
-94.8836165969155,-94.7831305370229,-94.6834347573304,-94.583881934408,
-94.4840733642914,-94.3846996365841,-94.2853587198211,-94.1860201701505,
-94.0858684709817,-93.9863854932605,-93.8858994333679,-93.7854133734753,
-93.6857175937827,-93.5861647708604,-93.4863562007438,-93.3869824730366,
-93.2876415562734,-93.1883030066032,-93.0881513074343,-92.9886683297131,
-92.8881822698204,-92.7876962099277,-92.6890183930632,-92.5904711330326,
-92.492022572886,-92.3936409753712,-92.2952704891613,-92.1969067553828,
-92.0984785297572,-92.0561643711217),.UNSPECIFIED.);
#518=B_SPLINE_CURVE_WITH_KNOTS('',3,(#37897,#37898,#37899,#37900,#37901,
#37902,#37903,#37904,#37905,#37906,#37907,#37908,#37909,#37910,#37911,#37912,
#37913,#37914,#37915,#37916,#37917,#37918,#37919,#37920,#37921,#37922,#37923,
#37924,#37925,#37926,#37927,#37928,#37929,#37930,#37931,#37932,#37933,#37934,
#37935,#37936,#37937,#37938,#37939,#37940,#37941,#37942,#37943,#37944,#37945,
#37946,#37947,#37948,#37949,#37950,#37951,#37952,#37953,#37954,#37955,#37956,
#37957,#37958,#37959,#37960,#37961,#37962,#37963,#37964,#37965,#37966,#37967,
#37968,#37969,#37970,#37971,#37972,#37973,#37974,#37975,#37976,#37977,#37978,
#37979,#37980,#37981,#37982,#37983,#37984,#37985,#37986,#37987,#37988,#37989,
#37990,#37991,#37992,#37993,#37994,#37995,#37996,#37997,#37998,#37999,#38000,
#38001,#38002,#38003,#38004,#38005,#38006,#38007,#38008,#38009,#38010,#38011,
#38012,#38013,#38014,#38015,#38016,#38017,#38018,#38019,#38020,#38021,#38022,
#38023,#38024,#38025,#38026,#38027,#38028,#38029,#38030,#38031,#38032,#38033,
#38034,#38035,#38036,#38037,#38038,#38039,#38040,#38041,#38042,#38043,#38044,
#38045,#38046,#38047,#38048,#38049,#38050,#38051,#38052,#38053,#38054,#38055,
#38056,#38057,#38058,#38059,#38060,#38061,#38062,#38063,#38064,#38065,#38066,
#38067,#38068,#38069,#38070,#38071,#38072,#38073,#38074,#38075,#38076,#38077,
#38078,#38079,#38080,#38081,#38082,#38083,#38084,#38085,#38086,#38087,#38088,
#38089),.UNSPECIFIED.,.F.,.F.,(4,3,3,3,3,3,3,3,3,3,3,3,3,3,3,3,3,3,3,3,
3,3,3,3,3,3,3,3,3,3,3,3,3,3,3,3,3,3,3,3,3,3,3,3,3,3,3,3,3,3,3,3,3,3,3,3,
3,3,3,3,3,3,3,3,4),(-92.0561643707478,-91.931627218391,-91.8046642324725,
-91.7899790463801,-91.6902832666874,-91.5907304437651,-91.4909218736485,
-91.3915481459411,-91.292207229178,-91.1928686795075,-91.0927169803387,
-90.9932340026175,-90.892747942725,-90.7922618828325,-90.6925661031399,
-90.5930132802175,-90.4932047101009,-90.3938309823936,-90.2944900656304,
-90.1951515159601,-90.0949998167913,-89.9955168390701,-89.8950307791775,
-89.7945447192849,-89.6948489395923,-89.5952961166701,-89.4954875465535,
-89.3961138188463,-89.2967729020832,-89.197434352413,-89.097282653244,-88.9977996755229,
-88.8973136156301,-88.7968275557373,-88.6971317760447,-88.5975789531223,
-88.4977703830058,-88.3983966552984,-88.2990557385353,-88.1997171888649,
-88.0995654896961,-88.000082511975,-87.8995964520823,-87.7991103921897,
-87.6994146124971,-87.5998617895749,-87.5000532194583,-87.400679491751,
-87.301338574988,-87.2020000253177,-87.1018483261488,-87.0023653484277,
-86.9018792885349,-86.8013932286421,-86.7016974489495,-86.6021446260272,
-86.5023360559106,-86.4029623282033,-86.3036214114402,-86.20428286177,-86.1041311626011,
-86.00464818488,-85.9041621249873,-85.8036760650945,-85.7729790639421),
 .UNSPECIFIED.);
#519=B_SPLINE_CURVE_WITH_KNOTS('',3,(#38091,#38092,#38093,#38094,#38095,
#38096,#38097,#38098,#38099,#38100,#38101,#38102,#38103,#38104,#38105,#38106,
#38107,#38108,#38109,#38110,#38111,#38112,#38113,#38114,#38115,#38116,#38117,
#38118,#38119,#38120,#38121,#38122,#38123,#38124,#38125,#38126,#38127,#38128,
#38129,#38130,#38131,#38132,#38133,#38134,#38135,#38136,#38137,#38138,#38139,
#38140,#38141,#38142,#38143,#38144,#38145,#38146,#38147,#38148,#38149,#38150,
#38151,#38152,#38153,#38154,#38155,#38156,#38157,#38158,#38159,#38160,#38161,
#38162,#38163,#38164,#38165,#38166,#38167,#38168,#38169,#38170,#38171,#38172,
#38173,#38174,#38175,#38176,#38177,#38178,#38179,#38180,#38181,#38182,#38183,
#38184,#38185,#38186,#38187,#38188,#38189,#38190,#38191,#38192,#38193,#38194,
#38195,#38196,#38197,#38198,#38199,#38200,#38201,#38202,#38203,#38204,#38205,
#38206,#38207,#38208,#38209,#38210,#38211,#38212,#38213,#38214,#38215,#38216,
#38217,#38218,#38219,#38220,#38221,#38222,#38223,#38224,#38225,#38226,#38227,
#38228,#38229,#38230,#38231,#38232,#38233,#38234,#38235,#38236,#38237,#38238,
#38239,#38240,#38241,#38242,#38243,#38244,#38245,#38246,#38247,#38248,#38249,
#38250,#38251,#38252,#38253,#38254,#38255,#38256,#38257,#38258,#38259,#38260,
#38261,#38262,#38263,#38264,#38265,#38266,#38267,#38268,#38269,#38270,#38271,
#38272,#38273,#38274,#38275,#38276,#38277,#38278,#38279,#38280),
 .UNSPECIFIED.,.F.,.F.,(4,3,3,3,3,3,3,3,3,3,3,3,3,3,3,3,3,3,3,3,3,3,3,3,
3,3,3,3,3,3,3,3,3,3,3,3,3,3,3,3,3,3,3,3,3,3,3,3,3,3,3,3,3,3,3,3,3,3,3,3,
3,3,3,4),(-85.7729790637246,-85.6737911039112,-85.5747441639126,-85.475808919837,
-85.3769340092717,-85.2780883091123,-85.1792407338146,-85.0802938326087,
-84.98129593964,-84.8821251945386,-84.8059589015468,-84.7062631218542,-84.6067102989321,
-84.5069017288155,-84.4075280011082,-84.3081870843452,-84.2088485346748,
-84.1086968355059,-84.0092138577848,-83.908727797892,-83.8082417379992,
-83.7085459583067,-83.6089931353844,-83.5091845652678,-83.4098108375605,
-83.3104699207974,-83.2111313711273,-83.1109796719583,-83.0114966942372,
-82.9110106343444,-82.8105245744516,-82.710828794759,-82.6112759718368,
-82.5114674017202,-82.4120936740129,-82.3127527572499,-82.2134142075797,
-82.1132625084108,-82.0137795306895,-81.9132934707968,-81.812807410904,
-81.7131116312114,-81.613558808289,-81.5137502381724,-81.4143765104651,
-81.3150355937019,-81.2156970440318,-81.1155453448629,-81.0160623671418,
-80.9155763072491,-80.8150902473564,-80.7153944676637,-80.6158416447413,
-80.5160330746247,-80.4166593469174,-80.3173184301543,-80.217979880484,
-80.1178281813152,-80.0183452035941,-79.9178591437014,-79.8173730838088,
-79.6996970766505,-79.5832300154978,-79.489793756973),.UNSPECIFIED.);
#520=B_SPLINE_CURVE_WITH_KNOTS('',3,(#38282,#38283,#38284,#38285,#38286,
#38287,#38288,#38289,#38290,#38291,#38292,#38293,#38294,#38295,#38296,#38297,
#38298,#38299,#38300,#38301,#38302,#38303,#38304,#38305,#38306,#38307,#38308,
#38309,#38310,#38311,#38312,#38313,#38314,#38315,#38316,#38317,#38318,#38319,
#38320,#38321,#38322,#38323,#38324,#38325,#38326,#38327,#38328,#38329,#38330,
#38331,#38332,#38333,#38334,#38335,#38336,#38337,#38338,#38339,#38340,#38341,
#38342,#38343,#38344,#38345,#38346,#38347,#38348,#38349,#38350,#38351,#38352,
#38353,#38354,#38355,#38356,#38357,#38358,#38359,#38360,#38361,#38362,#38363,
#38364,#38365,#38366,#38367,#38368,#38369,#38370,#38371,#38372,#38373,#38374,
#38375,#38376,#38377,#38378,#38379,#38380,#38381,#38382,#38383,#38384,#38385,
#38386,#38387,#38388,#38389,#38390,#38391,#38392,#38393,#38394,#38395,#38396,
#38397,#38398,#38399,#38400,#38401,#38402,#38403,#38404,#38405,#38406,#38407,
#38408,#38409,#38410,#38411,#38412,#38413,#38414,#38415,#38416,#38417,#38418,
#38419,#38420,#38421,#38422,#38423,#38424,#38425,#38426,#38427,#38428,#38429,
#38430,#38431,#38432,#38433,#38434,#38435,#38436,#38437,#38438,#38439,#38440,
#38441,#38442,#38443,#38444,#38445,#38446,#38447,#38448,#38449,#38450,#38451,
#38452,#38453,#38454,#38455,#38456,#38457,#38458,#38459,#38460,#38461,#38462,
#38463,#38464,#38465,#38466,#38467,#38468,#38469,#38470,#38471,#38472,#38473,
#38474),.UNSPECIFIED.,.F.,.F.,(4,3,3,3,3,3,3,3,3,3,3,3,3,3,3,3,3,3,3,3,
3,3,3,3,3,3,3,3,3,3,3,3,3,3,3,3,3,3,3,3,3,3,3,3,3,3,3,3,3,3,3,3,3,3,3,3,
3,3,3,3,3,3,3,3,4),(-79.4897937567625,-79.3905970449177,-79.2914199481721,
-79.192231915772,-79.0929327497898,-78.9935756638494,-78.8940377107173,
-78.8196559202612,-78.7199601405687,-78.6204073176465,-78.5205987475299,
-78.4212250198226,-78.3218841030596,-78.2225455533893,-78.1223938542204,
-78.0229108764993,-77.9224248166065,-77.8219387567136,-77.722242977021,
-77.6226901540989,-77.5228815839823,-77.423507856275,-77.3241669395119,
-77.2248283898415,-77.1246766906727,-77.0251937129515,-76.9247076530588,
-76.824221593166,-76.7245258134733,-76.6249729905509,-76.5251644204344,
-76.425790692727,-76.3264497759638,-76.2271112262934,-76.1269595271247,
-76.0274765494036,-75.926990489511,-75.8265044296184,-75.7268086499258,
-75.6272558270034,-75.5274472568868,-75.4280735291795,-75.3287326124164,
-75.2293940627459,-75.1292423635771,-75.0297593858559,-74.9292733259633,
-74.8287872660707,-74.7290914863781,-74.6295386634556,-74.5297300933391,
-74.4303563656318,-74.3310154488686,-74.2316768991982,-74.1315252000294,
-74.0320422223083,-73.9315561624157,-73.8310701025231,-73.7305796798271,
-73.6302379772179,-73.530015697372,-73.4298907195394,-73.3298214476302,
-73.229770789038,-73.206608449583),.UNSPECIFIED.);
#521=B_SPLINE_CURVE_WITH_KNOTS('',3,(#38476,#38477,#38478,#38479,#38480,
#38481,#38482,#38483,#38484,#38485,#38486,#38487,#38488,#38489,#38490,#38491,
#38492,#38493,#38494,#38495,#38496,#38497,#38498,#38499,#38500,#38501,#38502,
#38503,#38504,#38505,#38506,#38507,#38508,#38509,#38510,#38511,#38512,#38513,
#38514,#38515,#38516,#38517,#38518,#38519,#38520,#38521,#38522,#38523,#38524,
#38525,#38526,#38527,#38528,#38529,#38530,#38531,#38532,#38533,#38534,#38535,
#38536,#38537,#38538,#38539,#38540,#38541,#38542,#38543,#38544,#38545,#38546,
#38547,#38548,#38549,#38550,#38551,#38552,#38553,#38554,#38555,#38556,#38557,
#38558,#38559,#38560,#38561,#38562,#38563,#38564,#38565,#38566,#38567,#38568,
#38569,#38570,#38571,#38572,#38573,#38574,#38575,#38576,#38577,#38578,#38579,
#38580,#38581,#38582,#38583,#38584,#38585,#38586,#38587,#38588,#38589,#38590,
#38591,#38592,#38593,#38594,#38595,#38596,#38597,#38598,#38599,#38600,#38601,
#38602,#38603,#38604,#38605,#38606,#38607,#38608,#38609,#38610,#38611,#38612,
#38613,#38614,#38615,#38616,#38617,#38618,#38619,#38620,#38621,#38622,#38623,
#38624,#38625,#38626,#38627,#38628,#38629,#38630,#38631,#38632,#38633,#38634,
#38635,#38636,#38637,#38638,#38639,#38640,#38641,#38642,#38643,#38644,#38645,
#38646,#38647,#38648,#38649,#38650,#38651,#38652,#38653,#38654,#38655,#38656,
#38657,#38658,#38659,#38660,#38661,#38662,#38663,#38664,#38665,#38666,#38667,
#38668),.UNSPECIFIED.,.F.,.F.,(4,3,3,3,3,3,3,3,3,3,3,3,3,3,3,3,3,3,3,3,
3,3,3,3,3,3,3,3,3,3,3,3,3,3,3,3,3,3,3,3,3,3,3,3,3,3,3,3,3,3,3,3,3,3,3,3,
3,3,3,3,3,3,3,3,4),(-73.2066084493534,-73.0947351858594,-72.9823558650838,
-72.8693592293596,-72.8333529389755,-72.733657159283,-72.634104336361,-72.5342957662444,
-72.4349220385372,-72.3355811217742,-72.2362425721041,-72.136090872935,
-72.0366078952139,-71.9361218353209,-71.8356357754279,-71.7359399957353,
-71.6363871728129,-71.5365786026964,-71.437204874989,-71.3378639582259,
-71.2385254085555,-71.1383737093867,-71.0388907316655,-70.9384046717729,
-70.8379186118803,-70.7382228321877,-70.6386700092655,-70.5388614391489,
-70.4394877114416,-70.3401467946786,-70.2408082450082,-70.1406565458394,
-70.0411735681182,-69.9406875082255,-69.8402014483327,-69.7405056686401,
-69.6409528457178,-69.5411442756012,-69.4417705478939,-69.3424296311308,
-69.2430910814604,-69.1429393822916,-69.0434564045704,-68.9429703446778,
-68.8424842847851,-68.7427885050925,-68.6432356821703,-68.5434271120537,
-68.4440533843464,-68.3447124675833,-68.245373917913,-68.1452222187441,
-68.045739241023,-67.9452531811302,-67.8447671212375,-67.7461212768715,
-67.6432840100895,-67.5448962910023,-67.4465673157563,-67.3482653708917,
-67.2499587801198,-67.151559441021,-67.0531052122828,-66.9545027531578,
-66.923423142615),.UNSPECIFIED.);
#522=B_SPLINE_CURVE_WITH_KNOTS('',3,(#38670,#38671,#38672,#38673,#38674,
#38675,#38676,#38677,#38678,#38679,#38680,#38681,#38682,#38683,#38684,#38685,
#38686,#38687,#38688,#38689,#38690,#38691,#38692,#38693,#38694,#38695,#38696,
#38697,#38698,#38699,#38700,#38701,#38702,#38703,#38704,#38705,#38706,#38707,
#38708,#38709,#38710,#38711,#38712,#38713,#38714,#38715,#38716,#38717,#38718,
#38719,#38720,#38721,#38722,#38723,#38724,#38725,#38726,#38727,#38728,#38729,
#38730,#38731,#38732,#38733,#38734,#38735,#38736,#38737,#38738,#38739,#38740,
#38741,#38742,#38743,#38744,#38745,#38746,#38747,#38748,#38749,#38750,#38751,
#38752,#38753,#38754,#38755,#38756,#38757,#38758,#38759,#38760,#38761,#38762,
#38763,#38764,#38765,#38766,#38767,#38768,#38769,#38770,#38771,#38772,#38773,
#38774,#38775,#38776,#38777,#38778,#38779,#38780,#38781,#38782,#38783,#38784,
#38785,#38786,#38787,#38788,#38789,#38790,#38791,#38792,#38793,#38794,#38795,
#38796,#38797,#38798,#38799,#38800,#38801,#38802,#38803,#38804,#38805,#38806,
#38807,#38808,#38809,#38810,#38811,#38812,#38813,#38814,#38815,#38816,#38817,
#38818,#38819,#38820,#38821,#38822,#38823,#38824,#38825,#38826,#38827,#38828,
#38829,#38830,#38831,#38832,#38833,#38834,#38835,#38836,#38837,#38838,#38839,
#38840,#38841,#38842,#38843,#38844,#38845,#38846,#38847,#38848,#38849,#38850,
#38851,#38852,#38853,#38854,#38855,#38856,#38857,#38858,#38859),
 .UNSPECIFIED.,.F.,.F.,(4,3,3,3,3,3,3,3,3,3,3,3,3,3,3,3,3,3,3,3,3,3,3,3,
3,3,3,3,3,3,3,3,3,3,3,3,3,3,3,3,3,3,3,3,3,3,3,3,3,3,3,3,3,3,3,3,3,3,3,3,
3,3,3,4),(-66.9234231424034,-66.8470499576899,-66.7473541779973,-66.647801355075,
-66.5479927849585,-66.4486190572512,-66.3492781404881,-66.2499395908178,
-66.1497878916489,-66.0503049139278,-65.949818854035,-65.8493327941423,
-65.7496370144496,-65.6500841915273,-65.5502756214107,-65.4509018937034,
-65.3515609769403,-65.25222242727,-65.1520707281011,-65.0525877503799,-64.9521016904873,
-64.8516156305946,-64.751919850902,-64.6523670279797,-64.5525584578631,
-64.4531847301558,-64.3538438133927,-64.2545052637224,-64.1543535645535,
-64.0548705868324,-63.9543845269397,-63.853898467047,-63.7542026873544,
-63.6546498644322,-63.5548412943156,-63.4554675666083,-63.3561266498452,
-63.2567881001749,-63.156636401006,-63.0571534232849,-62.9566673633921,
-62.8561813034994,-62.7564855238068,-62.6569327008845,-62.5571241307679,
-62.4577504030606,-62.3584094862975,-62.2590709366272,-62.1589192374583,
-62.0594362597372,-61.9589501998445,-61.8584641399518,-61.7587683602592,
-61.6592155373369,-61.5594069672203,-61.4600332395129,-61.3606923227499,
-61.2613537730796,-61.1612020739108,-61.0617190961896,-60.9612330362969,
-60.8607469764042,-60.7246295825628,-60.6402378352238),.UNSPECIFIED.);
#523=B_SPLINE_CURVE_WITH_KNOTS('',3,(#38861,#38862,#38863,#38864,#38865,
#38866,#38867,#38868,#38869,#38870,#38871,#38872,#38873,#38874,#38875,#38876,
#38877,#38878,#38879,#38880,#38881,#38882,#38883,#38884,#38885,#38886,#38887,
#38888,#38889,#38890,#38891,#38892,#38893,#38894,#38895,#38896,#38897,#38898,
#38899,#38900,#38901,#38902,#38903,#38904,#38905,#38906,#38907,#38908,#38909,
#38910,#38911,#38912,#38913,#38914,#38915,#38916,#38917,#38918,#38919,#38920,
#38921,#38922,#38923,#38924,#38925,#38926,#38927,#38928,#38929,#38930,#38931,
#38932,#38933,#38934,#38935,#38936,#38937,#38938,#38939,#38940,#38941,#38942,
#38943,#38944,#38945,#38946,#38947,#38948,#38949,#38950,#38951,#38952,#38953,
#38954,#38955,#38956,#38957,#38958,#38959,#38960,#38961,#38962,#38963,#38964,
#38965,#38966,#38967,#38968,#38969,#38970,#38971,#38972,#38973,#38974,#38975,
#38976,#38977,#38978,#38979,#38980,#38981,#38982,#38983,#38984,#38985,#38986,
#38987,#38988,#38989,#38990,#38991,#38992,#38993,#38994,#38995,#38996,#38997,
#38998,#38999,#39000,#39001,#39002,#39003,#39004,#39005,#39006,#39007,#39008,
#39009,#39010,#39011,#39012,#39013,#39014,#39015,#39016,#39017,#39018,#39019,
#39020,#39021,#39022,#39023,#39024,#39025,#39026,#39027,#39028,#39029,#39030,
#39031,#39032,#39033,#39034,#39035,#39036,#39037,#39038,#39039,#39040,#39041,
#39042,#39043,#39044,#39045,#39046,#39047,#39048,#39049,#39050),
 .UNSPECIFIED.,.F.,.F.,(4,3,3,3,3,3,3,3,3,3,3,3,3,3,3,3,3,3,3,3,3,3,3,3,
3,3,3,3,3,3,3,3,3,3,3,3,3,3,3,3,3,3,3,3,3,3,3,3,3,3,3,3,3,3,3,3,3,3,3,3,
3,3,3,4),(-60.6402378349658,-60.5421067500117,-60.4440484045844,-60.3460307800577,
-60.2480219114026,-60.1499231427379,-60.0517813064526,-59.9534650966384,
-59.8630298128566,-59.763334033164,-59.6637812102418,-59.5639726401252,
-59.4645989124179,-59.3652579956548,-59.2659194459845,-59.1657677468156,
-59.0662847690945,-58.9657987092017,-58.865312649309,-58.7656168696164,
-58.6660640466941,-58.5662554765775,-58.4668817488702,-58.3675408321072,
-58.2682022824368,-58.1680505832679,-58.0685676055468,-57.9680815456541,
-57.8675954857614,-57.7678997060687,-57.6683468831465,-57.5685383130299,
-57.4691645853226,-57.3698236685596,-57.2704851188893,-57.1703334197204,
-57.0708504419992,-56.9703643821065,-56.8698783222138,-56.7701825425212,
-56.6706297195989,-56.5708211494823,-56.4714474217751,-56.3721065050121,
-56.2727679553418,-56.1726162561729,-56.0731332784519,-55.9726472185591,
-55.8721611586662,-55.7724653789736,-55.6729125560515,-55.5731039859349,
-55.4737302582276,-55.3743893414644,-55.2750507917943,-55.1748990926253,
-55.0754161149041,-54.9749300550113,-54.8744439951185,-54.7704583063323,
-54.6667439665697,-54.5631892926208,-54.4598284734441,-54.3570525280442),
 .UNSPECIFIED.);
#524=B_SPLINE_CURVE_WITH_KNOTS('',3,(#39052,#39053,#39054,#39055,#39056,
#39057,#39058,#39059,#39060,#39061,#39062,#39063,#39064,#39065,#39066,#39067,
#39068,#39069,#39070,#39071,#39072,#39073,#39074,#39075,#39076,#39077,#39078,
#39079,#39080,#39081,#39082,#39083,#39084,#39085,#39086,#39087,#39088,#39089,
#39090,#39091,#39092,#39093,#39094,#39095,#39096,#39097,#39098,#39099,#39100,
#39101,#39102,#39103,#39104,#39105,#39106,#39107,#39108,#39109,#39110,#39111,
#39112,#39113,#39114,#39115,#39116,#39117,#39118,#39119,#39120,#39121,#39122,
#39123,#39124,#39125,#39126,#39127,#39128,#39129,#39130,#39131,#39132,#39133,
#39134,#39135,#39136,#39137,#39138,#39139,#39140,#39141,#39142,#39143,#39144,
#39145,#39146,#39147,#39148,#39149,#39150,#39151,#39152,#39153,#39154,#39155,
#39156,#39157,#39158,#39159,#39160,#39161,#39162,#39163,#39164,#39165,#39166,
#39167,#39168,#39169,#39170,#39171,#39172,#39173,#39174,#39175,#39176,#39177,
#39178,#39179,#39180,#39181,#39182,#39183,#39184,#39185,#39186,#39187,#39188,
#39189,#39190,#39191,#39192,#39193,#39194,#39195,#39196,#39197,#39198,#39199,
#39200,#39201,#39202,#39203,#39204,#39205,#39206,#39207,#39208,#39209,#39210,
#39211,#39212,#39213,#39214,#39215,#39216,#39217,#39218,#39219,#39220,#39221,
#39222,#39223,#39224,#39225,#39226,#39227,#39228,#39229,#39230,#39231,#39232,
#39233,#39234,#39235,#39236,#39237,#39238,#39239,#39240,#39241,#39242,#39243,
#39244),.UNSPECIFIED.,.F.,.F.,(4,3,3,3,3,3,3,3,3,3,3,3,3,3,3,3,3,3,3,3,
3,3,3,3,3,3,3,3,3,3,3,3,3,3,3,3,3,3,3,3,3,3,3,3,3,3,3,3,3,3,3,3,3,3,3,3,
3,3,3,3,3,3,3,3,4),(-54.3570525276504,-54.2521726206048,-54.1469650788617,
-54.0415854281849,-53.9359076806462,-53.8767268315709,-53.7770310518783,
-53.6774782289559,-53.5776696588393,-53.4782959311319,-53.3789550143688,
-53.2796164646985,-53.1794647655297,-53.0799817878085,-52.9794957279159,
-52.8790096680233,-52.7793138883307,-52.6797610654085,-52.5799524952919,
-52.4805787675846,-52.3812378508216,-52.2818993011513,-52.1817476019824,
-52.0822646242613,-51.9817785643685,-51.8812925044757,-51.7815967247831,
-51.6820439018608,-51.5822353317442,-51.4828616040369,-51.3835206872739,
-51.2841821376035,-51.1840304384347,-51.0845474607135,-50.9840614008208,
-50.8835753409281,-50.7838795612355,-50.6843267383132,-50.5845181681966,
-50.4851444404893,-50.3858035237262,-50.2864649740559,-50.1863132748871,
-50.0868302971659,-49.9863442372732,-49.8858581773805,-49.7861623976879,
-49.6866095747656,-49.5868010046491,-49.4874272769417,-49.3880863601787,
-49.2887478105084,-49.1885961113395,-49.0891131336184,-48.9886270737257,
-48.8881410138329,-48.7863567897428,-48.6883018854676,-48.5903387778308,
-48.4924352823033,-48.3945592942371,-48.2966378664563,-48.1986884936107,
-48.1006313286397,-48.0738672211117),.UNSPECIFIED.);
#525=B_SPLINE_CURVE_WITH_KNOTS('',3,(#39246,#39247,#39248,#39249,#39250,
#39251,#39252,#39253,#39254,#39255,#39256,#39257,#39258,#39259,#39260,#39261,
#39262,#39263,#39264,#39265,#39266,#39267,#39268,#39269,#39270,#39271,#39272,
#39273,#39274,#39275,#39276,#39277,#39278,#39279,#39280,#39281,#39282,#39283,
#39284,#39285,#39286,#39287,#39288,#39289,#39290,#39291,#39292,#39293,#39294,
#39295,#39296,#39297,#39298,#39299,#39300,#39301,#39302,#39303,#39304,#39305,
#39306,#39307,#39308,#39309,#39310,#39311,#39312,#39313,#39314,#39315,#39316,
#39317,#39318,#39319,#39320,#39321,#39322,#39323,#39324,#39325,#39326,#39327,
#39328,#39329,#39330,#39331,#39332,#39333,#39334,#39335,#39336,#39337,#39338,
#39339,#39340,#39341,#39342,#39343,#39344,#39345,#39346,#39347,#39348,#39349,
#39350,#39351,#39352,#39353,#39354,#39355,#39356,#39357,#39358,#39359,#39360,
#39361,#39362,#39363,#39364,#39365,#39366,#39367,#39368,#39369,#39370,#39371,
#39372,#39373,#39374,#39375,#39376,#39377,#39378,#39379,#39380,#39381,#39382,
#39383,#39384,#39385,#39386,#39387,#39388,#39389,#39390,#39391,#39392,#39393,
#39394,#39395,#39396,#39397,#39398,#39399,#39400,#39401,#39402,#39403,#39404,
#39405,#39406,#39407,#39408,#39409,#39410,#39411,#39412,#39413,#39414,#39415,
#39416,#39417,#39418,#39419,#39420,#39421,#39422,#39423,#39424,#39425,#39426,
#39427,#39428,#39429,#39430,#39431,#39432,#39433,#39434,#39435),
 .UNSPECIFIED.,.F.,.F.,(4,3,3,3,3,3,3,3,3,3,3,3,3,3,3,3,3,3,3,3,3,3,3,3,
3,3,3,3,3,3,3,3,3,3,3,3,3,3,3,3,3,3,3,3,3,3,3,3,3,3,3,3,3,3,3,3,3,3,3,3,
3,3,3,4),(-48.0738672208646,-47.9246215794861,-47.8904238502853,-47.790728070593,
-47.6911752476712,-47.5913666775545,-47.4919929498476,-47.3926520330849,
-47.2933134834149,-47.1931617842456,-47.0936788065248,-46.9931927466313,
-46.8927066867377,-46.7930109070449,-46.6934580841225,-46.5936495140059,
-46.4942757862985,-46.3949348695353,-46.2955963198648,-46.1954446206961,
-46.0959616429748,-45.9954755830824,-45.89498952319,-45.7952937434974,-45.6957409205751,
-45.5959323504585,-45.4965586227512,-45.3972177059881,-45.2978791563177,
-45.1977274571489,-45.0982444794277,-44.9977584195351,-44.8972723596424,
-44.7975765799498,-44.6980237570276,-44.598215186911,-44.4988414592038,
-44.3995005424408,-44.3001619927705,-44.2000102936016,-44.1005273158805,
-44.0000412559877,-43.8995551960948,-43.7998594164022,-43.7003065934799,
-43.6004980233633,-43.501124295656,-43.4017833788929,-43.3024448292225,
-43.2022931300537,-43.1028101523325,-43.0023240924398,-42.9018380325472,
-42.8021422528546,-42.7025894299324,-42.6027808598158,-42.5034071321085,
-42.4040662153454,-42.304727665675,-42.2045759665062,-42.105092988785,-42.0046069288923,
-41.9041208689996,-41.790681913685),.UNSPECIFIED.);
#526=B_SPLINE_CURVE_WITH_KNOTS('',3,(#39437,#39438,#39439,#39440,#39441,
#39442,#39443,#39444,#39445,#39446,#39447,#39448,#39449,#39450,#39451,#39452,
#39453,#39454,#39455,#39456,#39457,#39458,#39459,#39460,#39461,#39462,#39463,
#39464,#39465,#39466,#39467,#39468,#39469,#39470,#39471,#39472,#39473,#39474,
#39475,#39476,#39477,#39478,#39479,#39480,#39481,#39482,#39483,#39484,#39485,
#39486,#39487,#39488,#39489,#39490,#39491,#39492,#39493,#39494,#39495,#39496,
#39497,#39498,#39499,#39500,#39501,#39502,#39503,#39504,#39505,#39506,#39507,
#39508,#39509,#39510,#39511,#39512,#39513,#39514,#39515,#39516,#39517,#39518,
#39519,#39520,#39521,#39522,#39523,#39524,#39525,#39526,#39527,#39528,#39529,
#39530,#39531,#39532,#39533,#39534,#39535,#39536,#39537,#39538,#39539,#39540,
#39541,#39542,#39543,#39544,#39545,#39546,#39547,#39548,#39549,#39550,#39551,
#39552,#39553,#39554,#39555,#39556,#39557,#39558,#39559,#39560,#39561,#39562,
#39563,#39564,#39565,#39566,#39567,#39568,#39569,#39570,#39571,#39572,#39573,
#39574,#39575,#39576,#39577,#39578,#39579,#39580,#39581,#39582,#39583,#39584,
#39585,#39586,#39587,#39588,#39589,#39590,#39591,#39592,#39593,#39594,#39595,
#39596,#39597,#39598,#39599,#39600,#39601,#39602,#39603,#39604,#39605,#39606,
#39607,#39608,#39609,#39610,#39611,#39612,#39613,#39614,#39615,#39616,#39617,
#39618,#39619,#39620,#39621,#39622,#39623,#39624,#39625,#39626),
 .UNSPECIFIED.,.F.,.F.,(4,3,3,3,3,3,3,3,3,3,3,3,3,3,3,3,3,3,3,3,3,3,3,3,
3,3,3,3,3,3,3,3,3,3,3,3,3,3,3,3,3,3,3,3,3,3,3,3,3,3,3,3,3,3,3,3,3,3,3,3,
3,3,3,4),(-41.790681913461,-41.692389330571,-41.5941411274311,-41.4960606609849,
-41.3980237415933,-41.299998413901,-41.2015997367888,-41.1034458577189,
-41.0049247815855,-40.906403705452,-40.8067079257594,-40.7071551028373,
-40.6073465327207,-40.5079728050133,-40.4086318882502,-40.3092933385798,
-40.209141639411,-40.1096586616898,-40.0091726017971,-39.9086865419044,
-39.8089907622117,-39.7094379392893,-39.6096293691727,-39.5102556414654,
-39.4109147247024,-39.3115761750321,-39.2114244758632,-39.1119414981421,
-39.0114554382495,-38.9109693783568,-38.8112735986641,-38.7117207757417,
-38.6119122056251,-38.5125384779178,-38.4131975611546,-38.3138590114842,
-38.2137073123155,-38.1142243345942,-38.0137382747017,-37.9132522148092,
-37.8135564351165,-37.714003612194,-37.6141950420775,-37.5148213143702,
-37.4154803976071,-37.3161418479371,-37.2159901487682,-37.116507171047,
-37.0160211111543,-36.9155350512616,-36.8158392715691,-36.716286448647,
-36.6164778785303,-36.5171041508231,-36.41776323406,-36.3184246843897,-36.2182729852208,
-36.1187900074996,-36.0183039476068,-35.917817887714,-35.8079248438542,
-35.6983489447371,-35.5893126975054,-35.5074966068976),.UNSPECIFIED.);
#527=B_SPLINE_CURVE_WITH_KNOTS('',3,(#39628,#39629,#39630,#39631,#39632,
#39633,#39634,#39635,#39636,#39637,#39638,#39639,#39640,#39641,#39642,#39643,
#39644,#39645,#39646,#39647,#39648,#39649,#39650,#39651,#39652,#39653,#39654,
#39655,#39656,#39657,#39658,#39659,#39660,#39661,#39662,#39663,#39664,#39665,
#39666,#39667,#39668,#39669,#39670,#39671,#39672,#39673,#39674,#39675,#39676,
#39677,#39678,#39679,#39680,#39681,#39682,#39683,#39684,#39685,#39686,#39687,
#39688,#39689,#39690,#39691,#39692,#39693,#39694,#39695,#39696,#39697,#39698,
#39699,#39700,#39701,#39702,#39703,#39704,#39705,#39706,#39707,#39708,#39709,
#39710,#39711,#39712,#39713,#39714,#39715,#39716,#39717,#39718,#39719,#39720,
#39721,#39722,#39723,#39724,#39725,#39726,#39727,#39728,#39729,#39730,#39731,
#39732,#39733,#39734,#39735,#39736,#39737,#39738,#39739,#39740,#39741,#39742,
#39743,#39744,#39745,#39746,#39747,#39748,#39749,#39750,#39751,#39752,#39753,
#39754,#39755,#39756,#39757,#39758,#39759,#39760,#39761,#39762,#39763,#39764,
#39765,#39766,#39767,#39768,#39769,#39770,#39771,#39772,#39773,#39774,#39775,
#39776,#39777,#39778,#39779,#39780,#39781,#39782,#39783,#39784,#39785,#39786,
#39787,#39788,#39789,#39790,#39791,#39792,#39793,#39794,#39795,#39796,#39797,
#39798,#39799,#39800,#39801,#39802,#39803,#39804,#39805,#39806,#39807,#39808,
#39809,#39810,#39811,#39812,#39813,#39814,#39815,#39816,#39817,#39818,#39819,
#39820),.UNSPECIFIED.,.F.,.F.,(4,3,3,3,3,3,3,3,3,3,3,3,3,3,3,3,3,3,3,3,
3,3,3,3,3,3,3,3,3,3,3,3,3,3,3,3,3,3,3,3,3,3,3,3,3,3,3,3,3,3,3,3,3,3,3,3,
3,3,3,3,3,3,3,3,4),(-35.5074966065054,-35.4065248779729,-35.305509076606,
-35.2043396116514,-35.1030905086744,-35.001630744129,-34.9201007241663,
-34.8204049444737,-34.7208521215515,-34.6210435514349,-34.5216698237276,
-34.4223289069646,-34.3229903572942,-34.2228386581253,-34.1233556804042,
-34.0228696205115,-33.9223835606187,-33.8226877809265,-33.7231349580045,
-33.6233263878879,-33.5239526601809,-33.4246117434182,-33.3252731937481,
-33.2251214945789,-33.1256385168581,-33.0251524569646,-32.9246663970711,
-32.8249706173775,-32.7254177944543,-32.625609224338,-32.5262354966298,
-32.4268945798657,-32.3275560301946,-32.2274043310268,-32.1279213533048,
-32.0274352934141,-31.9269492335235,-31.8272534538316,-31.7277006309103,
-31.6278920607935,-31.528518333087,-31.4291774163247,-31.3298388666551,
-31.2296871674853,-31.1302041897648,-31.0297181298704,-30.9292320699759,
-30.829536290285,-30.7299834673647,-30.6301748972477,-30.530801169542,-30.4314602527805,
-30.332121703112,-30.2319700039411,-30.1324870262215,-30.0320009663249,
-29.9315149064283,-29.8325486555065,-29.7337156387982,-29.6349843102171,
-29.5323160574943,-29.4336769479537,-29.3350464532442,-29.2363682515395,
-29.2243112993258),.UNSPECIFIED.);
#528=B_SPLINE_CURVE_WITH_KNOTS('',3,(#39822,#39823,#39824,#39825,#39826,
#39827,#39828,#39829,#39830,#39831,#39832,#39833,#39834,#39835,#39836,#39837,
#39838,#39839,#39840,#39841,#39842,#39843,#39844,#39845,#39846,#39847,#39848,
#39849,#39850,#39851,#39852,#39853,#39854,#39855,#39856,#39857,#39858,#39859,
#39860,#39861,#39862,#39863,#39864,#39865,#39866,#39867,#39868,#39869,#39870,
#39871,#39872,#39873,#39874,#39875,#39876,#39877,#39878,#39879,#39880,#39881,
#39882,#39883,#39884,#39885,#39886,#39887,#39888,#39889,#39890,#39891,#39892,
#39893,#39894,#39895,#39896,#39897,#39898,#39899,#39900,#39901,#39902,#39903,
#39904,#39905,#39906,#39907,#39908,#39909,#39910,#39911,#39912,#39913,#39914,
#39915,#39916,#39917,#39918,#39919,#39920,#39921,#39922,#39923,#39924,#39925,
#39926,#39927,#39928,#39929,#39930,#39931,#39932,#39933,#39934,#39935,#39936,
#39937,#39938,#39939,#39940,#39941,#39942,#39943,#39944,#39945,#39946,#39947,
#39948,#39949,#39950,#39951,#39952,#39953,#39954,#39955,#39956,#39957,#39958,
#39959,#39960,#39961,#39962,#39963,#39964,#39965,#39966,#39967,#39968,#39969,
#39970,#39971,#39972,#39973,#39974,#39975,#39976,#39977,#39978,#39979,#39980,
#39981,#39982,#39983,#39984,#39985,#39986,#39987,#39988,#39989,#39990,#39991,
#39992,#39993,#39994,#39995,#39996,#39997,#39998,#39999,#40000,#40001,#40002,
#40003,#40004,#40005,#40006,#40007,#40008,#40009,#40010,#40011,#40012,#40013,
#40014),.UNSPECIFIED.,.F.,.F.,(4,3,3,3,3,3,3,3,3,3,3,3,3,3,3,3,3,3,3,3,
3,3,3,3,3,3,3,3,3,3,3,3,3,3,3,3,3,3,3,3,3,3,3,3,3,3,3,3,3,3,3,3,3,3,3,3,
3,3,3,3,3,3,3,3,4),(-29.2243112990236,-29.103492898179,-28.9808497567486,
-28.9337977428807,-28.8341019631958,-28.7345491402811,-28.6347405701626,
-28.5353668424629,-28.4360259257073,-28.3366873760444,-28.2365356768666,
-28.1370526991525,-28.0365666392428,-27.9360805793331,-27.8363847996496,
-27.7368319767364,-27.6370234066176,-27.5376496789196,-27.438308762166,
-27.3389702125051,-27.2388185133252,-27.1393355356136,-27.0388494756995,
-26.9383634157855,-26.8386676360441,-26.7391148130729,-26.6393062429686,
-26.5399325152125,-26.4405915984007,-26.3412530486819,-26.2411013495709,
-26.1416183718023,-26.0411323120201,-25.9406462522379,-25.8409504726143,
-25.7413976497608,-25.641589079627,-25.5422153519875,-25.4428744352918,
-25.3435358856882,-25.2433841864387,-25.1439012087821,-25.0434151487361,
-24.9429290886902,-24.8432333090377,-24.7436804861565,-24.6438719160297,
-24.5444981883652,-24.4451572716455,-24.345818722019,-24.2456670227999,
-24.1461840451234,-24.045697985133,-23.9452119251426,-23.8455161451008,
-23.7459633218283,-23.6461547517991,-23.5467810237416,-23.447440106629,
-23.3481015566104,-23.2479498578566,-23.1484668797938,-23.0479808206944,
-22.947494761595,-22.9411259921462),.UNSPECIFIED.);
#529=B_SPLINE_CURVE_WITH_KNOTS('',3,(#40016,#40017,#40018,#40019,#40020,
#40021,#40022,#40023,#40024,#40025,#40026,#40027,#40028,#40029,#40030,#40031,
#40032,#40033,#40034,#40035,#40036,#40037,#40038,#40039,#40040,#40041,#40042,
#40043,#40044,#40045,#40046,#40047,#40048,#40049,#40050,#40051,#40052,#40053,
#40054,#40055,#40056,#40057,#40058,#40059,#40060,#40061,#40062,#40063,#40064,
#40065,#40066,#40067,#40068,#40069,#40070,#40071,#40072,#40073,#40074,#40075,
#40076,#40077,#40078,#40079,#40080,#40081,#40082,#40083,#40084,#40085,#40086,
#40087,#40088,#40089,#40090,#40091,#40092,#40093,#40094,#40095,#40096,#40097,
#40098,#40099,#40100,#40101,#40102,#40103,#40104,#40105,#40106,#40107,#40108,
#40109,#40110,#40111,#40112,#40113,#40114,#40115,#40116,#40117,#40118,#40119,
#40120,#40121,#40122,#40123,#40124,#40125,#40126,#40127,#40128,#40129,#40130,
#40131,#40132,#40133,#40134,#40135,#40136,#40137,#40138,#40139,#40140,#40141,
#40142,#40143,#40144,#40145,#40146,#40147,#40148,#40149,#40150,#40151,#40152,
#40153,#40154,#40155,#40156,#40157,#40158,#40159,#40160,#40161,#40162,#40163,
#40164,#40165,#40166,#40167,#40168,#40169,#40170,#40171,#40172,#40173,#40174,
#40175,#40176,#40177,#40178,#40179,#40180,#40181,#40182,#40183,#40184,#40185,
#40186,#40187,#40188,#40189,#40190,#40191,#40192,#40193,#40194,#40195,#40196,
#40197,#40198,#40199,#40200,#40201,#40202,#40203,#40204,#40205),
 .UNSPECIFIED.,.F.,.F.,(4,3,3,3,3,3,3,3,3,3,3,3,3,3,3,3,3,3,3,3,3,3,3,3,
3,3,3,3,3,3,3,3,3,3,3,3,3,3,3,3,3,3,3,3,3,3,3,3,3,3,3,3,3,3,3,3,3,3,3,3,
3,3,3,4),(-22.9411259917746,-22.8415435429852,-22.7421039011161,-22.6427792851694,
-22.5435176208825,-22.4442882702793,-22.3450606352053,-22.2457348632547,
-22.1463622498412,-22.0468091209728,-21.9497775980474,-21.850081818445,
-21.7505289956196,-21.6507204254796,-21.5513466978833,-21.4520057812365,
-21.3526672316874,-21.2525155323905,-21.1530325548013,-21.0525464946505,
-20.9520604344998,-20.8523646523694,-20.7528118270002,-20.6530032574942,
-20.5536295273353,-20.4542886081243,-20.3549500560131,-20.2547983597479,
-20.1553153796278,-20.05482932529,-19.9543432709522,-19.8546474960847,-19.7550946779828,
-19.6552861066605,-19.5559123837282,-19.4565714717126,-19.3572329267559,
-19.2570812219181,-19.1575982487803,-19.0571121780925,-18.9566261074046,
-18.8569303268034,-18.7573775030175,-18.6575689331224,-18.5581952046655,
-18.4588542871971,-18.3595157368665,-18.2593640386141,-18.1598810603482,
-18.0593950021026,-17.958908943857,-17.8592131476343,-17.759660308104,-17.6598517421297,
-17.560477997747,-17.4611370643201,-17.3617984980203,-17.2616468185926,
-17.1621638244946,-17.061677802402,-16.9611917803094,-16.8403231294146,
-16.7210048959573,-16.6579408702691),.UNSPECIFIED.);
#530=B_SPLINE_CURVE_WITH_KNOTS('',3,(#40207,#40208,#40209,#40210,#40211,
#40212,#40213,#40214,#40215,#40216),.UNSPECIFIED.,.F.,.F.,(4,1,1,1,1,1,
1,4),(-16.6579406849666,-15.9634746167618,-14.9657574532142,-13.9680402896665,
-12.9703231261189,-11.9726059625713,-10.9748887990237,-10.374755377787),
 .UNSPECIFIED.);
#531=B_SPLINE_CURVE_WITH_KNOTS('',3,(#40217,#40218,#40219,#40220,#40221,
#40222,#40223,#40224,#40225,#40226,#40227,#40228,#40229,#40230,#40231,#40232,
#40233,#40234,#40235,#40236,#40237,#40238,#40239,#40240,#40241,#40242,#40243,
#40244,#40245,#40246,#40247,#40248,#40249,#40250,#40251,#40252,#40253,#40254,
#40255,#40256,#40257,#40258,#40259,#40260,#40261,#40262,#40263,#40264,#40265,
#40266,#40267,#40268,#40269,#40270,#40271,#40272,#40273,#40274,#40275,#40276,
#40277,#40278,#40279,#40280,#40281,#40282,#40283,#40284,#40285,#40286,#40287,
#40288,#40289,#40290,#40291,#40292,#40293,#40294,#40295,#40296,#40297,#40298,
#40299,#40300,#40301,#40302,#40303,#40304,#40305,#40306,#40307,#40308,#40309,
#40310,#40311,#40312,#40313,#40314,#40315,#40316,#40317,#40318,#40319,#40320,
#40321,#40322,#40323,#40324,#40325,#40326,#40327,#40328,#40329,#40330,#40331,
#40332,#40333,#40334,#40335,#40336,#40337,#40338,#40339,#40340,#40341,#40342,
#40343,#40344,#40345,#40346,#40347,#40348,#40349,#40350,#40351,#40352,#40353,
#40354,#40355,#40356,#40357,#40358,#40359,#40360,#40361,#40362,#40363,#40364,
#40365,#40366,#40367,#40368,#40369,#40370,#40371,#40372,#40373,#40374,#40375,
#40376,#40377,#40378,#40379,#40380,#40381,#40382,#40383,#40384,#40385,#40386,
#40387,#40388,#40389,#40390,#40391,#40392,#40393,#40394,#40395,#40396,#40397,
#40398,#40399,#40400,#40401,#40402,#40403,#40404,#40405,#40406),
 .UNSPECIFIED.,.F.,.F.,(4,3,3,3,3,3,3,3,3,3,3,3,3,3,3,3,3,3,3,3,3,3,3,3,
3,3,3,3,3,3,3,3,3,3,3,3,3,3,3,3,3,3,3,3,3,3,3,3,3,3,3,3,3,3,3,3,3,3,3,3,
3,3,3,4),(-10.374755156708,-10.2647876514522,-10.1544297250587,-10.0435333536381,
-9.9771716354761,-9.8774735922054,-9.77791851937864,-9.67811051344737,-9.5787345848517,
-9.47939149034969,-9.38005078887961,-9.27990170964183,-9.18041666501551,
-9.079935568472,-8.97945447192849,-8.87975475068599,-8.78019794692404,-8.68039036710614,
-8.5810125929777,-8.48166761426253,-8.38232499271131,-8.2821780716287,-8.18269103968926,
-8.08221417403507,-7.98173730838088,-7.88205853932025,-7.78252275788716,
-7.68270993125542,-7.58335319660954,-7.48402921742459,-7.38470752738062,
-7.28453568174378,-7.18506920224763,-7.08454467354045,-6.98402014483327,
-6.88430333738403,-6.78472957127026,-6.68492624752219,-6.58553193070912,
-6.48617060257183,-6.38681184575184,-6.2866846296353,-6.18718214676953,
-6.08674256402759,-5.98630298128566,-5.88658666295721,-5.78701300292329,
-5.68720960477514,-5.58781447444025,-5.48845199143677,-5.38909174229588,
-5.28896526115642,-5.18946048386327,-5.08902315080066,-4.98858581773805,
-4.89025187082946,-4.79041664580171,-4.69233891542646,-4.59432039421673,
-4.49632908436476,-4.39513933092544,-4.29705324421013,-4.1943116574088,
-4.09157007060747),.UNSPECIFIED.);
#532=B_SPLINE_CURVE_WITH_KNOTS('',3,(#40409,#40410,#40411,#40412,#40413),
 .UNSPECIFIED.,.F.,.F.,(4,1,4),(158.568767222197,159.278533402388,160.221218674128),
 .UNSPECIFIED.);
#533=B_SPLINE_CURVE_WITH_KNOTS('',3,(#40415,#40416,#40417,#40418,#40419,
#40420,#40421,#40422,#40423,#40424,#40425,#40426,#40427,#40428,#40429,#40430,
#40431,#40432,#40433,#40434,#40435,#40436,#40437,#40438,#40439,#40440,#40441,
#40442,#40443,#40444,#40445,#40446,#40447,#40448,#40449,#40450,#40451,#40452,
#40453,#40454,#40455,#40456,#40457,#40458,#40459,#40460,#40461,#40462,#40463,
#40464,#40465,#40466,#40467,#40468,#40469,#40470,#40471,#40472,#40473,#40474,
#40475,#40476,#40477,#40478,#40479,#40480,#40481,#40482,#40483,#40484,#40485,
#40486,#40487,#40488,#40489,#40490,#40491,#40492,#40493,#40494,#40495,#40496,
#40497,#40498,#40499,#40500,#40501,#40502,#40503,#40504,#40505),
 .UNSPECIFIED.,.F.,.F.,(4,3,3,3,3,3,3,3,3,3,3,3,3,3,3,3,3,3,3,3,3,3,3,3,
3,3,3,3,3,3,4),(160.221225333079,160.276250565935,160.381079054541,160.485749756296,
160.590297379016,160.694779341089,160.799231394165,160.90368924618,161.008259430969,
161.112891606325,161.217708400402,161.273967729483,161.379121029899,161.484116312145,
161.588986618703,161.693789907966,161.798561461836,161.903336516804,162.008218273126,
162.113159280045,162.218277378404,162.271684893031,162.375628464312,162.479397941196,
162.583070245111,162.686682340639,162.790271110867,162.893943190511,162.997653572182,
163.101547205486,163.19821022681),.UNSPECIFIED.);
#534=B_SPLINE_CURVE_WITH_KNOTS('',3,(#40509,#40510,#40511,#40512,#40513,
#40514,#40515,#40516,#40517,#40518,#40519,#40520,#40521,#40522,#40523,#40524,
#40525,#40526,#40527,#40528,#40529,#40530,#40531,#40532,#40533,#40534,#40535,
#40536,#40537,#40538,#40539,#40540,#40541,#40542,#40543,#40544,#40545,#40546,
#40547,#40548,#40549,#40550,#40551,#40552,#40553,#40554,#40555,#40556,#40557,
#40558,#40559,#40560,#40561,#40562,#40563),.UNSPECIFIED.,.F.,.F.,(4,3,3,
3,3,3,3,3,3,3,3,3,3,3,3,3,3,3,4),(160.221225333079,160.323576356247,160.425868943639,
160.528141137588,160.6304309436,160.732846323553,160.835338090606,160.93801420435,
160.958883749947,161.066718047386,161.17795340565,161.285428499209,161.392801978492,
161.500102932275,161.607360355761,161.714633268257,161.821914162531,161.929269085492,
161.956600913495),.UNSPECIFIED.);
#535=B_SPLINE_CURVE_WITH_KNOTS('',3,(#40564,#40565,#40566,#40567,#40568,
#40569,#40570,#40571,#40572,#40573,#40574,#40575,#40576,#40577,#40578,#40579,
#40580,#40581,#40582,#40583,#40584,#40585,#40586,#40587,#40588,#40589,#40590,
#40591,#40592,#40593,#40594,#40595,#40596,#40597,#40598,#40599,#40600,#40601,
#40602,#40603,#40604,#40605,#40606,#40607,#40608,#40609,#40610,#40611,#40612),
 .UNSPECIFIED.,.F.,.F.,(4,3,3,3,3,3,3,3,3,3,3,3,3,3,3,3,4),(158.567664456021,
158.672535944769,158.777458396884,158.882566263536,158.963449422852,159.068511569472,
159.173418639729,159.278205451186,159.382928208473,159.487622287813,159.592323023176,
159.697135689129,159.8020104782,159.907067470358,159.961166586399,160.094360320626,
160.221225332746),.UNSPECIFIED.);
#536=B_SPLINE_CURVE_WITH_KNOTS('',3,(#40617,#40618,#40619,#40620,#40621,
#40622,#40623,#40624,#40625,#40626,#40627,#40628,#40629,#40630,#40631,#40632,
#40633,#40634,#40635,#40636,#40637,#40638,#40639,#40640,#40641,#40642,#40643,
#40644,#40645,#40646,#40647,#40648,#40649,#40650,#40651,#40652,#40653,#40654,
#40655,#40656,#40657,#40658,#40659,#40660,#40661,#40662,#40663,#40664,#40665,
#40666,#40667,#40668,#40669,#40670,#40671,#40672,#40673,#40674,#40675,#40676,
#40677,#40678,#40679,#40680,#40681,#40682,#40683,#40684,#40685,#40686,#40687,
#40688,#40689,#40690,#40691,#40692,#40693,#40694,#40695,#40696,#40697,#40698,
#40699,#40700,#40701,#40702,#40703,#40704),.UNSPECIFIED.,.F.,.F.,(4,3,3,
3,3,3,3,3,3,3,3,3,3,3,3,3,3,3,3,3,3,3,3,3,3,3,3,3,3,4),(-0.457078985060659,
-0.444385276561842,-0.418760344151197,-0.405811846153069,-0.39886744604032,
-0.394362276912132,-0.368978176374782,-0.349303253656113,-0.340015563076288,
-0.335861856280851,-0.331696484383836,-0.306965526627292,-0.282519434519426,
-0.258814906883348,-0.248499275797862,-0.244444801260351,-0.220954016702682,
-0.211584376181149,-0.187623099299552,-0.164170211887108,-0.158777333143535,
-0.135446414563357,-0.112194632335021,-0.0891371093918709,-0.0803323653505391,
-0.0766178985924528,-0.0541145820763493,-0.0322395508690489,-0.010671129319354,
0.),.UNSPECIFIED.);
#537=B_SPLINE_CURVE_WITH_KNOTS('',3,(#40705,#40706,#40707,#40708,#40709,
#40710,#40711,#40712,#40713,#40714,#40715,#40716,#40717,#40718,#40719,#40720,
#40721,#40722,#40723,#40724,#40725,#40726,#40727,#40728,#40729,#40730,#40731,
#40732,#40733,#40734,#40735,#40736,#40737,#40738,#40739,#40740,#40741,#40742,
#40743,#40744,#40745,#40746,#40747,#40748,#40749,#40750,#40751,#40752,#40753,
#40754,#40755,#40756,#40757,#40758,#40759,#40760,#40761,#40762,#40763,#40764,
#40765,#40766,#40767,#40768,#40769,#40770,#40771,#40772,#40773,#40774,#40775,
#40776,#40777,#40778,#40779,#40780,#40781,#40782,#40783,#40784,#40785,#40786,
#40787,#40788,#40789),.UNSPECIFIED.,.F.,.F.,(4,3,3,3,3,3,3,3,3,3,3,3,3,
3,3,3,3,3,3,3,3,3,3,3,3,3,3,3,4),(-0.463803050843693,-0.449398219400782,
-0.427690690340653,-0.415681595796131,-0.410727534513478,-0.405863614198107,
-0.383202928459213,-0.364728962044393,-0.357056800645003,-0.352630059545498,
-0.329188375163953,-0.305452986562277,-0.281845294580705,-0.274917746668043,
-0.270966521906024,-0.246538221694511,-0.235545177628289,-0.211713588834806,
-0.187882000041323,-0.183828909444003,-0.159579091238228,-0.134520943597755,
-0.109462795957281,-0.0941651274920544,-0.0900064894898221,-0.0642581539445237,
-0.0384830703539072,-0.01326410743577,0.),.UNSPECIFIED.);
#538=B_SPLINE_CURVE_WITH_KNOTS('',3,(#41419,#41420,#41421,#41422),
 .UNSPECIFIED.,.F.,.F.,(4,4),(-0.0473137948812196,0.),.UNSPECIFIED.);
#539=B_SPLINE_CURVE_WITH_KNOTS('',3,(#41424,#41425,#41426,#41427,#41428,
#41429,#41430,#41431,#41432,#41433,#41434,#41435,#41436,#41437,#41438,#41439,
#41440,#41441,#41442,#41443,#41444,#41445,#41446,#41447,#41448,#41449,#41450,
#41451,#41452,#41453,#41454,#41455,#41456,#41457,#41458,#41459,#41460,#41461,
#41462,#41463,#41464,#41465,#41466,#41467,#41468,#41469,#41470,#41471,#41472,
#41473,#41474,#41475,#41476,#41477,#41478,#41479,#41480,#41481,#41482,#41483,
#41484,#41485,#41486,#41487,#41488,#41489,#41490,#41491,#41492,#41493,#41494,
#41495,#41496,#41497,#41498,#41499,#41500,#41501,#41502,#41503,#41504,#41505,
#41506,#41507,#41508),.UNSPECIFIED.,.F.,.F.,(4,3,3,3,3,3,3,3,3,3,3,3,3,
3,3,3,3,3,3,3,3,3,3,3,3,3,3,3,4),(-0.463803050843679,-0.44939821940076,
-0.427589341418366,-0.415681597634893,-0.410727519266437,-0.405863611030377,
-0.38318378630743,-0.360186208150004,-0.357056795907073,-0.352630060245515,
-0.329269893234261,-0.305500004932649,-0.288041937515757,-0.274917747543885,
-0.270966522774074,-0.246538222518605,-0.23554517762827,-0.211959515268067,
-0.18788200185284,-0.183828910437428,-0.159579093158968,-0.134520946152716,
-0.109462799146463,-0.0941651345645707,-0.0900064900507649,-0.0642581550076631,
-0.0384830708873975,-0.0132641052952493,0.),.UNSPECIFIED.);
#540=B_SPLINE_CURVE_WITH_KNOTS('',3,(#41509,#41510,#41511,#41512),
 .UNSPECIFIED.,.F.,.F.,(4,4),(-0.0138026843193199,0.),.UNSPECIFIED.);
#541=B_SPLINE_CURVE_WITH_KNOTS('',3,(#41517,#41518,#41519,#41520,#41521,
#41522,#41523,#41524,#41525,#41526,#41527,#41528,#41529,#41530,#41531,#41532,
#41533,#41534,#41535,#41536,#41537,#41538,#41539,#41540,#41541,#41542,#41543,
#41544,#41545,#41546,#41547,#41548,#41549,#41550,#41551,#41552,#41553,#41554,
#41555,#41556,#41557,#41558,#41559,#41560,#41561,#41562,#41563,#41564,#41565,
#41566,#41567,#41568,#41569,#41570,#41571,#41572,#41573,#41574,#41575,#41576,
#41577,#41578,#41579,#41580,#41581,#41582,#41583,#41584,#41585,#41586,#41587,
#41588,#41589,#41590,#41591,#41592,#41593,#41594,#41595,#41596,#41597,#41598,
#41599,#41600,#41601,#41602,#41603,#41604),.UNSPECIFIED.,.F.,.F.,(4,3,3,
3,3,3,3,3,3,3,3,3,3,3,3,3,3,3,3,3,3,3,3,3,3,3,3,3,3,4),(-0.457078999239372,
-0.444385276561864,-0.418678196115324,-0.405811846078769,-0.398867444205902,
-0.394362273327402,-0.368978172738963,-0.349303250493666,-0.340015558281466,
-0.335861852484767,-0.331696483073541,-0.306947318623066,-0.2827283572022,
-0.259025657312411,-0.248499263812912,-0.244444801048436,-0.220954014795881,
-0.211584376181152,-0.18752381564345,-0.164170210903559,-0.158777333342259,
-0.135446414038975,-0.112194633282033,-0.0891371124572476,-0.0803323657407222,
-0.076617898847751,-0.0541145839112134,-0.0322395556953983,-0.0106711375989012,
0.),.UNSPECIFIED.);
#542=B_SPLINE_CURVE_WITH_KNOTS('',3,(#42234,#42235,#42236,#42237),
 .UNSPECIFIED.,.F.,.F.,(4,4),(-0.0475340594435537,0.),.UNSPECIFIED.);
#817=SHAPE_REPRESENTATION_RELATIONSHIP('SRR','None',#81136,#827);
#827=ADVANCED_BREP_SHAPE_REPRESENTATION('',(#847),#81036);
#837=STYLED_ITEM('',(#81195),#847);
#847=MANIFOLD_SOLID_BREP('Body1',#15090);
#991=CYLINDRICAL_SURFACE('',#16086,1.99475);
#992=CYLINDRICAL_SURFACE('',#16088,1.99475);
#993=CYLINDRICAL_SURFACE('',#16089,1.99475);
#994=CYLINDRICAL_SURFACE('',#16090,1.99475);
#995=CYLINDRICAL_SURFACE('',#16091,1.99475);
#996=CYLINDRICAL_SURFACE('',#16092,1.99475);
#997=CYLINDRICAL_SURFACE('',#16093,1.99475);
#998=CYLINDRICAL_SURFACE('',#16094,1.99475);
#999=CYLINDRICAL_SURFACE('',#16095,1.99475);
#1000=CYLINDRICAL_SURFACE('',#16096,1.99475);
#1001=CYLINDRICAL_SURFACE('',#16097,1.99475);
#1002=CYLINDRICAL_SURFACE('',#16098,1.99475);
#1003=CYLINDRICAL_SURFACE('',#16099,1.99475);
#1004=CYLINDRICAL_SURFACE('',#16100,1.99475);
#1005=CYLINDRICAL_SURFACE('',#16101,1.99475);
#1006=CYLINDRICAL_SURFACE('',#16102,1.99475);
#1007=CYLINDRICAL_SURFACE('',#16103,1.99475);
#1008=CYLINDRICAL_SURFACE('',#16104,1.99475);
#1009=CYLINDRICAL_SURFACE('',#16105,1.99475);
#1010=CYLINDRICAL_SURFACE('',#16106,1.99475);
#1011=CYLINDRICAL_SURFACE('',#16107,1.99475);
#1012=CYLINDRICAL_SURFACE('',#16108,1.99475);
#1013=CYLINDRICAL_SURFACE('',#16109,1.99475);
#1014=CYLINDRICAL_SURFACE('',#16110,1.99475);
#1015=CYLINDRICAL_SURFACE('',#16111,2.4505);
#1016=CYLINDRICAL_SURFACE('',#16114,1.99475);
#1017=CYLINDRICAL_SURFACE('',#16134,4.25);
#1018=CYLINDRICAL_SURFACE('',#16326,2.2594010767585);
#1019=CYLINDRICAL_SURFACE('',#16328,2.2594010767585);
#1020=CYLINDRICAL_SURFACE('',#16330,2.2594010767585);
#1021=CYLINDRICAL_SURFACE('',#16332,2.2594010767585);
#1022=CYLINDRICAL_SURFACE('',#16334,2.2594010767585);
#1023=CYLINDRICAL_SURFACE('',#16336,2.2594010767585);
#1206=FACE_BOUND('',#2952,.T.);
#1207=FACE_BOUND('',#3067,.T.);
#1430=PLANE('',#16116);
#1431=PLANE('',#16119);
#1432=PLANE('',#16125);
#1433=PLANE('',#16129);
#1434=PLANE('',#16130);
#1435=PLANE('',#16132);
#1436=PLANE('',#16133);
#1437=PLANE('',#16208);
#1438=PLANE('',#16209);
#1439=PLANE('',#16210);
#1440=PLANE('',#16213);
#1441=PLANE('',#16214);
#1442=PLANE('',#16215);
#1443=PLANE('',#16216);
#1444=PLANE('',#16217);
#1445=PLANE('',#16218);
#1446=PLANE('',#16219);
#1447=PLANE('',#16220);
#1448=PLANE('',#16221);
#1449=PLANE('',#16222);
#1450=PLANE('',#16223);
#1451=PLANE('',#16224);
#1452=PLANE('',#16225);
#1453=PLANE('',#16226);
#1454=PLANE('',#16227);
#1455=PLANE('',#16228);
#1456=PLANE('',#16229);
#1457=PLANE('',#16230);
#1458=PLANE('',#16231);
#1459=PLANE('',#16232);
#1460=PLANE('',#16233);
#1461=PLANE('',#16234);
#1462=PLANE('',#16235);
#1463=PLANE('',#16236);
#1464=PLANE('',#16237);
#1465=PLANE('',#16238);
#1466=PLANE('',#16239);
#1467=PLANE('',#16240);
#1468=PLANE('',#16241);
#1469=PLANE('',#16242);
#1470=PLANE('',#16243);
#1471=PLANE('',#16244);
#1472=PLANE('',#16245);
#1473=PLANE('',#16246);
#1474=PLANE('',#16247);
#1475=PLANE('',#16248);
#1476=PLANE('',#16249);
#1477=PLANE('',#16250);
#1478=PLANE('',#16251);
#1479=PLANE('',#16252);
#1480=PLANE('',#16253);
#1481=PLANE('',#16254);
#1482=PLANE('',#16255);
#1483=PLANE('',#16256);
#1484=PLANE('',#16257);
#1485=PLANE('',#16258);
#1486=PLANE('',#16259);
#1487=PLANE('',#16260);
#1488=PLANE('',#16261);
#1489=PLANE('',#16262);
#1490=PLANE('',#16263);
#1491=PLANE('',#16264);
#1492=PLANE('',#16265);
#1493=PLANE('',#16266);
#1494=PLANE('',#16267);
#1495=PLANE('',#16268);
#1496=PLANE('',#16269);
#1497=PLANE('',#16270);
#1498=PLANE('',#16271);
#1499=PLANE('',#16272);
#1500=PLANE('',#16273);
#1501=PLANE('',#16274);
#1502=PLANE('',#16275);
#1503=PLANE('',#16276);
#1504=PLANE('',#16277);
#1505=PLANE('',#16278);
#1506=PLANE('',#16279);
#1507=PLANE('',#16280);
#1508=PLANE('',#16281);
#1509=PLANE('',#16282);
#1510=PLANE('',#16283);
#1511=PLANE('',#16284);
#1512=PLANE('',#16285);
#1513=PLANE('',#16286);
#1514=PLANE('',#16287);
#1515=PLANE('',#16288);
#1516=PLANE('',#16289);
#1517=PLANE('',#16290);
#1518=PLANE('',#16291);
#1519=PLANE('',#16292);
#1520=PLANE('',#16293);
#1521=PLANE('',#16294);
#1522=PLANE('',#16295);
#1523=PLANE('',#16296);
#1524=PLANE('',#16297);
#1525=PLANE('',#16298);
#1526=PLANE('',#16299);
#1527=PLANE('',#16300);
#1528=PLANE('',#16301);
#1529=PLANE('',#16302);
#1530=PLANE('',#16303);
#1531=PLANE('',#16304);
#1532=PLANE('',#16305);
#1533=PLANE('',#16306);
#1534=PLANE('',#16307);
#1535=PLANE('',#16308);
#1536=PLANE('',#16309);
#1537=PLANE('',#16310);
#1538=PLANE('',#16311);
#1539=PLANE('',#16312);
#1540=PLANE('',#16313);
#1541=PLANE('',#16314);
#1542=PLANE('',#16317);
#1543=PLANE('',#16338);
#1544=PLANE('',#16339);
#1545=PLANE('',#16340);
#1546=PLANE('',#16341);
#1547=PLANE('',#16342);
#1548=PLANE('',#16343);
#1549=PLANE('',#16344);
#1550=PLANE('',#16345);
#1551=PLANE('',#16346);
#1552=PLANE('',#16347);
#1553=PLANE('',#16349);
#1554=PLANE('',#16351);
#1555=PLANE('',#16353);
#1556=PLANE('',#16355);
#1557=PLANE('',#16357);
#1558=PLANE('',#16360);
#1559=PLANE('',#16361);
#1560=PLANE('',#16362);
#2054=FACE_OUTER_BOUND('',#2920,.T.);
#2055=FACE_OUTER_BOUND('',#2921,.T.);
#2056=FACE_OUTER_BOUND('',#2922,.T.);
#2057=FACE_OUTER_BOUND('',#2923,.T.);
#2058=FACE_OUTER_BOUND('',#2924,.T.);
#2059=FACE_OUTER_BOUND('',#2925,.T.);
#2060=FACE_OUTER_BOUND('',#2926,.T.);
#2061=FACE_OUTER_BOUND('',#2927,.T.);
#2062=FACE_OUTER_BOUND('',#2928,.T.);
#2063=FACE_OUTER_BOUND('',#2929,.T.);
#2064=FACE_OUTER_BOUND('',#2930,.T.);
#2065=FACE_OUTER_BOUND('',#2931,.T.);
#2066=FACE_OUTER_BOUND('',#2932,.T.);
#2067=FACE_OUTER_BOUND('',#2933,.T.);
#2068=FACE_OUTER_BOUND('',#2934,.T.);
#2069=FACE_OUTER_BOUND('',#2935,.T.);
#2070=FACE_OUTER_BOUND('',#2936,.T.);
#2071=FACE_OUTER_BOUND('',#2937,.T.);
#2072=FACE_OUTER_BOUND('',#2938,.T.);
#2073=FACE_OUTER_BOUND('',#2939,.T.);
#2074=FACE_OUTER_BOUND('',#2940,.T.);
#2075=FACE_OUTER_BOUND('',#2941,.T.);
#2076=FACE_OUTER_BOUND('',#2942,.T.);
#2077=FACE_OUTER_BOUND('',#2943,.T.);
#2078=FACE_OUTER_BOUND('',#2944,.T.);
#2079=FACE_OUTER_BOUND('',#2945,.T.);
#2080=FACE_OUTER_BOUND('',#2946,.T.);
#2081=FACE_OUTER_BOUND('',#2947,.T.);
#2082=FACE_OUTER_BOUND('',#2948,.T.);
#2083=FACE_OUTER_BOUND('',#2949,.T.);
#2084=FACE_OUTER_BOUND('',#2950,.T.);
#2085=FACE_OUTER_BOUND('',#2951,.T.);
#2086=FACE_OUTER_BOUND('',#2953,.T.);
#2087=FACE_OUTER_BOUND('',#2954,.T.);
#2088=FACE_OUTER_BOUND('',#2955,.T.);
#2089=FACE_OUTER_BOUND('',#2956,.T.);
#2090=FACE_OUTER_BOUND('',#2957,.T.);
#2091=FACE_OUTER_BOUND('',#2958,.T.);
#2092=FACE_OUTER_BOUND('',#2959,.T.);
#2093=FACE_OUTER_BOUND('',#2960,.T.);
#2094=FACE_OUTER_BOUND('',#2961,.T.);
#2095=FACE_OUTER_BOUND('',#2962,.T.);
#2096=FACE_OUTER_BOUND('',#2963,.T.);
#2097=FACE_OUTER_BOUND('',#2964,.T.);
#2098=FACE_OUTER_BOUND('',#2965,.T.);
#2099=FACE_OUTER_BOUND('',#2966,.T.);
#2100=FACE_OUTER_BOUND('',#2967,.T.);
#2101=FACE_OUTER_BOUND('',#2968,.T.);
#2102=FACE_OUTER_BOUND('',#2969,.T.);
#2103=FACE_OUTER_BOUND('',#2970,.T.);
#2104=FACE_OUTER_BOUND('',#2971,.T.);
#2105=FACE_OUTER_BOUND('',#2972,.T.);
#2106=FACE_OUTER_BOUND('',#2973,.T.);
#2107=FACE_OUTER_BOUND('',#2974,.T.);
#2108=FACE_OUTER_BOUND('',#2975,.T.);
#2109=FACE_OUTER_BOUND('',#2976,.T.);
#2110=FACE_OUTER_BOUND('',#2977,.T.);
#2111=FACE_OUTER_BOUND('',#2978,.T.);
#2112=FACE_OUTER_BOUND('',#2979,.T.);
#2113=FACE_OUTER_BOUND('',#2980,.T.);
#2114=FACE_OUTER_BOUND('',#2981,.T.);
#2115=FACE_OUTER_BOUND('',#2982,.T.);
#2116=FACE_OUTER_BOUND('',#2983,.T.);
#2117=FACE_OUTER_BOUND('',#2984,.T.);
#2118=FACE_OUTER_BOUND('',#2985,.T.);
#2119=FACE_OUTER_BOUND('',#2986,.T.);
#2120=FACE_OUTER_BOUND('',#2987,.T.);
#2121=FACE_OUTER_BOUND('',#2988,.T.);
#2122=FACE_OUTER_BOUND('',#2989,.T.);
#2123=FACE_OUTER_BOUND('',#2990,.T.);
#2124=FACE_OUTER_BOUND('',#2991,.T.);
#2125=FACE_OUTER_BOUND('',#2992,.T.);
#2126=FACE_OUTER_BOUND('',#2993,.T.);
#2127=FACE_OUTER_BOUND('',#2994,.T.);
#2128=FACE_OUTER_BOUND('',#2995,.T.);
#2129=FACE_OUTER_BOUND('',#2996,.T.);
#2130=FACE_OUTER_BOUND('',#2997,.T.);
#2131=FACE_OUTER_BOUND('',#2998,.T.);
#2132=FACE_OUTER_BOUND('',#2999,.T.);
#2133=FACE_OUTER_BOUND('',#3000,.T.);
#2134=FACE_OUTER_BOUND('',#3001,.T.);
#2135=FACE_OUTER_BOUND('',#3002,.T.);
#2136=FACE_OUTER_BOUND('',#3003,.T.);
#2137=FACE_OUTER_BOUND('',#3004,.T.);
#2138=FACE_OUTER_BOUND('',#3005,.T.);
#2139=FACE_OUTER_BOUND('',#3006,.T.);
#2140=FACE_OUTER_BOUND('',#3007,.T.);
#2141=FACE_OUTER_BOUND('',#3008,.T.);
#2142=FACE_OUTER_BOUND('',#3009,.T.);
#2143=FACE_OUTER_BOUND('',#3010,.T.);
#2144=FACE_OUTER_BOUND('',#3011,.T.);
#2145=FACE_OUTER_BOUND('',#3012,.T.);
#2146=FACE_OUTER_BOUND('',#3013,.T.);
#2147=FACE_OUTER_BOUND('',#3014,.T.);
#2148=FACE_OUTER_BOUND('',#3015,.T.);
#2149=FACE_OUTER_BOUND('',#3016,.T.);
#2150=FACE_OUTER_BOUND('',#3017,.T.);
#2151=FACE_OUTER_BOUND('',#3018,.T.);
#2152=FACE_OUTER_BOUND('',#3019,.T.);
#2153=FACE_OUTER_BOUND('',#3020,.T.);
#2154=FACE_OUTER_BOUND('',#3021,.T.);
#2155=FACE_OUTER_BOUND('',#3022,.T.);
#2156=FACE_OUTER_BOUND('',#3023,.T.);
#2157=FACE_OUTER_BOUND('',#3024,.T.);
#2158=FACE_OUTER_BOUND('',#3025,.T.);
#2159=FACE_OUTER_BOUND('',#3026,.T.);
#2160=FACE_OUTER_BOUND('',#3027,.T.);
#2161=FACE_OUTER_BOUND('',#3028,.T.);
#2162=FACE_OUTER_BOUND('',#3029,.T.);
#2163=FACE_OUTER_BOUND('',#3030,.T.);
#2164=FACE_OUTER_BOUND('',#3031,.T.);
#2165=FACE_OUTER_BOUND('',#3032,.T.);
#2166=FACE_OUTER_BOUND('',#3033,.T.);
#2167=FACE_OUTER_BOUND('',#3034,.T.);
#2168=FACE_OUTER_BOUND('',#3035,.T.);
#2169=FACE_OUTER_BOUND('',#3036,.T.);
#2170=FACE_OUTER_BOUND('',#3037,.T.);
#2171=FACE_OUTER_BOUND('',#3038,.T.);
#2172=FACE_OUTER_BOUND('',#3039,.T.);
#2173=FACE_OUTER_BOUND('',#3040,.T.);
#2174=FACE_OUTER_BOUND('',#3041,.T.);
#2175=FACE_OUTER_BOUND('',#3042,.T.);
#2176=FACE_OUTER_BOUND('',#3043,.T.);
#2177=FACE_OUTER_BOUND('',#3044,.T.);
#2178=FACE_OUTER_BOUND('',#3045,.T.);
#2179=FACE_OUTER_BOUND('',#3046,.T.);
#2180=FACE_OUTER_BOUND('',#3047,.T.);
#2181=FACE_OUTER_BOUND('',#3048,.T.);
#2182=FACE_OUTER_BOUND('',#3049,.T.);
#2183=FACE_OUTER_BOUND('',#3050,.T.);
#2184=FACE_OUTER_BOUND('',#3051,.T.);
#2185=FACE_OUTER_BOUND('',#3052,.T.);
#2186=FACE_OUTER_BOUND('',#3053,.T.);
#2187=FACE_OUTER_BOUND('',#3054,.T.);
#2188=FACE_OUTER_BOUND('',#3055,.T.);
#2189=FACE_OUTER_BOUND('',#3056,.T.);
#2190=FACE_OUTER_BOUND('',#3057,.T.);
#2191=FACE_OUTER_BOUND('',#3058,.T.);
#2192=FACE_OUTER_BOUND('',#3059,.T.);
#2193=FACE_OUTER_BOUND('',#3060,.T.);
#2194=FACE_OUTER_BOUND('',#3061,.T.);
#2195=FACE_OUTER_BOUND('',#3062,.T.);
#2196=FACE_OUTER_BOUND('',#3063,.T.);
#2197=FACE_OUTER_BOUND('',#3064,.T.);
#2198=FACE_OUTER_BOUND('',#3065,.T.);
#2199=FACE_OUTER_BOUND('',#3066,.T.);
#2200=FACE_OUTER_BOUND('',#3068,.T.);
#2201=FACE_OUTER_BOUND('',#3069,.T.);
#2202=FACE_OUTER_BOUND('',#3070,.T.);
#2203=FACE_OUTER_BOUND('',#3071,.T.);
#2204=FACE_OUTER_BOUND('',#3072,.T.);
#2205=FACE_OUTER_BOUND('',#3073,.T.);
#2206=FACE_OUTER_BOUND('',#3074,.T.);
#2207=FACE_OUTER_BOUND('',#3075,.T.);
#2208=FACE_OUTER_BOUND('',#3076,.T.);
#2209=FACE_OUTER_BOUND('',#3077,.T.);
#2210=FACE_OUTER_BOUND('',#3078,.T.);
#2211=FACE_OUTER_BOUND('',#3079,.T.);
#2212=FACE_OUTER_BOUND('',#3080,.T.);
#2213=FACE_OUTER_BOUND('',#3081,.T.);
#2214=FACE_OUTER_BOUND('',#3082,.T.);
#2215=FACE_OUTER_BOUND('',#3083,.T.);
#2216=FACE_OUTER_BOUND('',#3084,.T.);
#2217=FACE_OUTER_BOUND('',#3085,.T.);
#2218=FACE_OUTER_BOUND('',#3086,.T.);
#2219=FACE_OUTER_BOUND('',#3087,.T.);
#2220=FACE_OUTER_BOUND('',#3088,.T.);
#2221=FACE_OUTER_BOUND('',#3089,.T.);
#2222=FACE_OUTER_BOUND('',#3090,.T.);
#2223=FACE_OUTER_BOUND('',#3091,.T.);
#2224=FACE_OUTER_BOUND('',#3092,.T.);
#2225=FACE_OUTER_BOUND('',#3093,.T.);
#2920=EDGE_LOOP('',(#12182,#12183,#12184,#12185));
#2921=EDGE_LOOP('',(#12186,#12187,#12188,#12189,#12190));
#2922=EDGE_LOOP('',(#12191,#12192,#12193,#12194,#12195));
#2923=EDGE_LOOP('',(#12196,#12197,#12198,#12199,#12200));
#2924=EDGE_LOOP('',(#12201,#12202,#12203,#12204,#12205));
#2925=EDGE_LOOP('',(#12206,#12207,#12208,#12209,#12210));
#2926=EDGE_LOOP('',(#12211,#12212,#12213,#12214,#12215));
#2927=EDGE_LOOP('',(#12216,#12217,#12218,#12219,#12220,#12221));
#2928=EDGE_LOOP('',(#12222,#12223,#12224,#12225));
#2929=EDGE_LOOP('',(#12226,#12227,#12228,#12229,#12230,#12231));
#2930=EDGE_LOOP('',(#12232,#12233,#12234,#12235,#12236,#12237));
#2931=EDGE_LOOP('',(#12238,#12239,#12240,#12241,#12242));
#2932=EDGE_LOOP('',(#12243,#12244,#12245,#12246,#12247));
#2933=EDGE_LOOP('',(#12248,#12249,#12250,#12251,#12252));
#2934=EDGE_LOOP('',(#12253,#12254,#12255,#12256,#12257));
#2935=EDGE_LOOP('',(#12258,#12259,#12260,#12261,#12262));
#2936=EDGE_LOOP('',(#12263,#12264,#12265,#12266,#12267));
#2937=EDGE_LOOP('',(#12268,#12269,#12270,#12271,#12272));
#2938=EDGE_LOOP('',(#12273,#12274,#12275,#12276,#12277));
#2939=EDGE_LOOP('',(#12278,#12279,#12280,#12281,#12282));
#2940=EDGE_LOOP('',(#12283,#12284,#12285,#12286,#12287));
#2941=EDGE_LOOP('',(#12288,#12289,#12290,#12291,#12292));
#2942=EDGE_LOOP('',(#12293,#12294,#12295,#12296,#12297));
#2943=EDGE_LOOP('',(#12298,#12299,#12300,#12301,#12302,#12303));
#2944=EDGE_LOOP('',(#12304,#12305,#12306,#12307,#12308,#12309,#12310,#12311,
#12312,#12313,#12314,#12315,#12316,#12317,#12318,#12319,#12320,#12321,#12322,
#12323,#12324,#12325,#12326,#12327,#12328,#12329,#12330,#12331,#12332,#12333,
#12334,#12335,#12336,#12337,#12338,#12339,#12340,#12341,#12342,#12343,#12344,
#12345,#12346,#12347,#12348,#12349,#12350,#12351,#12352,#12353,#12354,#12355));
#2945=EDGE_LOOP('',(#12356,#12357,#12358,#12359,#12360,#12361));
#2946=EDGE_LOOP('',(#12362,#12363,#12364,#12365,#12366));
#2947=EDGE_LOOP('',(#12367,#12368,#12369,#12370,#12371,#12372,#12373,#12374,
#12375,#12376,#12377,#12378,#12379,#12380,#12381,#12382,#12383,#12384,#12385,
#12386,#12387,#12388,#12389,#12390,#12391,#12392,#12393,#12394,#12395,#12396,
#12397,#12398,#12399,#12400,#12401,#12402,#12403,#12404,#12405,#12406,#12407,
#12408,#12409,#12410,#12411,#12412,#12413,#12414,#12415,#12416,#12417,#12418,
#12419,#12420,#12421,#12422,#12423,#12424,#12425,#12426,#12427,#12428,#12429,
#12430,#12431,#12432,#12433,#12434));
#2948=EDGE_LOOP('',(#12435,#12436,#12437,#12438,#12439,#12440));
#2949=EDGE_LOOP('',(#12441,#12442,#12443,#12444,#12445,#12446,#12447,#12448,
#12449,#12450,#12451,#12452,#12453,#12454,#12455,#12456,#12457,#12458,#12459,
#12460,#12461,#12462,#12463,#12464,#12465,#12466,#12467,#12468,#12469,#12470,
#12471,#12472,#12473,#12474,#12475,#12476,#12477,#12478,#12479,#12480,#12481,
#12482,#12483,#12484,#12485,#12486,#12487,#12488,#12489,#12490,#12491,#12492,
#12493,#12494,#12495,#12496,#12497,#12498,#12499,#12500,#12501,#12502,#12503,
#12504,#12505,#12506,#12507));
#2950=EDGE_LOOP('',(#12508,#12509,#12510,#12511,#12512,#12513,#12514));
#2951=EDGE_LOOP('',(#12515));
#2952=EDGE_LOOP('',(#12516));
#2953=EDGE_LOOP('',(#12517,#12518,#12519,#12520,#12521,#12522,#12523));
#2954=EDGE_LOOP('',(#12524));
#2955=EDGE_LOOP('',(#12525,#12526,#12527));
#2956=EDGE_LOOP('',(#12528,#12529,#12530,#12531));
#2957=EDGE_LOOP('',(#12532,#12533,#12534,#12535));
#2958=EDGE_LOOP('',(#12536,#12537,#12538,#12539,#12540,#12541,#12542,#12543,
#12544,#12545,#12546,#12547,#12548,#12549,#12550,#12551,#12552,#12553,#12554,
#12555,#12556,#12557,#12558,#12559,#12560,#12561,#12562,#12563,#12564,#12565,
#12566,#12567,#12568,#12569,#12570,#12571,#12572,#12573,#12574,#12575,#12576,
#12577,#12578,#12579,#12580,#12581,#12582,#12583,#12584,#12585,#12586,#12587,
#12588,#12589,#12590,#12591,#12592,#12593,#12594,#12595,#12596,#12597,#12598,
#12599,#12600,#12601,#12602,#12603,#12604,#12605,#12606,#12607,#12608,#12609,
#12610,#12611,#12612,#12613,#12614,#12615,#12616,#12617,#12618,#12619,#12620,
#12621,#12622,#12623,#12624,#12625,#12626,#12627,#12628,#12629,#12630,#12631,
#12632,#12633,#12634,#12635,#12636,#12637,#12638,#12639,#12640,#12641,#12642,
#12643,#12644,#12645,#12646,#12647,#12648,#12649,#12650,#12651,#12652,#12653,
#12654,#12655,#12656,#12657,#12658,#12659,#12660,#12661,#12662,#12663,#12664,
#12665,#12666,#12667,#12668,#12669,#12670,#12671,#12672,#12673,#12674,#12675,
#12676,#12677,#12678,#12679,#12680,#12681,#12682,#12683));
#2959=EDGE_LOOP('',(#12684,#12685,#12686,#12687));
#2960=EDGE_LOOP('',(#12688,#12689,#12690,#12691));
#2961=EDGE_LOOP('',(#12692,#12693,#12694));
#2962=EDGE_LOOP('',(#12695,#12696,#12697,#12698,#12699,#12700,#12701,#12702,
#12703,#12704,#12705,#12706,#12707,#12708,#12709,#12710,#12711,#12712,#12713,
#12714,#12715,#12716,#12717,#12718,#12719,#12720,#12721,#12722,#12723,#12724,
#12725,#12726,#12727,#12728,#12729,#12730,#12731,#12732,#12733,#12734,#12735,
#12736,#12737,#12738,#12739,#12740,#12741,#12742,#12743,#12744,#12745,#12746,
#12747,#12748,#12749,#12750,#12751,#12752,#12753,#12754,#12755,#12756,#12757,
#12758,#12759,#12760,#12761,#12762,#12763,#12764,#12765,#12766,#12767,#12768,
#12769,#12770,#12771,#12772,#12773,#12774,#12775,#12776,#12777,#12778,#12779,
#12780,#12781,#12782,#12783,#12784,#12785,#12786,#12787,#12788,#12789,#12790,
#12791,#12792,#12793,#12794,#12795,#12796,#12797,#12798,#12799,#12800,#12801,
#12802,#12803,#12804,#12805));
#2963=EDGE_LOOP('',(#12806,#12807,#12808));
#2964=EDGE_LOOP('',(#12809,#12810,#12811,#12812));
#2965=EDGE_LOOP('',(#12813,#12814,#12815,#12816));
#2966=EDGE_LOOP('',(#12817,#12818,#12819,#12820));
#2967=EDGE_LOOP('',(#12821,#12822,#12823,#12824));
#2968=EDGE_LOOP('',(#12825,#12826,#12827));
#2969=EDGE_LOOP('',(#12828,#12829,#12830));
#2970=EDGE_LOOP('',(#12831,#12832,#12833,#12834));
#2971=EDGE_LOOP('',(#12835,#12836,#12837,#12838));
#2972=EDGE_LOOP('',(#12839,#12840,#12841,#12842));
#2973=EDGE_LOOP('',(#12843,#12844,#12845,#12846));
#2974=EDGE_LOOP('',(#12847,#12848,#12849));
#2975=EDGE_LOOP('',(#12850,#12851,#12852));
#2976=EDGE_LOOP('',(#12853,#12854,#12855,#12856));
#2977=EDGE_LOOP('',(#12857,#12858,#12859,#12860));
#2978=EDGE_LOOP('',(#12861,#12862,#12863,#12864));
#2979=EDGE_LOOP('',(#12865,#12866,#12867,#12868));
#2980=EDGE_LOOP('',(#12869,#12870,#12871));
#2981=EDGE_LOOP('',(#12872,#12873,#12874));
#2982=EDGE_LOOP('',(#12875,#12876,#12877,#12878));
#2983=EDGE_LOOP('',(#12879,#12880,#12881,#12882));
#2984=EDGE_LOOP('',(#12883,#12884,#12885,#12886));
#2985=EDGE_LOOP('',(#12887,#12888,#12889,#12890));
#2986=EDGE_LOOP('',(#12891,#12892,#12893));
#2987=EDGE_LOOP('',(#12894,#12895,#12896));
#2988=EDGE_LOOP('',(#12897,#12898,#12899,#12900));
#2989=EDGE_LOOP('',(#12901,#12902,#12903,#12904));
#2990=EDGE_LOOP('',(#12905,#12906,#12907,#12908));
#2991=EDGE_LOOP('',(#12909,#12910,#12911,#12912));
#2992=EDGE_LOOP('',(#12913,#12914,#12915));
#2993=EDGE_LOOP('',(#12916,#12917,#12918));
#2994=EDGE_LOOP('',(#12919,#12920,#12921,#12922));
#2995=EDGE_LOOP('',(#12923,#12924,#12925,#12926));
#2996=EDGE_LOOP('',(#12927,#12928,#12929,#12930));
#2997=EDGE_LOOP('',(#12931,#12932,#12933,#12934));
#2998=EDGE_LOOP('',(#12935,#12936,#12937));
#2999=EDGE_LOOP('',(#12938,#12939,#12940));
#3000=EDGE_LOOP('',(#12941,#12942,#12943,#12944));
#3001=EDGE_LOOP('',(#12945,#12946,#12947,#12948));
#3002=EDGE_LOOP('',(#12949,#12950,#12951,#12952));
#3003=EDGE_LOOP('',(#12953,#12954,#12955,#12956));
#3004=EDGE_LOOP('',(#12957,#12958,#12959));
#3005=EDGE_LOOP('',(#12960,#12961,#12962));
#3006=EDGE_LOOP('',(#12963,#12964,#12965,#12966));
#3007=EDGE_LOOP('',(#12967,#12968,#12969,#12970));
#3008=EDGE_LOOP('',(#12971,#12972,#12973,#12974));
#3009=EDGE_LOOP('',(#12975,#12976,#12977,#12978));
#3010=EDGE_LOOP('',(#12979,#12980,#12981,#12982));
#3011=EDGE_LOOP('',(#12983,#12984,#12985));
#3012=EDGE_LOOP('',(#12986,#12987,#12988,#12989));
#3013=EDGE_LOOP('',(#12990,#12991,#12992,#12993));
#3014=EDGE_LOOP('',(#12994,#12995,#12996,#12997));
#3015=EDGE_LOOP('',(#12998,#12999,#13000,#13001));
#3016=EDGE_LOOP('',(#13002,#13003,#13004));
#3017=EDGE_LOOP('',(#13005,#13006,#13007));
#3018=EDGE_LOOP('',(#13008,#13009,#13010,#13011));
#3019=EDGE_LOOP('',(#13012,#13013,#13014,#13015));
#3020=EDGE_LOOP('',(#13016,#13017,#13018,#13019));
#3021=EDGE_LOOP('',(#13020,#13021,#13022,#13023));
#3022=EDGE_LOOP('',(#13024,#13025,#13026));
#3023=EDGE_LOOP('',(#13027,#13028,#13029));
#3024=EDGE_LOOP('',(#13030,#13031,#13032,#13033));
#3025=EDGE_LOOP('',(#13034,#13035,#13036,#13037));
#3026=EDGE_LOOP('',(#13038,#13039,#13040,#13041));
#3027=EDGE_LOOP('',(#13042,#13043,#13044,#13045));
#3028=EDGE_LOOP('',(#13046,#13047,#13048));
#3029=EDGE_LOOP('',(#13049,#13050,#13051));
#3030=EDGE_LOOP('',(#13052,#13053,#13054,#13055));
#3031=EDGE_LOOP('',(#13056,#13057,#13058,#13059));
#3032=EDGE_LOOP('',(#13060,#13061,#13062,#13063));
#3033=EDGE_LOOP('',(#13064,#13065,#13066,#13067));
#3034=EDGE_LOOP('',(#13068,#13069,#13070));
#3035=EDGE_LOOP('',(#13071,#13072,#13073));
#3036=EDGE_LOOP('',(#13074,#13075,#13076,#13077));
#3037=EDGE_LOOP('',(#13078,#13079,#13080,#13081));
#3038=EDGE_LOOP('',(#13082,#13083,#13084,#13085));
#3039=EDGE_LOOP('',(#13086,#13087,#13088,#13089));
#3040=EDGE_LOOP('',(#13090,#13091,#13092));
#3041=EDGE_LOOP('',(#13093,#13094,#13095));
#3042=EDGE_LOOP('',(#13096,#13097,#13098,#13099));
#3043=EDGE_LOOP('',(#13100,#13101,#13102,#13103));
#3044=EDGE_LOOP('',(#13104,#13105,#13106,#13107));
#3045=EDGE_LOOP('',(#13108,#13109,#13110,#13111));
#3046=EDGE_LOOP('',(#13112,#13113,#13114));
#3047=EDGE_LOOP('',(#13115,#13116,#13117));
#3048=EDGE_LOOP('',(#13118,#13119,#13120,#13121));
#3049=EDGE_LOOP('',(#13122,#13123,#13124,#13125));
#3050=EDGE_LOOP('',(#13126,#13127,#13128,#13129));
#3051=EDGE_LOOP('',(#13130,#13131,#13132,#13133));
#3052=EDGE_LOOP('',(#13134,#13135,#13136));
#3053=EDGE_LOOP('',(#13137,#13138,#13139));
#3054=EDGE_LOOP('',(#13140,#13141,#13142,#13143));
#3055=EDGE_LOOP('',(#13144,#13145,#13146,#13147));
#3056=EDGE_LOOP('',(#13148,#13149,#13150,#13151));
#3057=EDGE_LOOP('',(#13152,#13153,#13154,#13155));
#3058=EDGE_LOOP('',(#13156,#13157,#13158));
#3059=EDGE_LOOP('',(#13159,#13160,#13161));
#3060=EDGE_LOOP('',(#13162,#13163,#13164,#13165));
#3061=EDGE_LOOP('',(#13166,#13167,#13168,#13169));
#3062=EDGE_LOOP('',(#13170,#13171,#13172,#13173));
#3063=EDGE_LOOP('',(#13174,#13175,#13176,#13177));
#3064=EDGE_LOOP('',(#13178,#13179,#13180));
#3065=EDGE_LOOP('',(#13181,#13182,#13183,#13184));
#3066=EDGE_LOOP('',(#13185));
#3067=EDGE_LOOP('',(#13186));
#3068=EDGE_LOOP('',(#13187,#13188,#13189,#13190,#13191,#13192,#13193,#13194,
#13195,#13196,#13197,#13198,#13199,#13200,#13201,#13202,#13203,#13204,#13205,
#13206,#13207));
#3069=EDGE_LOOP('',(#13208,#13209,#13210,#13211));
#3070=EDGE_LOOP('',(#13212,#13213,#13214,#13215));
#3071=EDGE_LOOP('',(#13216,#13217,#13218,#13219));
#3072=EDGE_LOOP('',(#13220,#13221,#13222,#13223));
#3073=EDGE_LOOP('',(#13224,#13225,#13226,#13227));
#3074=EDGE_LOOP('',(#13228,#13229,#13230,#13231));
#3075=EDGE_LOOP('',(#13232,#13233,#13234,#13235,#13236,#13237,#13238,#13239));
#3076=EDGE_LOOP('',(#13240,#13241,#13242,#13243,#13244,#13245,#13246,#13247));
#3077=EDGE_LOOP('',(#13248,#13249,#13250,#13251,#13252,#13253,#13254,#13255));
#3078=EDGE_LOOP('',(#13256,#13257));
#3079=EDGE_LOOP('',(#13258,#13259));
#3080=EDGE_LOOP('',(#13260,#13261));
#3081=EDGE_LOOP('',(#13262,#13263));
#3082=EDGE_LOOP('',(#13264,#13265));
#3083=EDGE_LOOP('',(#13266,#13267));
#3084=EDGE_LOOP('',(#13268,#13269));
#3085=EDGE_LOOP('',(#13270,#13271));
#3086=EDGE_LOOP('',(#13272,#13273));
#3087=EDGE_LOOP('',(#13274,#13275));
#3088=EDGE_LOOP('',(#13276,#13277));
#3089=EDGE_LOOP('',(#13278,#13279));
#3090=EDGE_LOOP('',(#13280,#13281,#13282,#13283,#13284,#13285,#13286,#13287));
#3091=EDGE_LOOP('',(#13288,#13289,#13290,#13291,#13292,#13293,#13294,#13295));
#3092=EDGE_LOOP('',(#13296,#13297,#13298,#13299,#13300,#13301,#13302,#13303));
#3093=EDGE_LOOP('',(#13304,#13305,#13306,#13307,#13308,#13309,#13310,#13311));
#3989=LINE('',#23038,#5101);
#3990=LINE('',#23279,#5102);
#3991=LINE('',#23718,#5103);
#3992=LINE('',#24155,#5104);
#3993=LINE('',#24596,#5105);
#3994=LINE('',#25079,#5106);
#3995=LINE('',#25510,#5107);
#3996=LINE('',#25798,#5108);
#3997=LINE('',#26266,#5109);
#3998=LINE('',#26700,#5110);
#3999=LINE('',#26872,#5111);
#4000=LINE('',#27194,#5112);
#4001=LINE('',#27647,#5113);
#4002=LINE('',#28096,#5114);
#4003=LINE('',#28531,#5115);
#4004=LINE('',#28990,#5116);
#4005=LINE('',#29435,#5117);
#4006=LINE('',#29914,#5118);
#4007=LINE('',#30399,#5119);
#4008=LINE('',#30846,#5120);
#4009=LINE('',#31293,#5121);
#4010=LINE('',#31726,#5122);
#4011=LINE('',#32243,#5123);
#4012=LINE('',#32694,#5124);
#4013=LINE('',#42247,#5125);
#4014=LINE('',#42255,#5126);
#4015=LINE('',#42256,#5127);
#4016=LINE('',#42259,#5128);
#4017=LINE('',#42261,#5129);
#4018=LINE('',#42267,#5130);
#4019=LINE('',#42276,#5131);
#4020=LINE('',#42281,#5132);
#4021=LINE('',#42285,#5133);
#4022=LINE('',#42289,#5134);
#4023=LINE('',#42293,#5135);
#4024=LINE('',#42297,#5136);
#4025=LINE('',#42301,#5137);
#4026=LINE('',#42305,#5138);
#4027=LINE('',#42309,#5139);
#4028=LINE('',#42313,#5140);
#4029=LINE('',#42317,#5141);
#4030=LINE('',#42321,#5142);
#4031=LINE('',#42325,#5143);
#4032=LINE('',#42329,#5144);
#4033=LINE('',#42333,#5145);
#4034=LINE('',#42337,#5146);
#4035=LINE('',#42341,#5147);
#4036=LINE('',#42345,#5148);
#4037=LINE('',#42349,#5149);
#4038=LINE('',#42353,#5150);
#4039=LINE('',#42357,#5151);
#4040=LINE('',#42361,#5152);
#4041=LINE('',#42365,#5153);
#4042=LINE('',#42369,#5154);
#4043=LINE('',#42373,#5155);
#4044=LINE('',#42377,#5156);
#4045=LINE('',#42381,#5157);
#4046=LINE('',#42385,#5158);
#4047=LINE('',#42389,#5159);
#4048=LINE('',#42393,#5160);
#4049=LINE('',#42397,#5161);
#4050=LINE('',#42401,#5162);
#4051=LINE('',#42405,#5163);
#4052=LINE('',#42409,#5164);
#4053=LINE('',#42414,#5165);
#4054=LINE('',#42418,#5166);
#4055=LINE('',#42422,#5167);
#4056=LINE('',#42426,#5168);
#4057=LINE('',#42430,#5169);
#4058=LINE('',#42434,#5170);
#4059=LINE('',#42438,#5171);
#4060=LINE('',#42442,#5172);
#4061=LINE('',#42446,#5173);
#4062=LINE('',#42450,#5174);
#4063=LINE('',#42454,#5175);
#4064=LINE('',#42458,#5176);
#4065=LINE('',#42462,#5177);
#4066=LINE('',#42466,#5178);
#4067=LINE('',#42470,#5179);
#4068=LINE('',#42474,#5180);
#4069=LINE('',#42478,#5181);
#4070=LINE('',#42482,#5182);
#4071=LINE('',#42486,#5183);
#4072=LINE('',#42490,#5184);
#4073=LINE('',#42494,#5185);
#4074=LINE('',#42498,#5186);
#4075=LINE('',#42502,#5187);
#4076=LINE('',#42506,#5188);
#4077=LINE('',#42510,#5189);
#4078=LINE('',#42514,#5190);
#4079=LINE('',#42518,#5191);
#4080=LINE('',#42522,#5192);
#4081=LINE('',#42526,#5193);
#4082=LINE('',#42530,#5194);
#4083=LINE('',#42534,#5195);
#4084=LINE('',#42538,#5196);
#4085=LINE('',#42542,#5197);
#4086=LINE('',#42546,#5198);
#4087=LINE('',#42550,#5199);
#4088=LINE('',#42554,#5200);
#4089=LINE('',#42557,#5201);
#4090=LINE('',#42560,#5202);
#4091=LINE('',#42562,#5203);
#4092=LINE('',#42570,#5204);
#4093=LINE('',#42812,#5205);
#4094=LINE('',#42816,#5206);
#4095=LINE('',#42817,#5207);
#4096=LINE('',#42819,#5208);
#4097=LINE('',#42823,#5209);
#4098=LINE('',#42824,#5210);
#4099=LINE('',#42826,#5211);
#4100=LINE('',#42830,#5212);
#4101=LINE('',#42831,#5213);
#4102=LINE('',#42833,#5214);
#4103=LINE('',#42837,#5215);
#4104=LINE('',#42838,#5216);
#4105=LINE('',#42840,#5217);
#4106=LINE('',#42844,#5218);
#4107=LINE('',#42845,#5219);
#4108=LINE('',#42847,#5220);
#4109=LINE('',#42851,#5221);
#4110=LINE('',#42852,#5222);
#4111=LINE('',#42854,#5223);
#4112=LINE('',#42858,#5224);
#4113=LINE('',#42859,#5225);
#4114=LINE('',#42861,#5226);
#4115=LINE('',#42865,#5227);
#4116=LINE('',#42866,#5228);
#4117=LINE('',#42868,#5229);
#4118=LINE('',#42872,#5230);
#4119=LINE('',#42873,#5231);
#4120=LINE('',#42875,#5232);
#4121=LINE('',#42879,#5233);
#4122=LINE('',#42880,#5234);
#4123=LINE('',#42882,#5235);
#4124=LINE('',#42886,#5236);
#4125=LINE('',#42887,#5237);
#4126=LINE('',#42889,#5238);
#4127=LINE('',#42893,#5239);
#4128=LINE('',#42894,#5240);
#4129=LINE('',#42896,#5241);
#4130=LINE('',#42900,#5242);
#4131=LINE('',#42901,#5243);
#4132=LINE('',#42903,#5244);
#4133=LINE('',#42907,#5245);
#4134=LINE('',#42908,#5246);
#4135=LINE('',#42910,#5247);
#4136=LINE('',#42914,#5248);
#4137=LINE('',#42915,#5249);
#4138=LINE('',#42917,#5250);
#4139=LINE('',#42921,#5251);
#4140=LINE('',#42922,#5252);
#4141=LINE('',#42924,#5253);
#4142=LINE('',#42928,#5254);
#4143=LINE('',#42929,#5255);
#4144=LINE('',#42931,#5256);
#4145=LINE('',#42935,#5257);
#4146=LINE('',#42936,#5258);
#4147=LINE('',#42938,#5259);
#4148=LINE('',#42942,#5260);
#4149=LINE('',#42943,#5261);
#4150=LINE('',#42945,#5262);
#4151=LINE('',#42949,#5263);
#4152=LINE('',#42950,#5264);
#4153=LINE('',#42952,#5265);
#4154=LINE('',#42956,#5266);
#4155=LINE('',#42957,#5267);
#4156=LINE('',#42959,#5268);
#4157=LINE('',#42963,#5269);
#4158=LINE('',#42964,#5270);
#4159=LINE('',#42966,#5271);
#4160=LINE('',#42970,#5272);
#4161=LINE('',#42971,#5273);
#4162=LINE('',#42973,#5274);
#4163=LINE('',#42977,#5275);
#4164=LINE('',#42978,#5276);
#4165=LINE('',#42980,#5277);
#4166=LINE('',#42984,#5278);
#4167=LINE('',#42985,#5279);
#4168=LINE('',#42987,#5280);
#4169=LINE('',#42991,#5281);
#4170=LINE('',#42992,#5282);
#4171=LINE('',#42994,#5283);
#4172=LINE('',#42998,#5284);
#4173=LINE('',#42999,#5285);
#4174=LINE('',#43001,#5286);
#4175=LINE('',#43005,#5287);
#4176=LINE('',#43006,#5288);
#4177=LINE('',#43008,#5289);
#4178=LINE('',#43012,#5290);
#4179=LINE('',#43013,#5291);
#4180=LINE('',#43015,#5292);
#4181=LINE('',#43019,#5293);
#4182=LINE('',#43020,#5294);
#4183=LINE('',#43022,#5295);
#4184=LINE('',#43026,#5296);
#4185=LINE('',#43027,#5297);
#4186=LINE('',#43029,#5298);
#4187=LINE('',#43033,#5299);
#4188=LINE('',#43034,#5300);
#4189=LINE('',#43036,#5301);
#4190=LINE('',#43040,#5302);
#4191=LINE('',#43041,#5303);
#4192=LINE('',#43043,#5304);
#4193=LINE('',#43047,#5305);
#4194=LINE('',#43048,#5306);
#4195=LINE('',#43050,#5307);
#4196=LINE('',#43118,#5308);
#4197=LINE('',#43121,#5309);
#4198=LINE('',#43123,#5310);
#4199=LINE('',#43127,#5311);
#4200=LINE('',#43129,#5312);
#4201=LINE('',#43133,#5313);
#4202=LINE('',#43136,#5314);
#4203=LINE('',#43139,#5315);
#4204=LINE('',#43141,#5316);
#4205=LINE('',#43145,#5317);
#4206=LINE('',#43148,#5318);
#4207=LINE('',#43151,#5319);
#4208=LINE('',#43154,#5320);
#4209=LINE('',#43156,#5321);
#4210=LINE('',#43158,#5322);
#4211=LINE('',#43160,#5323);
#4212=LINE('',#43161,#5324);
#4213=LINE('',#43163,#5325);
#4214=LINE('',#43165,#5326);
#4215=LINE('',#43166,#5327);
#4216=LINE('',#43168,#5328);
#4217=LINE('',#43170,#5329);
#4218=LINE('',#43171,#5330);
#4219=LINE('',#43175,#5331);
#4220=LINE('',#43178,#5332);
#4221=LINE('',#43180,#5333);
#4222=LINE('',#43183,#5334);
#4223=LINE('',#43193,#5335);
#4224=LINE('',#43196,#5336);
#4225=LINE('',#43200,#5337);
#4226=LINE('',#43202,#5338);
#4227=LINE('',#43204,#5339);
#5101=VECTOR('',#19153,1.99475);
#5102=VECTOR('',#19158,1.99475);
#5103=VECTOR('',#19161,1.99475);
#5104=VECTOR('',#19164,1.99475);
#5105=VECTOR('',#19167,1.99475);
#5106=VECTOR('',#19170,1.99475);
#5107=VECTOR('',#19173,1.99475);
#5108=VECTOR('',#19176,1.99475);
#5109=VECTOR('',#19179,1.99475);
#5110=VECTOR('',#19182,1.99475);
#5111=VECTOR('',#19185,1.99475);
#5112=VECTOR('',#19188,1.99475);
#5113=VECTOR('',#19191,1.99475);
#5114=VECTOR('',#19194,1.99475);
#5115=VECTOR('',#19197,1.99475);
#5116=VECTOR('',#19200,1.99475);
#5117=VECTOR('',#19203,1.99475);
#5118=VECTOR('',#19206,1.99475);
#5119=VECTOR('',#19209,1.99475);
#5120=VECTOR('',#19212,1.99475);
#5121=VECTOR('',#19215,1.99475);
#5122=VECTOR('',#19218,1.99475);
#5123=VECTOR('',#19221,1.99475);
#5124=VECTOR('',#19224,1.99475);
#5125=VECTOR('',#19259,2.2005);
#5126=VECTOR('',#19268,10.);
#5127=VECTOR('',#19269,10.);
#5128=VECTOR('',#19272,10.);
#5129=VECTOR('',#19273,10.);
#5130=VECTOR('',#19276,10.);
#5131=VECTOR('',#19281,4.25);
#5132=VECTOR('',#19286,10.);
#5133=VECTOR('',#19289,10.);
#5134=VECTOR('',#19292,10.);
#5135=VECTOR('',#19295,10.);
#5136=VECTOR('',#19298,10.);
#5137=VECTOR('',#19301,10.);
#5138=VECTOR('',#19304,10.);
#5139=VECTOR('',#19307,10.);
#5140=VECTOR('',#19310,10.);
#5141=VECTOR('',#19313,10.);
#5142=VECTOR('',#19316,10.);
#5143=VECTOR('',#19319,10.);
#5144=VECTOR('',#19322,10.);
#5145=VECTOR('',#19325,10.);
#5146=VECTOR('',#19328,10.);
#5147=VECTOR('',#19331,10.);
#5148=VECTOR('',#19334,10.);
#5149=VECTOR('',#19337,10.);
#5150=VECTOR('',#19340,10.);
#5151=VECTOR('',#19343,10.);
#5152=VECTOR('',#19346,10.);
#5153=VECTOR('',#19349,10.);
#5154=VECTOR('',#19352,10.);
#5155=VECTOR('',#19355,10.);
#5156=VECTOR('',#19358,10.);
#5157=VECTOR('',#19361,10.);
#5158=VECTOR('',#19364,10.);
#5159=VECTOR('',#19367,10.);
#5160=VECTOR('',#19370,10.);
#5161=VECTOR('',#19373,10.);
#5162=VECTOR('',#19376,10.);
#5163=VECTOR('',#19379,10.);
#5164=VECTOR('',#19382,10.);
#5165=VECTOR('',#19387,10.);
#5166=VECTOR('',#19390,10.);
#5167=VECTOR('',#19393,10.);
#5168=VECTOR('',#19396,10.);
#5169=VECTOR('',#19399,10.);
#5170=VECTOR('',#19402,10.);
#5171=VECTOR('',#19405,10.);
#5172=VECTOR('',#19408,10.);
#5173=VECTOR('',#19411,10.);
#5174=VECTOR('',#19414,10.);
#5175=VECTOR('',#19417,10.);
#5176=VECTOR('',#19420,10.);
#5177=VECTOR('',#19423,10.);
#5178=VECTOR('',#19426,10.);
#5179=VECTOR('',#19429,10.);
#5180=VECTOR('',#19432,10.);
#5181=VECTOR('',#19435,10.);
#5182=VECTOR('',#19438,10.);
#5183=VECTOR('',#19441,10.);
#5184=VECTOR('',#19444,10.);
#5185=VECTOR('',#19447,10.);
#5186=VECTOR('',#19450,10.);
#5187=VECTOR('',#19453,10.);
#5188=VECTOR('',#19456,10.);
#5189=VECTOR('',#19459,10.);
#5190=VECTOR('',#19462,10.);
#5191=VECTOR('',#19465,10.);
#5192=VECTOR('',#19468,10.);
#5193=VECTOR('',#19471,10.);
#5194=VECTOR('',#19474,10.);
#5195=VECTOR('',#19477,10.);
#5196=VECTOR('',#19480,10.);
#5197=VECTOR('',#19483,10.);
#5198=VECTOR('',#19486,10.);
#5199=VECTOR('',#19489,10.);
#5200=VECTOR('',#19492,10.);
#5201=VECTOR('',#19495,10.);
#5202=VECTOR('',#19498,10.);
#5203=VECTOR('',#19499,10.);
#5204=VECTOR('',#19502,10.);
#5205=VECTOR('',#19507,4.05);
#5206=VECTOR('',#19512,10.);
#5207=VECTOR('',#19513,10.);
#5208=VECTOR('',#19516,10.);
#5209=VECTOR('',#19521,10.);
#5210=VECTOR('',#19522,10.);
#5211=VECTOR('',#19525,10.);
#5212=VECTOR('',#19530,10.);
#5213=VECTOR('',#19531,10.);
#5214=VECTOR('',#19534,10.);
#5215=VECTOR('',#19539,10.);
#5216=VECTOR('',#19540,10.);
#5217=VECTOR('',#19543,10.);
#5218=VECTOR('',#19548,10.);
#5219=VECTOR('',#19549,9.99999999999999);
#5220=VECTOR('',#19552,10.);
#5221=VECTOR('',#19557,10.);
#5222=VECTOR('',#19558,10.);
#5223=VECTOR('',#19561,10.);
#5224=VECTOR('',#19566,10.);
#5225=VECTOR('',#19567,10.);
#5226=VECTOR('',#19570,10.);
#5227=VECTOR('',#19575,10.);
#5228=VECTOR('',#19576,10.);
#5229=VECTOR('',#19579,10.);
#5230=VECTOR('',#19584,10.);
#5231=VECTOR('',#19585,10.);
#5232=VECTOR('',#19588,10.);
#5233=VECTOR('',#19593,10.);
#5234=VECTOR('',#19594,10.);
#5235=VECTOR('',#19597,10.);
#5236=VECTOR('',#19602,10.);
#5237=VECTOR('',#19603,10.);
#5238=VECTOR('',#19606,10.);
#5239=VECTOR('',#19611,10.);
#5240=VECTOR('',#19612,10.);
#5241=VECTOR('',#19615,10.);
#5242=VECTOR('',#19620,10.);
#5243=VECTOR('',#19621,10.);
#5244=VECTOR('',#19624,10.);
#5245=VECTOR('',#19629,10.);
#5246=VECTOR('',#19630,10.);
#5247=VECTOR('',#19633,10.);
#5248=VECTOR('',#19638,10.);
#5249=VECTOR('',#19639,10.);
#5250=VECTOR('',#19642,10.);
#5251=VECTOR('',#19647,10.);
#5252=VECTOR('',#19648,10.);
#5253=VECTOR('',#19651,10.);
#5254=VECTOR('',#19656,10.);
#5255=VECTOR('',#19657,10.);
#5256=VECTOR('',#19660,10.);
#5257=VECTOR('',#19665,10.);
#5258=VECTOR('',#19666,10.);
#5259=VECTOR('',#19669,10.);
#5260=VECTOR('',#19674,10.);
#5261=VECTOR('',#19675,10.);
#5262=VECTOR('',#19678,10.);
#5263=VECTOR('',#19683,10.);
#5264=VECTOR('',#19684,10.);
#5265=VECTOR('',#19687,10.);
#5266=VECTOR('',#19692,10.);
#5267=VECTOR('',#19693,10.);
#5268=VECTOR('',#19696,10.);
#5269=VECTOR('',#19701,10.);
#5270=VECTOR('',#19702,10.);
#5271=VECTOR('',#19705,10.);
#5272=VECTOR('',#19710,10.);
#5273=VECTOR('',#19711,10.);
#5274=VECTOR('',#19714,10.);
#5275=VECTOR('',#19719,10.);
#5276=VECTOR('',#19720,10.);
#5277=VECTOR('',#19723,10.);
#5278=VECTOR('',#19728,10.);
#5279=VECTOR('',#19729,10.);
#5280=VECTOR('',#19732,10.);
#5281=VECTOR('',#19737,10.);
#5282=VECTOR('',#19738,10.);
#5283=VECTOR('',#19741,10.);
#5284=VECTOR('',#19746,10.);
#5285=VECTOR('',#19747,10.);
#5286=VECTOR('',#19750,10.);
#5287=VECTOR('',#19755,10.);
#5288=VECTOR('',#19756,10.);
#5289=VECTOR('',#19759,10.);
#5290=VECTOR('',#19764,10.);
#5291=VECTOR('',#19765,10.);
#5292=VECTOR('',#19768,10.);
#5293=VECTOR('',#19773,10.);
#5294=VECTOR('',#19774,10.);
#5295=VECTOR('',#19777,10.);
#5296=VECTOR('',#19782,10.);
#5297=VECTOR('',#19783,10.);
#5298=VECTOR('',#19786,10.);
#5299=VECTOR('',#19791,10.);
#5300=VECTOR('',#19792,10.);
#5301=VECTOR('',#19795,10.);
#5302=VECTOR('',#19800,10.);
#5303=VECTOR('',#19801,10.);
#5304=VECTOR('',#19804,10.);
#5305=VECTOR('',#19809,10.);
#5306=VECTOR('',#19810,10.);
#5307=VECTOR('',#19813,10.);
#5308=VECTOR('',#19838,2.40940107675851);
#5309=VECTOR('',#19841,10.);
#5310=VECTOR('',#19842,10.);
#5311=VECTOR('',#19847,10.);
#5312=VECTOR('',#19848,10.);
#5313=VECTOR('',#19853,10.);
#5314=VECTOR('',#19856,10.);
#5315=VECTOR('',#19859,10.);
#5316=VECTOR('',#19860,10.);
#5317=VECTOR('',#19865,10.);
#5318=VECTOR('',#19868,10.);
#5319=VECTOR('',#19871,10.);
#5320=VECTOR('',#19874,10.);
#5321=VECTOR('',#19877,10.);
#5322=VECTOR('',#19878,10.);
#5323=VECTOR('',#19879,10.);
#5324=VECTOR('',#19880,10.);
#5325=VECTOR('',#19883,10.);
#5326=VECTOR('',#19884,10.);
#5327=VECTOR('',#19885,10.);
#5328=VECTOR('',#19888,10.);
#5329=VECTOR('',#19889,10.);
#5330=VECTOR('',#19890,10.);
#5331=VECTOR('',#19897,10.);
#5332=VECTOR('',#19902,10.);
#5333=VECTOR('',#19905,10.);
#5334=VECTOR('',#19908,10.);
#5335=VECTOR('',#19925,10.);
#5336=VECTOR('',#19930,10.);
#5337=VECTOR('',#19935,2.30940107675851);
#5338=VECTOR('',#19938,10.);
#5339=VECTOR('',#19941,10.);
#5841=CIRCLE('',#16087,1.99475);
#5842=CIRCLE('',#16112,2.4505);
#5843=CIRCLE('',#16113,2.4505);
#5844=CIRCLE('',#16115,1.99475);
#5845=CIRCLE('',#16117,2.4505);
#5846=CIRCLE('',#16118,2.4505);
#5847=CIRCLE('',#16120,2.4505);
#5848=CIRCLE('',#16121,2.4505);
#5849=CIRCLE('',#16123,2.6505);
#5850=CIRCLE('',#16124,0.2);
#5851=CIRCLE('',#16126,4.05);
#5852=CIRCLE('',#16128,1.9505);
#5853=CIRCLE('',#16131,4.25);
#5854=CIRCLE('',#16135,4.25);
#5855=CIRCLE('',#16136,4.25);
#5856=CIRCLE('',#16137,4.25);
#5857=CIRCLE('',#16138,4.25);
#5858=CIRCLE('',#16139,4.25);
#5859=CIRCLE('',#16140,4.25);
#5860=CIRCLE('',#16141,4.25);
#5861=CIRCLE('',#16142,4.25);
#5862=CIRCLE('',#16143,4.25);
#5863=CIRCLE('',#16144,4.25);
#5864=CIRCLE('',#16145,4.25);
#5865=CIRCLE('',#16146,4.25);
#5866=CIRCLE('',#16147,4.25);
#5867=CIRCLE('',#16148,4.25);
#5868=CIRCLE('',#16149,4.25);
#5869=CIRCLE('',#16150,4.25);
#5870=CIRCLE('',#16151,4.25);
#5871=CIRCLE('',#16152,4.25);
#5872=CIRCLE('',#16153,4.25);
#5873=CIRCLE('',#16154,4.25);
#5874=CIRCLE('',#16155,4.25);
#5875=CIRCLE('',#16156,4.25);
#5876=CIRCLE('',#16157,4.25);
#5877=CIRCLE('',#16158,4.25);
#5878=CIRCLE('',#16159,4.25);
#5879=CIRCLE('',#16160,4.25);
#5880=CIRCLE('',#16161,4.25);
#5881=CIRCLE('',#16162,4.25);
#5882=CIRCLE('',#16163,4.25);
#5883=CIRCLE('',#16164,4.25);
#5884=CIRCLE('',#16165,4.25);
#5885=CIRCLE('',#16166,4.25);
#5886=CIRCLE('',#16167,4.25);
#5887=CIRCLE('',#16168,4.25);
#5888=CIRCLE('',#16169,4.25);
#5889=CIRCLE('',#16170,4.25);
#5890=CIRCLE('',#16171,4.25);
#5891=CIRCLE('',#16172,4.25);
#5892=CIRCLE('',#16173,4.25);
#5893=CIRCLE('',#16174,4.25);
#5894=CIRCLE('',#16175,4.25);
#5895=CIRCLE('',#16176,4.25);
#5896=CIRCLE('',#16177,4.25);
#5897=CIRCLE('',#16178,4.25);
#5898=CIRCLE('',#16179,4.25);
#5899=CIRCLE('',#16180,4.25);
#5900=CIRCLE('',#16181,4.25);
#5901=CIRCLE('',#16182,4.25);
#5902=CIRCLE('',#16183,4.25);
#5903=CIRCLE('',#16184,4.25);
#5904=CIRCLE('',#16185,4.25);
#5905=CIRCLE('',#16186,4.25);
#5906=CIRCLE('',#16187,4.25);
#5907=CIRCLE('',#16188,4.25);
#5908=CIRCLE('',#16189,4.25);
#5909=CIRCLE('',#16190,4.25);
#5910=CIRCLE('',#16191,4.25);
#5911=CIRCLE('',#16192,4.25);
#5912=CIRCLE('',#16193,4.25);
#5913=CIRCLE('',#16194,4.25);
#5914=CIRCLE('',#16195,4.25);
#5915=CIRCLE('',#16196,4.25);
#5916=CIRCLE('',#16197,4.25);
#5917=CIRCLE('',#16198,4.25);
#5918=CIRCLE('',#16199,4.25);
#5919=CIRCLE('',#16200,4.25);
#5920=CIRCLE('',#16201,4.25);
#5921=CIRCLE('',#16202,4.25);
#5922=CIRCLE('',#16203,4.25);
#5923=CIRCLE('',#16204,4.25);
#5924=CIRCLE('',#16205,4.25);
#5925=CIRCLE('',#16206,4.25);
#5926=CIRCLE('',#16207,4.25);
#5927=CIRCLE('',#16212,3.85);
#5928=CIRCLE('',#16316,0.2);
#5929=CIRCLE('',#16318,2.55940107675851);
#5930=CIRCLE('',#16320,2.2594010767585);
#5931=CIRCLE('',#16321,2.2594010767585);
#5932=CIRCLE('',#16322,2.2594010767585);
#5933=CIRCLE('',#16323,2.2594010767585);
#5934=CIRCLE('',#16324,2.2594010767585);
#5935=CIRCLE('',#16325,2.2594010767585);
#5936=CIRCLE('',#16327,2.2594010767585);
#5937=CIRCLE('',#16329,2.2594010767585);
#5938=CIRCLE('',#16331,2.2594010767585);
#5939=CIRCLE('',#16333,2.2594010767585);
#5940=CIRCLE('',#16335,2.2594010767585);
#5941=CIRCLE('',#16337,2.2594010767585);
#5942=CIRCLE('',#16348,2.30940107675851);
#5943=CIRCLE('',#16350,2.30940107675851);
#5944=CIRCLE('',#16352,2.30940107675851);
#5945=CIRCLE('',#16354,2.30940107675851);
#5946=CIRCLE('',#16356,2.30940107675851);
#5947=CIRCLE('',#16358,2.30940107675851);
#6808=VERTEX_POINT('',#23036);
#6809=VERTEX_POINT('',#23037);
#6810=VERTEX_POINT('',#23039);
#6811=VERTEX_POINT('',#23198);
#6812=VERTEX_POINT('',#23277);
#6813=VERTEX_POINT('',#23278);
#6814=VERTEX_POINT('',#23502);
#6815=VERTEX_POINT('',#23716);
#6816=VERTEX_POINT('',#23717);
#6817=VERTEX_POINT('',#23719);
#6818=VERTEX_POINT('',#24153);
#6819=VERTEX_POINT('',#24154);
#6820=VERTEX_POINT('',#24372);
#6821=VERTEX_POINT('',#24594);
#6822=VERTEX_POINT('',#24595);
#6823=VERTEX_POINT('',#24597);
#6824=VERTEX_POINT('',#25077);
#6825=VERTEX_POINT('',#25078);
#6826=VERTEX_POINT('',#25294);
#6827=VERTEX_POINT('',#25508);
#6828=VERTEX_POINT('',#25509);
#6829=VERTEX_POINT('',#25511);
#6830=VERTEX_POINT('',#25796);
#6831=VERTEX_POINT('',#25797);
#6832=VERTEX_POINT('',#25799);
#6833=VERTEX_POINT('',#25960);
#6834=VERTEX_POINT('',#26264);
#6835=VERTEX_POINT('',#26265);
#6836=VERTEX_POINT('',#26698);
#6837=VERTEX_POINT('',#26699);
#6838=VERTEX_POINT('',#26701);
#6839=VERTEX_POINT('',#26767);
#6840=VERTEX_POINT('',#26870);
#6841=VERTEX_POINT('',#26871);
#6842=VERTEX_POINT('',#26873);
#6843=VERTEX_POINT('',#27019);
#6844=VERTEX_POINT('',#27192);
#6845=VERTEX_POINT('',#27193);
#6846=VERTEX_POINT('',#27195);
#6847=VERTEX_POINT('',#27645);
#6848=VERTEX_POINT('',#27646);
#6849=VERTEX_POINT('',#27852);
#6850=VERTEX_POINT('',#28094);
#6851=VERTEX_POINT('',#28095);
#6852=VERTEX_POINT('',#28097);
#6853=VERTEX_POINT('',#28529);
#6854=VERTEX_POINT('',#28530);
#6855=VERTEX_POINT('',#28734);
#6856=VERTEX_POINT('',#28988);
#6857=VERTEX_POINT('',#28989);
#6858=VERTEX_POINT('',#28991);
#6859=VERTEX_POINT('',#29433);
#6860=VERTEX_POINT('',#29434);
#6861=VERTEX_POINT('',#29652);
#6862=VERTEX_POINT('',#29912);
#6863=VERTEX_POINT('',#29913);
#6864=VERTEX_POINT('',#29915);
#6865=VERTEX_POINT('',#30397);
#6866=VERTEX_POINT('',#30398);
#6867=VERTEX_POINT('',#30622);
#6868=VERTEX_POINT('',#30844);
#6869=VERTEX_POINT('',#30845);
#6870=VERTEX_POINT('',#30847);
#6871=VERTEX_POINT('',#31291);
#6872=VERTEX_POINT('',#31292);
#6873=VERTEX_POINT('',#31510);
#6874=VERTEX_POINT('',#31724);
#6875=VERTEX_POINT('',#31725);
#6876=VERTEX_POINT('',#31727);
#6877=VERTEX_POINT('',#32241);
#6878=VERTEX_POINT('',#32242);
#6879=VERTEX_POINT('',#32462);
#6880=VERTEX_POINT('',#32692);
#6881=VERTEX_POINT('',#32693);
#6882=VERTEX_POINT('',#32695);
#6883=VERTEX_POINT('',#32910);
#6884=VERTEX_POINT('',#32976);
#6885=VERTEX_POINT('',#32977);
#6886=VERTEX_POINT('',#32984);
#6887=VERTEX_POINT('',#32986);
#6888=VERTEX_POINT('',#32992);
#6889=VERTEX_POINT('',#33183);
#6890=VERTEX_POINT('',#33377);
#6891=VERTEX_POINT('',#33571);
#6892=VERTEX_POINT('',#33762);
#6893=VERTEX_POINT('',#33773);
#6894=VERTEX_POINT('',#33967);
#6895=VERTEX_POINT('',#34158);
#6896=VERTEX_POINT('',#34169);
#6897=VERTEX_POINT('',#34360);
#6898=VERTEX_POINT('',#34551);
#6899=VERTEX_POINT('',#34745);
#6900=VERTEX_POINT('',#34756);
#6901=VERTEX_POINT('',#34947);
#6902=VERTEX_POINT('',#35141);
#6903=VERTEX_POINT('',#35335);
#6904=VERTEX_POINT('',#35526);
#6905=VERTEX_POINT('',#35538);
#6906=VERTEX_POINT('',#35732);
#6907=VERTEX_POINT('',#35923);
#6908=VERTEX_POINT('',#35935);
#6909=VERTEX_POINT('',#36129);
#6910=VERTEX_POINT('',#36323);
#6911=VERTEX_POINT('',#36334);
#6912=VERTEX_POINT('',#36519);
#6913=VERTEX_POINT('',#36521);
#6914=VERTEX_POINT('',#36531);
#6915=VERTEX_POINT('',#36722);
#6916=VERTEX_POINT('',#36916);
#6917=VERTEX_POINT('',#37107);
#6918=VERTEX_POINT('',#37298);
#6919=VERTEX_POINT('',#37309);
#6920=VERTEX_POINT('',#37503);
#6921=VERTEX_POINT('',#37691);
#6922=VERTEX_POINT('',#37702);
#6923=VERTEX_POINT('',#37896);
#6924=VERTEX_POINT('',#38090);
#6925=VERTEX_POINT('',#38281);
#6926=VERTEX_POINT('',#38475);
#6927=VERTEX_POINT('',#38669);
#6928=VERTEX_POINT('',#38860);
#6929=VERTEX_POINT('',#39051);
#6930=VERTEX_POINT('',#39245);
#6931=VERTEX_POINT('',#39436);
#6932=VERTEX_POINT('',#39627);
#6933=VERTEX_POINT('',#39821);
#6934=VERTEX_POINT('',#40015);
#6935=VERTEX_POINT('',#40206);
#6936=VERTEX_POINT('',#40408);
#6937=VERTEX_POINT('',#40414);
#6938=VERTEX_POINT('',#40506);
#6939=VERTEX_POINT('',#40508);
#6940=VERTEX_POINT('',#40614);
#6941=VERTEX_POINT('',#40615);
#6942=VERTEX_POINT('',#41423);
#6943=VERTEX_POINT('',#41514);
#6944=VERTEX_POINT('',#41515);
#6945=VERTEX_POINT('',#42239);
#6946=VERTEX_POINT('',#42243);
#6947=VERTEX_POINT('',#42246);
#6948=VERTEX_POINT('',#42251);
#6949=VERTEX_POINT('',#42252);
#6950=VERTEX_POINT('',#42254);
#6951=VERTEX_POINT('',#42258);
#6952=VERTEX_POINT('',#42260);
#6953=VERTEX_POINT('',#42266);
#6954=VERTEX_POINT('',#42272);
#6955=VERTEX_POINT('',#42273);
#6956=VERTEX_POINT('',#42275);
#6957=VERTEX_POINT('',#42278);
#6958=VERTEX_POINT('',#42280);
#6959=VERTEX_POINT('',#42282);
#6960=VERTEX_POINT('',#42284);
#6961=VERTEX_POINT('',#42286);
#6962=VERTEX_POINT('',#42288);
#6963=VERTEX_POINT('',#42290);
#6964=VERTEX_POINT('',#42292);
#6965=VERTEX_POINT('',#42294);
#6966=VERTEX_POINT('',#42296);
#6967=VERTEX_POINT('',#42298);
#6968=VERTEX_POINT('',#42300);
#6969=VERTEX_POINT('',#42302);
#6970=VERTEX_POINT('',#42304);
#6971=VERTEX_POINT('',#42306);
#6972=VERTEX_POINT('',#42308);
#6973=VERTEX_POINT('',#42310);
#6974=VERTEX_POINT('',#42312);
#6975=VERTEX_POINT('',#42314);
#6976=VERTEX_POINT('',#42316);
#6977=VERTEX_POINT('',#42318);
#6978=VERTEX_POINT('',#42320);
#6979=VERTEX_POINT('',#42322);
#6980=VERTEX_POINT('',#42324);
#6981=VERTEX_POINT('',#42326);
#6982=VERTEX_POINT('',#42328);
#6983=VERTEX_POINT('',#42330);
#6984=VERTEX_POINT('',#42332);
#6985=VERTEX_POINT('',#42334);
#6986=VERTEX_POINT('',#42336);
#6987=VERTEX_POINT('',#42338);
#6988=VERTEX_POINT('',#42340);
#6989=VERTEX_POINT('',#42342);
#6990=VERTEX_POINT('',#42344);
#6991=VERTEX_POINT('',#42346);
#6992=VERTEX_POINT('',#42348);
#6993=VERTEX_POINT('',#42350);
#6994=VERTEX_POINT('',#42352);
#6995=VERTEX_POINT('',#42354);
#6996=VERTEX_POINT('',#42356);
#6997=VERTEX_POINT('',#42358);
#6998=VERTEX_POINT('',#42360);
#6999=VERTEX_POINT('',#42362);
#7000=VERTEX_POINT('',#42364);
#7001=VERTEX_POINT('',#42366);
#7002=VERTEX_POINT('',#42368);
#7003=VERTEX_POINT('',#42370);
#7004=VERTEX_POINT('',#42372);
#7005=VERTEX_POINT('',#42374);
#7006=VERTEX_POINT('',#42376);
#7007=VERTEX_POINT('',#42378);
#7008=VERTEX_POINT('',#42380);
#7009=VERTEX_POINT('',#42382);
#7010=VERTEX_POINT('',#42384);
#7011=VERTEX_POINT('',#42386);
#7012=VERTEX_POINT('',#42388);
#7013=VERTEX_POINT('',#42390);
#7014=VERTEX_POINT('',#42392);
#7015=VERTEX_POINT('',#42394);
#7016=VERTEX_POINT('',#42396);
#7017=VERTEX_POINT('',#42398);
#7018=VERTEX_POINT('',#42400);
#7019=VERTEX_POINT('',#42402);
#7020=VERTEX_POINT('',#42404);
#7021=VERTEX_POINT('',#42406);
#7022=VERTEX_POINT('',#42408);
#7023=VERTEX_POINT('',#42411);
#7024=VERTEX_POINT('',#42413);
#7025=VERTEX_POINT('',#42415);
#7026=VERTEX_POINT('',#42417);
#7027=VERTEX_POINT('',#42419);
#7028=VERTEX_POINT('',#42421);
#7029=VERTEX_POINT('',#42423);
#7030=VERTEX_POINT('',#42425);
#7031=VERTEX_POINT('',#42427);
#7032=VERTEX_POINT('',#42429);
#7033=VERTEX_POINT('',#42431);
#7034=VERTEX_POINT('',#42433);
#7035=VERTEX_POINT('',#42435);
#7036=VERTEX_POINT('',#42437);
#7037=VERTEX_POINT('',#42439);
#7038=VERTEX_POINT('',#42441);
#7039=VERTEX_POINT('',#42443);
#7040=VERTEX_POINT('',#42445);
#7041=VERTEX_POINT('',#42447);
#7042=VERTEX_POINT('',#42449);
#7043=VERTEX_POINT('',#42451);
#7044=VERTEX_POINT('',#42453);
#7045=VERTEX_POINT('',#42455);
#7046=VERTEX_POINT('',#42457);
#7047=VERTEX_POINT('',#42459);
#7048=VERTEX_POINT('',#42461);
#7049=VERTEX_POINT('',#42463);
#7050=VERTEX_POINT('',#42465);
#7051=VERTEX_POINT('',#42467);
#7052=VERTEX_POINT('',#42469);
#7053=VERTEX_POINT('',#42471);
#7054=VERTEX_POINT('',#42473);
#7055=VERTEX_POINT('',#42475);
#7056=VERTEX_POINT('',#42477);
#7057=VERTEX_POINT('',#42479);
#7058=VERTEX_POINT('',#42481);
#7059=VERTEX_POINT('',#42483);
#7060=VERTEX_POINT('',#42485);
#7061=VERTEX_POINT('',#42487);
#7062=VERTEX_POINT('',#42489);
#7063=VERTEX_POINT('',#42491);
#7064=VERTEX_POINT('',#42493);
#7065=VERTEX_POINT('',#42495);
#7066=VERTEX_POINT('',#42497);
#7067=VERTEX_POINT('',#42499);
#7068=VERTEX_POINT('',#42501);
#7069=VERTEX_POINT('',#42503);
#7070=VERTEX_POINT('',#42505);
#7071=VERTEX_POINT('',#42507);
#7072=VERTEX_POINT('',#42509);
#7073=VERTEX_POINT('',#42511);
#7074=VERTEX_POINT('',#42513);
#7075=VERTEX_POINT('',#42515);
#7076=VERTEX_POINT('',#42517);
#7077=VERTEX_POINT('',#42519);
#7078=VERTEX_POINT('',#42521);
#7079=VERTEX_POINT('',#42523);
#7080=VERTEX_POINT('',#42525);
#7081=VERTEX_POINT('',#42527);
#7082=VERTEX_POINT('',#42529);
#7083=VERTEX_POINT('',#42531);
#7084=VERTEX_POINT('',#42533);
#7085=VERTEX_POINT('',#42535);
#7086=VERTEX_POINT('',#42537);
#7087=VERTEX_POINT('',#42539);
#7088=VERTEX_POINT('',#42541);
#7089=VERTEX_POINT('',#42543);
#7090=VERTEX_POINT('',#42545);
#7091=VERTEX_POINT('',#42547);
#7092=VERTEX_POINT('',#42549);
#7093=VERTEX_POINT('',#42551);
#7094=VERTEX_POINT('',#42553);
#7095=VERTEX_POINT('',#42555);
#7096=VERTEX_POINT('',#42559);
#7097=VERTEX_POINT('',#42561);
#7098=VERTEX_POINT('',#42573);
#7099=VERTEX_POINT('',#42577);
#7100=VERTEX_POINT('',#42584);
#7101=VERTEX_POINT('',#42591);
#7102=VERTEX_POINT('',#42598);
#7103=VERTEX_POINT('',#42605);
#7104=VERTEX_POINT('',#42612);
#7105=VERTEX_POINT('',#42619);
#7106=VERTEX_POINT('',#42626);
#7107=VERTEX_POINT('',#42633);
#7108=VERTEX_POINT('',#42640);
#7109=VERTEX_POINT('',#42647);
#7110=VERTEX_POINT('',#42654);
#7111=VERTEX_POINT('',#42661);
#7112=VERTEX_POINT('',#42668);
#7113=VERTEX_POINT('',#42675);
#7114=VERTEX_POINT('',#42682);
#7115=VERTEX_POINT('',#42689);
#7116=VERTEX_POINT('',#42696);
#7117=VERTEX_POINT('',#42703);
#7118=VERTEX_POINT('',#42710);
#7119=VERTEX_POINT('',#42717);
#7120=VERTEX_POINT('',#42724);
#7121=VERTEX_POINT('',#42731);
#7122=VERTEX_POINT('',#42738);
#7123=VERTEX_POINT('',#42745);
#7124=VERTEX_POINT('',#42752);
#7125=VERTEX_POINT('',#42759);
#7126=VERTEX_POINT('',#42766);
#7127=VERTEX_POINT('',#42773);
#7128=VERTEX_POINT('',#42780);
#7129=VERTEX_POINT('',#42787);
#7130=VERTEX_POINT('',#42794);
#7131=VERTEX_POINT('',#42801);
#7132=VERTEX_POINT('',#42811);
#7133=VERTEX_POINT('',#42815);
#7134=VERTEX_POINT('',#42822);
#7135=VERTEX_POINT('',#42829);
#7136=VERTEX_POINT('',#42836);
#7137=VERTEX_POINT('',#42843);
#7138=VERTEX_POINT('',#42850);
#7139=VERTEX_POINT('',#42857);
#7140=VERTEX_POINT('',#42864);
#7141=VERTEX_POINT('',#42871);
#7142=VERTEX_POINT('',#42878);
#7143=VERTEX_POINT('',#42885);
#7144=VERTEX_POINT('',#42892);
#7145=VERTEX_POINT('',#42899);
#7146=VERTEX_POINT('',#42906);
#7147=VERTEX_POINT('',#42913);
#7148=VERTEX_POINT('',#42920);
#7149=VERTEX_POINT('',#42927);
#7150=VERTEX_POINT('',#42934);
#7151=VERTEX_POINT('',#42941);
#7152=VERTEX_POINT('',#42948);
#7153=VERTEX_POINT('',#42955);
#7154=VERTEX_POINT('',#42962);
#7155=VERTEX_POINT('',#42969);
#7156=VERTEX_POINT('',#42976);
#7157=VERTEX_POINT('',#42983);
#7158=VERTEX_POINT('',#42990);
#7159=VERTEX_POINT('',#42997);
#7160=VERTEX_POINT('',#43004);
#7161=VERTEX_POINT('',#43011);
#7162=VERTEX_POINT('',#43018);
#7163=VERTEX_POINT('',#43025);
#7164=VERTEX_POINT('',#43032);
#7165=VERTEX_POINT('',#43039);
#7166=VERTEX_POINT('',#43046);
#7167=VERTEX_POINT('',#43055);
#7168=VERTEX_POINT('',#43058);
#7169=VERTEX_POINT('',#43059);
#7170=VERTEX_POINT('',#43063);
#7171=VERTEX_POINT('',#43065);
#7172=VERTEX_POINT('',#43069);
#7173=VERTEX_POINT('',#43073);
#7174=VERTEX_POINT('',#43075);
#7175=VERTEX_POINT('',#43079);
#7176=VERTEX_POINT('',#43083);
#7177=VERTEX_POINT('',#43085);
#7178=VERTEX_POINT('',#43089);
#7179=VERTEX_POINT('',#43093);
#7180=VERTEX_POINT('',#43095);
#7181=VERTEX_POINT('',#43099);
#7182=VERTEX_POINT('',#43103);
#7183=VERTEX_POINT('',#43105);
#7184=VERTEX_POINT('',#43109);
#7185=VERTEX_POINT('',#43113);
#7186=VERTEX_POINT('',#43120);
#7187=VERTEX_POINT('',#43122);
#7188=VERTEX_POINT('',#43126);
#7189=VERTEX_POINT('',#43128);
#7190=VERTEX_POINT('',#43132);
#7191=VERTEX_POINT('',#43134);
#7192=VERTEX_POINT('',#43138);
#7193=VERTEX_POINT('',#43140);
#7194=VERTEX_POINT('',#43144);
#7195=VERTEX_POINT('',#43146);
#7196=VERTEX_POINT('',#43150);
#7197=VERTEX_POINT('',#43152);
#7198=VERTEX_POINT('',#43157);
#7199=VERTEX_POINT('',#43159);
#7200=VERTEX_POINT('',#43164);
#7201=VERTEX_POINT('',#43169);
#7202=VERTEX_POINT('',#43182);
#7203=VERTEX_POINT('',#43192);
#7204=VERTEX_POINT('',#43199);
#8754=EDGE_CURVE('',#6808,#6809,#3989,.T.);
#8755=EDGE_CURVE('',#6810,#6808,#408,.F.);
#8756=EDGE_CURVE('',#6811,#6810,#5841,.T.);
#8757=EDGE_CURVE('',#6811,#6809,#409,.T.);
#8758=EDGE_CURVE('',#6812,#6813,#3990,.T.);
#8759=EDGE_CURVE('',#6808,#6812,#410,.F.);
#8760=EDGE_CURVE('',#6809,#6814,#411,.T.);
#8761=EDGE_CURVE('',#6814,#6813,#412,.T.);
#8762=EDGE_CURVE('',#6815,#6816,#3991,.T.);
#8763=EDGE_CURVE('',#6817,#6815,#413,.F.);
#8764=EDGE_CURVE('',#6812,#6817,#414,.F.);
#8765=EDGE_CURVE('',#6813,#6816,#415,.T.);
#8766=EDGE_CURVE('',#6818,#6819,#3992,.T.);
#8767=EDGE_CURVE('',#6815,#6818,#416,.F.);
#8768=EDGE_CURVE('',#6816,#6820,#417,.T.);
#8769=EDGE_CURVE('',#6820,#6819,#418,.T.);
#8770=EDGE_CURVE('',#6821,#6822,#3993,.T.);
#8771=EDGE_CURVE('',#6823,#6821,#419,.F.);
#8772=EDGE_CURVE('',#6818,#6823,#420,.F.);
#8773=EDGE_CURVE('',#6819,#6822,#421,.T.);
#8774=EDGE_CURVE('',#6824,#6825,#3994,.T.);
#8775=EDGE_CURVE('',#6821,#6824,#422,.F.);
#8776=EDGE_CURVE('',#6822,#6826,#423,.T.);
#8777=EDGE_CURVE('',#6826,#6825,#424,.T.);
#8778=EDGE_CURVE('',#6827,#6828,#3995,.T.);
#8779=EDGE_CURVE('',#6829,#6827,#425,.T.);
#8780=EDGE_CURVE('',#6824,#6829,#426,.F.);
#8781=EDGE_CURVE('',#6825,#6828,#427,.T.);
#8782=EDGE_CURVE('',#6830,#6831,#3996,.T.);
#8783=EDGE_CURVE('',#6832,#6830,#428,.F.);
#8784=EDGE_CURVE('',#6827,#6832,#429,.T.);
#8785=EDGE_CURVE('',#6828,#6833,#430,.T.);
#8786=EDGE_CURVE('',#6833,#6831,#431,.T.);
#8787=EDGE_CURVE('',#6834,#6835,#3997,.T.);
#8788=EDGE_CURVE('',#6830,#6834,#432,.F.);
#8789=EDGE_CURVE('',#6831,#6835,#433,.T.);
#8790=EDGE_CURVE('',#6836,#6837,#3998,.T.);
#8791=EDGE_CURVE('',#6838,#6836,#434,.T.);
#8792=EDGE_CURVE('',#6834,#6838,#435,.F.);
#8793=EDGE_CURVE('',#6835,#6839,#436,.T.);
#8794=EDGE_CURVE('',#6839,#6837,#437,.T.);
#8795=EDGE_CURVE('',#6840,#6841,#3999,.T.);
#8796=EDGE_CURVE('',#6842,#6840,#438,.T.);
#8797=EDGE_CURVE('',#6836,#6842,#439,.T.);
#8798=EDGE_CURVE('',#6837,#6843,#440,.T.);
#8799=EDGE_CURVE('',#6843,#6841,#441,.T.);
#8800=EDGE_CURVE('',#6844,#6845,#4000,.T.);
#8801=EDGE_CURVE('',#6846,#6844,#442,.F.);
#8802=EDGE_CURVE('',#6840,#6846,#443,.T.);
#8803=EDGE_CURVE('',#6841,#6845,#444,.T.);
#8804=EDGE_CURVE('',#6847,#6848,#4001,.T.);
#8805=EDGE_CURVE('',#6844,#6847,#445,.F.);
#8806=EDGE_CURVE('',#6845,#6849,#446,.T.);
#8807=EDGE_CURVE('',#6849,#6848,#447,.T.);
#8808=EDGE_CURVE('',#6850,#6851,#4002,.T.);
#8809=EDGE_CURVE('',#6852,#6850,#448,.F.);
#8810=EDGE_CURVE('',#6847,#6852,#449,.F.);
#8811=EDGE_CURVE('',#6848,#6851,#450,.T.);
#8812=EDGE_CURVE('',#6853,#6854,#4003,.T.);
#8813=EDGE_CURVE('',#6850,#6853,#451,.F.);
#8814=EDGE_CURVE('',#6851,#6855,#452,.T.);
#8815=EDGE_CURVE('',#6855,#6854,#453,.T.);
#8816=EDGE_CURVE('',#6856,#6857,#4004,.T.);
#8817=EDGE_CURVE('',#6858,#6856,#454,.F.);
#8818=EDGE_CURVE('',#6853,#6858,#455,.F.);
#8819=EDGE_CURVE('',#6854,#6857,#456,.T.);
#8820=EDGE_CURVE('',#6859,#6860,#4005,.T.);
#8821=EDGE_CURVE('',#6856,#6859,#457,.F.);
#8822=EDGE_CURVE('',#6857,#6861,#458,.T.);
#8823=EDGE_CURVE('',#6861,#6860,#459,.T.);
#8824=EDGE_CURVE('',#6862,#6863,#4006,.T.);
#8825=EDGE_CURVE('',#6864,#6862,#460,.F.);
#8826=EDGE_CURVE('',#6859,#6864,#461,.F.);
#8827=EDGE_CURVE('',#6860,#6863,#462,.T.);
#8828=EDGE_CURVE('',#6865,#6866,#4007,.T.);
#8829=EDGE_CURVE('',#6862,#6865,#463,.F.);
#8830=EDGE_CURVE('',#6863,#6867,#464,.T.);
#8831=EDGE_CURVE('',#6867,#6866,#465,.T.);
#8832=EDGE_CURVE('',#6868,#6869,#4008,.T.);
#8833=EDGE_CURVE('',#6870,#6868,#466,.F.);
#8834=EDGE_CURVE('',#6865,#6870,#467,.F.);
#8835=EDGE_CURVE('',#6866,#6869,#468,.T.);
#8836=EDGE_CURVE('',#6871,#6872,#4009,.T.);
#8837=EDGE_CURVE('',#6868,#6871,#469,.F.);
#8838=EDGE_CURVE('',#6869,#6873,#470,.T.);
#8839=EDGE_CURVE('',#6873,#6872,#471,.T.);
#8840=EDGE_CURVE('',#6874,#6875,#4010,.T.);
#8841=EDGE_CURVE('',#6876,#6874,#472,.F.);
#8842=EDGE_CURVE('',#6871,#6876,#473,.F.);
#8843=EDGE_CURVE('',#6872,#6875,#474,.T.);
#8844=EDGE_CURVE('',#6877,#6878,#4011,.T.);
#8845=EDGE_CURVE('',#6874,#6877,#475,.F.);
#8846=EDGE_CURVE('',#6875,#6879,#476,.T.);
#8847=EDGE_CURVE('',#6879,#6878,#477,.T.);
#8848=EDGE_CURVE('',#6880,#6881,#4012,.T.);
#8849=EDGE_CURVE('',#6882,#6880,#478,.T.);
#8850=EDGE_CURVE('',#6877,#6882,#479,.F.);
#8851=EDGE_CURVE('',#6878,#6883,#480,.T.);
#8852=EDGE_CURVE('',#6883,#6881,#481,.T.);
#8853=EDGE_CURVE('',#6884,#6885,#482,.T.);
#8854=EDGE_CURVE('',#6886,#6885,#5842,.T.);
#8855=EDGE_CURVE('',#6886,#6887,#483,.T.);
#8856=EDGE_CURVE('',#6887,#6888,#484,.T.);
#8857=EDGE_CURVE('',#6888,#6889,#485,.T.);
#8858=EDGE_CURVE('',#6889,#6890,#486,.T.);
#8859=EDGE_CURVE('',#6890,#6891,#487,.T.);
#8860=EDGE_CURVE('',#6891,#6892,#488,.T.);
#8861=EDGE_CURVE('',#6892,#6893,#489,.T.);
#8862=EDGE_CURVE('',#6893,#6894,#490,.T.);
#8863=EDGE_CURVE('',#6894,#6895,#491,.T.);
#8864=EDGE_CURVE('',#6895,#6896,#492,.T.);
#8865=EDGE_CURVE('',#6896,#6897,#493,.T.);
#8866=EDGE_CURVE('',#6897,#6898,#494,.T.);
#8867=EDGE_CURVE('',#6898,#6899,#495,.T.);
#8868=EDGE_CURVE('',#6899,#6900,#496,.T.);
#8869=EDGE_CURVE('',#6900,#6901,#497,.T.);
#8870=EDGE_CURVE('',#6901,#6902,#498,.T.);
#8871=EDGE_CURVE('',#6902,#6903,#499,.T.);
#8872=EDGE_CURVE('',#6903,#6904,#500,.T.);
#8873=EDGE_CURVE('',#6904,#6905,#501,.T.);
#8874=EDGE_CURVE('',#6905,#6906,#502,.T.);
#8875=EDGE_CURVE('',#6906,#6907,#503,.T.);
#8876=EDGE_CURVE('',#6907,#6908,#504,.T.);
#8877=EDGE_CURVE('',#6908,#6909,#505,.T.);
#8878=EDGE_CURVE('',#6909,#6910,#506,.T.);
#8879=EDGE_CURVE('',#6910,#6911,#507,.T.);
#8880=EDGE_CURVE('',#6912,#6911,#5843,.T.);
#8881=EDGE_CURVE('',#6912,#6913,#508,.T.);
#8882=EDGE_CURVE('',#6913,#6914,#509,.T.);
#8883=EDGE_CURVE('',#6914,#6915,#510,.T.);
#8884=EDGE_CURVE('',#6915,#6916,#511,.T.);
#8885=EDGE_CURVE('',#6916,#6917,#512,.T.);
#8886=EDGE_CURVE('',#6917,#6918,#513,.T.);
#8887=EDGE_CURVE('',#6918,#6919,#514,.T.);
#8888=EDGE_CURVE('',#6919,#6920,#515,.T.);
#8889=EDGE_CURVE('',#6920,#6921,#516,.T.);
#8890=EDGE_CURVE('',#6921,#6922,#517,.T.);
#8891=EDGE_CURVE('',#6922,#6923,#518,.T.);
#8892=EDGE_CURVE('',#6923,#6924,#519,.T.);
#8893=EDGE_CURVE('',#6924,#6925,#520,.T.);
#8894=EDGE_CURVE('',#6925,#6926,#521,.T.);
#8895=EDGE_CURVE('',#6926,#6927,#522,.T.);
#8896=EDGE_CURVE('',#6927,#6928,#523,.T.);
#8897=EDGE_CURVE('',#6928,#6929,#524,.T.);
#8898=EDGE_CURVE('',#6929,#6930,#525,.T.);
#8899=EDGE_CURVE('',#6930,#6931,#526,.T.);
#8900=EDGE_CURVE('',#6931,#6932,#527,.T.);
#8901=EDGE_CURVE('',#6932,#6933,#528,.T.);
#8902=EDGE_CURVE('',#6933,#6934,#529,.T.);
#8903=EDGE_CURVE('',#6934,#6935,#530,.T.);
#8904=EDGE_CURVE('',#6935,#6884,#531,.T.);
#8905=EDGE_CURVE('',#6881,#6936,#532,.T.);
#8906=EDGE_CURVE('',#6936,#6937,#533,.T.);
#8907=EDGE_CURVE('',#6938,#6937,#5844,.T.);
#8908=EDGE_CURVE('',#6939,#6938,#534,.T.);
#8909=EDGE_CURVE('',#6880,#6939,#535,.T.);
#8910=EDGE_CURVE('',#6940,#6941,#5845,.T.);
#8911=EDGE_CURVE('',#6940,#6938,#536,.T.);
#8912=EDGE_CURVE('',#6937,#6912,#537,.T.);
#8913=EDGE_CURVE('',#6941,#6912,#5846,.T.);
#8914=EDGE_CURVE('',#6911,#6940,#538,.T.);
#8915=EDGE_CURVE('',#6942,#6886,#539,.T.);
#8916=EDGE_CURVE('',#6942,#6810,#540,.T.);
#8917=EDGE_CURVE('',#6943,#6944,#5847,.T.);
#8918=EDGE_CURVE('',#6943,#6811,#541,.T.);
#8919=EDGE_CURVE('',#6944,#6886,#5848,.T.);
#8920=EDGE_CURVE('',#6885,#6943,#542,.T.);
#8921=EDGE_CURVE('',#6945,#6945,#5849,.T.);
#8922=EDGE_CURVE('',#6945,#6944,#5850,.T.);
#8923=EDGE_CURVE('',#6946,#6946,#5851,.T.);
#8924=EDGE_CURVE('',#6941,#6947,#4013,.T.);
#8925=EDGE_CURVE('',#6947,#6947,#5852,.T.);
#8926=EDGE_CURVE('',#6948,#6949,#5853,.T.);
#8927=EDGE_CURVE('',#6950,#6948,#4014,.T.);
#8928=EDGE_CURVE('',#6949,#6950,#4015,.T.);
#8929=EDGE_CURVE('',#6949,#6951,#4016,.T.);
#8930=EDGE_CURVE('',#6952,#6950,#4017,.T.);
#8931=EDGE_CURVE('',#6951,#6952,#260,.T.);
#8932=EDGE_CURVE('',#6953,#6948,#4018,.T.);
#8933=EDGE_CURVE('',#6952,#6953,#261,.T.);
#8934=EDGE_CURVE('',#6954,#6955,#5854,.T.);
#8935=EDGE_CURVE('',#6955,#6956,#4019,.T.);
#8936=EDGE_CURVE('',#6956,#6956,#5855,.T.);
#8937=EDGE_CURVE('',#6955,#6957,#5856,.T.);
#8938=EDGE_CURVE('',#6957,#6958,#4020,.T.);
#8939=EDGE_CURVE('',#6959,#6958,#5857,.T.);
#8940=EDGE_CURVE('',#6959,#6960,#4021,.T.);
#8941=EDGE_CURVE('',#6960,#6961,#5858,.T.);
#8942=EDGE_CURVE('',#6961,#6962,#4022,.T.);
#8943=EDGE_CURVE('',#6963,#6962,#5859,.T.);
#8944=EDGE_CURVE('',#6963,#6964,#4023,.T.);
#8945=EDGE_CURVE('',#6964,#6965,#5860,.T.);
#8946=EDGE_CURVE('',#6965,#6966,#4024,.T.);
#8947=EDGE_CURVE('',#6967,#6966,#5861,.T.);
#8948=EDGE_CURVE('',#6967,#6968,#4025,.T.);
#8949=EDGE_CURVE('',#6968,#6969,#5862,.T.);
#8950=EDGE_CURVE('',#6969,#6970,#4026,.T.);
#8951=EDGE_CURVE('',#6971,#6970,#5863,.T.);
#8952=EDGE_CURVE('',#6971,#6972,#4027,.T.);
#8953=EDGE_CURVE('',#6972,#6973,#5864,.T.);
#8954=EDGE_CURVE('',#6973,#6974,#4028,.T.);
#8955=EDGE_CURVE('',#6975,#6974,#5865,.T.);
#8956=EDGE_CURVE('',#6975,#6976,#4029,.T.);
#8957=EDGE_CURVE('',#6976,#6977,#5866,.T.);
#8958=EDGE_CURVE('',#6977,#6978,#4030,.T.);
#8959=EDGE_CURVE('',#6979,#6978,#5867,.T.);
#8960=EDGE_CURVE('',#6979,#6980,#4031,.T.);
#8961=EDGE_CURVE('',#6980,#6981,#5868,.T.);
#8962=EDGE_CURVE('',#6981,#6982,#4032,.T.);
#8963=EDGE_CURVE('',#6983,#6982,#5869,.T.);
#8964=EDGE_CURVE('',#6983,#6984,#4033,.T.);
#8965=EDGE_CURVE('',#6984,#6985,#5870,.T.);
#8966=EDGE_CURVE('',#6985,#6986,#4034,.T.);
#8967=EDGE_CURVE('',#6987,#6986,#5871,.T.);
#8968=EDGE_CURVE('',#6987,#6988,#4035,.T.);
#8969=EDGE_CURVE('',#6988,#6989,#5872,.T.);
#8970=EDGE_CURVE('',#6989,#6990,#4036,.T.);
#8971=EDGE_CURVE('',#6991,#6990,#5873,.T.);
#8972=EDGE_CURVE('',#6991,#6992,#4037,.T.);
#8973=EDGE_CURVE('',#6992,#6993,#5874,.T.);
#8974=EDGE_CURVE('',#6993,#6994,#4038,.T.);
#8975=EDGE_CURVE('',#6995,#6994,#5875,.T.);
#8976=EDGE_CURVE('',#6995,#6996,#4039,.T.);
#8977=EDGE_CURVE('',#6996,#6997,#5876,.T.);
#8978=EDGE_CURVE('',#6997,#6998,#4040,.T.);
#8979=EDGE_CURVE('',#6999,#6998,#5877,.T.);
#8980=EDGE_CURVE('',#6999,#7000,#4041,.T.);
#8981=EDGE_CURVE('',#7000,#7001,#5878,.T.);
#8982=EDGE_CURVE('',#7001,#7002,#4042,.T.);
#8983=EDGE_CURVE('',#7003,#7002,#5879,.T.);
#8984=EDGE_CURVE('',#7003,#7004,#4043,.T.);
#8985=EDGE_CURVE('',#7004,#7005,#5880,.T.);
#8986=EDGE_CURVE('',#7005,#7006,#4044,.T.);
#8987=EDGE_CURVE('',#7007,#7006,#5881,.T.);
#8988=EDGE_CURVE('',#7007,#7008,#4045,.T.);
#8989=EDGE_CURVE('',#7008,#7009,#5882,.T.);
#8990=EDGE_CURVE('',#7009,#7010,#4046,.T.);
#8991=EDGE_CURVE('',#7011,#7010,#5883,.T.);
#8992=EDGE_CURVE('',#7011,#7012,#4047,.T.);
#8993=EDGE_CURVE('',#7012,#7013,#5884,.T.);
#8994=EDGE_CURVE('',#7013,#7014,#4048,.T.);
#8995=EDGE_CURVE('',#7015,#7014,#5885,.T.);
#8996=EDGE_CURVE('',#7015,#7016,#4049,.T.);
#8997=EDGE_CURVE('',#7016,#7017,#5886,.T.);
#8998=EDGE_CURVE('',#7017,#7018,#4050,.T.);
#8999=EDGE_CURVE('',#7019,#7018,#5887,.T.);
#9000=EDGE_CURVE('',#7019,#7020,#4051,.T.);
#9001=EDGE_CURVE('',#7020,#7021,#5888,.T.);
#9002=EDGE_CURVE('',#7021,#7022,#4052,.T.);
#9003=EDGE_CURVE('',#6953,#7022,#5889,.T.);
#9004=EDGE_CURVE('',#7023,#6951,#5890,.T.);
#9005=EDGE_CURVE('',#7023,#7024,#4053,.T.);
#9006=EDGE_CURVE('',#7024,#7025,#5891,.T.);
#9007=EDGE_CURVE('',#7025,#7026,#4054,.T.);
#9008=EDGE_CURVE('',#7027,#7026,#5892,.T.);
#9009=EDGE_CURVE('',#7027,#7028,#4055,.T.);
#9010=EDGE_CURVE('',#7028,#7029,#5893,.T.);
#9011=EDGE_CURVE('',#7029,#7030,#4056,.T.);
#9012=EDGE_CURVE('',#7031,#7030,#5894,.T.);
#9013=EDGE_CURVE('',#7031,#7032,#4057,.T.);
#9014=EDGE_CURVE('',#7032,#7033,#5895,.T.);
#9015=EDGE_CURVE('',#7033,#7034,#4058,.T.);
#9016=EDGE_CURVE('',#7035,#7034,#5896,.T.);
#9017=EDGE_CURVE('',#7035,#7036,#4059,.T.);
#9018=EDGE_CURVE('',#7036,#7037,#5897,.T.);
#9019=EDGE_CURVE('',#7037,#7038,#4060,.T.);
#9020=EDGE_CURVE('',#7039,#7038,#5898,.T.);
#9021=EDGE_CURVE('',#7039,#7040,#4061,.T.);
#9022=EDGE_CURVE('',#7040,#7041,#5899,.T.);
#9023=EDGE_CURVE('',#7041,#7042,#4062,.T.);
#9024=EDGE_CURVE('',#7043,#7042,#5900,.T.);
#9025=EDGE_CURVE('',#7043,#7044,#4063,.T.);
#9026=EDGE_CURVE('',#7044,#7045,#5901,.T.);
#9027=EDGE_CURVE('',#7045,#7046,#4064,.T.);
#9028=EDGE_CURVE('',#7047,#7046,#5902,.T.);
#9029=EDGE_CURVE('',#7047,#7048,#4065,.T.);
#9030=EDGE_CURVE('',#7048,#7049,#5903,.T.);
#9031=EDGE_CURVE('',#7049,#7050,#4066,.T.);
#9032=EDGE_CURVE('',#7051,#7050,#5904,.T.);
#9033=EDGE_CURVE('',#7051,#7052,#4067,.T.);
#9034=EDGE_CURVE('',#7052,#7053,#5905,.T.);
#9035=EDGE_CURVE('',#7053,#7054,#4068,.T.);
#9036=EDGE_CURVE('',#7055,#7054,#5906,.T.);
#9037=EDGE_CURVE('',#7055,#7056,#4069,.T.);
#9038=EDGE_CURVE('',#7056,#7057,#5907,.T.);
#9039=EDGE_CURVE('',#7057,#7058,#4070,.T.);
#9040=EDGE_CURVE('',#7059,#7058,#5908,.T.);
#9041=EDGE_CURVE('',#7059,#7060,#4071,.T.);
#9042=EDGE_CURVE('',#7060,#7061,#5909,.T.);
#9043=EDGE_CURVE('',#7061,#7062,#4072,.T.);
#9044=EDGE_CURVE('',#7063,#7062,#5910,.T.);
#9045=EDGE_CURVE('',#7063,#7064,#4073,.T.);
#9046=EDGE_CURVE('',#7064,#7065,#5911,.T.);
#9047=EDGE_CURVE('',#7065,#7066,#4074,.T.);
#9048=EDGE_CURVE('',#7067,#7066,#5912,.T.);
#9049=EDGE_CURVE('',#7067,#7068,#4075,.T.);
#9050=EDGE_CURVE('',#7068,#7069,#5913,.T.);
#9051=EDGE_CURVE('',#7069,#7070,#4076,.T.);
#9052=EDGE_CURVE('',#7071,#7070,#5914,.T.);
#9053=EDGE_CURVE('',#7071,#7072,#4077,.T.);
#9054=EDGE_CURVE('',#7072,#7073,#5915,.T.);
#9055=EDGE_CURVE('',#7073,#7074,#4078,.T.);
#9056=EDGE_CURVE('',#7075,#7074,#5916,.T.);
#9057=EDGE_CURVE('',#7075,#7076,#4079,.T.);
#9058=EDGE_CURVE('',#7076,#7077,#5917,.T.);
#9059=EDGE_CURVE('',#7077,#7078,#4080,.T.);
#9060=EDGE_CURVE('',#7079,#7078,#5918,.T.);
#9061=EDGE_CURVE('',#7079,#7080,#4081,.T.);
#9062=EDGE_CURVE('',#7080,#7081,#5919,.T.);
#9063=EDGE_CURVE('',#7081,#7082,#4082,.T.);
#9064=EDGE_CURVE('',#7083,#7082,#5920,.T.);
#9065=EDGE_CURVE('',#7083,#7084,#4083,.T.);
#9066=EDGE_CURVE('',#7084,#7085,#5921,.T.);
#9067=EDGE_CURVE('',#7085,#7086,#4084,.T.);
#9068=EDGE_CURVE('',#7087,#7086,#5922,.T.);
#9069=EDGE_CURVE('',#7087,#7088,#4085,.T.);
#9070=EDGE_CURVE('',#7088,#7089,#5923,.T.);
#9071=EDGE_CURVE('',#7089,#7090,#4086,.T.);
#9072=EDGE_CURVE('',#7091,#7090,#5924,.T.);
#9073=EDGE_CURVE('',#7091,#7092,#4087,.T.);
#9074=EDGE_CURVE('',#7092,#7093,#5925,.T.);
#9075=EDGE_CURVE('',#7093,#7094,#4088,.T.);
#9076=EDGE_CURVE('',#7095,#7094,#5926,.T.);
#9077=EDGE_CURVE('',#7095,#6954,#4089,.T.);
#9078=EDGE_CURVE('',#7021,#7096,#4090,.T.);
#9079=EDGE_CURVE('',#7097,#7096,#4091,.T.);
#9080=EDGE_CURVE('',#7022,#7097,#262,.T.);
#9081=EDGE_CURVE('',#7097,#7019,#263,.T.);
#9082=EDGE_CURVE('',#7096,#7020,#4092,.T.);
#9083=EDGE_CURVE('',#7098,#7095,#264,.T.);
#9084=EDGE_CURVE('',#7094,#7099,#265,.T.);
#9085=EDGE_CURVE('',#7099,#7091,#266,.T.);
#9086=EDGE_CURVE('',#7090,#7100,#267,.T.);
#9087=EDGE_CURVE('',#7100,#7087,#268,.T.);
#9088=EDGE_CURVE('',#7086,#7101,#269,.T.);
#9089=EDGE_CURVE('',#7101,#7083,#270,.T.);
#9090=EDGE_CURVE('',#7082,#7102,#271,.T.);
#9091=EDGE_CURVE('',#7102,#7079,#272,.T.);
#9092=EDGE_CURVE('',#7078,#7103,#273,.T.);
#9093=EDGE_CURVE('',#7103,#7075,#274,.T.);
#9094=EDGE_CURVE('',#7074,#7104,#275,.T.);
#9095=EDGE_CURVE('',#7104,#7071,#276,.T.);
#9096=EDGE_CURVE('',#7070,#7105,#277,.T.);
#9097=EDGE_CURVE('',#7105,#7067,#278,.T.);
#9098=EDGE_CURVE('',#7066,#7106,#279,.T.);
#9099=EDGE_CURVE('',#7106,#7063,#280,.T.);
#9100=EDGE_CURVE('',#7062,#7107,#281,.T.);
#9101=EDGE_CURVE('',#7107,#7059,#282,.T.);
#9102=EDGE_CURVE('',#7058,#7108,#283,.T.);
#9103=EDGE_CURVE('',#7108,#7055,#284,.T.);
#9104=EDGE_CURVE('',#7054,#7109,#285,.T.);
#9105=EDGE_CURVE('',#7109,#7051,#286,.T.);
#9106=EDGE_CURVE('',#7050,#7110,#287,.T.);
#9107=EDGE_CURVE('',#7110,#7047,#288,.T.);
#9108=EDGE_CURVE('',#7046,#7111,#289,.T.);
#9109=EDGE_CURVE('',#7111,#7043,#290,.T.);
#9110=EDGE_CURVE('',#7042,#7112,#291,.T.);
#9111=EDGE_CURVE('',#7112,#7039,#292,.T.);
#9112=EDGE_CURVE('',#7038,#7113,#293,.T.);
#9113=EDGE_CURVE('',#7113,#7035,#294,.T.);
#9114=EDGE_CURVE('',#7034,#7114,#295,.T.);
#9115=EDGE_CURVE('',#7114,#7031,#296,.T.);
#9116=EDGE_CURVE('',#7030,#7115,#297,.T.);
#9117=EDGE_CURVE('',#7115,#7027,#298,.T.);
#9118=EDGE_CURVE('',#7026,#7116,#299,.T.);
#9119=EDGE_CURVE('',#7116,#7023,#300,.T.);
#9120=EDGE_CURVE('',#7018,#7117,#301,.T.);
#9121=EDGE_CURVE('',#7117,#7015,#302,.T.);
#9122=EDGE_CURVE('',#7014,#7118,#303,.T.);
#9123=EDGE_CURVE('',#7118,#7011,#304,.T.);
#9124=EDGE_CURVE('',#7010,#7119,#305,.T.);
#9125=EDGE_CURVE('',#7119,#7007,#306,.T.);
#9126=EDGE_CURVE('',#7006,#7120,#307,.T.);
#9127=EDGE_CURVE('',#7120,#7003,#308,.T.);
#9128=EDGE_CURVE('',#7002,#7121,#309,.T.);
#9129=EDGE_CURVE('',#7121,#6999,#310,.T.);
#9130=EDGE_CURVE('',#6998,#7122,#311,.T.);
#9131=EDGE_CURVE('',#7122,#6995,#312,.T.);
#9132=EDGE_CURVE('',#6994,#7123,#313,.T.);
#9133=EDGE_CURVE('',#7123,#6991,#314,.T.);
#9134=EDGE_CURVE('',#6990,#7124,#315,.T.);
#9135=EDGE_CURVE('',#7124,#6987,#316,.T.);
#9136=EDGE_CURVE('',#6986,#7125,#317,.T.);
#9137=EDGE_CURVE('',#7125,#6983,#318,.T.);
#9138=EDGE_CURVE('',#6982,#7126,#319,.T.);
#9139=EDGE_CURVE('',#7126,#6979,#320,.T.);
#9140=EDGE_CURVE('',#6978,#7127,#321,.T.);
#9141=EDGE_CURVE('',#7127,#6975,#322,.T.);
#9142=EDGE_CURVE('',#6974,#7128,#323,.T.);
#9143=EDGE_CURVE('',#7128,#6971,#324,.T.);
#9144=EDGE_CURVE('',#6970,#7129,#325,.T.);
#9145=EDGE_CURVE('',#7129,#6967,#326,.T.);
#9146=EDGE_CURVE('',#6966,#7130,#327,.T.);
#9147=EDGE_CURVE('',#7130,#6963,#328,.T.);
#9148=EDGE_CURVE('',#6962,#7131,#329,.T.);
#9149=EDGE_CURVE('',#7131,#6959,#330,.T.);
#9150=EDGE_CURVE('',#6958,#7098,#331,.T.);
#9151=EDGE_CURVE('',#7098,#7132,#4093,.T.);
#9152=EDGE_CURVE('',#7132,#7132,#5927,.T.);
#9153=EDGE_CURVE('',#7133,#7016,#4094,.T.);
#9154=EDGE_CURVE('',#7017,#7133,#4095,.T.);
#9155=EDGE_CURVE('',#7117,#7133,#4096,.T.);
#9156=EDGE_CURVE('',#7013,#7134,#4097,.T.);
#9157=EDGE_CURVE('',#7118,#7134,#4098,.T.);
#9158=EDGE_CURVE('',#7134,#7012,#4099,.T.);
#9159=EDGE_CURVE('',#7135,#7008,#4100,.T.);
#9160=EDGE_CURVE('',#7009,#7135,#4101,.T.);
#9161=EDGE_CURVE('',#7119,#7135,#4102,.T.);
#9162=EDGE_CURVE('',#7005,#7136,#4103,.T.);
#9163=EDGE_CURVE('',#7120,#7136,#4104,.T.);
#9164=EDGE_CURVE('',#7136,#7004,#4105,.T.);
#9165=EDGE_CURVE('',#7137,#7000,#4106,.T.);
#9166=EDGE_CURVE('',#7001,#7137,#4107,.T.);
#9167=EDGE_CURVE('',#7121,#7137,#4108,.T.);
#9168=EDGE_CURVE('',#6997,#7138,#4109,.T.);
#9169=EDGE_CURVE('',#7122,#7138,#4110,.T.);
#9170=EDGE_CURVE('',#7138,#6996,#4111,.T.);
#9171=EDGE_CURVE('',#7139,#6992,#4112,.T.);
#9172=EDGE_CURVE('',#6993,#7139,#4113,.T.);
#9173=EDGE_CURVE('',#7123,#7139,#4114,.T.);
#9174=EDGE_CURVE('',#6989,#7140,#4115,.T.);
#9175=EDGE_CURVE('',#7124,#7140,#4116,.T.);
#9176=EDGE_CURVE('',#7140,#6988,#4117,.T.);
#9177=EDGE_CURVE('',#7141,#6984,#4118,.T.);
#9178=EDGE_CURVE('',#6985,#7141,#4119,.T.);
#9179=EDGE_CURVE('',#7125,#7141,#4120,.T.);
#9180=EDGE_CURVE('',#6981,#7142,#4121,.T.);
#9181=EDGE_CURVE('',#7126,#7142,#4122,.T.);
#9182=EDGE_CURVE('',#7142,#6980,#4123,.T.);
#9183=EDGE_CURVE('',#7143,#6976,#4124,.T.);
#9184=EDGE_CURVE('',#6977,#7143,#4125,.T.);
#9185=EDGE_CURVE('',#7127,#7143,#4126,.T.);
#9186=EDGE_CURVE('',#6973,#7144,#4127,.T.);
#9187=EDGE_CURVE('',#7128,#7144,#4128,.T.);
#9188=EDGE_CURVE('',#7144,#6972,#4129,.T.);
#9189=EDGE_CURVE('',#7145,#6968,#4130,.T.);
#9190=EDGE_CURVE('',#6969,#7145,#4131,.T.);
#9191=EDGE_CURVE('',#7129,#7145,#4132,.T.);
#9192=EDGE_CURVE('',#6965,#7146,#4133,.T.);
#9193=EDGE_CURVE('',#7130,#7146,#4134,.T.);
#9194=EDGE_CURVE('',#7146,#6964,#4135,.T.);
#9195=EDGE_CURVE('',#7147,#6960,#4136,.T.);
#9196=EDGE_CURVE('',#6961,#7147,#4137,.T.);
#9197=EDGE_CURVE('',#7131,#7147,#4138,.T.);
#9198=EDGE_CURVE('',#6957,#7148,#4139,.T.);
#9199=EDGE_CURVE('',#7098,#7148,#4140,.T.);
#9200=EDGE_CURVE('',#7148,#6954,#4141,.T.);
#9201=EDGE_CURVE('',#7149,#7092,#4142,.T.);
#9202=EDGE_CURVE('',#7093,#7149,#4143,.T.);
#9203=EDGE_CURVE('',#7099,#7149,#4144,.T.);
#9204=EDGE_CURVE('',#7089,#7150,#4145,.T.);
#9205=EDGE_CURVE('',#7100,#7150,#4146,.T.);
#9206=EDGE_CURVE('',#7150,#7088,#4147,.T.);
#9207=EDGE_CURVE('',#7151,#7084,#4148,.T.);
#9208=EDGE_CURVE('',#7085,#7151,#4149,.T.);
#9209=EDGE_CURVE('',#7101,#7151,#4150,.T.);
#9210=EDGE_CURVE('',#7081,#7152,#4151,.T.);
#9211=EDGE_CURVE('',#7102,#7152,#4152,.T.);
#9212=EDGE_CURVE('',#7152,#7080,#4153,.T.);
#9213=EDGE_CURVE('',#7153,#7076,#4154,.T.);
#9214=EDGE_CURVE('',#7077,#7153,#4155,.T.);
#9215=EDGE_CURVE('',#7103,#7153,#4156,.T.);
#9216=EDGE_CURVE('',#7073,#7154,#4157,.T.);
#9217=EDGE_CURVE('',#7104,#7154,#4158,.T.);
#9218=EDGE_CURVE('',#7154,#7072,#4159,.T.);
#9219=EDGE_CURVE('',#7155,#7068,#4160,.T.);
#9220=EDGE_CURVE('',#7069,#7155,#4161,.T.);
#9221=EDGE_CURVE('',#7105,#7155,#4162,.T.);
#9222=EDGE_CURVE('',#7065,#7156,#4163,.T.);
#9223=EDGE_CURVE('',#7106,#7156,#4164,.T.);
#9224=EDGE_CURVE('',#7156,#7064,#4165,.T.);
#9225=EDGE_CURVE('',#7157,#7060,#4166,.T.);
#9226=EDGE_CURVE('',#7061,#7157,#4167,.T.);
#9227=EDGE_CURVE('',#7107,#7157,#4168,.T.);
#9228=EDGE_CURVE('',#7057,#7158,#4169,.T.);
#9229=EDGE_CURVE('',#7108,#7158,#4170,.T.);
#9230=EDGE_CURVE('',#7158,#7056,#4171,.T.);
#9231=EDGE_CURVE('',#7159,#7052,#4172,.T.);
#9232=EDGE_CURVE('',#7053,#7159,#4173,.T.);
#9233=EDGE_CURVE('',#7109,#7159,#4174,.T.);
#9234=EDGE_CURVE('',#7049,#7160,#4175,.T.);
#9235=EDGE_CURVE('',#7110,#7160,#4176,.T.);
#9236=EDGE_CURVE('',#7160,#7048,#4177,.T.);
#9237=EDGE_CURVE('',#7161,#7044,#4178,.T.);
#9238=EDGE_CURVE('',#7045,#7161,#4179,.T.);
#9239=EDGE_CURVE('',#7111,#7161,#4180,.T.);
#9240=EDGE_CURVE('',#7041,#7162,#4181,.T.);
#9241=EDGE_CURVE('',#7112,#7162,#4182,.T.);
#9242=EDGE_CURVE('',#7162,#7040,#4183,.T.);
#9243=EDGE_CURVE('',#7163,#7036,#4184,.T.);
#9244=EDGE_CURVE('',#7037,#7163,#4185,.T.);
#9245=EDGE_CURVE('',#7113,#7163,#4186,.T.);
#9246=EDGE_CURVE('',#7033,#7164,#4187,.T.);
#9247=EDGE_CURVE('',#7114,#7164,#4188,.T.);
#9248=EDGE_CURVE('',#7164,#7032,#4189,.T.);
#9249=EDGE_CURVE('',#7165,#7028,#4190,.T.);
#9250=EDGE_CURVE('',#7029,#7165,#4191,.T.);
#9251=EDGE_CURVE('',#7115,#7165,#4192,.T.);
#9252=EDGE_CURVE('',#7025,#7166,#4193,.T.);
#9253=EDGE_CURVE('',#7116,#7166,#4194,.T.);
#9254=EDGE_CURVE('',#7166,#7024,#4195,.T.);
#9255=EDGE_CURVE('',#6946,#6956,#5928,.T.);
#9256=EDGE_CURVE('',#7167,#7167,#5929,.T.);
#9257=EDGE_CURVE('',#7168,#7169,#332,.T.);
#9258=EDGE_CURVE('',#7168,#7170,#5930,.T.);
#9259=EDGE_CURVE('',#7171,#7170,#333,.T.);
#9260=EDGE_CURVE('',#7172,#7171,#334,.T.);
#9261=EDGE_CURVE('',#7172,#7173,#5931,.T.);
#9262=EDGE_CURVE('',#7174,#7173,#335,.T.);
#9263=EDGE_CURVE('',#7175,#7174,#336,.T.);
#9264=EDGE_CURVE('',#7175,#7176,#5932,.T.);
#9265=EDGE_CURVE('',#7177,#7176,#337,.T.);
#9266=EDGE_CURVE('',#7178,#7177,#338,.T.);
#9267=EDGE_CURVE('',#7178,#7179,#5933,.T.);
#9268=EDGE_CURVE('',#7180,#7179,#339,.T.);
#9269=EDGE_CURVE('',#7181,#7180,#340,.T.);
#9270=EDGE_CURVE('',#7181,#7182,#5934,.T.);
#9271=EDGE_CURVE('',#7183,#7182,#341,.T.);
#9272=EDGE_CURVE('',#7184,#7183,#342,.T.);
#9273=EDGE_CURVE('',#7184,#7185,#5935,.T.);
#9274=EDGE_CURVE('',#7169,#7185,#343,.T.);
#9275=EDGE_CURVE('',#7169,#7167,#4196,.T.);
#9276=EDGE_CURVE('',#7176,#7186,#4197,.T.);
#9277=EDGE_CURVE('',#7187,#7175,#4198,.T.);
#9278=EDGE_CURVE('',#7186,#7187,#5936,.T.);
#9279=EDGE_CURVE('',#7179,#7188,#4199,.T.);
#9280=EDGE_CURVE('',#7189,#7178,#4200,.T.);
#9281=EDGE_CURVE('',#7188,#7189,#5937,.T.);
#9282=EDGE_CURVE('',#7190,#7172,#4201,.T.);
#9283=EDGE_CURVE('',#7191,#7190,#5938,.T.);
#9284=EDGE_CURVE('',#7173,#7191,#4202,.T.);
#9285=EDGE_CURVE('',#7182,#7192,#4203,.T.);
#9286=EDGE_CURVE('',#7193,#7181,#4204,.T.);
#9287=EDGE_CURVE('',#7192,#7193,#5939,.T.);
#9288=EDGE_CURVE('',#7194,#7168,#4205,.T.);
#9289=EDGE_CURVE('',#7195,#7194,#5940,.T.);
#9290=EDGE_CURVE('',#7170,#7195,#4206,.T.);
#9291=EDGE_CURVE('',#7196,#7184,#4207,.T.);
#9292=EDGE_CURVE('',#7197,#7196,#5941,.T.);
#9293=EDGE_CURVE('',#7185,#7197,#4208,.T.);
#9294=EDGE_CURVE('',#7193,#7192,#4209,.T.);
#9295=EDGE_CURVE('',#7180,#7198,#4210,.T.);
#9296=EDGE_CURVE('',#7198,#7199,#4211,.T.);
#9297=EDGE_CURVE('',#7183,#7199,#4212,.T.);
#9298=EDGE_CURVE('',#7189,#7188,#4213,.T.);
#9299=EDGE_CURVE('',#7177,#7200,#4214,.T.);
#9300=EDGE_CURVE('',#7200,#7198,#4215,.T.);
#9301=EDGE_CURVE('',#7187,#7186,#4216,.T.);
#9302=EDGE_CURVE('',#7174,#7201,#4217,.T.);
#9303=EDGE_CURVE('',#7201,#7200,#4218,.T.);
#9304=EDGE_CURVE('',#7190,#7191,#4219,.T.);
#9305=EDGE_CURVE('',#7194,#7195,#4220,.T.);
#9306=EDGE_CURVE('',#7196,#7197,#4221,.T.);
#9307=EDGE_CURVE('',#7202,#7201,#4222,.T.);
#9308=EDGE_CURVE('',#7202,#7201,#5942,.T.);
#9309=EDGE_CURVE('',#7201,#7200,#5943,.T.);
#9310=EDGE_CURVE('',#7200,#7198,#5944,.T.);
#9311=EDGE_CURVE('',#7198,#7199,#5945,.T.);
#9312=EDGE_CURVE('',#7199,#7203,#4223,.T.);
#9313=EDGE_CURVE('',#7199,#7203,#5946,.T.);
#9314=EDGE_CURVE('',#7203,#7202,#4224,.T.);
#9315=EDGE_CURVE('',#7203,#7202,#5947,.T.);
#9316=EDGE_CURVE('',#7204,#7203,#4225,.T.);
#9317=EDGE_CURVE('',#7171,#7202,#4226,.T.);
#9318=EDGE_CURVE('',#7169,#7203,#4227,.T.);
#12182=ORIENTED_EDGE('',*,*,#8754,.F.);
#12183=ORIENTED_EDGE('',*,*,#8755,.F.);
#12184=ORIENTED_EDGE('',*,*,#8756,.F.);
#12185=ORIENTED_EDGE('',*,*,#8757,.T.);
#12186=ORIENTED_EDGE('',*,*,#8758,.F.);
#12187=ORIENTED_EDGE('',*,*,#8759,.F.);
#12188=ORIENTED_EDGE('',*,*,#8754,.T.);
#12189=ORIENTED_EDGE('',*,*,#8760,.T.);
#12190=ORIENTED_EDGE('',*,*,#8761,.T.);
#12191=ORIENTED_EDGE('',*,*,#8762,.F.);
#12192=ORIENTED_EDGE('',*,*,#8763,.F.);
#12193=ORIENTED_EDGE('',*,*,#8764,.F.);
#12194=ORIENTED_EDGE('',*,*,#8758,.T.);
#12195=ORIENTED_EDGE('',*,*,#8765,.T.);
#12196=ORIENTED_EDGE('',*,*,#8766,.F.);
#12197=ORIENTED_EDGE('',*,*,#8767,.F.);
#12198=ORIENTED_EDGE('',*,*,#8762,.T.);
#12199=ORIENTED_EDGE('',*,*,#8768,.T.);
#12200=ORIENTED_EDGE('',*,*,#8769,.T.);
#12201=ORIENTED_EDGE('',*,*,#8770,.F.);
#12202=ORIENTED_EDGE('',*,*,#8771,.F.);
#12203=ORIENTED_EDGE('',*,*,#8772,.F.);
#12204=ORIENTED_EDGE('',*,*,#8766,.T.);
#12205=ORIENTED_EDGE('',*,*,#8773,.T.);
#12206=ORIENTED_EDGE('',*,*,#8774,.F.);
#12207=ORIENTED_EDGE('',*,*,#8775,.F.);
#12208=ORIENTED_EDGE('',*,*,#8770,.T.);
#12209=ORIENTED_EDGE('',*,*,#8776,.T.);
#12210=ORIENTED_EDGE('',*,*,#8777,.T.);
#12211=ORIENTED_EDGE('',*,*,#8778,.F.);
#12212=ORIENTED_EDGE('',*,*,#8779,.F.);
#12213=ORIENTED_EDGE('',*,*,#8780,.F.);
#12214=ORIENTED_EDGE('',*,*,#8774,.T.);
#12215=ORIENTED_EDGE('',*,*,#8781,.T.);
#12216=ORIENTED_EDGE('',*,*,#8782,.F.);
#12217=ORIENTED_EDGE('',*,*,#8783,.F.);
#12218=ORIENTED_EDGE('',*,*,#8784,.F.);
#12219=ORIENTED_EDGE('',*,*,#8778,.T.);
#12220=ORIENTED_EDGE('',*,*,#8785,.T.);
#12221=ORIENTED_EDGE('',*,*,#8786,.T.);
#12222=ORIENTED_EDGE('',*,*,#8787,.F.);
#12223=ORIENTED_EDGE('',*,*,#8788,.F.);
#12224=ORIENTED_EDGE('',*,*,#8782,.T.);
#12225=ORIENTED_EDGE('',*,*,#8789,.T.);
#12226=ORIENTED_EDGE('',*,*,#8790,.F.);
#12227=ORIENTED_EDGE('',*,*,#8791,.F.);
#12228=ORIENTED_EDGE('',*,*,#8792,.F.);
#12229=ORIENTED_EDGE('',*,*,#8787,.T.);
#12230=ORIENTED_EDGE('',*,*,#8793,.T.);
#12231=ORIENTED_EDGE('',*,*,#8794,.T.);
#12232=ORIENTED_EDGE('',*,*,#8795,.F.);
#12233=ORIENTED_EDGE('',*,*,#8796,.F.);
#12234=ORIENTED_EDGE('',*,*,#8797,.F.);
#12235=ORIENTED_EDGE('',*,*,#8790,.T.);
#12236=ORIENTED_EDGE('',*,*,#8798,.T.);
#12237=ORIENTED_EDGE('',*,*,#8799,.T.);
#12238=ORIENTED_EDGE('',*,*,#8800,.F.);
#12239=ORIENTED_EDGE('',*,*,#8801,.F.);
#12240=ORIENTED_EDGE('',*,*,#8802,.F.);
#12241=ORIENTED_EDGE('',*,*,#8795,.T.);
#12242=ORIENTED_EDGE('',*,*,#8803,.T.);
#12243=ORIENTED_EDGE('',*,*,#8804,.F.);
#12244=ORIENTED_EDGE('',*,*,#8805,.F.);
#12245=ORIENTED_EDGE('',*,*,#8800,.T.);
#12246=ORIENTED_EDGE('',*,*,#8806,.T.);
#12247=ORIENTED_EDGE('',*,*,#8807,.T.);
#12248=ORIENTED_EDGE('',*,*,#8808,.F.);
#12249=ORIENTED_EDGE('',*,*,#8809,.F.);
#12250=ORIENTED_EDGE('',*,*,#8810,.F.);
#12251=ORIENTED_EDGE('',*,*,#8804,.T.);
#12252=ORIENTED_EDGE('',*,*,#8811,.T.);
#12253=ORIENTED_EDGE('',*,*,#8812,.F.);
#12254=ORIENTED_EDGE('',*,*,#8813,.F.);
#12255=ORIENTED_EDGE('',*,*,#8808,.T.);
#12256=ORIENTED_EDGE('',*,*,#8814,.T.);
#12257=ORIENTED_EDGE('',*,*,#8815,.T.);
#12258=ORIENTED_EDGE('',*,*,#8816,.F.);
#12259=ORIENTED_EDGE('',*,*,#8817,.F.);
#12260=ORIENTED_EDGE('',*,*,#8818,.F.);
#12261=ORIENTED_EDGE('',*,*,#8812,.T.);
#12262=ORIENTED_EDGE('',*,*,#8819,.T.);
#12263=ORIENTED_EDGE('',*,*,#8820,.F.);
#12264=ORIENTED_EDGE('',*,*,#8821,.F.);
#12265=ORIENTED_EDGE('',*,*,#8816,.T.);
#12266=ORIENTED_EDGE('',*,*,#8822,.T.);
#12267=ORIENTED_EDGE('',*,*,#8823,.T.);
#12268=ORIENTED_EDGE('',*,*,#8824,.F.);
#12269=ORIENTED_EDGE('',*,*,#8825,.F.);
#12270=ORIENTED_EDGE('',*,*,#8826,.F.);
#12271=ORIENTED_EDGE('',*,*,#8820,.T.);
#12272=ORIENTED_EDGE('',*,*,#8827,.T.);
#12273=ORIENTED_EDGE('',*,*,#8828,.F.);
#12274=ORIENTED_EDGE('',*,*,#8829,.F.);
#12275=ORIENTED_EDGE('',*,*,#8824,.T.);
#12276=ORIENTED_EDGE('',*,*,#8830,.T.);
#12277=ORIENTED_EDGE('',*,*,#8831,.T.);
#12278=ORIENTED_EDGE('',*,*,#8832,.F.);
#12279=ORIENTED_EDGE('',*,*,#8833,.F.);
#12280=ORIENTED_EDGE('',*,*,#8834,.F.);
#12281=ORIENTED_EDGE('',*,*,#8828,.T.);
#12282=ORIENTED_EDGE('',*,*,#8835,.T.);
#12283=ORIENTED_EDGE('',*,*,#8836,.F.);
#12284=ORIENTED_EDGE('',*,*,#8837,.F.);
#12285=ORIENTED_EDGE('',*,*,#8832,.T.);
#12286=ORIENTED_EDGE('',*,*,#8838,.T.);
#12287=ORIENTED_EDGE('',*,*,#8839,.T.);
#12288=ORIENTED_EDGE('',*,*,#8840,.F.);
#12289=ORIENTED_EDGE('',*,*,#8841,.F.);
#12290=ORIENTED_EDGE('',*,*,#8842,.F.);
#12291=ORIENTED_EDGE('',*,*,#8836,.T.);
#12292=ORIENTED_EDGE('',*,*,#8843,.T.);
#12293=ORIENTED_EDGE('',*,*,#8844,.F.);
#12294=ORIENTED_EDGE('',*,*,#8845,.F.);
#12295=ORIENTED_EDGE('',*,*,#8840,.T.);
#12296=ORIENTED_EDGE('',*,*,#8846,.T.);
#12297=ORIENTED_EDGE('',*,*,#8847,.T.);
#12298=ORIENTED_EDGE('',*,*,#8848,.F.);
#12299=ORIENTED_EDGE('',*,*,#8849,.F.);
#12300=ORIENTED_EDGE('',*,*,#8850,.F.);
#12301=ORIENTED_EDGE('',*,*,#8844,.T.);
#12302=ORIENTED_EDGE('',*,*,#8851,.T.);
#12303=ORIENTED_EDGE('',*,*,#8852,.T.);
#12304=ORIENTED_EDGE('',*,*,#8853,.T.);
#12305=ORIENTED_EDGE('',*,*,#8854,.F.);
#12306=ORIENTED_EDGE('',*,*,#8855,.T.);
#12307=ORIENTED_EDGE('',*,*,#8856,.T.);
#12308=ORIENTED_EDGE('',*,*,#8857,.T.);
#12309=ORIENTED_EDGE('',*,*,#8858,.T.);
#12310=ORIENTED_EDGE('',*,*,#8859,.T.);
#12311=ORIENTED_EDGE('',*,*,#8860,.T.);
#12312=ORIENTED_EDGE('',*,*,#8861,.T.);
#12313=ORIENTED_EDGE('',*,*,#8862,.T.);
#12314=ORIENTED_EDGE('',*,*,#8863,.T.);
#12315=ORIENTED_EDGE('',*,*,#8864,.T.);
#12316=ORIENTED_EDGE('',*,*,#8865,.T.);
#12317=ORIENTED_EDGE('',*,*,#8866,.T.);
#12318=ORIENTED_EDGE('',*,*,#8867,.T.);
#12319=ORIENTED_EDGE('',*,*,#8868,.T.);
#12320=ORIENTED_EDGE('',*,*,#8869,.T.);
#12321=ORIENTED_EDGE('',*,*,#8870,.T.);
#12322=ORIENTED_EDGE('',*,*,#8871,.T.);
#12323=ORIENTED_EDGE('',*,*,#8872,.T.);
#12324=ORIENTED_EDGE('',*,*,#8873,.T.);
#12325=ORIENTED_EDGE('',*,*,#8874,.T.);
#12326=ORIENTED_EDGE('',*,*,#8875,.T.);
#12327=ORIENTED_EDGE('',*,*,#8876,.T.);
#12328=ORIENTED_EDGE('',*,*,#8877,.T.);
#12329=ORIENTED_EDGE('',*,*,#8878,.T.);
#12330=ORIENTED_EDGE('',*,*,#8879,.T.);
#12331=ORIENTED_EDGE('',*,*,#8880,.F.);
#12332=ORIENTED_EDGE('',*,*,#8881,.T.);
#12333=ORIENTED_EDGE('',*,*,#8882,.T.);
#12334=ORIENTED_EDGE('',*,*,#8883,.T.);
#12335=ORIENTED_EDGE('',*,*,#8884,.T.);
#12336=ORIENTED_EDGE('',*,*,#8885,.T.);
#12337=ORIENTED_EDGE('',*,*,#8886,.T.);
#12338=ORIENTED_EDGE('',*,*,#8887,.T.);
#12339=ORIENTED_EDGE('',*,*,#8888,.T.);
#12340=ORIENTED_EDGE('',*,*,#8889,.T.);
#12341=ORIENTED_EDGE('',*,*,#8890,.T.);
#12342=ORIENTED_EDGE('',*,*,#8891,.T.);
#12343=ORIENTED_EDGE('',*,*,#8892,.T.);
#12344=ORIENTED_EDGE('',*,*,#8893,.T.);
#12345=ORIENTED_EDGE('',*,*,#8894,.T.);
#12346=ORIENTED_EDGE('',*,*,#8895,.T.);
#12347=ORIENTED_EDGE('',*,*,#8896,.T.);
#12348=ORIENTED_EDGE('',*,*,#8897,.T.);
#12349=ORIENTED_EDGE('',*,*,#8898,.T.);
#12350=ORIENTED_EDGE('',*,*,#8899,.T.);
#12351=ORIENTED_EDGE('',*,*,#8900,.T.);
#12352=ORIENTED_EDGE('',*,*,#8901,.T.);
#12353=ORIENTED_EDGE('',*,*,#8902,.T.);
#12354=ORIENTED_EDGE('',*,*,#8903,.T.);
#12355=ORIENTED_EDGE('',*,*,#8904,.T.);
#12356=ORIENTED_EDGE('',*,*,#8848,.T.);
#12357=ORIENTED_EDGE('',*,*,#8905,.T.);
#12358=ORIENTED_EDGE('',*,*,#8906,.T.);
#12359=ORIENTED_EDGE('',*,*,#8907,.F.);
#12360=ORIENTED_EDGE('',*,*,#8908,.F.);
#12361=ORIENTED_EDGE('',*,*,#8909,.F.);
#12362=ORIENTED_EDGE('',*,*,#8910,.F.);
#12363=ORIENTED_EDGE('',*,*,#8911,.T.);
#12364=ORIENTED_EDGE('',*,*,#8907,.T.);
#12365=ORIENTED_EDGE('',*,*,#8912,.T.);
#12366=ORIENTED_EDGE('',*,*,#8913,.F.);
#12367=ORIENTED_EDGE('',*,*,#8911,.F.);
#12368=ORIENTED_EDGE('',*,*,#8914,.F.);
#12369=ORIENTED_EDGE('',*,*,#8879,.F.);
#12370=ORIENTED_EDGE('',*,*,#8878,.F.);
#12371=ORIENTED_EDGE('',*,*,#8877,.F.);
#12372=ORIENTED_EDGE('',*,*,#8876,.F.);
#12373=ORIENTED_EDGE('',*,*,#8875,.F.);
#12374=ORIENTED_EDGE('',*,*,#8874,.F.);
#12375=ORIENTED_EDGE('',*,*,#8873,.F.);
#12376=ORIENTED_EDGE('',*,*,#8872,.F.);
#12377=ORIENTED_EDGE('',*,*,#8871,.F.);
#12378=ORIENTED_EDGE('',*,*,#8870,.F.);
#12379=ORIENTED_EDGE('',*,*,#8869,.F.);
#12380=ORIENTED_EDGE('',*,*,#8868,.F.);
#12381=ORIENTED_EDGE('',*,*,#8867,.F.);
#12382=ORIENTED_EDGE('',*,*,#8866,.F.);
#12383=ORIENTED_EDGE('',*,*,#8865,.F.);
#12384=ORIENTED_EDGE('',*,*,#8864,.F.);
#12385=ORIENTED_EDGE('',*,*,#8863,.F.);
#12386=ORIENTED_EDGE('',*,*,#8862,.F.);
#12387=ORIENTED_EDGE('',*,*,#8861,.F.);
#12388=ORIENTED_EDGE('',*,*,#8860,.F.);
#12389=ORIENTED_EDGE('',*,*,#8859,.F.);
#12390=ORIENTED_EDGE('',*,*,#8858,.F.);
#12391=ORIENTED_EDGE('',*,*,#8857,.F.);
#12392=ORIENTED_EDGE('',*,*,#8856,.F.);
#12393=ORIENTED_EDGE('',*,*,#8855,.F.);
#12394=ORIENTED_EDGE('',*,*,#8915,.F.);
#12395=ORIENTED_EDGE('',*,*,#8916,.T.);
#12396=ORIENTED_EDGE('',*,*,#8755,.T.);
#12397=ORIENTED_EDGE('',*,*,#8759,.T.);
#12398=ORIENTED_EDGE('',*,*,#8764,.T.);
#12399=ORIENTED_EDGE('',*,*,#8763,.T.);
#12400=ORIENTED_EDGE('',*,*,#8767,.T.);
#12401=ORIENTED_EDGE('',*,*,#8772,.T.);
#12402=ORIENTED_EDGE('',*,*,#8771,.T.);
#12403=ORIENTED_EDGE('',*,*,#8775,.T.);
#12404=ORIENTED_EDGE('',*,*,#8780,.T.);
#12405=ORIENTED_EDGE('',*,*,#8779,.T.);
#12406=ORIENTED_EDGE('',*,*,#8784,.T.);
#12407=ORIENTED_EDGE('',*,*,#8783,.T.);
#12408=ORIENTED_EDGE('',*,*,#8788,.T.);
#12409=ORIENTED_EDGE('',*,*,#8792,.T.);
#12410=ORIENTED_EDGE('',*,*,#8791,.T.);
#12411=ORIENTED_EDGE('',*,*,#8797,.T.);
#12412=ORIENTED_EDGE('',*,*,#8796,.T.);
#12413=ORIENTED_EDGE('',*,*,#8802,.T.);
#12414=ORIENTED_EDGE('',*,*,#8801,.T.);
#12415=ORIENTED_EDGE('',*,*,#8805,.T.);
#12416=ORIENTED_EDGE('',*,*,#8810,.T.);
#12417=ORIENTED_EDGE('',*,*,#8809,.T.);
#12418=ORIENTED_EDGE('',*,*,#8813,.T.);
#12419=ORIENTED_EDGE('',*,*,#8818,.T.);
#12420=ORIENTED_EDGE('',*,*,#8817,.T.);
#12421=ORIENTED_EDGE('',*,*,#8821,.T.);
#12422=ORIENTED_EDGE('',*,*,#8826,.T.);
#12423=ORIENTED_EDGE('',*,*,#8825,.T.);
#12424=ORIENTED_EDGE('',*,*,#8829,.T.);
#12425=ORIENTED_EDGE('',*,*,#8834,.T.);
#12426=ORIENTED_EDGE('',*,*,#8833,.T.);
#12427=ORIENTED_EDGE('',*,*,#8837,.T.);
#12428=ORIENTED_EDGE('',*,*,#8842,.T.);
#12429=ORIENTED_EDGE('',*,*,#8841,.T.);
#12430=ORIENTED_EDGE('',*,*,#8845,.T.);
#12431=ORIENTED_EDGE('',*,*,#8850,.T.);
#12432=ORIENTED_EDGE('',*,*,#8849,.T.);
#12433=ORIENTED_EDGE('',*,*,#8909,.T.);
#12434=ORIENTED_EDGE('',*,*,#8908,.T.);
#12435=ORIENTED_EDGE('',*,*,#8917,.F.);
#12436=ORIENTED_EDGE('',*,*,#8918,.T.);
#12437=ORIENTED_EDGE('',*,*,#8756,.T.);
#12438=ORIENTED_EDGE('',*,*,#8916,.F.);
#12439=ORIENTED_EDGE('',*,*,#8915,.T.);
#12440=ORIENTED_EDGE('',*,*,#8919,.F.);
#12441=ORIENTED_EDGE('',*,*,#8912,.F.);
#12442=ORIENTED_EDGE('',*,*,#8906,.F.);
#12443=ORIENTED_EDGE('',*,*,#8905,.F.);
#12444=ORIENTED_EDGE('',*,*,#8852,.F.);
#12445=ORIENTED_EDGE('',*,*,#8851,.F.);
#12446=ORIENTED_EDGE('',*,*,#8847,.F.);
#12447=ORIENTED_EDGE('',*,*,#8846,.F.);
#12448=ORIENTED_EDGE('',*,*,#8843,.F.);
#12449=ORIENTED_EDGE('',*,*,#8839,.F.);
#12450=ORIENTED_EDGE('',*,*,#8838,.F.);
#12451=ORIENTED_EDGE('',*,*,#8835,.F.);
#12452=ORIENTED_EDGE('',*,*,#8831,.F.);
#12453=ORIENTED_EDGE('',*,*,#8830,.F.);
#12454=ORIENTED_EDGE('',*,*,#8827,.F.);
#12455=ORIENTED_EDGE('',*,*,#8823,.F.);
#12456=ORIENTED_EDGE('',*,*,#8822,.F.);
#12457=ORIENTED_EDGE('',*,*,#8819,.F.);
#12458=ORIENTED_EDGE('',*,*,#8815,.F.);
#12459=ORIENTED_EDGE('',*,*,#8814,.F.);
#12460=ORIENTED_EDGE('',*,*,#8811,.F.);
#12461=ORIENTED_EDGE('',*,*,#8807,.F.);
#12462=ORIENTED_EDGE('',*,*,#8806,.F.);
#12463=ORIENTED_EDGE('',*,*,#8803,.F.);
#12464=ORIENTED_EDGE('',*,*,#8799,.F.);
#12465=ORIENTED_EDGE('',*,*,#8798,.F.);
#12466=ORIENTED_EDGE('',*,*,#8794,.F.);
#12467=ORIENTED_EDGE('',*,*,#8793,.F.);
#12468=ORIENTED_EDGE('',*,*,#8789,.F.);
#12469=ORIENTED_EDGE('',*,*,#8786,.F.);
#12470=ORIENTED_EDGE('',*,*,#8785,.F.);
#12471=ORIENTED_EDGE('',*,*,#8781,.F.);
#12472=ORIENTED_EDGE('',*,*,#8777,.F.);
#12473=ORIENTED_EDGE('',*,*,#8776,.F.);
#12474=ORIENTED_EDGE('',*,*,#8773,.F.);
#12475=ORIENTED_EDGE('',*,*,#8769,.F.);
#12476=ORIENTED_EDGE('',*,*,#8768,.F.);
#12477=ORIENTED_EDGE('',*,*,#8765,.F.);
#12478=ORIENTED_EDGE('',*,*,#8761,.F.);
#12479=ORIENTED_EDGE('',*,*,#8760,.F.);
#12480=ORIENTED_EDGE('',*,*,#8757,.F.);
#12481=ORIENTED_EDGE('',*,*,#8918,.F.);
#12482=ORIENTED_EDGE('',*,*,#8920,.F.);
#12483=ORIENTED_EDGE('',*,*,#8853,.F.);
#12484=ORIENTED_EDGE('',*,*,#8904,.F.);
#12485=ORIENTED_EDGE('',*,*,#8903,.F.);
#12486=ORIENTED_EDGE('',*,*,#8902,.F.);
#12487=ORIENTED_EDGE('',*,*,#8901,.F.);
#12488=ORIENTED_EDGE('',*,*,#8900,.F.);
#12489=ORIENTED_EDGE('',*,*,#8899,.F.);
#12490=ORIENTED_EDGE('',*,*,#8898,.F.);
#12491=ORIENTED_EDGE('',*,*,#8897,.F.);
#12492=ORIENTED_EDGE('',*,*,#8896,.F.);
#12493=ORIENTED_EDGE('',*,*,#8895,.F.);
#12494=ORIENTED_EDGE('',*,*,#8894,.F.);
#12495=ORIENTED_EDGE('',*,*,#8893,.F.);
#12496=ORIENTED_EDGE('',*,*,#8892,.F.);
#12497=ORIENTED_EDGE('',*,*,#8891,.F.);
#12498=ORIENTED_EDGE('',*,*,#8890,.F.);
#12499=ORIENTED_EDGE('',*,*,#8889,.F.);
#12500=ORIENTED_EDGE('',*,*,#8888,.F.);
#12501=ORIENTED_EDGE('',*,*,#8887,.F.);
#12502=ORIENTED_EDGE('',*,*,#8886,.F.);
#12503=ORIENTED_EDGE('',*,*,#8885,.F.);
#12504=ORIENTED_EDGE('',*,*,#8884,.F.);
#12505=ORIENTED_EDGE('',*,*,#8883,.F.);
#12506=ORIENTED_EDGE('',*,*,#8882,.F.);
#12507=ORIENTED_EDGE('',*,*,#8881,.F.);
#12508=ORIENTED_EDGE('',*,*,#8921,.T.);
#12509=ORIENTED_EDGE('',*,*,#8922,.T.);
#12510=ORIENTED_EDGE('',*,*,#8919,.T.);
#12511=ORIENTED_EDGE('',*,*,#8854,.T.);
#12512=ORIENTED_EDGE('',*,*,#8920,.T.);
#12513=ORIENTED_EDGE('',*,*,#8917,.T.);
#12514=ORIENTED_EDGE('',*,*,#8922,.F.);
#12515=ORIENTED_EDGE('',*,*,#8923,.F.);
#12516=ORIENTED_EDGE('',*,*,#8921,.F.);
#12517=ORIENTED_EDGE('',*,*,#8910,.T.);
#12518=ORIENTED_EDGE('',*,*,#8924,.T.);
#12519=ORIENTED_EDGE('',*,*,#8925,.T.);
#12520=ORIENTED_EDGE('',*,*,#8924,.F.);
#12521=ORIENTED_EDGE('',*,*,#8913,.T.);
#12522=ORIENTED_EDGE('',*,*,#8880,.T.);
#12523=ORIENTED_EDGE('',*,*,#8914,.T.);
#12524=ORIENTED_EDGE('',*,*,#8925,.F.);
#12525=ORIENTED_EDGE('',*,*,#8926,.F.);
#12526=ORIENTED_EDGE('',*,*,#8927,.F.);
#12527=ORIENTED_EDGE('',*,*,#8928,.F.);
#12528=ORIENTED_EDGE('',*,*,#8929,.F.);
#12529=ORIENTED_EDGE('',*,*,#8928,.T.);
#12530=ORIENTED_EDGE('',*,*,#8930,.F.);
#12531=ORIENTED_EDGE('',*,*,#8931,.F.);
#12532=ORIENTED_EDGE('',*,*,#8932,.F.);
#12533=ORIENTED_EDGE('',*,*,#8933,.F.);
#12534=ORIENTED_EDGE('',*,*,#8930,.T.);
#12535=ORIENTED_EDGE('',*,*,#8927,.T.);
#12536=ORIENTED_EDGE('',*,*,#8934,.T.);
#12537=ORIENTED_EDGE('',*,*,#8935,.T.);
#12538=ORIENTED_EDGE('',*,*,#8936,.F.);
#12539=ORIENTED_EDGE('',*,*,#8935,.F.);
#12540=ORIENTED_EDGE('',*,*,#8937,.T.);
#12541=ORIENTED_EDGE('',*,*,#8938,.T.);
#12542=ORIENTED_EDGE('',*,*,#8939,.F.);
#12543=ORIENTED_EDGE('',*,*,#8940,.T.);
#12544=ORIENTED_EDGE('',*,*,#8941,.T.);
#12545=ORIENTED_EDGE('',*,*,#8942,.T.);
#12546=ORIENTED_EDGE('',*,*,#8943,.F.);
#12547=ORIENTED_EDGE('',*,*,#8944,.T.);
#12548=ORIENTED_EDGE('',*,*,#8945,.T.);
#12549=ORIENTED_EDGE('',*,*,#8946,.T.);
#12550=ORIENTED_EDGE('',*,*,#8947,.F.);
#12551=ORIENTED_EDGE('',*,*,#8948,.T.);
#12552=ORIENTED_EDGE('',*,*,#8949,.T.);
#12553=ORIENTED_EDGE('',*,*,#8950,.T.);
#12554=ORIENTED_EDGE('',*,*,#8951,.F.);
#12555=ORIENTED_EDGE('',*,*,#8952,.T.);
#12556=ORIENTED_EDGE('',*,*,#8953,.T.);
#12557=ORIENTED_EDGE('',*,*,#8954,.T.);
#12558=ORIENTED_EDGE('',*,*,#8955,.F.);
#12559=ORIENTED_EDGE('',*,*,#8956,.T.);
#12560=ORIENTED_EDGE('',*,*,#8957,.T.);
#12561=ORIENTED_EDGE('',*,*,#8958,.T.);
#12562=ORIENTED_EDGE('',*,*,#8959,.F.);
#12563=ORIENTED_EDGE('',*,*,#8960,.T.);
#12564=ORIENTED_EDGE('',*,*,#8961,.T.);
#12565=ORIENTED_EDGE('',*,*,#8962,.T.);
#12566=ORIENTED_EDGE('',*,*,#8963,.F.);
#12567=ORIENTED_EDGE('',*,*,#8964,.T.);
#12568=ORIENTED_EDGE('',*,*,#8965,.T.);
#12569=ORIENTED_EDGE('',*,*,#8966,.T.);
#12570=ORIENTED_EDGE('',*,*,#8967,.F.);
#12571=ORIENTED_EDGE('',*,*,#8968,.T.);
#12572=ORIENTED_EDGE('',*,*,#8969,.T.);
#12573=ORIENTED_EDGE('',*,*,#8970,.T.);
#12574=ORIENTED_EDGE('',*,*,#8971,.F.);
#12575=ORIENTED_EDGE('',*,*,#8972,.T.);
#12576=ORIENTED_EDGE('',*,*,#8973,.T.);
#12577=ORIENTED_EDGE('',*,*,#8974,.T.);
#12578=ORIENTED_EDGE('',*,*,#8975,.F.);
#12579=ORIENTED_EDGE('',*,*,#8976,.T.);
#12580=ORIENTED_EDGE('',*,*,#8977,.T.);
#12581=ORIENTED_EDGE('',*,*,#8978,.T.);
#12582=ORIENTED_EDGE('',*,*,#8979,.F.);
#12583=ORIENTED_EDGE('',*,*,#8980,.T.);
#12584=ORIENTED_EDGE('',*,*,#8981,.T.);
#12585=ORIENTED_EDGE('',*,*,#8982,.T.);
#12586=ORIENTED_EDGE('',*,*,#8983,.F.);
#12587=ORIENTED_EDGE('',*,*,#8984,.T.);
#12588=ORIENTED_EDGE('',*,*,#8985,.T.);
#12589=ORIENTED_EDGE('',*,*,#8986,.T.);
#12590=ORIENTED_EDGE('',*,*,#8987,.F.);
#12591=ORIENTED_EDGE('',*,*,#8988,.T.);
#12592=ORIENTED_EDGE('',*,*,#8989,.T.);
#12593=ORIENTED_EDGE('',*,*,#8990,.T.);
#12594=ORIENTED_EDGE('',*,*,#8991,.F.);
#12595=ORIENTED_EDGE('',*,*,#8992,.T.);
#12596=ORIENTED_EDGE('',*,*,#8993,.T.);
#12597=ORIENTED_EDGE('',*,*,#8994,.T.);
#12598=ORIENTED_EDGE('',*,*,#8995,.F.);
#12599=ORIENTED_EDGE('',*,*,#8996,.T.);
#12600=ORIENTED_EDGE('',*,*,#8997,.T.);
#12601=ORIENTED_EDGE('',*,*,#8998,.T.);
#12602=ORIENTED_EDGE('',*,*,#8999,.F.);
#12603=ORIENTED_EDGE('',*,*,#9000,.T.);
#12604=ORIENTED_EDGE('',*,*,#9001,.T.);
#12605=ORIENTED_EDGE('',*,*,#9002,.T.);
#12606=ORIENTED_EDGE('',*,*,#9003,.F.);
#12607=ORIENTED_EDGE('',*,*,#8932,.T.);
#12608=ORIENTED_EDGE('',*,*,#8926,.T.);
#12609=ORIENTED_EDGE('',*,*,#8929,.T.);
#12610=ORIENTED_EDGE('',*,*,#9004,.F.);
#12611=ORIENTED_EDGE('',*,*,#9005,.T.);
#12612=ORIENTED_EDGE('',*,*,#9006,.T.);
#12613=ORIENTED_EDGE('',*,*,#9007,.T.);
#12614=ORIENTED_EDGE('',*,*,#9008,.F.);
#12615=ORIENTED_EDGE('',*,*,#9009,.T.);
#12616=ORIENTED_EDGE('',*,*,#9010,.T.);
#12617=ORIENTED_EDGE('',*,*,#9011,.T.);
#12618=ORIENTED_EDGE('',*,*,#9012,.F.);
#12619=ORIENTED_EDGE('',*,*,#9013,.T.);
#12620=ORIENTED_EDGE('',*,*,#9014,.T.);
#12621=ORIENTED_EDGE('',*,*,#9015,.T.);
#12622=ORIENTED_EDGE('',*,*,#9016,.F.);
#12623=ORIENTED_EDGE('',*,*,#9017,.T.);
#12624=ORIENTED_EDGE('',*,*,#9018,.T.);
#12625=ORIENTED_EDGE('',*,*,#9019,.T.);
#12626=ORIENTED_EDGE('',*,*,#9020,.F.);
#12627=ORIENTED_EDGE('',*,*,#9021,.T.);
#12628=ORIENTED_EDGE('',*,*,#9022,.T.);
#12629=ORIENTED_EDGE('',*,*,#9023,.T.);
#12630=ORIENTED_EDGE('',*,*,#9024,.F.);
#12631=ORIENTED_EDGE('',*,*,#9025,.T.);
#12632=ORIENTED_EDGE('',*,*,#9026,.T.);
#12633=ORIENTED_EDGE('',*,*,#9027,.T.);
#12634=ORIENTED_EDGE('',*,*,#9028,.F.);
#12635=ORIENTED_EDGE('',*,*,#9029,.T.);
#12636=ORIENTED_EDGE('',*,*,#9030,.T.);
#12637=ORIENTED_EDGE('',*,*,#9031,.T.);
#12638=ORIENTED_EDGE('',*,*,#9032,.F.);
#12639=ORIENTED_EDGE('',*,*,#9033,.T.);
#12640=ORIENTED_EDGE('',*,*,#9034,.T.);
#12641=ORIENTED_EDGE('',*,*,#9035,.T.);
#12642=ORIENTED_EDGE('',*,*,#9036,.F.);
#12643=ORIENTED_EDGE('',*,*,#9037,.T.);
#12644=ORIENTED_EDGE('',*,*,#9038,.T.);
#12645=ORIENTED_EDGE('',*,*,#9039,.T.);
#12646=ORIENTED_EDGE('',*,*,#9040,.F.);
#12647=ORIENTED_EDGE('',*,*,#9041,.T.);
#12648=ORIENTED_EDGE('',*,*,#9042,.T.);
#12649=ORIENTED_EDGE('',*,*,#9043,.T.);
#12650=ORIENTED_EDGE('',*,*,#9044,.F.);
#12651=ORIENTED_EDGE('',*,*,#9045,.T.);
#12652=ORIENTED_EDGE('',*,*,#9046,.T.);
#12653=ORIENTED_EDGE('',*,*,#9047,.T.);
#12654=ORIENTED_EDGE('',*,*,#9048,.F.);
#12655=ORIENTED_EDGE('',*,*,#9049,.T.);
#12656=ORIENTED_EDGE('',*,*,#9050,.T.);
#12657=ORIENTED_EDGE('',*,*,#9051,.T.);
#12658=ORIENTED_EDGE('',*,*,#9052,.F.);
#12659=ORIENTED_EDGE('',*,*,#9053,.T.);
#12660=ORIENTED_EDGE('',*,*,#9054,.T.);
#12661=ORIENTED_EDGE('',*,*,#9055,.T.);
#12662=ORIENTED_EDGE('',*,*,#9056,.F.);
#12663=ORIENTED_EDGE('',*,*,#9057,.T.);
#12664=ORIENTED_EDGE('',*,*,#9058,.T.);
#12665=ORIENTED_EDGE('',*,*,#9059,.T.);
#12666=ORIENTED_EDGE('',*,*,#9060,.F.);
#12667=ORIENTED_EDGE('',*,*,#9061,.T.);
#12668=ORIENTED_EDGE('',*,*,#9062,.T.);
#12669=ORIENTED_EDGE('',*,*,#9063,.T.);
#12670=ORIENTED_EDGE('',*,*,#9064,.F.);
#12671=ORIENTED_EDGE('',*,*,#9065,.T.);
#12672=ORIENTED_EDGE('',*,*,#9066,.T.);
#12673=ORIENTED_EDGE('',*,*,#9067,.T.);
#12674=ORIENTED_EDGE('',*,*,#9068,.F.);
#12675=ORIENTED_EDGE('',*,*,#9069,.T.);
#12676=ORIENTED_EDGE('',*,*,#9070,.T.);
#12677=ORIENTED_EDGE('',*,*,#9071,.T.);
#12678=ORIENTED_EDGE('',*,*,#9072,.F.);
#12679=ORIENTED_EDGE('',*,*,#9073,.T.);
#12680=ORIENTED_EDGE('',*,*,#9074,.T.);
#12681=ORIENTED_EDGE('',*,*,#9075,.T.);
#12682=ORIENTED_EDGE('',*,*,#9076,.F.);
#12683=ORIENTED_EDGE('',*,*,#9077,.T.);
#12684=ORIENTED_EDGE('',*,*,#9002,.F.);
#12685=ORIENTED_EDGE('',*,*,#9078,.T.);
#12686=ORIENTED_EDGE('',*,*,#9079,.F.);
#12687=ORIENTED_EDGE('',*,*,#9080,.F.);
#12688=ORIENTED_EDGE('',*,*,#9081,.F.);
#12689=ORIENTED_EDGE('',*,*,#9079,.T.);
#12690=ORIENTED_EDGE('',*,*,#9082,.T.);
#12691=ORIENTED_EDGE('',*,*,#9000,.F.);
#12692=ORIENTED_EDGE('',*,*,#9001,.F.);
#12693=ORIENTED_EDGE('',*,*,#9082,.F.);
#12694=ORIENTED_EDGE('',*,*,#9078,.F.);
#12695=ORIENTED_EDGE('',*,*,#9083,.T.);
#12696=ORIENTED_EDGE('',*,*,#9076,.T.);
#12697=ORIENTED_EDGE('',*,*,#9084,.T.);
#12698=ORIENTED_EDGE('',*,*,#9085,.T.);
#12699=ORIENTED_EDGE('',*,*,#9072,.T.);
#12700=ORIENTED_EDGE('',*,*,#9086,.T.);
#12701=ORIENTED_EDGE('',*,*,#9087,.T.);
#12702=ORIENTED_EDGE('',*,*,#9068,.T.);
#12703=ORIENTED_EDGE('',*,*,#9088,.T.);
#12704=ORIENTED_EDGE('',*,*,#9089,.T.);
#12705=ORIENTED_EDGE('',*,*,#9064,.T.);
#12706=ORIENTED_EDGE('',*,*,#9090,.T.);
#12707=ORIENTED_EDGE('',*,*,#9091,.T.);
#12708=ORIENTED_EDGE('',*,*,#9060,.T.);
#12709=ORIENTED_EDGE('',*,*,#9092,.T.);
#12710=ORIENTED_EDGE('',*,*,#9093,.T.);
#12711=ORIENTED_EDGE('',*,*,#9056,.T.);
#12712=ORIENTED_EDGE('',*,*,#9094,.T.);
#12713=ORIENTED_EDGE('',*,*,#9095,.T.);
#12714=ORIENTED_EDGE('',*,*,#9052,.T.);
#12715=ORIENTED_EDGE('',*,*,#9096,.T.);
#12716=ORIENTED_EDGE('',*,*,#9097,.T.);
#12717=ORIENTED_EDGE('',*,*,#9048,.T.);
#12718=ORIENTED_EDGE('',*,*,#9098,.T.);
#12719=ORIENTED_EDGE('',*,*,#9099,.T.);
#12720=ORIENTED_EDGE('',*,*,#9044,.T.);
#12721=ORIENTED_EDGE('',*,*,#9100,.T.);
#12722=ORIENTED_EDGE('',*,*,#9101,.T.);
#12723=ORIENTED_EDGE('',*,*,#9040,.T.);
#12724=ORIENTED_EDGE('',*,*,#9102,.T.);
#12725=ORIENTED_EDGE('',*,*,#9103,.T.);
#12726=ORIENTED_EDGE('',*,*,#9036,.T.);
#12727=ORIENTED_EDGE('',*,*,#9104,.T.);
#12728=ORIENTED_EDGE('',*,*,#9105,.T.);
#12729=ORIENTED_EDGE('',*,*,#9032,.T.);
#12730=ORIENTED_EDGE('',*,*,#9106,.T.);
#12731=ORIENTED_EDGE('',*,*,#9107,.T.);
#12732=ORIENTED_EDGE('',*,*,#9028,.T.);
#12733=ORIENTED_EDGE('',*,*,#9108,.T.);
#12734=ORIENTED_EDGE('',*,*,#9109,.T.);
#12735=ORIENTED_EDGE('',*,*,#9024,.T.);
#12736=ORIENTED_EDGE('',*,*,#9110,.T.);
#12737=ORIENTED_EDGE('',*,*,#9111,.T.);
#12738=ORIENTED_EDGE('',*,*,#9020,.T.);
#12739=ORIENTED_EDGE('',*,*,#9112,.T.);
#12740=ORIENTED_EDGE('',*,*,#9113,.T.);
#12741=ORIENTED_EDGE('',*,*,#9016,.T.);
#12742=ORIENTED_EDGE('',*,*,#9114,.T.);
#12743=ORIENTED_EDGE('',*,*,#9115,.T.);
#12744=ORIENTED_EDGE('',*,*,#9012,.T.);
#12745=ORIENTED_EDGE('',*,*,#9116,.T.);
#12746=ORIENTED_EDGE('',*,*,#9117,.T.);
#12747=ORIENTED_EDGE('',*,*,#9008,.T.);
#12748=ORIENTED_EDGE('',*,*,#9118,.T.);
#12749=ORIENTED_EDGE('',*,*,#9119,.T.);
#12750=ORIENTED_EDGE('',*,*,#9004,.T.);
#12751=ORIENTED_EDGE('',*,*,#8931,.T.);
#12752=ORIENTED_EDGE('',*,*,#8933,.T.);
#12753=ORIENTED_EDGE('',*,*,#9003,.T.);
#12754=ORIENTED_EDGE('',*,*,#9080,.T.);
#12755=ORIENTED_EDGE('',*,*,#9081,.T.);
#12756=ORIENTED_EDGE('',*,*,#8999,.T.);
#12757=ORIENTED_EDGE('',*,*,#9120,.T.);
#12758=ORIENTED_EDGE('',*,*,#9121,.T.);
#12759=ORIENTED_EDGE('',*,*,#8995,.T.);
#12760=ORIENTED_EDGE('',*,*,#9122,.T.);
#12761=ORIENTED_EDGE('',*,*,#9123,.T.);
#12762=ORIENTED_EDGE('',*,*,#8991,.T.);
#12763=ORIENTED_EDGE('',*,*,#9124,.T.);
#12764=ORIENTED_EDGE('',*,*,#9125,.T.);
#12765=ORIENTED_EDGE('',*,*,#8987,.T.);
#12766=ORIENTED_EDGE('',*,*,#9126,.T.);
#12767=ORIENTED_EDGE('',*,*,#9127,.T.);
#12768=ORIENTED_EDGE('',*,*,#8983,.T.);
#12769=ORIENTED_EDGE('',*,*,#9128,.T.);
#12770=ORIENTED_EDGE('',*,*,#9129,.T.);
#12771=ORIENTED_EDGE('',*,*,#8979,.T.);
#12772=ORIENTED_EDGE('',*,*,#9130,.T.);
#12773=ORIENTED_EDGE('',*,*,#9131,.T.);
#12774=ORIENTED_EDGE('',*,*,#8975,.T.);
#12775=ORIENTED_EDGE('',*,*,#9132,.T.);
#12776=ORIENTED_EDGE('',*,*,#9133,.T.);
#12777=ORIENTED_EDGE('',*,*,#8971,.T.);
#12778=ORIENTED_EDGE('',*,*,#9134,.T.);
#12779=ORIENTED_EDGE('',*,*,#9135,.T.);
#12780=ORIENTED_EDGE('',*,*,#8967,.T.);
#12781=ORIENTED_EDGE('',*,*,#9136,.T.);
#12782=ORIENTED_EDGE('',*,*,#9137,.T.);
#12783=ORIENTED_EDGE('',*,*,#8963,.T.);
#12784=ORIENTED_EDGE('',*,*,#9138,.T.);
#12785=ORIENTED_EDGE('',*,*,#9139,.T.);
#12786=ORIENTED_EDGE('',*,*,#8959,.T.);
#12787=ORIENTED_EDGE('',*,*,#9140,.T.);
#12788=ORIENTED_EDGE('',*,*,#9141,.T.);
#12789=ORIENTED_EDGE('',*,*,#8955,.T.);
#12790=ORIENTED_EDGE('',*,*,#9142,.T.);
#12791=ORIENTED_EDGE('',*,*,#9143,.T.);
#12792=ORIENTED_EDGE('',*,*,#8951,.T.);
#12793=ORIENTED_EDGE('',*,*,#9144,.T.);
#12794=ORIENTED_EDGE('',*,*,#9145,.T.);
#12795=ORIENTED_EDGE('',*,*,#8947,.T.);
#12796=ORIENTED_EDGE('',*,*,#9146,.T.);
#12797=ORIENTED_EDGE('',*,*,#9147,.T.);
#12798=ORIENTED_EDGE('',*,*,#8943,.T.);
#12799=ORIENTED_EDGE('',*,*,#9148,.T.);
#12800=ORIENTED_EDGE('',*,*,#9149,.T.);
#12801=ORIENTED_EDGE('',*,*,#8939,.T.);
#12802=ORIENTED_EDGE('',*,*,#9150,.T.);
#12803=ORIENTED_EDGE('',*,*,#9151,.T.);
#12804=ORIENTED_EDGE('',*,*,#9152,.T.);
#12805=ORIENTED_EDGE('',*,*,#9151,.F.);
#12806=ORIENTED_EDGE('',*,*,#8997,.F.);
#12807=ORIENTED_EDGE('',*,*,#9153,.F.);
#12808=ORIENTED_EDGE('',*,*,#9154,.F.);
#12809=ORIENTED_EDGE('',*,*,#8998,.F.);
#12810=ORIENTED_EDGE('',*,*,#9154,.T.);
#12811=ORIENTED_EDGE('',*,*,#9155,.F.);
#12812=ORIENTED_EDGE('',*,*,#9120,.F.);
#12813=ORIENTED_EDGE('',*,*,#8996,.F.);
#12814=ORIENTED_EDGE('',*,*,#9121,.F.);
#12815=ORIENTED_EDGE('',*,*,#9155,.T.);
#12816=ORIENTED_EDGE('',*,*,#9153,.T.);
#12817=ORIENTED_EDGE('',*,*,#8994,.F.);
#12818=ORIENTED_EDGE('',*,*,#9156,.T.);
#12819=ORIENTED_EDGE('',*,*,#9157,.F.);
#12820=ORIENTED_EDGE('',*,*,#9122,.F.);
#12821=ORIENTED_EDGE('',*,*,#9123,.F.);
#12822=ORIENTED_EDGE('',*,*,#9157,.T.);
#12823=ORIENTED_EDGE('',*,*,#9158,.T.);
#12824=ORIENTED_EDGE('',*,*,#8992,.F.);
#12825=ORIENTED_EDGE('',*,*,#8993,.F.);
#12826=ORIENTED_EDGE('',*,*,#9158,.F.);
#12827=ORIENTED_EDGE('',*,*,#9156,.F.);
#12828=ORIENTED_EDGE('',*,*,#8989,.F.);
#12829=ORIENTED_EDGE('',*,*,#9159,.F.);
#12830=ORIENTED_EDGE('',*,*,#9160,.F.);
#12831=ORIENTED_EDGE('',*,*,#8990,.F.);
#12832=ORIENTED_EDGE('',*,*,#9160,.T.);
#12833=ORIENTED_EDGE('',*,*,#9161,.F.);
#12834=ORIENTED_EDGE('',*,*,#9124,.F.);
#12835=ORIENTED_EDGE('',*,*,#8988,.F.);
#12836=ORIENTED_EDGE('',*,*,#9125,.F.);
#12837=ORIENTED_EDGE('',*,*,#9161,.T.);
#12838=ORIENTED_EDGE('',*,*,#9159,.T.);
#12839=ORIENTED_EDGE('',*,*,#8986,.F.);
#12840=ORIENTED_EDGE('',*,*,#9162,.T.);
#12841=ORIENTED_EDGE('',*,*,#9163,.F.);
#12842=ORIENTED_EDGE('',*,*,#9126,.F.);
#12843=ORIENTED_EDGE('',*,*,#9127,.F.);
#12844=ORIENTED_EDGE('',*,*,#9163,.T.);
#12845=ORIENTED_EDGE('',*,*,#9164,.T.);
#12846=ORIENTED_EDGE('',*,*,#8984,.F.);
#12847=ORIENTED_EDGE('',*,*,#8985,.F.);
#12848=ORIENTED_EDGE('',*,*,#9164,.F.);
#12849=ORIENTED_EDGE('',*,*,#9162,.F.);
#12850=ORIENTED_EDGE('',*,*,#8981,.F.);
#12851=ORIENTED_EDGE('',*,*,#9165,.F.);
#12852=ORIENTED_EDGE('',*,*,#9166,.F.);
#12853=ORIENTED_EDGE('',*,*,#8982,.F.);
#12854=ORIENTED_EDGE('',*,*,#9166,.T.);
#12855=ORIENTED_EDGE('',*,*,#9167,.F.);
#12856=ORIENTED_EDGE('',*,*,#9128,.F.);
#12857=ORIENTED_EDGE('',*,*,#8980,.F.);
#12858=ORIENTED_EDGE('',*,*,#9129,.F.);
#12859=ORIENTED_EDGE('',*,*,#9167,.T.);
#12860=ORIENTED_EDGE('',*,*,#9165,.T.);
#12861=ORIENTED_EDGE('',*,*,#8978,.F.);
#12862=ORIENTED_EDGE('',*,*,#9168,.T.);
#12863=ORIENTED_EDGE('',*,*,#9169,.F.);
#12864=ORIENTED_EDGE('',*,*,#9130,.F.);
#12865=ORIENTED_EDGE('',*,*,#9131,.F.);
#12866=ORIENTED_EDGE('',*,*,#9169,.T.);
#12867=ORIENTED_EDGE('',*,*,#9170,.T.);
#12868=ORIENTED_EDGE('',*,*,#8976,.F.);
#12869=ORIENTED_EDGE('',*,*,#8977,.F.);
#12870=ORIENTED_EDGE('',*,*,#9170,.F.);
#12871=ORIENTED_EDGE('',*,*,#9168,.F.);
#12872=ORIENTED_EDGE('',*,*,#8973,.F.);
#12873=ORIENTED_EDGE('',*,*,#9171,.F.);
#12874=ORIENTED_EDGE('',*,*,#9172,.F.);
#12875=ORIENTED_EDGE('',*,*,#8974,.F.);
#12876=ORIENTED_EDGE('',*,*,#9172,.T.);
#12877=ORIENTED_EDGE('',*,*,#9173,.F.);
#12878=ORIENTED_EDGE('',*,*,#9132,.F.);
#12879=ORIENTED_EDGE('',*,*,#8972,.F.);
#12880=ORIENTED_EDGE('',*,*,#9133,.F.);
#12881=ORIENTED_EDGE('',*,*,#9173,.T.);
#12882=ORIENTED_EDGE('',*,*,#9171,.T.);
#12883=ORIENTED_EDGE('',*,*,#8970,.F.);
#12884=ORIENTED_EDGE('',*,*,#9174,.T.);
#12885=ORIENTED_EDGE('',*,*,#9175,.F.);
#12886=ORIENTED_EDGE('',*,*,#9134,.F.);
#12887=ORIENTED_EDGE('',*,*,#9135,.F.);
#12888=ORIENTED_EDGE('',*,*,#9175,.T.);
#12889=ORIENTED_EDGE('',*,*,#9176,.T.);
#12890=ORIENTED_EDGE('',*,*,#8968,.F.);
#12891=ORIENTED_EDGE('',*,*,#8969,.F.);
#12892=ORIENTED_EDGE('',*,*,#9176,.F.);
#12893=ORIENTED_EDGE('',*,*,#9174,.F.);
#12894=ORIENTED_EDGE('',*,*,#8965,.F.);
#12895=ORIENTED_EDGE('',*,*,#9177,.F.);
#12896=ORIENTED_EDGE('',*,*,#9178,.F.);
#12897=ORIENTED_EDGE('',*,*,#8966,.F.);
#12898=ORIENTED_EDGE('',*,*,#9178,.T.);
#12899=ORIENTED_EDGE('',*,*,#9179,.F.);
#12900=ORIENTED_EDGE('',*,*,#9136,.F.);
#12901=ORIENTED_EDGE('',*,*,#8964,.F.);
#12902=ORIENTED_EDGE('',*,*,#9137,.F.);
#12903=ORIENTED_EDGE('',*,*,#9179,.T.);
#12904=ORIENTED_EDGE('',*,*,#9177,.T.);
#12905=ORIENTED_EDGE('',*,*,#8962,.F.);
#12906=ORIENTED_EDGE('',*,*,#9180,.T.);
#12907=ORIENTED_EDGE('',*,*,#9181,.F.);
#12908=ORIENTED_EDGE('',*,*,#9138,.F.);
#12909=ORIENTED_EDGE('',*,*,#9139,.F.);
#12910=ORIENTED_EDGE('',*,*,#9181,.T.);
#12911=ORIENTED_EDGE('',*,*,#9182,.T.);
#12912=ORIENTED_EDGE('',*,*,#8960,.F.);
#12913=ORIENTED_EDGE('',*,*,#8961,.F.);
#12914=ORIENTED_EDGE('',*,*,#9182,.F.);
#12915=ORIENTED_EDGE('',*,*,#9180,.F.);
#12916=ORIENTED_EDGE('',*,*,#8957,.F.);
#12917=ORIENTED_EDGE('',*,*,#9183,.F.);
#12918=ORIENTED_EDGE('',*,*,#9184,.F.);
#12919=ORIENTED_EDGE('',*,*,#8958,.F.);
#12920=ORIENTED_EDGE('',*,*,#9184,.T.);
#12921=ORIENTED_EDGE('',*,*,#9185,.F.);
#12922=ORIENTED_EDGE('',*,*,#9140,.F.);
#12923=ORIENTED_EDGE('',*,*,#8956,.F.);
#12924=ORIENTED_EDGE('',*,*,#9141,.F.);
#12925=ORIENTED_EDGE('',*,*,#9185,.T.);
#12926=ORIENTED_EDGE('',*,*,#9183,.T.);
#12927=ORIENTED_EDGE('',*,*,#8954,.F.);
#12928=ORIENTED_EDGE('',*,*,#9186,.T.);
#12929=ORIENTED_EDGE('',*,*,#9187,.F.);
#12930=ORIENTED_EDGE('',*,*,#9142,.F.);
#12931=ORIENTED_EDGE('',*,*,#9143,.F.);
#12932=ORIENTED_EDGE('',*,*,#9187,.T.);
#12933=ORIENTED_EDGE('',*,*,#9188,.T.);
#12934=ORIENTED_EDGE('',*,*,#8952,.F.);
#12935=ORIENTED_EDGE('',*,*,#8953,.F.);
#12936=ORIENTED_EDGE('',*,*,#9188,.F.);
#12937=ORIENTED_EDGE('',*,*,#9186,.F.);
#12938=ORIENTED_EDGE('',*,*,#8949,.F.);
#12939=ORIENTED_EDGE('',*,*,#9189,.F.);
#12940=ORIENTED_EDGE('',*,*,#9190,.F.);
#12941=ORIENTED_EDGE('',*,*,#8950,.F.);
#12942=ORIENTED_EDGE('',*,*,#9190,.T.);
#12943=ORIENTED_EDGE('',*,*,#9191,.F.);
#12944=ORIENTED_EDGE('',*,*,#9144,.F.);
#12945=ORIENTED_EDGE('',*,*,#8948,.F.);
#12946=ORIENTED_EDGE('',*,*,#9145,.F.);
#12947=ORIENTED_EDGE('',*,*,#9191,.T.);
#12948=ORIENTED_EDGE('',*,*,#9189,.T.);
#12949=ORIENTED_EDGE('',*,*,#8946,.F.);
#12950=ORIENTED_EDGE('',*,*,#9192,.T.);
#12951=ORIENTED_EDGE('',*,*,#9193,.F.);
#12952=ORIENTED_EDGE('',*,*,#9146,.F.);
#12953=ORIENTED_EDGE('',*,*,#9147,.F.);
#12954=ORIENTED_EDGE('',*,*,#9193,.T.);
#12955=ORIENTED_EDGE('',*,*,#9194,.T.);
#12956=ORIENTED_EDGE('',*,*,#8944,.F.);
#12957=ORIENTED_EDGE('',*,*,#8945,.F.);
#12958=ORIENTED_EDGE('',*,*,#9194,.F.);
#12959=ORIENTED_EDGE('',*,*,#9192,.F.);
#12960=ORIENTED_EDGE('',*,*,#8941,.F.);
#12961=ORIENTED_EDGE('',*,*,#9195,.F.);
#12962=ORIENTED_EDGE('',*,*,#9196,.F.);
#12963=ORIENTED_EDGE('',*,*,#8942,.F.);
#12964=ORIENTED_EDGE('',*,*,#9196,.T.);
#12965=ORIENTED_EDGE('',*,*,#9197,.F.);
#12966=ORIENTED_EDGE('',*,*,#9148,.F.);
#12967=ORIENTED_EDGE('',*,*,#8940,.F.);
#12968=ORIENTED_EDGE('',*,*,#9149,.F.);
#12969=ORIENTED_EDGE('',*,*,#9197,.T.);
#12970=ORIENTED_EDGE('',*,*,#9195,.T.);
#12971=ORIENTED_EDGE('',*,*,#8938,.F.);
#12972=ORIENTED_EDGE('',*,*,#9198,.T.);
#12973=ORIENTED_EDGE('',*,*,#9199,.F.);
#12974=ORIENTED_EDGE('',*,*,#9150,.F.);
#12975=ORIENTED_EDGE('',*,*,#9083,.F.);
#12976=ORIENTED_EDGE('',*,*,#9199,.T.);
#12977=ORIENTED_EDGE('',*,*,#9200,.T.);
#12978=ORIENTED_EDGE('',*,*,#9077,.F.);
#12979=ORIENTED_EDGE('',*,*,#8934,.F.);
#12980=ORIENTED_EDGE('',*,*,#9200,.F.);
#12981=ORIENTED_EDGE('',*,*,#9198,.F.);
#12982=ORIENTED_EDGE('',*,*,#8937,.F.);
#12983=ORIENTED_EDGE('',*,*,#9074,.F.);
#12984=ORIENTED_EDGE('',*,*,#9201,.F.);
#12985=ORIENTED_EDGE('',*,*,#9202,.F.);
#12986=ORIENTED_EDGE('',*,*,#9075,.F.);
#12987=ORIENTED_EDGE('',*,*,#9202,.T.);
#12988=ORIENTED_EDGE('',*,*,#9203,.F.);
#12989=ORIENTED_EDGE('',*,*,#9084,.F.);
#12990=ORIENTED_EDGE('',*,*,#9073,.F.);
#12991=ORIENTED_EDGE('',*,*,#9085,.F.);
#12992=ORIENTED_EDGE('',*,*,#9203,.T.);
#12993=ORIENTED_EDGE('',*,*,#9201,.T.);
#12994=ORIENTED_EDGE('',*,*,#9071,.F.);
#12995=ORIENTED_EDGE('',*,*,#9204,.T.);
#12996=ORIENTED_EDGE('',*,*,#9205,.F.);
#12997=ORIENTED_EDGE('',*,*,#9086,.F.);
#12998=ORIENTED_EDGE('',*,*,#9087,.F.);
#12999=ORIENTED_EDGE('',*,*,#9205,.T.);
#13000=ORIENTED_EDGE('',*,*,#9206,.T.);
#13001=ORIENTED_EDGE('',*,*,#9069,.F.);
#13002=ORIENTED_EDGE('',*,*,#9070,.F.);
#13003=ORIENTED_EDGE('',*,*,#9206,.F.);
#13004=ORIENTED_EDGE('',*,*,#9204,.F.);
#13005=ORIENTED_EDGE('',*,*,#9066,.F.);
#13006=ORIENTED_EDGE('',*,*,#9207,.F.);
#13007=ORIENTED_EDGE('',*,*,#9208,.F.);
#13008=ORIENTED_EDGE('',*,*,#9067,.F.);
#13009=ORIENTED_EDGE('',*,*,#9208,.T.);
#13010=ORIENTED_EDGE('',*,*,#9209,.F.);
#13011=ORIENTED_EDGE('',*,*,#9088,.F.);
#13012=ORIENTED_EDGE('',*,*,#9065,.F.);
#13013=ORIENTED_EDGE('',*,*,#9089,.F.);
#13014=ORIENTED_EDGE('',*,*,#9209,.T.);
#13015=ORIENTED_EDGE('',*,*,#9207,.T.);
#13016=ORIENTED_EDGE('',*,*,#9063,.F.);
#13017=ORIENTED_EDGE('',*,*,#9210,.T.);
#13018=ORIENTED_EDGE('',*,*,#9211,.F.);
#13019=ORIENTED_EDGE('',*,*,#9090,.F.);
#13020=ORIENTED_EDGE('',*,*,#9091,.F.);
#13021=ORIENTED_EDGE('',*,*,#9211,.T.);
#13022=ORIENTED_EDGE('',*,*,#9212,.T.);
#13023=ORIENTED_EDGE('',*,*,#9061,.F.);
#13024=ORIENTED_EDGE('',*,*,#9062,.F.);
#13025=ORIENTED_EDGE('',*,*,#9212,.F.);
#13026=ORIENTED_EDGE('',*,*,#9210,.F.);
#13027=ORIENTED_EDGE('',*,*,#9058,.F.);
#13028=ORIENTED_EDGE('',*,*,#9213,.F.);
#13029=ORIENTED_EDGE('',*,*,#9214,.F.);
#13030=ORIENTED_EDGE('',*,*,#9059,.F.);
#13031=ORIENTED_EDGE('',*,*,#9214,.T.);
#13032=ORIENTED_EDGE('',*,*,#9215,.F.);
#13033=ORIENTED_EDGE('',*,*,#9092,.F.);
#13034=ORIENTED_EDGE('',*,*,#9057,.F.);
#13035=ORIENTED_EDGE('',*,*,#9093,.F.);
#13036=ORIENTED_EDGE('',*,*,#9215,.T.);
#13037=ORIENTED_EDGE('',*,*,#9213,.T.);
#13038=ORIENTED_EDGE('',*,*,#9055,.F.);
#13039=ORIENTED_EDGE('',*,*,#9216,.T.);
#13040=ORIENTED_EDGE('',*,*,#9217,.F.);
#13041=ORIENTED_EDGE('',*,*,#9094,.F.);
#13042=ORIENTED_EDGE('',*,*,#9095,.F.);
#13043=ORIENTED_EDGE('',*,*,#9217,.T.);
#13044=ORIENTED_EDGE('',*,*,#9218,.T.);
#13045=ORIENTED_EDGE('',*,*,#9053,.F.);
#13046=ORIENTED_EDGE('',*,*,#9054,.F.);
#13047=ORIENTED_EDGE('',*,*,#9218,.F.);
#13048=ORIENTED_EDGE('',*,*,#9216,.F.);
#13049=ORIENTED_EDGE('',*,*,#9050,.F.);
#13050=ORIENTED_EDGE('',*,*,#9219,.F.);
#13051=ORIENTED_EDGE('',*,*,#9220,.F.);
#13052=ORIENTED_EDGE('',*,*,#9051,.F.);
#13053=ORIENTED_EDGE('',*,*,#9220,.T.);
#13054=ORIENTED_EDGE('',*,*,#9221,.F.);
#13055=ORIENTED_EDGE('',*,*,#9096,.F.);
#13056=ORIENTED_EDGE('',*,*,#9049,.F.);
#13057=ORIENTED_EDGE('',*,*,#9097,.F.);
#13058=ORIENTED_EDGE('',*,*,#9221,.T.);
#13059=ORIENTED_EDGE('',*,*,#9219,.T.);
#13060=ORIENTED_EDGE('',*,*,#9047,.F.);
#13061=ORIENTED_EDGE('',*,*,#9222,.T.);
#13062=ORIENTED_EDGE('',*,*,#9223,.F.);
#13063=ORIENTED_EDGE('',*,*,#9098,.F.);
#13064=ORIENTED_EDGE('',*,*,#9099,.F.);
#13065=ORIENTED_EDGE('',*,*,#9223,.T.);
#13066=ORIENTED_EDGE('',*,*,#9224,.T.);
#13067=ORIENTED_EDGE('',*,*,#9045,.F.);
#13068=ORIENTED_EDGE('',*,*,#9046,.F.);
#13069=ORIENTED_EDGE('',*,*,#9224,.F.);
#13070=ORIENTED_EDGE('',*,*,#9222,.F.);
#13071=ORIENTED_EDGE('',*,*,#9042,.F.);
#13072=ORIENTED_EDGE('',*,*,#9225,.F.);
#13073=ORIENTED_EDGE('',*,*,#9226,.F.);
#13074=ORIENTED_EDGE('',*,*,#9043,.F.);
#13075=ORIENTED_EDGE('',*,*,#9226,.T.);
#13076=ORIENTED_EDGE('',*,*,#9227,.F.);
#13077=ORIENTED_EDGE('',*,*,#9100,.F.);
#13078=ORIENTED_EDGE('',*,*,#9041,.F.);
#13079=ORIENTED_EDGE('',*,*,#9101,.F.);
#13080=ORIENTED_EDGE('',*,*,#9227,.T.);
#13081=ORIENTED_EDGE('',*,*,#9225,.T.);
#13082=ORIENTED_EDGE('',*,*,#9039,.F.);
#13083=ORIENTED_EDGE('',*,*,#9228,.T.);
#13084=ORIENTED_EDGE('',*,*,#9229,.F.);
#13085=ORIENTED_EDGE('',*,*,#9102,.F.);
#13086=ORIENTED_EDGE('',*,*,#9103,.F.);
#13087=ORIENTED_EDGE('',*,*,#9229,.T.);
#13088=ORIENTED_EDGE('',*,*,#9230,.T.);
#13089=ORIENTED_EDGE('',*,*,#9037,.F.);
#13090=ORIENTED_EDGE('',*,*,#9038,.F.);
#13091=ORIENTED_EDGE('',*,*,#9230,.F.);
#13092=ORIENTED_EDGE('',*,*,#9228,.F.);
#13093=ORIENTED_EDGE('',*,*,#9034,.F.);
#13094=ORIENTED_EDGE('',*,*,#9231,.F.);
#13095=ORIENTED_EDGE('',*,*,#9232,.F.);
#13096=ORIENTED_EDGE('',*,*,#9035,.F.);
#13097=ORIENTED_EDGE('',*,*,#9232,.T.);
#13098=ORIENTED_EDGE('',*,*,#9233,.F.);
#13099=ORIENTED_EDGE('',*,*,#9104,.F.);
#13100=ORIENTED_EDGE('',*,*,#9033,.F.);
#13101=ORIENTED_EDGE('',*,*,#9105,.F.);
#13102=ORIENTED_EDGE('',*,*,#9233,.T.);
#13103=ORIENTED_EDGE('',*,*,#9231,.T.);
#13104=ORIENTED_EDGE('',*,*,#9031,.F.);
#13105=ORIENTED_EDGE('',*,*,#9234,.T.);
#13106=ORIENTED_EDGE('',*,*,#9235,.F.);
#13107=ORIENTED_EDGE('',*,*,#9106,.F.);
#13108=ORIENTED_EDGE('',*,*,#9107,.F.);
#13109=ORIENTED_EDGE('',*,*,#9235,.T.);
#13110=ORIENTED_EDGE('',*,*,#9236,.T.);
#13111=ORIENTED_EDGE('',*,*,#9029,.F.);
#13112=ORIENTED_EDGE('',*,*,#9030,.F.);
#13113=ORIENTED_EDGE('',*,*,#9236,.F.);
#13114=ORIENTED_EDGE('',*,*,#9234,.F.);
#13115=ORIENTED_EDGE('',*,*,#9026,.F.);
#13116=ORIENTED_EDGE('',*,*,#9237,.F.);
#13117=ORIENTED_EDGE('',*,*,#9238,.F.);
#13118=ORIENTED_EDGE('',*,*,#9027,.F.);
#13119=ORIENTED_EDGE('',*,*,#9238,.T.);
#13120=ORIENTED_EDGE('',*,*,#9239,.F.);
#13121=ORIENTED_EDGE('',*,*,#9108,.F.);
#13122=ORIENTED_EDGE('',*,*,#9025,.F.);
#13123=ORIENTED_EDGE('',*,*,#9109,.F.);
#13124=ORIENTED_EDGE('',*,*,#9239,.T.);
#13125=ORIENTED_EDGE('',*,*,#9237,.T.);
#13126=ORIENTED_EDGE('',*,*,#9023,.F.);
#13127=ORIENTED_EDGE('',*,*,#9240,.T.);
#13128=ORIENTED_EDGE('',*,*,#9241,.F.);
#13129=ORIENTED_EDGE('',*,*,#9110,.F.);
#13130=ORIENTED_EDGE('',*,*,#9111,.F.);
#13131=ORIENTED_EDGE('',*,*,#9241,.T.);
#13132=ORIENTED_EDGE('',*,*,#9242,.T.);
#13133=ORIENTED_EDGE('',*,*,#9021,.F.);
#13134=ORIENTED_EDGE('',*,*,#9022,.F.);
#13135=ORIENTED_EDGE('',*,*,#9242,.F.);
#13136=ORIENTED_EDGE('',*,*,#9240,.F.);
#13137=ORIENTED_EDGE('',*,*,#9018,.F.);
#13138=ORIENTED_EDGE('',*,*,#9243,.F.);
#13139=ORIENTED_EDGE('',*,*,#9244,.F.);
#13140=ORIENTED_EDGE('',*,*,#9019,.F.);
#13141=ORIENTED_EDGE('',*,*,#9244,.T.);
#13142=ORIENTED_EDGE('',*,*,#9245,.F.);
#13143=ORIENTED_EDGE('',*,*,#9112,.F.);
#13144=ORIENTED_EDGE('',*,*,#9017,.F.);
#13145=ORIENTED_EDGE('',*,*,#9113,.F.);
#13146=ORIENTED_EDGE('',*,*,#9245,.T.);
#13147=ORIENTED_EDGE('',*,*,#9243,.T.);
#13148=ORIENTED_EDGE('',*,*,#9015,.F.);
#13149=ORIENTED_EDGE('',*,*,#9246,.T.);
#13150=ORIENTED_EDGE('',*,*,#9247,.F.);
#13151=ORIENTED_EDGE('',*,*,#9114,.F.);
#13152=ORIENTED_EDGE('',*,*,#9115,.F.);
#13153=ORIENTED_EDGE('',*,*,#9247,.T.);
#13154=ORIENTED_EDGE('',*,*,#9248,.T.);
#13155=ORIENTED_EDGE('',*,*,#9013,.F.);
#13156=ORIENTED_EDGE('',*,*,#9014,.F.);
#13157=ORIENTED_EDGE('',*,*,#9248,.F.);
#13158=ORIENTED_EDGE('',*,*,#9246,.F.);
#13159=ORIENTED_EDGE('',*,*,#9010,.F.);
#13160=ORIENTED_EDGE('',*,*,#9249,.F.);
#13161=ORIENTED_EDGE('',*,*,#9250,.F.);
#13162=ORIENTED_EDGE('',*,*,#9011,.F.);
#13163=ORIENTED_EDGE('',*,*,#9250,.T.);
#13164=ORIENTED_EDGE('',*,*,#9251,.F.);
#13165=ORIENTED_EDGE('',*,*,#9116,.F.);
#13166=ORIENTED_EDGE('',*,*,#9009,.F.);
#13167=ORIENTED_EDGE('',*,*,#9117,.F.);
#13168=ORIENTED_EDGE('',*,*,#9251,.T.);
#13169=ORIENTED_EDGE('',*,*,#9249,.T.);
#13170=ORIENTED_EDGE('',*,*,#9007,.F.);
#13171=ORIENTED_EDGE('',*,*,#9252,.T.);
#13172=ORIENTED_EDGE('',*,*,#9253,.F.);
#13173=ORIENTED_EDGE('',*,*,#9118,.F.);
#13174=ORIENTED_EDGE('',*,*,#9119,.F.);
#13175=ORIENTED_EDGE('',*,*,#9253,.T.);
#13176=ORIENTED_EDGE('',*,*,#9254,.T.);
#13177=ORIENTED_EDGE('',*,*,#9005,.F.);
#13178=ORIENTED_EDGE('',*,*,#9006,.F.);
#13179=ORIENTED_EDGE('',*,*,#9254,.F.);
#13180=ORIENTED_EDGE('',*,*,#9252,.F.);
#13181=ORIENTED_EDGE('',*,*,#8923,.T.);
#13182=ORIENTED_EDGE('',*,*,#9255,.T.);
#13183=ORIENTED_EDGE('',*,*,#8936,.T.);
#13184=ORIENTED_EDGE('',*,*,#9255,.F.);
#13185=ORIENTED_EDGE('',*,*,#9152,.F.);
#13186=ORIENTED_EDGE('',*,*,#9256,.T.);
#13187=ORIENTED_EDGE('',*,*,#9257,.F.);
#13188=ORIENTED_EDGE('',*,*,#9258,.T.);
#13189=ORIENTED_EDGE('',*,*,#9259,.F.);
#13190=ORIENTED_EDGE('',*,*,#9260,.F.);
#13191=ORIENTED_EDGE('',*,*,#9261,.T.);
#13192=ORIENTED_EDGE('',*,*,#9262,.F.);
#13193=ORIENTED_EDGE('',*,*,#9263,.F.);
#13194=ORIENTED_EDGE('',*,*,#9264,.T.);
#13195=ORIENTED_EDGE('',*,*,#9265,.F.);
#13196=ORIENTED_EDGE('',*,*,#9266,.F.);
#13197=ORIENTED_EDGE('',*,*,#9267,.T.);
#13198=ORIENTED_EDGE('',*,*,#9268,.F.);
#13199=ORIENTED_EDGE('',*,*,#9269,.F.);
#13200=ORIENTED_EDGE('',*,*,#9270,.T.);
#13201=ORIENTED_EDGE('',*,*,#9271,.F.);
#13202=ORIENTED_EDGE('',*,*,#9272,.F.);
#13203=ORIENTED_EDGE('',*,*,#9273,.T.);
#13204=ORIENTED_EDGE('',*,*,#9274,.F.);
#13205=ORIENTED_EDGE('',*,*,#9275,.T.);
#13206=ORIENTED_EDGE('',*,*,#9256,.F.);
#13207=ORIENTED_EDGE('',*,*,#9275,.F.);
#13208=ORIENTED_EDGE('',*,*,#9276,.F.);
#13209=ORIENTED_EDGE('',*,*,#9264,.F.);
#13210=ORIENTED_EDGE('',*,*,#9277,.F.);
#13211=ORIENTED_EDGE('',*,*,#9278,.F.);
#13212=ORIENTED_EDGE('',*,*,#9279,.F.);
#13213=ORIENTED_EDGE('',*,*,#9267,.F.);
#13214=ORIENTED_EDGE('',*,*,#9280,.F.);
#13215=ORIENTED_EDGE('',*,*,#9281,.F.);
#13216=ORIENTED_EDGE('',*,*,#9282,.F.);
#13217=ORIENTED_EDGE('',*,*,#9283,.F.);
#13218=ORIENTED_EDGE('',*,*,#9284,.F.);
#13219=ORIENTED_EDGE('',*,*,#9261,.F.);
#13220=ORIENTED_EDGE('',*,*,#9285,.F.);
#13221=ORIENTED_EDGE('',*,*,#9270,.F.);
#13222=ORIENTED_EDGE('',*,*,#9286,.F.);
#13223=ORIENTED_EDGE('',*,*,#9287,.F.);
#13224=ORIENTED_EDGE('',*,*,#9288,.F.);
#13225=ORIENTED_EDGE('',*,*,#9289,.F.);
#13226=ORIENTED_EDGE('',*,*,#9290,.F.);
#13227=ORIENTED_EDGE('',*,*,#9258,.F.);
#13228=ORIENTED_EDGE('',*,*,#9291,.F.);
#13229=ORIENTED_EDGE('',*,*,#9292,.F.);
#13230=ORIENTED_EDGE('',*,*,#9293,.F.);
#13231=ORIENTED_EDGE('',*,*,#9273,.F.);
#13232=ORIENTED_EDGE('',*,*,#9271,.T.);
#13233=ORIENTED_EDGE('',*,*,#9285,.T.);
#13234=ORIENTED_EDGE('',*,*,#9294,.F.);
#13235=ORIENTED_EDGE('',*,*,#9286,.T.);
#13236=ORIENTED_EDGE('',*,*,#9269,.T.);
#13237=ORIENTED_EDGE('',*,*,#9295,.T.);
#13238=ORIENTED_EDGE('',*,*,#9296,.T.);
#13239=ORIENTED_EDGE('',*,*,#9297,.F.);
#13240=ORIENTED_EDGE('',*,*,#9268,.T.);
#13241=ORIENTED_EDGE('',*,*,#9279,.T.);
#13242=ORIENTED_EDGE('',*,*,#9298,.F.);
#13243=ORIENTED_EDGE('',*,*,#9280,.T.);
#13244=ORIENTED_EDGE('',*,*,#9266,.T.);
#13245=ORIENTED_EDGE('',*,*,#9299,.T.);
#13246=ORIENTED_EDGE('',*,*,#9300,.T.);
#13247=ORIENTED_EDGE('',*,*,#9295,.F.);
#13248=ORIENTED_EDGE('',*,*,#9265,.T.);
#13249=ORIENTED_EDGE('',*,*,#9276,.T.);
#13250=ORIENTED_EDGE('',*,*,#9301,.F.);
#13251=ORIENTED_EDGE('',*,*,#9277,.T.);
#13252=ORIENTED_EDGE('',*,*,#9263,.T.);
#13253=ORIENTED_EDGE('',*,*,#9302,.T.);
#13254=ORIENTED_EDGE('',*,*,#9303,.T.);
#13255=ORIENTED_EDGE('',*,*,#9299,.F.);
#13256=ORIENTED_EDGE('',*,*,#9278,.T.);
#13257=ORIENTED_EDGE('',*,*,#9301,.T.);
#13258=ORIENTED_EDGE('',*,*,#9281,.T.);
#13259=ORIENTED_EDGE('',*,*,#9298,.T.);
#13260=ORIENTED_EDGE('',*,*,#9283,.T.);
#13261=ORIENTED_EDGE('',*,*,#9304,.T.);
#13262=ORIENTED_EDGE('',*,*,#9287,.T.);
#13263=ORIENTED_EDGE('',*,*,#9294,.T.);
#13264=ORIENTED_EDGE('',*,*,#9289,.T.);
#13265=ORIENTED_EDGE('',*,*,#9305,.T.);
#13266=ORIENTED_EDGE('',*,*,#9292,.T.);
#13267=ORIENTED_EDGE('',*,*,#9306,.T.);
#13268=ORIENTED_EDGE('',*,*,#9307,.F.);
#13269=ORIENTED_EDGE('',*,*,#9308,.T.);
#13270=ORIENTED_EDGE('',*,*,#9303,.F.);
#13271=ORIENTED_EDGE('',*,*,#9309,.T.);
#13272=ORIENTED_EDGE('',*,*,#9300,.F.);
#13273=ORIENTED_EDGE('',*,*,#9310,.T.);
#13274=ORIENTED_EDGE('',*,*,#9296,.F.);
#13275=ORIENTED_EDGE('',*,*,#9311,.T.);
#13276=ORIENTED_EDGE('',*,*,#9312,.F.);
#13277=ORIENTED_EDGE('',*,*,#9313,.T.);
#13278=ORIENTED_EDGE('',*,*,#9314,.F.);
#13279=ORIENTED_EDGE('',*,*,#9315,.T.);
#13280=ORIENTED_EDGE('',*,*,#9316,.T.);
#13281=ORIENTED_EDGE('',*,*,#9313,.F.);
#13282=ORIENTED_EDGE('',*,*,#9311,.F.);
#13283=ORIENTED_EDGE('',*,*,#9310,.F.);
#13284=ORIENTED_EDGE('',*,*,#9309,.F.);
#13285=ORIENTED_EDGE('',*,*,#9308,.F.);
#13286=ORIENTED_EDGE('',*,*,#9315,.F.);
#13287=ORIENTED_EDGE('',*,*,#9316,.F.);
#13288=ORIENTED_EDGE('',*,*,#9260,.T.);
#13289=ORIENTED_EDGE('',*,*,#9317,.T.);
#13290=ORIENTED_EDGE('',*,*,#9307,.T.);
#13291=ORIENTED_EDGE('',*,*,#9302,.F.);
#13292=ORIENTED_EDGE('',*,*,#9262,.T.);
#13293=ORIENTED_EDGE('',*,*,#9284,.T.);
#13294=ORIENTED_EDGE('',*,*,#9304,.F.);
#13295=ORIENTED_EDGE('',*,*,#9282,.T.);
#13296=ORIENTED_EDGE('',*,*,#9257,.T.);
#13297=ORIENTED_EDGE('',*,*,#9318,.T.);
#13298=ORIENTED_EDGE('',*,*,#9314,.T.);
#13299=ORIENTED_EDGE('',*,*,#9317,.F.);
#13300=ORIENTED_EDGE('',*,*,#9259,.T.);
#13301=ORIENTED_EDGE('',*,*,#9290,.T.);
#13302=ORIENTED_EDGE('',*,*,#9305,.F.);
#13303=ORIENTED_EDGE('',*,*,#9288,.T.);
#13304=ORIENTED_EDGE('',*,*,#9272,.T.);
#13305=ORIENTED_EDGE('',*,*,#9297,.T.);
#13306=ORIENTED_EDGE('',*,*,#9312,.T.);
#13307=ORIENTED_EDGE('',*,*,#9318,.F.);
#13308=ORIENTED_EDGE('',*,*,#9274,.T.);
#13309=ORIENTED_EDGE('',*,*,#9293,.T.);
#13310=ORIENTED_EDGE('',*,*,#9306,.F.);
#13311=ORIENTED_EDGE('',*,*,#9291,.T.);
#14327=CONICAL_SURFACE('',#16127,2.2005,0.785398163397448);
#14328=CONICAL_SURFACE('',#16211,4.05,0.785398163397448);
#14329=CONICAL_SURFACE('',#16319,2.40940107675851,0.785398163397453);
#14330=CONICAL_SURFACE('',#16359,2.30940107675851,1.02974425867666);
#14789=ADVANCED_FACE('',(#2054),#991,.T.);
#14790=ADVANCED_FACE('',(#2055),#992,.T.);
#14791=ADVANCED_FACE('',(#2056),#993,.T.);
#14792=ADVANCED_FACE('',(#2057),#994,.T.);
#14793=ADVANCED_FACE('',(#2058),#995,.T.);
#14794=ADVANCED_FACE('',(#2059),#996,.T.);
#14795=ADVANCED_FACE('',(#2060),#997,.T.);
#14796=ADVANCED_FACE('',(#2061),#998,.T.);
#14797=ADVANCED_FACE('',(#2062),#999,.T.);
#14798=ADVANCED_FACE('',(#2063),#1000,.T.);
#14799=ADVANCED_FACE('',(#2064),#1001,.T.);
#14800=ADVANCED_FACE('',(#2065),#1002,.T.);
#14801=ADVANCED_FACE('',(#2066),#1003,.T.);
#14802=ADVANCED_FACE('',(#2067),#1004,.T.);
#14803=ADVANCED_FACE('',(#2068),#1005,.T.);
#14804=ADVANCED_FACE('',(#2069),#1006,.T.);
#14805=ADVANCED_FACE('',(#2070),#1007,.T.);
#14806=ADVANCED_FACE('',(#2071),#1008,.T.);
#14807=ADVANCED_FACE('',(#2072),#1009,.T.);
#14808=ADVANCED_FACE('',(#2073),#1010,.T.);
#14809=ADVANCED_FACE('',(#2074),#1011,.T.);
#14810=ADVANCED_FACE('',(#2075),#1012,.T.);
#14811=ADVANCED_FACE('',(#2076),#1013,.T.);
#14812=ADVANCED_FACE('',(#2077),#1014,.T.);
#14813=ADVANCED_FACE('',(#2078),#1015,.T.);
#14814=ADVANCED_FACE('',(#2079),#1016,.T.);
#14815=ADVANCED_FACE('',(#2080),#1430,.F.);
#14816=ADVANCED_FACE('',(#2081),#364,.F.);
#14817=ADVANCED_FACE('',(#2082),#1431,.T.);
#14818=ADVANCED_FACE('',(#2083),#365,.F.);
#14819=ADVANCED_FACE('',(#2084),#360,.F.);
#14820=ADVANCED_FACE('',(#2085,#1206),#1432,.T.);
#14821=ADVANCED_FACE('',(#2086),#14327,.T.);
#14822=ADVANCED_FACE('',(#2087),#1433,.T.);
#14823=ADVANCED_FACE('',(#2088),#1434,.F.);
#14824=ADVANCED_FACE('',(#2089),#1435,.F.);
#14825=ADVANCED_FACE('',(#2090),#1436,.F.);
#14826=ADVANCED_FACE('',(#2091),#1017,.T.);
#14827=ADVANCED_FACE('',(#2092),#1437,.F.);
#14828=ADVANCED_FACE('',(#2093),#1438,.F.);
#14829=ADVANCED_FACE('',(#2094),#1439,.F.);
#14830=ADVANCED_FACE('',(#2095),#14328,.T.);
#14831=ADVANCED_FACE('',(#2096),#1440,.F.);
#14832=ADVANCED_FACE('',(#2097),#1441,.F.);
#14833=ADVANCED_FACE('',(#2098),#1442,.F.);
#14834=ADVANCED_FACE('',(#2099),#1443,.F.);
#14835=ADVANCED_FACE('',(#2100),#1444,.F.);
#14836=ADVANCED_FACE('',(#2101),#1445,.F.);
#14837=ADVANCED_FACE('',(#2102),#1446,.F.);
#14838=ADVANCED_FACE('',(#2103),#1447,.F.);
#14839=ADVANCED_FACE('',(#2104),#1448,.F.);
#14840=ADVANCED_FACE('',(#2105),#1449,.F.);
#14841=ADVANCED_FACE('',(#2106),#1450,.F.);
#14842=ADVANCED_FACE('',(#2107),#1451,.F.);
#14843=ADVANCED_FACE('',(#2108),#1452,.F.);
#14844=ADVANCED_FACE('',(#2109),#1453,.F.);
#14845=ADVANCED_FACE('',(#2110),#1454,.F.);
#14846=ADVANCED_FACE('',(#2111),#1455,.F.);
#14847=ADVANCED_FACE('',(#2112),#1456,.F.);
#14848=ADVANCED_FACE('',(#2113),#1457,.F.);
#14849=ADVANCED_FACE('',(#2114),#1458,.F.);
#14850=ADVANCED_FACE('',(#2115),#1459,.F.);
#14851=ADVANCED_FACE('',(#2116),#1460,.F.);
#14852=ADVANCED_FACE('',(#2117),#1461,.F.);
#14853=ADVANCED_FACE('',(#2118),#1462,.F.);
#14854=ADVANCED_FACE('',(#2119),#1463,.F.);
#14855=ADVANCED_FACE('',(#2120),#1464,.F.);
#14856=ADVANCED_FACE('',(#2121),#1465,.F.);
#14857=ADVANCED_FACE('',(#2122),#1466,.F.);
#14858=ADVANCED_FACE('',(#2123),#1467,.F.);
#14859=ADVANCED_FACE('',(#2124),#1468,.F.);
#14860=ADVANCED_FACE('',(#2125),#1469,.F.);
#14861=ADVANCED_FACE('',(#2126),#1470,.F.);
#14862=ADVANCED_FACE('',(#2127),#1471,.F.);
#14863=ADVANCED_FACE('',(#2128),#1472,.F.);
#14864=ADVANCED_FACE('',(#2129),#1473,.F.);
#14865=ADVANCED_FACE('',(#2130),#1474,.F.);
#14866=ADVANCED_FACE('',(#2131),#1475,.F.);
#14867=ADVANCED_FACE('',(#2132),#1476,.F.);
#14868=ADVANCED_FACE('',(#2133),#1477,.F.);
#14869=ADVANCED_FACE('',(#2134),#1478,.F.);
#14870=ADVANCED_FACE('',(#2135),#1479,.F.);
#14871=ADVANCED_FACE('',(#2136),#1480,.F.);
#14872=ADVANCED_FACE('',(#2137),#1481,.F.);
#14873=ADVANCED_FACE('',(#2138),#1482,.F.);
#14874=ADVANCED_FACE('',(#2139),#1483,.F.);
#14875=ADVANCED_FACE('',(#2140),#1484,.F.);
#14876=ADVANCED_FACE('',(#2141),#1485,.F.);
#14877=ADVANCED_FACE('',(#2142),#1486,.F.);
#14878=ADVANCED_FACE('',(#2143),#1487,.F.);
#14879=ADVANCED_FACE('',(#2144),#1488,.F.);
#14880=ADVANCED_FACE('',(#2145),#1489,.F.);
#14881=ADVANCED_FACE('',(#2146),#1490,.F.);
#14882=ADVANCED_FACE('',(#2147),#1491,.F.);
#14883=ADVANCED_FACE('',(#2148),#1492,.F.);
#14884=ADVANCED_FACE('',(#2149),#1493,.F.);
#14885=ADVANCED_FACE('',(#2150),#1494,.F.);
#14886=ADVANCED_FACE('',(#2151),#1495,.F.);
#14887=ADVANCED_FACE('',(#2152),#1496,.F.);
#14888=ADVANCED_FACE('',(#2153),#1497,.F.);
#14889=ADVANCED_FACE('',(#2154),#1498,.F.);
#14890=ADVANCED_FACE('',(#2155),#1499,.F.);
#14891=ADVANCED_FACE('',(#2156),#1500,.F.);
#14892=ADVANCED_FACE('',(#2157),#1501,.F.);
#14893=ADVANCED_FACE('',(#2158),#1502,.F.);
#14894=ADVANCED_FACE('',(#2159),#1503,.F.);
#14895=ADVANCED_FACE('',(#2160),#1504,.F.);
#14896=ADVANCED_FACE('',(#2161),#1505,.F.);
#14897=ADVANCED_FACE('',(#2162),#1506,.F.);
#14898=ADVANCED_FACE('',(#2163),#1507,.F.);
#14899=ADVANCED_FACE('',(#2164),#1508,.F.);
#14900=ADVANCED_FACE('',(#2165),#1509,.F.);
#14901=ADVANCED_FACE('',(#2166),#1510,.F.);
#14902=ADVANCED_FACE('',(#2167),#1511,.F.);
#14903=ADVANCED_FACE('',(#2168),#1512,.F.);
#14904=ADVANCED_FACE('',(#2169),#1513,.F.);
#14905=ADVANCED_FACE('',(#2170),#1514,.F.);
#14906=ADVANCED_FACE('',(#2171),#1515,.F.);
#14907=ADVANCED_FACE('',(#2172),#1516,.F.);
#14908=ADVANCED_FACE('',(#2173),#1517,.F.);
#14909=ADVANCED_FACE('',(#2174),#1518,.F.);
#14910=ADVANCED_FACE('',(#2175),#1519,.F.);
#14911=ADVANCED_FACE('',(#2176),#1520,.F.);
#14912=ADVANCED_FACE('',(#2177),#1521,.F.);
#14913=ADVANCED_FACE('',(#2178),#1522,.F.);
#14914=ADVANCED_FACE('',(#2179),#1523,.F.);
#14915=ADVANCED_FACE('',(#2180),#1524,.F.);
#14916=ADVANCED_FACE('',(#2181),#1525,.F.);
#14917=ADVANCED_FACE('',(#2182),#1526,.F.);
#14918=ADVANCED_FACE('',(#2183),#1527,.F.);
#14919=ADVANCED_FACE('',(#2184),#1528,.F.);
#14920=ADVANCED_FACE('',(#2185),#1529,.F.);
#14921=ADVANCED_FACE('',(#2186),#1530,.F.);
#14922=ADVANCED_FACE('',(#2187),#1531,.F.);
#14923=ADVANCED_FACE('',(#2188),#1532,.F.);
#14924=ADVANCED_FACE('',(#2189),#1533,.F.);
#14925=ADVANCED_FACE('',(#2190),#1534,.F.);
#14926=ADVANCED_FACE('',(#2191),#1535,.F.);
#14927=ADVANCED_FACE('',(#2192),#1536,.F.);
#14928=ADVANCED_FACE('',(#2193),#1537,.F.);
#14929=ADVANCED_FACE('',(#2194),#1538,.F.);
#14930=ADVANCED_FACE('',(#2195),#1539,.F.);
#14931=ADVANCED_FACE('',(#2196),#1540,.F.);
#14932=ADVANCED_FACE('',(#2197),#1541,.F.);
#14933=ADVANCED_FACE('',(#2198),#361,.T.);
#14934=ADVANCED_FACE('',(#2199,#1207),#1542,.F.);
#14935=ADVANCED_FACE('',(#2200),#14329,.F.);
#14936=ADVANCED_FACE('',(#2201),#1018,.T.);
#14937=ADVANCED_FACE('',(#2202),#1019,.T.);
#14938=ADVANCED_FACE('',(#2203),#1020,.T.);
#14939=ADVANCED_FACE('',(#2204),#1021,.T.);
#14940=ADVANCED_FACE('',(#2205),#1022,.T.);
#14941=ADVANCED_FACE('',(#2206),#1023,.T.);
#14942=ADVANCED_FACE('',(#2207),#1543,.F.);
#14943=ADVANCED_FACE('',(#2208),#1544,.F.);
#14944=ADVANCED_FACE('',(#2209),#1545,.F.);
#14945=ADVANCED_FACE('',(#2210),#1546,.F.);
#14946=ADVANCED_FACE('',(#2211),#1547,.F.);
#14947=ADVANCED_FACE('',(#2212),#1548,.F.);
#14948=ADVANCED_FACE('',(#2213),#1549,.F.);
#14949=ADVANCED_FACE('',(#2214),#1550,.F.);
#14950=ADVANCED_FACE('',(#2215),#1551,.F.);
#14951=ADVANCED_FACE('',(#2216),#1552,.F.);
#14952=ADVANCED_FACE('',(#2217),#1553,.F.);
#14953=ADVANCED_FACE('',(#2218),#1554,.F.);
#14954=ADVANCED_FACE('',(#2219),#1555,.F.);
#14955=ADVANCED_FACE('',(#2220),#1556,.F.);
#14956=ADVANCED_FACE('',(#2221),#1557,.F.);
#14957=ADVANCED_FACE('',(#2222),#14330,.F.);
#14958=ADVANCED_FACE('',(#2223),#1558,.F.);
#14959=ADVANCED_FACE('',(#2224),#1559,.F.);
#14960=ADVANCED_FACE('',(#2225),#1560,.F.);
#15090=CLOSED_SHELL('',(#14789,#14790,#14791,#14792,#14793,#14794,#14795,
#14796,#14797,#14798,#14799,#14800,#14801,#14802,#14803,#14804,#14805,#14806,
#14807,#14808,#14809,#14810,#14811,#14812,#14813,#14814,#14815,#14816,#14817,
#14818,#14819,#14820,#14821,#14822,#14823,#14824,#14825,#14826,#14827,#14828,
#14829,#14830,#14831,#14832,#14833,#14834,#14835,#14836,#14837,#14838,#14839,
#14840,#14841,#14842,#14843,#14844,#14845,#14846,#14847,#14848,#14849,#14850,
#14851,#14852,#14853,#14854,#14855,#14856,#14857,#14858,#14859,#14860,#14861,
#14862,#14863,#14864,#14865,#14866,#14867,#14868,#14869,#14870,#14871,#14872,
#14873,#14874,#14875,#14876,#14877,#14878,#14879,#14880,#14881,#14882,#14883,
#14884,#14885,#14886,#14887,#14888,#14889,#14890,#14891,#14892,#14893,#14894,
#14895,#14896,#14897,#14898,#14899,#14900,#14901,#14902,#14903,#14904,#14905,
#14906,#14907,#14908,#14909,#14910,#14911,#14912,#14913,#14914,#14915,#14916,
#14917,#14918,#14919,#14920,#14921,#14922,#14923,#14924,#14925,#14926,#14927,
#14928,#14929,#14930,#14931,#14932,#14933,#14934,#14935,#14936,#14937,#14938,
#14939,#14940,#14941,#14942,#14943,#14944,#14945,#14946,#14947,#14948,#14949,
#14950,#14951,#14952,#14953,#14954,#14955,#14956,#14957,#14958,#14959,#14960));
#16085=AXIS2_PLACEMENT_3D('',#23034,#19149,#19150);
#16086=AXIS2_PLACEMENT_3D('',#23035,#19151,#19152);
#16087=AXIS2_PLACEMENT_3D('',#23199,#19154,#19155);
#16088=AXIS2_PLACEMENT_3D('',#23276,#19156,#19157);
#16089=AXIS2_PLACEMENT_3D('',#23715,#19159,#19160);
#16090=AXIS2_PLACEMENT_3D('',#24152,#19162,#19163);
#16091=AXIS2_PLACEMENT_3D('',#24593,#19165,#19166);
#16092=AXIS2_PLACEMENT_3D('',#25076,#19168,#19169);
#16093=AXIS2_PLACEMENT_3D('',#25507,#19171,#19172);
#16094=AXIS2_PLACEMENT_3D('',#25795,#19174,#19175);
#16095=AXIS2_PLACEMENT_3D('',#26263,#19177,#19178);
#16096=AXIS2_PLACEMENT_3D('',#26697,#19180,#19181);
#16097=AXIS2_PLACEMENT_3D('',#26869,#19183,#19184);
#16098=AXIS2_PLACEMENT_3D('',#27191,#19186,#19187);
#16099=AXIS2_PLACEMENT_3D('',#27644,#19189,#19190);
#16100=AXIS2_PLACEMENT_3D('',#28093,#19192,#19193);
#16101=AXIS2_PLACEMENT_3D('',#28528,#19195,#19196);
#16102=AXIS2_PLACEMENT_3D('',#28987,#19198,#19199);
#16103=AXIS2_PLACEMENT_3D('',#29432,#19201,#19202);
#16104=AXIS2_PLACEMENT_3D('',#29911,#19204,#19205);
#16105=AXIS2_PLACEMENT_3D('',#30396,#19207,#19208);
#16106=AXIS2_PLACEMENT_3D('',#30843,#19210,#19211);
#16107=AXIS2_PLACEMENT_3D('',#31290,#19213,#19214);
#16108=AXIS2_PLACEMENT_3D('',#31723,#19216,#19217);
#16109=AXIS2_PLACEMENT_3D('',#32240,#19219,#19220);
#16110=AXIS2_PLACEMENT_3D('',#32691,#19222,#19223);
#16111=AXIS2_PLACEMENT_3D('',#32975,#19225,#19226);
#16112=AXIS2_PLACEMENT_3D('',#32985,#19227,#19228);
#16113=AXIS2_PLACEMENT_3D('',#36520,#19229,#19230);
#16114=AXIS2_PLACEMENT_3D('',#40407,#19231,#19232);
#16115=AXIS2_PLACEMENT_3D('',#40507,#19233,#19234);
#16116=AXIS2_PLACEMENT_3D('',#40613,#19235,#19236);
#16117=AXIS2_PLACEMENT_3D('',#40616,#19237,#19238);
#16118=AXIS2_PLACEMENT_3D('',#40790,#19239,#19240);
#16119=AXIS2_PLACEMENT_3D('',#41513,#19241,#19242);
#16120=AXIS2_PLACEMENT_3D('',#41516,#19243,#19244);
#16121=AXIS2_PLACEMENT_3D('',#41605,#19245,#19246);
#16122=AXIS2_PLACEMENT_3D('',#42238,#19247,#19248);
#16123=AXIS2_PLACEMENT_3D('',#42240,#19249,#19250);
#16124=AXIS2_PLACEMENT_3D('',#42241,#19251,#19252);
#16125=AXIS2_PLACEMENT_3D('',#42242,#19253,#19254);
#16126=AXIS2_PLACEMENT_3D('',#42244,#19255,#19256);
#16127=AXIS2_PLACEMENT_3D('',#42245,#19257,#19258);
#16128=AXIS2_PLACEMENT_3D('',#42248,#19260,#19261);
#16129=AXIS2_PLACEMENT_3D('',#42249,#19262,#19263);
#16130=AXIS2_PLACEMENT_3D('',#42250,#19264,#19265);
#16131=AXIS2_PLACEMENT_3D('',#42253,#19266,#19267);
#16132=AXIS2_PLACEMENT_3D('',#42257,#19270,#19271);
#16133=AXIS2_PLACEMENT_3D('',#42265,#19274,#19275);
#16134=AXIS2_PLACEMENT_3D('',#42271,#19277,#19278);
#16135=AXIS2_PLACEMENT_3D('',#42274,#19279,#19280);
#16136=AXIS2_PLACEMENT_3D('',#42277,#19282,#19283);
#16137=AXIS2_PLACEMENT_3D('',#42279,#19284,#19285);
#16138=AXIS2_PLACEMENT_3D('',#42283,#19287,#19288);
#16139=AXIS2_PLACEMENT_3D('',#42287,#19290,#19291);
#16140=AXIS2_PLACEMENT_3D('',#42291,#19293,#19294);
#16141=AXIS2_PLACEMENT_3D('',#42295,#19296,#19297);
#16142=AXIS2_PLACEMENT_3D('',#42299,#19299,#19300);
#16143=AXIS2_PLACEMENT_3D('',#42303,#19302,#19303);
#16144=AXIS2_PLACEMENT_3D('',#42307,#19305,#19306);
#16145=AXIS2_PLACEMENT_3D('',#42311,#19308,#19309);
#16146=AXIS2_PLACEMENT_3D('',#42315,#19311,#19312);
#16147=AXIS2_PLACEMENT_3D('',#42319,#19314,#19315);
#16148=AXIS2_PLACEMENT_3D('',#42323,#19317,#19318);
#16149=AXIS2_PLACEMENT_3D('',#42327,#19320,#19321);
#16150=AXIS2_PLACEMENT_3D('',#42331,#19323,#19324);
#16151=AXIS2_PLACEMENT_3D('',#42335,#19326,#19327);
#16152=AXIS2_PLACEMENT_3D('',#42339,#19329,#19330);
#16153=AXIS2_PLACEMENT_3D('',#42343,#19332,#19333);
#16154=AXIS2_PLACEMENT_3D('',#42347,#19335,#19336);
#16155=AXIS2_PLACEMENT_3D('',#42351,#19338,#19339);
#16156=AXIS2_PLACEMENT_3D('',#42355,#19341,#19342);
#16157=AXIS2_PLACEMENT_3D('',#42359,#19344,#19345);
#16158=AXIS2_PLACEMENT_3D('',#42363,#19347,#19348);
#16159=AXIS2_PLACEMENT_3D('',#42367,#19350,#19351);
#16160=AXIS2_PLACEMENT_3D('',#42371,#19353,#19354);
#16161=AXIS2_PLACEMENT_3D('',#42375,#19356,#19357);
#16162=AXIS2_PLACEMENT_3D('',#42379,#19359,#19360);
#16163=AXIS2_PLACEMENT_3D('',#42383,#19362,#19363);
#16164=AXIS2_PLACEMENT_3D('',#42387,#19365,#19366);
#16165=AXIS2_PLACEMENT_3D('',#42391,#19368,#19369);
#16166=AXIS2_PLACEMENT_3D('',#42395,#19371,#19372);
#16167=AXIS2_PLACEMENT_3D('',#42399,#19374,#19375);
#16168=AXIS2_PLACEMENT_3D('',#42403,#19377,#19378);
#16169=AXIS2_PLACEMENT_3D('',#42407,#19380,#19381);
#16170=AXIS2_PLACEMENT_3D('',#42410,#19383,#19384);
#16171=AXIS2_PLACEMENT_3D('',#42412,#19385,#19386);
#16172=AXIS2_PLACEMENT_3D('',#42416,#19388,#19389);
#16173=AXIS2_PLACEMENT_3D('',#42420,#19391,#19392);
#16174=AXIS2_PLACEMENT_3D('',#42424,#19394,#19395);
#16175=AXIS2_PLACEMENT_3D('',#42428,#19397,#19398);
#16176=AXIS2_PLACEMENT_3D('',#42432,#19400,#19401);
#16177=AXIS2_PLACEMENT_3D('',#42436,#19403,#19404);
#16178=AXIS2_PLACEMENT_3D('',#42440,#19406,#19407);
#16179=AXIS2_PLACEMENT_3D('',#42444,#19409,#19410);
#16180=AXIS2_PLACEMENT_3D('',#42448,#19412,#19413);
#16181=AXIS2_PLACEMENT_3D('',#42452,#19415,#19416);
#16182=AXIS2_PLACEMENT_3D('',#42456,#19418,#19419);
#16183=AXIS2_PLACEMENT_3D('',#42460,#19421,#19422);
#16184=AXIS2_PLACEMENT_3D('',#42464,#19424,#19425);
#16185=AXIS2_PLACEMENT_3D('',#42468,#19427,#19428);
#16186=AXIS2_PLACEMENT_3D('',#42472,#19430,#19431);
#16187=AXIS2_PLACEMENT_3D('',#42476,#19433,#19434);
#16188=AXIS2_PLACEMENT_3D('',#42480,#19436,#19437);
#16189=AXIS2_PLACEMENT_3D('',#42484,#19439,#19440);
#16190=AXIS2_PLACEMENT_3D('',#42488,#19442,#19443);
#16191=AXIS2_PLACEMENT_3D('',#42492,#19445,#19446);
#16192=AXIS2_PLACEMENT_3D('',#42496,#19448,#19449);
#16193=AXIS2_PLACEMENT_3D('',#42500,#19451,#19452);
#16194=AXIS2_PLACEMENT_3D('',#42504,#19454,#19455);
#16195=AXIS2_PLACEMENT_3D('',#42508,#19457,#19458);
#16196=AXIS2_PLACEMENT_3D('',#42512,#19460,#19461);
#16197=AXIS2_PLACEMENT_3D('',#42516,#19463,#19464);
#16198=AXIS2_PLACEMENT_3D('',#42520,#19466,#19467);
#16199=AXIS2_PLACEMENT_3D('',#42524,#19469,#19470);
#16200=AXIS2_PLACEMENT_3D('',#42528,#19472,#19473);
#16201=AXIS2_PLACEMENT_3D('',#42532,#19475,#19476);
#16202=AXIS2_PLACEMENT_3D('',#42536,#19478,#19479);
#16203=AXIS2_PLACEMENT_3D('',#42540,#19481,#19482);
#16204=AXIS2_PLACEMENT_3D('',#42544,#19484,#19485);
#16205=AXIS2_PLACEMENT_3D('',#42548,#19487,#19488);
#16206=AXIS2_PLACEMENT_3D('',#42552,#19490,#19491);
#16207=AXIS2_PLACEMENT_3D('',#42556,#19493,#19494);
#16208=AXIS2_PLACEMENT_3D('',#42558,#19496,#19497);
#16209=AXIS2_PLACEMENT_3D('',#42566,#19500,#19501);
#16210=AXIS2_PLACEMENT_3D('',#42571,#19503,#19504);
#16211=AXIS2_PLACEMENT_3D('',#42572,#19505,#19506);
#16212=AXIS2_PLACEMENT_3D('',#42813,#19508,#19509);
#16213=AXIS2_PLACEMENT_3D('',#42814,#19510,#19511);
#16214=AXIS2_PLACEMENT_3D('',#42818,#19514,#19515);
#16215=AXIS2_PLACEMENT_3D('',#42820,#19517,#19518);
#16216=AXIS2_PLACEMENT_3D('',#42821,#19519,#19520);
#16217=AXIS2_PLACEMENT_3D('',#42825,#19523,#19524);
#16218=AXIS2_PLACEMENT_3D('',#42827,#19526,#19527);
#16219=AXIS2_PLACEMENT_3D('',#42828,#19528,#19529);
#16220=AXIS2_PLACEMENT_3D('',#42832,#19532,#19533);
#16221=AXIS2_PLACEMENT_3D('',#42834,#19535,#19536);
#16222=AXIS2_PLACEMENT_3D('',#42835,#19537,#19538);
#16223=AXIS2_PLACEMENT_3D('',#42839,#19541,#19542);
#16224=AXIS2_PLACEMENT_3D('',#42841,#19544,#19545);
#16225=AXIS2_PLACEMENT_3D('',#42842,#19546,#19547);
#16226=AXIS2_PLACEMENT_3D('',#42846,#19550,#19551);
#16227=AXIS2_PLACEMENT_3D('',#42848,#19553,#19554);
#16228=AXIS2_PLACEMENT_3D('',#42849,#19555,#19556);
#16229=AXIS2_PLACEMENT_3D('',#42853,#19559,#19560);
#16230=AXIS2_PLACEMENT_3D('',#42855,#19562,#19563);
#16231=AXIS2_PLACEMENT_3D('',#42856,#19564,#19565);
#16232=AXIS2_PLACEMENT_3D('',#42860,#19568,#19569);
#16233=AXIS2_PLACEMENT_3D('',#42862,#19571,#19572);
#16234=AXIS2_PLACEMENT_3D('',#42863,#19573,#19574);
#16235=AXIS2_PLACEMENT_3D('',#42867,#19577,#19578);
#16236=AXIS2_PLACEMENT_3D('',#42869,#19580,#19581);
#16237=AXIS2_PLACEMENT_3D('',#42870,#19582,#19583);
#16238=AXIS2_PLACEMENT_3D('',#42874,#19586,#19587);
#16239=AXIS2_PLACEMENT_3D('',#42876,#19589,#19590);
#16240=AXIS2_PLACEMENT_3D('',#42877,#19591,#19592);
#16241=AXIS2_PLACEMENT_3D('',#42881,#19595,#19596);
#16242=AXIS2_PLACEMENT_3D('',#42883,#19598,#19599);
#16243=AXIS2_PLACEMENT_3D('',#42884,#19600,#19601);
#16244=AXIS2_PLACEMENT_3D('',#42888,#19604,#19605);
#16245=AXIS2_PLACEMENT_3D('',#42890,#19607,#19608);
#16246=AXIS2_PLACEMENT_3D('',#42891,#19609,#19610);
#16247=AXIS2_PLACEMENT_3D('',#42895,#19613,#19614);
#16248=AXIS2_PLACEMENT_3D('',#42897,#19616,#19617);
#16249=AXIS2_PLACEMENT_3D('',#42898,#19618,#19619);
#16250=AXIS2_PLACEMENT_3D('',#42902,#19622,#19623);
#16251=AXIS2_PLACEMENT_3D('',#42904,#19625,#19626);
#16252=AXIS2_PLACEMENT_3D('',#42905,#19627,#19628);
#16253=AXIS2_PLACEMENT_3D('',#42909,#19631,#19632);
#16254=AXIS2_PLACEMENT_3D('',#42911,#19634,#19635);
#16255=AXIS2_PLACEMENT_3D('',#42912,#19636,#19637);
#16256=AXIS2_PLACEMENT_3D('',#42916,#19640,#19641);
#16257=AXIS2_PLACEMENT_3D('',#42918,#19643,#19644);
#16258=AXIS2_PLACEMENT_3D('',#42919,#19645,#19646);
#16259=AXIS2_PLACEMENT_3D('',#42923,#19649,#19650);
#16260=AXIS2_PLACEMENT_3D('',#42925,#19652,#19653);
#16261=AXIS2_PLACEMENT_3D('',#42926,#19654,#19655);
#16262=AXIS2_PLACEMENT_3D('',#42930,#19658,#19659);
#16263=AXIS2_PLACEMENT_3D('',#42932,#19661,#19662);
#16264=AXIS2_PLACEMENT_3D('',#42933,#19663,#19664);
#16265=AXIS2_PLACEMENT_3D('',#42937,#19667,#19668);
#16266=AXIS2_PLACEMENT_3D('',#42939,#19670,#19671);
#16267=AXIS2_PLACEMENT_3D('',#42940,#19672,#19673);
#16268=AXIS2_PLACEMENT_3D('',#42944,#19676,#19677);
#16269=AXIS2_PLACEMENT_3D('',#42946,#19679,#19680);
#16270=AXIS2_PLACEMENT_3D('',#42947,#19681,#19682);
#16271=AXIS2_PLACEMENT_3D('',#42951,#19685,#19686);
#16272=AXIS2_PLACEMENT_3D('',#42953,#19688,#19689);
#16273=AXIS2_PLACEMENT_3D('',#42954,#19690,#19691);
#16274=AXIS2_PLACEMENT_3D('',#42958,#19694,#19695);
#16275=AXIS2_PLACEMENT_3D('',#42960,#19697,#19698);
#16276=AXIS2_PLACEMENT_3D('',#42961,#19699,#19700);
#16277=AXIS2_PLACEMENT_3D('',#42965,#19703,#19704);
#16278=AXIS2_PLACEMENT_3D('',#42967,#19706,#19707);
#16279=AXIS2_PLACEMENT_3D('',#42968,#19708,#19709);
#16280=AXIS2_PLACEMENT_3D('',#42972,#19712,#19713);
#16281=AXIS2_PLACEMENT_3D('',#42974,#19715,#19716);
#16282=AXIS2_PLACEMENT_3D('',#42975,#19717,#19718);
#16283=AXIS2_PLACEMENT_3D('',#42979,#19721,#19722);
#16284=AXIS2_PLACEMENT_3D('',#42981,#19724,#19725);
#16285=AXIS2_PLACEMENT_3D('',#42982,#19726,#19727);
#16286=AXIS2_PLACEMENT_3D('',#42986,#19730,#19731);
#16287=AXIS2_PLACEMENT_3D('',#42988,#19733,#19734);
#16288=AXIS2_PLACEMENT_3D('',#42989,#19735,#19736);
#16289=AXIS2_PLACEMENT_3D('',#42993,#19739,#19740);
#16290=AXIS2_PLACEMENT_3D('',#42995,#19742,#19743);
#16291=AXIS2_PLACEMENT_3D('',#42996,#19744,#19745);
#16292=AXIS2_PLACEMENT_3D('',#43000,#19748,#19749);
#16293=AXIS2_PLACEMENT_3D('',#43002,#19751,#19752);
#16294=AXIS2_PLACEMENT_3D('',#43003,#19753,#19754);
#16295=AXIS2_PLACEMENT_3D('',#43007,#19757,#19758);
#16296=AXIS2_PLACEMENT_3D('',#43009,#19760,#19761);
#16297=AXIS2_PLACEMENT_3D('',#43010,#19762,#19763);
#16298=AXIS2_PLACEMENT_3D('',#43014,#19766,#19767);
#16299=AXIS2_PLACEMENT_3D('',#43016,#19769,#19770);
#16300=AXIS2_PLACEMENT_3D('',#43017,#19771,#19772);
#16301=AXIS2_PLACEMENT_3D('',#43021,#19775,#19776);
#16302=AXIS2_PLACEMENT_3D('',#43023,#19778,#19779);
#16303=AXIS2_PLACEMENT_3D('',#43024,#19780,#19781);
#16304=AXIS2_PLACEMENT_3D('',#43028,#19784,#19785);
#16305=AXIS2_PLACEMENT_3D('',#43030,#19787,#19788);
#16306=AXIS2_PLACEMENT_3D('',#43031,#19789,#19790);
#16307=AXIS2_PLACEMENT_3D('',#43035,#19793,#19794);
#16308=AXIS2_PLACEMENT_3D('',#43037,#19796,#19797);
#16309=AXIS2_PLACEMENT_3D('',#43038,#19798,#19799);
#16310=AXIS2_PLACEMENT_3D('',#43042,#19802,#19803);
#16311=AXIS2_PLACEMENT_3D('',#43044,#19805,#19806);
#16312=AXIS2_PLACEMENT_3D('',#43045,#19807,#19808);
#16313=AXIS2_PLACEMENT_3D('',#43049,#19811,#19812);
#16314=AXIS2_PLACEMENT_3D('',#43051,#19814,#19815);
#16315=AXIS2_PLACEMENT_3D('',#43052,#19816,#19817);
#16316=AXIS2_PLACEMENT_3D('',#43053,#19818,#19819);
#16317=AXIS2_PLACEMENT_3D('',#43054,#19820,#19821);
#16318=AXIS2_PLACEMENT_3D('',#43056,#19822,#19823);
#16319=AXIS2_PLACEMENT_3D('',#43057,#19824,#19825);
#16320=AXIS2_PLACEMENT_3D('',#43064,#19826,#19827);
#16321=AXIS2_PLACEMENT_3D('',#43074,#19828,#19829);
#16322=AXIS2_PLACEMENT_3D('',#43084,#19830,#19831);
#16323=AXIS2_PLACEMENT_3D('',#43094,#19832,#19833);
#16324=AXIS2_PLACEMENT_3D('',#43104,#19834,#19835);
#16325=AXIS2_PLACEMENT_3D('',#43114,#19836,#19837);
#16326=AXIS2_PLACEMENT_3D('',#43119,#19839,#19840);
#16327=AXIS2_PLACEMENT_3D('',#43124,#19843,#19844);
#16328=AXIS2_PLACEMENT_3D('',#43125,#19845,#19846);
#16329=AXIS2_PLACEMENT_3D('',#43130,#19849,#19850);
#16330=AXIS2_PLACEMENT_3D('',#43131,#19851,#19852);
#16331=AXIS2_PLACEMENT_3D('',#43135,#19854,#19855);
#16332=AXIS2_PLACEMENT_3D('',#43137,#19857,#19858);
#16333=AXIS2_PLACEMENT_3D('',#43142,#19861,#19862);
#16334=AXIS2_PLACEMENT_3D('',#43143,#19863,#19864);
#16335=AXIS2_PLACEMENT_3D('',#43147,#19866,#19867);
#16336=AXIS2_PLACEMENT_3D('',#43149,#19869,#19870);
#16337=AXIS2_PLACEMENT_3D('',#43153,#19872,#19873);
#16338=AXIS2_PLACEMENT_3D('',#43155,#19875,#19876);
#16339=AXIS2_PLACEMENT_3D('',#43162,#19881,#19882);
#16340=AXIS2_PLACEMENT_3D('',#43167,#19886,#19887);
#16341=AXIS2_PLACEMENT_3D('',#43172,#19891,#19892);
#16342=AXIS2_PLACEMENT_3D('',#43173,#19893,#19894);
#16343=AXIS2_PLACEMENT_3D('',#43174,#19895,#19896);
#16344=AXIS2_PLACEMENT_3D('',#43176,#19898,#19899);
#16345=AXIS2_PLACEMENT_3D('',#43177,#19900,#19901);
#16346=AXIS2_PLACEMENT_3D('',#43179,#19903,#19904);
#16347=AXIS2_PLACEMENT_3D('',#43181,#19906,#19907);
#16348=AXIS2_PLACEMENT_3D('',#43184,#19909,#19910);
#16349=AXIS2_PLACEMENT_3D('',#43185,#19911,#19912);
#16350=AXIS2_PLACEMENT_3D('',#43186,#19913,#19914);
#16351=AXIS2_PLACEMENT_3D('',#43187,#19915,#19916);
#16352=AXIS2_PLACEMENT_3D('',#43188,#19917,#19918);
#16353=AXIS2_PLACEMENT_3D('',#43189,#19919,#19920);
#16354=AXIS2_PLACEMENT_3D('',#43190,#19921,#19922);
#16355=AXIS2_PLACEMENT_3D('',#43191,#19923,#19924);
#16356=AXIS2_PLACEMENT_3D('',#43194,#19926,#19927);
#16357=AXIS2_PLACEMENT_3D('',#43195,#19928,#19929);
#16358=AXIS2_PLACEMENT_3D('',#43197,#19931,#19932);
#16359=AXIS2_PLACEMENT_3D('',#43198,#19933,#19934);
#16360=AXIS2_PLACEMENT_3D('',#43201,#19936,#19937);
#16361=AXIS2_PLACEMENT_3D('',#43203,#19939,#19940);
#16362=AXIS2_PLACEMENT_3D('',#43205,#19942,#19943);
#19149=DIRECTION('axis',(0.,0.,1.));
#19150=DIRECTION('refdir',(1.,0.,0.));
#19151=DIRECTION('center_axis',(0.,0.,1.));
#19152=DIRECTION('ref_axis',(-0.0824405823441869,-0.996595981520471,0.));
#19153=DIRECTION('',(0.,0.,-1.));
#19154=DIRECTION('center_axis',(0.,0.,-1.));
#19155=DIRECTION('ref_axis',(1.,-2.89417707885741E-14,0.));
#19156=DIRECTION('center_axis',(0.,0.,1.));
#19157=DIRECTION('ref_axis',(-0.0824405823441869,-0.996595981520471,0.));
#19158=DIRECTION('',(0.,0.,-1.));
#19159=DIRECTION('center_axis',(0.,0.,1.));
#19160=DIRECTION('ref_axis',(-0.0824405823441869,-0.996595981520471,0.));
#19161=DIRECTION('',(0.,0.,-1.));
#19162=DIRECTION('center_axis',(0.,0.,1.));
#19163=DIRECTION('ref_axis',(-0.0824405823441869,-0.996595981520471,0.));
#19164=DIRECTION('',(0.,0.,-1.));
#19165=DIRECTION('center_axis',(0.,0.,1.));
#19166=DIRECTION('ref_axis',(-0.0824405823441869,-0.996595981520471,0.));
#19167=DIRECTION('',(0.,0.,-1.));
#19168=DIRECTION('center_axis',(0.,0.,1.));
#19169=DIRECTION('ref_axis',(-0.0824405823441869,-0.996595981520471,0.));
#19170=DIRECTION('',(0.,0.,-1.));
#19171=DIRECTION('center_axis',(0.,0.,1.));
#19172=DIRECTION('ref_axis',(-0.0824405823441869,-0.996595981520471,0.));
#19173=DIRECTION('',(0.,0.,-1.));
#19174=DIRECTION('center_axis',(0.,0.,1.));
#19175=DIRECTION('ref_axis',(-0.0824405823441869,-0.996595981520471,0.));
#19176=DIRECTION('',(0.,0.,-1.));
#19177=DIRECTION('center_axis',(0.,0.,1.));
#19178=DIRECTION('ref_axis',(-0.0824405823441869,-0.996595981520471,0.));
#19179=DIRECTION('',(0.,0.,-1.));
#19180=DIRECTION('center_axis',(0.,0.,1.));
#19181=DIRECTION('ref_axis',(-0.0824405823441869,-0.996595981520471,0.));
#19182=DIRECTION('',(0.,0.,-1.));
#19183=DIRECTION('center_axis',(0.,0.,1.));
#19184=DIRECTION('ref_axis',(-0.0824405823441869,-0.996595981520471,0.));
#19185=DIRECTION('',(0.,0.,-1.));
#19186=DIRECTION('center_axis',(0.,0.,1.));
#19187=DIRECTION('ref_axis',(-0.0824405823441869,-0.996595981520471,0.));
#19188=DIRECTION('',(0.,0.,-1.));
#19189=DIRECTION('center_axis',(0.,0.,1.));
#19190=DIRECTION('ref_axis',(-0.0824405823441869,-0.996595981520471,0.));
#19191=DIRECTION('',(0.,0.,-1.));
#19192=DIRECTION('center_axis',(0.,0.,1.));
#19193=DIRECTION('ref_axis',(-0.0824405823441869,-0.996595981520471,0.));
#19194=DIRECTION('',(0.,0.,-1.));
#19195=DIRECTION('center_axis',(0.,0.,1.));
#19196=DIRECTION('ref_axis',(-0.0824405823441869,-0.996595981520471,0.));
#19197=DIRECTION('',(0.,0.,-1.));
#19198=DIRECTION('center_axis',(0.,0.,1.));
#19199=DIRECTION('ref_axis',(-0.0824405823441869,-0.996595981520471,0.));
#19200=DIRECTION('',(0.,0.,-1.));
#19201=DIRECTION('center_axis',(0.,0.,1.));
#19202=DIRECTION('ref_axis',(-0.0824405823441869,-0.996595981520471,0.));
#19203=DIRECTION('',(0.,0.,-1.));
#19204=DIRECTION('center_axis',(0.,0.,1.));
#19205=DIRECTION('ref_axis',(-0.0824405823441869,-0.996595981520471,0.));
#19206=DIRECTION('',(0.,0.,-1.));
#19207=DIRECTION('center_axis',(0.,0.,1.));
#19208=DIRECTION('ref_axis',(-0.0824405823441869,-0.996595981520471,0.));
#19209=DIRECTION('',(0.,0.,-1.));
#19210=DIRECTION('center_axis',(0.,0.,1.));
#19211=DIRECTION('ref_axis',(-0.0824405823441869,-0.996595981520471,0.));
#19212=DIRECTION('',(0.,0.,-1.));
#19213=DIRECTION('center_axis',(0.,0.,1.));
#19214=DIRECTION('ref_axis',(-0.0824405823441869,-0.996595981520471,0.));
#19215=DIRECTION('',(0.,0.,-1.));
#19216=DIRECTION('center_axis',(0.,0.,1.));
#19217=DIRECTION('ref_axis',(-0.0824405823441869,-0.996595981520471,0.));
#19218=DIRECTION('',(0.,0.,-1.));
#19219=DIRECTION('center_axis',(0.,0.,1.));
#19220=DIRECTION('ref_axis',(-0.0824405823441869,-0.996595981520471,0.));
#19221=DIRECTION('',(0.,0.,-1.));
#19222=DIRECTION('center_axis',(0.,0.,1.));
#19223=DIRECTION('ref_axis',(-0.0824405823441869,-0.996595981520471,0.));
#19224=DIRECTION('',(0.,0.,-1.));
#19225=DIRECTION('center_axis',(0.,0.,1.));
#19226=DIRECTION('ref_axis',(1.,0.,0.));
#19227=DIRECTION('center_axis',(0.,0.,-1.));
#19228=DIRECTION('ref_axis',(1.,0.,0.));
#19229=DIRECTION('center_axis',(0.,0.,1.));
#19230=DIRECTION('ref_axis',(1.,0.,0.));
#19231=DIRECTION('center_axis',(0.,0.,1.));
#19232=DIRECTION('ref_axis',(-0.0824405823441869,-0.996595981520471,0.));
#19233=DIRECTION('center_axis',(0.,0.,1.));
#19234=DIRECTION('ref_axis',(1.,-2.89417707885741E-14,0.));
#19235=DIRECTION('center_axis',(0.,0.,1.));
#19236=DIRECTION('ref_axis',(1.,0.,0.));
#19237=DIRECTION('center_axis',(0.,0.,1.));
#19238=DIRECTION('ref_axis',(1.,0.,0.));
#19239=DIRECTION('center_axis',(0.,0.,1.));
#19240=DIRECTION('ref_axis',(1.,0.,0.));
#19241=DIRECTION('center_axis',(0.,0.,1.));
#19242=DIRECTION('ref_axis',(1.,0.,0.));
#19243=DIRECTION('center_axis',(0.,0.,-1.));
#19244=DIRECTION('ref_axis',(1.,0.,0.));
#19245=DIRECTION('center_axis',(0.,0.,-1.));
#19246=DIRECTION('ref_axis',(1.,0.,0.));
#19247=DIRECTION('center_axis',(0.,0.,-1.));
#19248=DIRECTION('ref_axis',(-1.,0.,0.));
#19249=DIRECTION('center_axis',(0.,0.,1.));
#19250=DIRECTION('ref_axis',(1.,0.,0.));
#19251=DIRECTION('center_axis',(0.,1.,0.));
#19252=DIRECTION('ref_axis',(1.,0.,0.));
#19253=DIRECTION('center_axis',(0.,0.,1.));
#19254=DIRECTION('ref_axis',(1.,0.,0.));
#19255=DIRECTION('center_axis',(0.,0.,-1.));
#19256=DIRECTION('ref_axis',(1.,0.,0.));
#19257=DIRECTION('center_axis',(0.,0.,-1.));
#19258=DIRECTION('ref_axis',(1.,0.,0.));
#19259=DIRECTION('',(0.707106781186547,-8.65956056235493E-17,0.707106781186548));
#19260=DIRECTION('center_axis',(0.,0.,-1.));
#19261=DIRECTION('ref_axis',(1.,0.,0.));
#19262=DIRECTION('center_axis',(0.,0.,1.));
#19263=DIRECTION('ref_axis',(1.,0.,0.));
#19264=DIRECTION('center_axis',(0.,0.,1.));
#19265=DIRECTION('ref_axis',(0.984807753012208,-0.17364817766693,0.));
#19266=DIRECTION('center_axis',(0.,0.,1.));
#19267=DIRECTION('ref_axis',(1.,0.,0.));
#19268=DIRECTION('',(0.808467844782638,-0.588540350318069,0.));
#19269=DIRECTION('',(-0.961003922853658,-0.276534736081891,0.));
#19270=DIRECTION('center_axis',(-0.276534736081891,0.961003922853658,0.));
#19271=DIRECTION('ref_axis',(-0.961003922853658,-0.276534736081891,0.));
#19272=DIRECTION('',(0.,0.,-1.));
#19273=DIRECTION('',(0.,0.,1.));
#19274=DIRECTION('center_axis',(-0.58854035031807,-0.808467844782638,0.));
#19275=DIRECTION('ref_axis',(0.808467844782638,-0.58854035031807,0.));
#19276=DIRECTION('',(0.,0.,1.));
#19277=DIRECTION('center_axis',(0.,0.,-1.));
#19278=DIRECTION('ref_axis',(1.,0.,0.));
#19279=DIRECTION('center_axis',(0.,0.,1.));
#19280=DIRECTION('ref_axis',(1.,0.,0.));
#19281=DIRECTION('',(0.,0.,1.));
#19282=DIRECTION('center_axis',(0.,0.,1.));
#19283=DIRECTION('ref_axis',(1.,0.,0.));
#19284=DIRECTION('center_axis',(0.,0.,1.));
#19285=DIRECTION('ref_axis',(1.,0.,0.));
#19286=DIRECTION('',(0.,0.,-1.));
#19287=DIRECTION('center_axis',(0.,0.,-1.));
#19288=DIRECTION('ref_axis',(1.,0.,0.));
#19289=DIRECTION('',(0.,0.,1.));
#19290=DIRECTION('center_axis',(0.,0.,1.));
#19291=DIRECTION('ref_axis',(1.,0.,0.));
#19292=DIRECTION('',(0.,0.,-1.));
#19293=DIRECTION('center_axis',(0.,0.,-1.));
#19294=DIRECTION('ref_axis',(1.,0.,0.));
#19295=DIRECTION('',(0.,0.,1.));
#19296=DIRECTION('center_axis',(0.,0.,1.));
#19297=DIRECTION('ref_axis',(1.,0.,0.));
#19298=DIRECTION('',(0.,0.,-1.));
#19299=DIRECTION('center_axis',(0.,0.,-1.));
#19300=DIRECTION('ref_axis',(1.,0.,0.));
#19301=DIRECTION('',(0.,0.,1.));
#19302=DIRECTION('center_axis',(0.,0.,1.));
#19303=DIRECTION('ref_axis',(1.,0.,0.));
#19304=DIRECTION('',(0.,0.,-1.));
#19305=DIRECTION('center_axis',(0.,0.,-1.));
#19306=DIRECTION('ref_axis',(1.,0.,0.));
#19307=DIRECTION('',(0.,0.,1.));
#19308=DIRECTION('center_axis',(0.,0.,1.));
#19309=DIRECTION('ref_axis',(1.,0.,0.));
#19310=DIRECTION('',(0.,0.,-1.));
#19311=DIRECTION('center_axis',(0.,0.,-1.));
#19312=DIRECTION('ref_axis',(1.,0.,0.));
#19313=DIRECTION('',(0.,0.,1.));
#19314=DIRECTION('center_axis',(0.,0.,1.));
#19315=DIRECTION('ref_axis',(1.,0.,0.));
#19316=DIRECTION('',(0.,0.,-1.));
#19317=DIRECTION('center_axis',(0.,0.,-1.));
#19318=DIRECTION('ref_axis',(1.,0.,0.));
#19319=DIRECTION('',(0.,0.,1.));
#19320=DIRECTION('center_axis',(0.,0.,1.));
#19321=DIRECTION('ref_axis',(1.,0.,0.));
#19322=DIRECTION('',(0.,0.,-1.));
#19323=DIRECTION('center_axis',(0.,0.,-1.));
#19324=DIRECTION('ref_axis',(1.,0.,0.));
#19325=DIRECTION('',(0.,0.,1.));
#19326=DIRECTION('center_axis',(0.,0.,1.));
#19327=DIRECTION('ref_axis',(1.,0.,0.));
#19328=DIRECTION('',(0.,0.,-1.));
#19329=DIRECTION('center_axis',(0.,0.,-1.));
#19330=DIRECTION('ref_axis',(1.,0.,0.));
#19331=DIRECTION('',(0.,0.,1.));
#19332=DIRECTION('center_axis',(0.,0.,1.));
#19333=DIRECTION('ref_axis',(1.,0.,0.));
#19334=DIRECTION('',(0.,0.,-1.));
#19335=DIRECTION('center_axis',(0.,0.,-1.));
#19336=DIRECTION('ref_axis',(1.,0.,0.));
#19337=DIRECTION('',(0.,0.,1.));
#19338=DIRECTION('center_axis',(0.,0.,1.));
#19339=DIRECTION('ref_axis',(1.,0.,0.));
#19340=DIRECTION('',(0.,0.,-1.));
#19341=DIRECTION('center_axis',(0.,0.,-1.));
#19342=DIRECTION('ref_axis',(1.,0.,0.));
#19343=DIRECTION('',(0.,0.,1.));
#19344=DIRECTION('center_axis',(0.,0.,1.));
#19345=DIRECTION('ref_axis',(1.,0.,0.));
#19346=DIRECTION('',(0.,0.,-1.));
#19347=DIRECTION('center_axis',(0.,0.,-1.));
#19348=DIRECTION('ref_axis',(1.,0.,0.));
#19349=DIRECTION('',(0.,0.,1.));
#19350=DIRECTION('center_axis',(0.,0.,1.));
#19351=DIRECTION('ref_axis',(1.,0.,0.));
#19352=DIRECTION('',(0.,0.,-1.));
#19353=DIRECTION('center_axis',(0.,0.,-1.));
#19354=DIRECTION('ref_axis',(1.,0.,0.));
#19355=DIRECTION('',(0.,0.,1.));
#19356=DIRECTION('center_axis',(0.,0.,1.));
#19357=DIRECTION('ref_axis',(1.,0.,0.));
#19358=DIRECTION('',(0.,0.,-1.));
#19359=DIRECTION('center_axis',(0.,0.,-1.));
#19360=DIRECTION('ref_axis',(1.,0.,0.));
#19361=DIRECTION('',(0.,0.,1.));
#19362=DIRECTION('center_axis',(0.,0.,1.));
#19363=DIRECTION('ref_axis',(1.,0.,0.));
#19364=DIRECTION('',(0.,0.,-1.));
#19365=DIRECTION('center_axis',(0.,0.,-1.));
#19366=DIRECTION('ref_axis',(1.,0.,0.));
#19367=DIRECTION('',(0.,0.,1.));
#19368=DIRECTION('center_axis',(0.,0.,1.));
#19369=DIRECTION('ref_axis',(1.,0.,0.));
#19370=DIRECTION('',(0.,0.,-1.));
#19371=DIRECTION('center_axis',(0.,0.,-1.));
#19372=DIRECTION('ref_axis',(1.,0.,0.));
#19373=DIRECTION('',(0.,0.,1.));
#19374=DIRECTION('center_axis',(0.,0.,1.));
#19375=DIRECTION('ref_axis',(1.,0.,0.));
#19376=DIRECTION('',(0.,0.,-1.));
#19377=DIRECTION('center_axis',(0.,0.,-1.));
#19378=DIRECTION('ref_axis',(1.,0.,0.));
#19379=DIRECTION('',(0.,0.,1.));
#19380=DIRECTION('center_axis',(0.,0.,1.));
#19381=DIRECTION('ref_axis',(1.,0.,0.));
#19382=DIRECTION('',(0.,0.,-1.));
#19383=DIRECTION('center_axis',(0.,0.,-1.));
#19384=DIRECTION('ref_axis',(1.,0.,0.));
#19385=DIRECTION('center_axis',(0.,0.,-1.));
#19386=DIRECTION('ref_axis',(1.,0.,0.));
#19387=DIRECTION('',(0.,0.,1.));
#19388=DIRECTION('center_axis',(0.,0.,1.));
#19389=DIRECTION('ref_axis',(1.,0.,0.));
#19390=DIRECTION('',(0.,0.,-1.));
#19391=DIRECTION('center_axis',(0.,0.,-1.));
#19392=DIRECTION('ref_axis',(1.,0.,0.));
#19393=DIRECTION('',(0.,0.,1.));
#19394=DIRECTION('center_axis',(0.,0.,1.));
#19395=DIRECTION('ref_axis',(1.,0.,0.));
#19396=DIRECTION('',(0.,0.,-1.));
#19397=DIRECTION('center_axis',(0.,0.,-1.));
#19398=DIRECTION('ref_axis',(1.,0.,0.));
#19399=DIRECTION('',(0.,0.,1.));
#19400=DIRECTION('center_axis',(0.,0.,1.));
#19401=DIRECTION('ref_axis',(1.,0.,0.));
#19402=DIRECTION('',(0.,0.,-1.));
#19403=DIRECTION('center_axis',(0.,0.,-1.));
#19404=DIRECTION('ref_axis',(1.,0.,0.));
#19405=DIRECTION('',(0.,0.,1.));
#19406=DIRECTION('center_axis',(0.,0.,1.));
#19407=DIRECTION('ref_axis',(1.,0.,0.));
#19408=DIRECTION('',(0.,0.,-1.));
#19409=DIRECTION('center_axis',(0.,0.,-1.));
#19410=DIRECTION('ref_axis',(1.,0.,0.));
#19411=DIRECTION('',(0.,0.,1.));
#19412=DIRECTION('center_axis',(0.,0.,1.));
#19413=DIRECTION('ref_axis',(1.,0.,0.));
#19414=DIRECTION('',(0.,0.,-1.));
#19415=DIRECTION('center_axis',(0.,0.,-1.));
#19416=DIRECTION('ref_axis',(1.,0.,0.));
#19417=DIRECTION('',(0.,0.,1.));
#19418=DIRECTION('center_axis',(0.,0.,1.));
#19419=DIRECTION('ref_axis',(1.,0.,0.));
#19420=DIRECTION('',(0.,0.,-1.));
#19421=DIRECTION('center_axis',(0.,0.,-1.));
#19422=DIRECTION('ref_axis',(1.,0.,0.));
#19423=DIRECTION('',(0.,0.,1.));
#19424=DIRECTION('center_axis',(0.,0.,1.));
#19425=DIRECTION('ref_axis',(1.,0.,0.));
#19426=DIRECTION('',(0.,0.,-1.));
#19427=DIRECTION('center_axis',(0.,0.,-1.));
#19428=DIRECTION('ref_axis',(1.,0.,0.));
#19429=DIRECTION('',(0.,0.,1.));
#19430=DIRECTION('center_axis',(0.,0.,1.));
#19431=DIRECTION('ref_axis',(1.,0.,0.));
#19432=DIRECTION('',(0.,0.,-1.));
#19433=DIRECTION('center_axis',(0.,0.,-1.));
#19434=DIRECTION('ref_axis',(1.,0.,0.));
#19435=DIRECTION('',(0.,0.,1.));
#19436=DIRECTION('center_axis',(0.,0.,1.));
#19437=DIRECTION('ref_axis',(1.,0.,0.));
#19438=DIRECTION('',(0.,0.,-1.));
#19439=DIRECTION('center_axis',(0.,0.,-1.));
#19440=DIRECTION('ref_axis',(1.,0.,0.));
#19441=DIRECTION('',(0.,0.,1.));
#19442=DIRECTION('center_axis',(0.,0.,1.));
#19443=DIRECTION('ref_axis',(1.,0.,0.));
#19444=DIRECTION('',(0.,0.,-1.));
#19445=DIRECTION('center_axis',(0.,0.,-1.));
#19446=DIRECTION('ref_axis',(1.,0.,0.));
#19447=DIRECTION('',(0.,0.,1.));
#19448=DIRECTION('center_axis',(0.,0.,1.));
#19449=DIRECTION('ref_axis',(1.,0.,0.));
#19450=DIRECTION('',(0.,0.,-1.));
#19451=DIRECTION('center_axis',(0.,0.,-1.));
#19452=DIRECTION('ref_axis',(1.,0.,0.));
#19453=DIRECTION('',(0.,0.,1.));
#19454=DIRECTION('center_axis',(0.,0.,1.));
#19455=DIRECTION('ref_axis',(1.,0.,0.));
#19456=DIRECTION('',(0.,0.,-1.));
#19457=DIRECTION('center_axis',(0.,0.,-1.));
#19458=DIRECTION('ref_axis',(1.,0.,0.));
#19459=DIRECTION('',(0.,0.,1.));
#19460=DIRECTION('center_axis',(0.,0.,1.));
#19461=DIRECTION('ref_axis',(1.,0.,0.));
#19462=DIRECTION('',(0.,0.,-1.));
#19463=DIRECTION('center_axis',(0.,0.,-1.));
#19464=DIRECTION('ref_axis',(1.,0.,0.));
#19465=DIRECTION('',(0.,0.,1.));
#19466=DIRECTION('center_axis',(0.,0.,1.));
#19467=DIRECTION('ref_axis',(1.,0.,0.));
#19468=DIRECTION('',(0.,0.,-1.));
#19469=DIRECTION('center_axis',(0.,0.,-1.));
#19470=DIRECTION('ref_axis',(1.,0.,0.));
#19471=DIRECTION('',(0.,0.,1.));
#19472=DIRECTION('center_axis',(0.,0.,1.));
#19473=DIRECTION('ref_axis',(1.,0.,0.));
#19474=DIRECTION('',(0.,0.,-1.));
#19475=DIRECTION('center_axis',(0.,0.,-1.));
#19476=DIRECTION('ref_axis',(1.,0.,0.));
#19477=DIRECTION('',(0.,0.,1.));
#19478=DIRECTION('center_axis',(0.,0.,1.));
#19479=DIRECTION('ref_axis',(1.,0.,0.));
#19480=DIRECTION('',(0.,0.,-1.));
#19481=DIRECTION('center_axis',(0.,0.,-1.));
#19482=DIRECTION('ref_axis',(1.,0.,0.));
#19483=DIRECTION('',(0.,0.,1.));
#19484=DIRECTION('center_axis',(0.,0.,1.));
#19485=DIRECTION('ref_axis',(1.,0.,0.));
#19486=DIRECTION('',(0.,0.,-1.));
#19487=DIRECTION('center_axis',(0.,0.,-1.));
#19488=DIRECTION('ref_axis',(1.,0.,0.));
#19489=DIRECTION('',(0.,0.,1.));
#19490=DIRECTION('center_axis',(0.,0.,1.));
#19491=DIRECTION('ref_axis',(1.,0.,0.));
#19492=DIRECTION('',(0.,0.,-1.));
#19493=DIRECTION('center_axis',(0.,0.,-1.));
#19494=DIRECTION('ref_axis',(1.,0.,0.));
#19495=DIRECTION('',(0.,0.,1.));
#19496=DIRECTION('center_axis',(-0.105456972136321,0.994423866883654,0.));
#19497=DIRECTION('ref_axis',(-0.994423866883654,-0.105456972136321,0.));
#19498=DIRECTION('',(-0.994423866883654,-0.105456972136321,0.));
#19499=DIRECTION('',(0.,0.,1.));
#19500=DIRECTION('center_axis',(-0.719988067902572,-0.693986442286822,0.));
#19501=DIRECTION('ref_axis',(0.693986442286822,-0.719988067902572,0.));
#19502=DIRECTION('',(0.693986442286822,-0.719988067902572,0.));
#19503=DIRECTION('center_axis',(0.,0.,1.));
#19504=DIRECTION('ref_axis',(0.939692620785908,-0.342020143325669,0.));
#19505=DIRECTION('center_axis',(0.,0.,1.));
#19506=DIRECTION('ref_axis',(1.,0.,0.));
#19507=DIRECTION('',(0.707106781186547,8.65956056235493E-17,-0.707106781186548));
#19508=DIRECTION('center_axis',(0.,0.,1.));
#19509=DIRECTION('ref_axis',(1.,0.,0.));
#19510=DIRECTION('center_axis',(0.,0.,1.));
#19511=DIRECTION('ref_axis',(0.866025403784438,-0.5,0.));
#19512=DIRECTION('',(0.558418612916207,-0.829559312375396,0.));
#19513=DIRECTION('',(-0.997628744921147,0.0688250485438069,0.));
#19514=DIRECTION('center_axis',(0.0688250485438069,0.997628744921147,0.));
#19515=DIRECTION('ref_axis',(-0.997628744921147,0.0688250485438069,0.));
#19516=DIRECTION('',(0.,0.,1.));
#19517=DIRECTION('center_axis',(-0.829559312375396,-0.558418612916207,0.));
#19518=DIRECTION('ref_axis',(0.558418612916207,-0.829559312375396,0.));
#19519=DIRECTION('center_axis',(0.241015854951086,0.970521178368714,0.));
#19520=DIRECTION('ref_axis',(-0.970521178368714,0.241015854951086,0.));
#19521=DIRECTION('',(-0.970521178368714,0.241015854951086,0.));
#19522=DIRECTION('',(0.,0.,1.));
#19523=DIRECTION('center_axis',(-0.91392481691896,-0.405883516565584,0.));
#19524=DIRECTION('ref_axis',(0.405883516565584,-0.91392481691896,0.));
#19525=DIRECTION('',(0.405883516565584,-0.91392481691896,0.));
#19526=DIRECTION('center_axis',(0.,0.,1.));
#19527=DIRECTION('ref_axis',(0.766044443118978,-0.64278760968654,0.));
#19528=DIRECTION('center_axis',(0.,0.,1.));
#19529=DIRECTION('ref_axis',(0.642787609686539,-0.766044443118978,0.));
#19530=DIRECTION('',(0.241015854951086,-0.970521178368714,0.));
#19531=DIRECTION('',(-0.91392481691896,0.405883516565585,0.));
#19532=DIRECTION('center_axis',(0.405883516565585,0.91392481691896,0.));
#19533=DIRECTION('ref_axis',(-0.91392481691896,0.405883516565585,0.));
#19534=DIRECTION('',(0.,0.,1.));
#19535=DIRECTION('center_axis',(-0.970521178368714,-0.241015854951086,0.));
#19536=DIRECTION('ref_axis',(0.241015854951086,-0.970521178368714,0.));
#19537=DIRECTION('center_axis',(0.558418612916207,0.829559312375396,0.));
#19538=DIRECTION('ref_axis',(-0.829559312375396,0.558418612916207,0.));
#19539=DIRECTION('',(-0.829559312375396,0.558418612916207,0.));
#19540=DIRECTION('',(0.,0.,1.));
#19541=DIRECTION('center_axis',(-0.997628744921147,-0.0688250485438065,
0.));
#19542=DIRECTION('ref_axis',(0.0688250485438065,-0.997628744921147,0.));
#19543=DIRECTION('',(0.0688250485438065,-0.997628744921147,0.));
#19544=DIRECTION('center_axis',(0.,0.,1.));
#19545=DIRECTION('ref_axis',(0.5,-0.866025403784439,0.));
#19546=DIRECTION('center_axis',(0.,0.,1.));
#19547=DIRECTION('ref_axis',(0.342020143325668,-0.939692620785909,0.));
#19548=DIRECTION('',(-0.105456972136323,-0.994423866883654,0.));
#19549=DIRECTION('',(-0.719988067902571,0.693986442286823,0.));
#19550=DIRECTION('center_axis',(0.693986442286823,0.719988067902571,0.));
#19551=DIRECTION('ref_axis',(-0.719988067902571,0.693986442286823,0.));
#19552=DIRECTION('',(0.,0.,1.));
#19553=DIRECTION('center_axis',(-0.994423866883654,0.105456972136322,0.));
#19554=DIRECTION('ref_axis',(-0.105456972136322,-0.994423866883654,0.));
#19555=DIRECTION('center_axis',(0.808467844782639,0.588540350318069,0.));
#19556=DIRECTION('ref_axis',(-0.588540350318069,0.808467844782639,0.));
#19557=DIRECTION('',(-0.588540350318069,0.808467844782638,0.));
#19558=DIRECTION('',(0.,0.,1.));
#19559=DIRECTION('center_axis',(-0.961003922853658,0.276534736081891,0.));
#19560=DIRECTION('ref_axis',(-0.276534736081891,-0.961003922853658,0.));
#19561=DIRECTION('',(-0.276534736081891,-0.961003922853658,0.));
#19562=DIRECTION('center_axis',(0.,0.,1.));
#19563=DIRECTION('ref_axis',(0.17364817766693,-0.984807753012208,0.));
#19564=DIRECTION('center_axis',(0.,0.,1.));
#19565=DIRECTION('ref_axis',(-1.83697019872103E-16,-1.,0.));
#19566=DIRECTION('',(-0.43921013200494,-0.898384360919202,0.));
#19567=DIRECTION('',(-0.43921013200494,0.898384360919202,0.));
#19568=DIRECTION('center_axis',(0.898384360919202,0.43921013200494,0.));
#19569=DIRECTION('ref_axis',(-0.43921013200494,0.898384360919202,0.));
#19570=DIRECTION('',(0.,0.,1.));
#19571=DIRECTION('center_axis',(-0.898384360919202,0.43921013200494,0.));
#19572=DIRECTION('ref_axis',(-0.43921013200494,-0.898384360919202,0.));
#19573=DIRECTION('center_axis',(0.961003922853658,0.276534736081891,0.));
#19574=DIRECTION('ref_axis',(-0.276534736081891,0.961003922853658,0.));
#19575=DIRECTION('',(-0.276534736081891,0.961003922853658,0.));
#19576=DIRECTION('',(0.,0.,1.));
#19577=DIRECTION('center_axis',(-0.808467844782638,0.58854035031807,0.));
#19578=DIRECTION('ref_axis',(-0.58854035031807,-0.808467844782638,0.));
#19579=DIRECTION('',(-0.588540350318069,-0.808467844782638,0.));
#19580=DIRECTION('center_axis',(0.,0.,1.));
#19581=DIRECTION('ref_axis',(-0.17364817766693,-0.984807753012208,0.));
#19582=DIRECTION('center_axis',(0.,0.,1.));
#19583=DIRECTION('ref_axis',(-0.342020143325669,-0.939692620785908,0.));
#19584=DIRECTION('',(-0.719988067902572,-0.693986442286823,0.));
#19585=DIRECTION('',(-0.105456972136321,0.994423866883654,0.));
#19586=DIRECTION('center_axis',(0.994423866883654,0.105456972136321,0.));
#19587=DIRECTION('ref_axis',(-0.105456972136321,0.994423866883654,0.));
#19588=DIRECTION('',(0.,0.,1.));
#19589=DIRECTION('center_axis',(-0.693986442286823,0.719988067902572,0.));
#19590=DIRECTION('ref_axis',(-0.719988067902572,-0.693986442286823,0.));
#19591=DIRECTION('center_axis',(0.997628744921147,-0.0688250485438069,0.));
#19592=DIRECTION('ref_axis',(0.0688250485438069,0.997628744921147,0.));
#19593=DIRECTION('',(0.0688250485438069,0.997628744921147,0.));
#19594=DIRECTION('',(0.,0.,1.));
#19595=DIRECTION('center_axis',(-0.558418612916207,0.829559312375396,0.));
#19596=DIRECTION('ref_axis',(-0.829559312375396,-0.558418612916207,0.));
#19597=DIRECTION('',(-0.829559312375396,-0.558418612916207,0.));
#19598=DIRECTION('center_axis',(0.,0.,1.));
#19599=DIRECTION('ref_axis',(-0.5,-0.866025403784438,0.));
#19600=DIRECTION('center_axis',(0.,0.,1.));
#19601=DIRECTION('ref_axis',(-0.642787609686539,-0.766044443118978,0.));
#19602=DIRECTION('',(-0.91392481691896,-0.405883516565584,0.));
#19603=DIRECTION('',(0.241015854951086,0.970521178368714,0.));
#19604=DIRECTION('center_axis',(0.970521178368714,-0.241015854951086,0.));
#19605=DIRECTION('ref_axis',(0.241015854951086,0.970521178368714,0.));
#19606=DIRECTION('',(0.,0.,1.));
#19607=DIRECTION('center_axis',(-0.405883516565584,0.91392481691896,0.));
#19608=DIRECTION('ref_axis',(-0.91392481691896,-0.405883516565584,0.));
#19609=DIRECTION('center_axis',(0.91392481691896,-0.405883516565585,0.));
#19610=DIRECTION('ref_axis',(0.405883516565585,0.91392481691896,0.));
#19611=DIRECTION('',(0.405883516565584,0.91392481691896,0.));
#19612=DIRECTION('',(0.,0.,1.));
#19613=DIRECTION('center_axis',(-0.241015854951086,0.970521178368714,0.));
#19614=DIRECTION('ref_axis',(-0.970521178368714,-0.241015854951086,0.));
#19615=DIRECTION('',(-0.970521178368714,-0.241015854951086,0.));
#19616=DIRECTION('center_axis',(0.,0.,1.));
#19617=DIRECTION('ref_axis',(-0.766044443118978,-0.642787609686539,0.));
#19618=DIRECTION('center_axis',(0.,0.,1.));
#19619=DIRECTION('ref_axis',(-0.866025403784439,-0.5,0.));
#19620=DIRECTION('',(-0.997628744921147,-0.0688250485438061,0.));
#19621=DIRECTION('',(0.558418612916207,0.829559312375396,0.));
#19622=DIRECTION('center_axis',(0.829559312375396,-0.558418612916207,0.));
#19623=DIRECTION('ref_axis',(0.558418612916207,0.829559312375396,0.));
#19624=DIRECTION('',(0.,0.,1.));
#19625=DIRECTION('center_axis',(-0.0688250485438061,0.997628744921147,0.));
#19626=DIRECTION('ref_axis',(-0.997628744921147,-0.0688250485438061,0.));
#19627=DIRECTION('center_axis',(0.719988067902572,-0.693986442286823,0.));
#19628=DIRECTION('ref_axis',(0.693986442286823,0.719988067902572,0.));
#19629=DIRECTION('',(0.693986442286823,0.719988067902572,0.));
#19630=DIRECTION('',(0.,0.,1.));
#19631=DIRECTION('center_axis',(0.105456972136322,0.994423866883654,0.));
#19632=DIRECTION('ref_axis',(-0.994423866883654,0.105456972136322,0.));
#19633=DIRECTION('',(-0.994423866883654,0.105456972136322,0.));
#19634=DIRECTION('center_axis',(0.,0.,1.));
#19635=DIRECTION('ref_axis',(-0.939692620785908,-0.342020143325669,0.));
#19636=DIRECTION('center_axis',(0.,0.,1.));
#19637=DIRECTION('ref_axis',(-0.984807753012208,-0.17364817766693,0.));
#19638=DIRECTION('',(-0.961003922853658,0.276534736081891,0.));
#19639=DIRECTION('',(0.808467844782638,0.588540350318069,0.));
#19640=DIRECTION('center_axis',(0.588540350318069,-0.808467844782638,0.));
#19641=DIRECTION('ref_axis',(0.808467844782639,0.588540350318069,0.));
#19642=DIRECTION('',(0.,0.,1.));
#19643=DIRECTION('center_axis',(0.276534736081891,0.961003922853658,0.));
#19644=DIRECTION('ref_axis',(-0.961003922853658,0.276534736081891,0.));
#19645=DIRECTION('center_axis',(0.43921013200494,-0.898384360919202,0.));
#19646=DIRECTION('ref_axis',(0.898384360919202,0.43921013200494,0.));
#19647=DIRECTION('',(0.898384360919202,0.43921013200494,0.));
#19648=DIRECTION('',(0.,0.,1.));
#19649=DIRECTION('center_axis',(0.43921013200494,0.898384360919202,0.));
#19650=DIRECTION('ref_axis',(-0.898384360919202,0.43921013200494,0.));
#19651=DIRECTION('',(-0.898384360919202,0.43921013200494,0.));
#19652=DIRECTION('center_axis',(0.,0.,1.));
#19653=DIRECTION('ref_axis',(-1.,1.22464679914735E-16,0.));
#19654=DIRECTION('center_axis',(0.,0.,1.));
#19655=DIRECTION('ref_axis',(-0.984807753012208,0.173648177666931,0.));
#19656=DIRECTION('',(-0.808467844782638,0.58854035031807,0.));
#19657=DIRECTION('',(0.961003922853658,0.276534736081891,0.));
#19658=DIRECTION('center_axis',(0.276534736081891,-0.961003922853658,0.));
#19659=DIRECTION('ref_axis',(0.961003922853658,0.276534736081891,0.));
#19660=DIRECTION('',(0.,0.,1.));
#19661=DIRECTION('center_axis',(0.58854035031807,0.808467844782638,0.));
#19662=DIRECTION('ref_axis',(-0.808467844782638,0.58854035031807,0.));
#19663=DIRECTION('center_axis',(0.105456972136322,-0.994423866883654,0.));
#19664=DIRECTION('ref_axis',(0.994423866883654,0.105456972136322,0.));
#19665=DIRECTION('',(0.994423866883654,0.105456972136322,0.));
#19666=DIRECTION('',(0.,0.,1.));
#19667=DIRECTION('center_axis',(0.719988067902572,0.693986442286823,0.));
#19668=DIRECTION('ref_axis',(-0.693986442286823,0.719988067902572,0.));
#19669=DIRECTION('',(-0.693986442286823,0.719988067902572,0.));
#19670=DIRECTION('center_axis',(0.,0.,1.));
#19671=DIRECTION('ref_axis',(-0.939692620785908,0.342020143325669,0.));
#19672=DIRECTION('center_axis',(0.,0.,1.));
#19673=DIRECTION('ref_axis',(-0.866025403784439,0.5,0.));
#19674=DIRECTION('',(-0.558418612916207,0.829559312375396,0.));
#19675=DIRECTION('',(0.997628744921147,-0.0688250485438063,0.));
#19676=DIRECTION('center_axis',(-0.0688250485438063,-0.997628744921147,
0.));
#19677=DIRECTION('ref_axis',(0.997628744921147,-0.0688250485438063,0.));
#19678=DIRECTION('',(0.,0.,1.));
#19679=DIRECTION('center_axis',(0.829559312375396,0.558418612916207,0.));
#19680=DIRECTION('ref_axis',(-0.558418612916207,0.829559312375396,0.));
#19681=DIRECTION('center_axis',(-0.241015854951086,-0.970521178368714,0.));
#19682=DIRECTION('ref_axis',(0.970521178368714,-0.241015854951086,0.));
#19683=DIRECTION('',(0.970521178368714,-0.241015854951086,0.));
#19684=DIRECTION('',(0.,0.,1.));
#19685=DIRECTION('center_axis',(0.91392481691896,0.405883516565584,0.));
#19686=DIRECTION('ref_axis',(-0.405883516565584,0.91392481691896,0.));
#19687=DIRECTION('',(-0.405883516565584,0.91392481691896,0.));
#19688=DIRECTION('center_axis',(0.,0.,1.));
#19689=DIRECTION('ref_axis',(-0.766044443118978,0.642787609686539,0.));
#19690=DIRECTION('center_axis',(0.,0.,1.));
#19691=DIRECTION('ref_axis',(-0.642787609686539,0.766044443118978,0.));
#19692=DIRECTION('',(-0.241015854951086,0.970521178368714,0.));
#19693=DIRECTION('',(0.91392481691896,-0.405883516565584,0.));
#19694=DIRECTION('center_axis',(-0.405883516565584,-0.91392481691896,0.));
#19695=DIRECTION('ref_axis',(0.91392481691896,-0.405883516565584,0.));
#19696=DIRECTION('',(0.,0.,1.));
#19697=DIRECTION('center_axis',(0.970521178368714,0.241015854951086,0.));
#19698=DIRECTION('ref_axis',(-0.241015854951086,0.970521178368714,0.));
#19699=DIRECTION('center_axis',(-0.558418612916207,-0.829559312375396,0.));
#19700=DIRECTION('ref_axis',(0.829559312375396,-0.558418612916207,0.));
#19701=DIRECTION('',(0.829559312375396,-0.558418612916207,0.));
#19702=DIRECTION('',(0.,0.,1.));
#19703=DIRECTION('center_axis',(0.997628744921147,0.0688250485438062,0.));
#19704=DIRECTION('ref_axis',(-0.0688250485438062,0.997628744921147,0.));
#19705=DIRECTION('',(-0.0688250485438062,0.997628744921147,0.));
#19706=DIRECTION('center_axis',(0.,0.,1.));
#19707=DIRECTION('ref_axis',(-0.5,0.866025403784439,0.));
#19708=DIRECTION('center_axis',(0.,0.,1.));
#19709=DIRECTION('ref_axis',(-0.342020143325669,0.939692620785908,0.));
#19710=DIRECTION('',(0.105456972136322,0.994423866883654,0.));
#19711=DIRECTION('',(0.719988067902572,-0.693986442286823,0.));
#19712=DIRECTION('center_axis',(-0.693986442286823,-0.719988067902572,0.));
#19713=DIRECTION('ref_axis',(0.719988067902572,-0.693986442286823,0.));
#19714=DIRECTION('',(0.,0.,1.));
#19715=DIRECTION('center_axis',(0.994423866883654,-0.105456972136322,0.));
#19716=DIRECTION('ref_axis',(0.105456972136322,0.994423866883654,0.));
#19717=DIRECTION('center_axis',(-0.808467844782638,-0.58854035031807,0.));
#19718=DIRECTION('ref_axis',(0.58854035031807,-0.808467844782638,0.));
#19719=DIRECTION('',(0.588540350318069,-0.808467844782638,0.));
#19720=DIRECTION('',(0.,0.,1.));
#19721=DIRECTION('center_axis',(0.961003922853658,-0.276534736081891,0.));
#19722=DIRECTION('ref_axis',(0.276534736081891,0.961003922853658,0.));
#19723=DIRECTION('',(0.276534736081891,0.961003922853658,0.));
#19724=DIRECTION('center_axis',(0.,0.,1.));
#19725=DIRECTION('ref_axis',(-0.17364817766693,0.984807753012208,0.));
#19726=DIRECTION('center_axis',(0.,0.,1.));
#19727=DIRECTION('ref_axis',(6.12323399573677E-17,1.,0.));
#19728=DIRECTION('',(0.43921013200494,0.898384360919202,0.));
#19729=DIRECTION('',(0.43921013200494,-0.898384360919202,0.));
#19730=DIRECTION('center_axis',(-0.898384360919202,-0.43921013200494,0.));
#19731=DIRECTION('ref_axis',(0.43921013200494,-0.898384360919202,0.));
#19732=DIRECTION('',(0.,0.,1.));
#19733=DIRECTION('center_axis',(0.898384360919202,-0.43921013200494,0.));
#19734=DIRECTION('ref_axis',(0.43921013200494,0.898384360919202,0.));
#19735=DIRECTION('center_axis',(-0.961003922853658,-0.276534736081891,0.));
#19736=DIRECTION('ref_axis',(0.276534736081891,-0.961003922853658,0.));
#19737=DIRECTION('',(0.276534736081891,-0.961003922853658,0.));
#19738=DIRECTION('',(0.,0.,1.));
#19739=DIRECTION('center_axis',(0.808467844782638,-0.58854035031807,0.));
#19740=DIRECTION('ref_axis',(0.58854035031807,0.808467844782638,0.));
#19741=DIRECTION('',(0.588540350318069,0.808467844782638,0.));
#19742=DIRECTION('center_axis',(0.,0.,1.));
#19743=DIRECTION('ref_axis',(0.17364817766693,0.984807753012208,0.));
#19744=DIRECTION('center_axis',(0.,0.,1.));
#19745=DIRECTION('ref_axis',(0.342020143325669,0.939692620785908,0.));
#19746=DIRECTION('',(0.719988067902572,0.693986442286823,0.));
#19747=DIRECTION('',(0.105456972136322,-0.994423866883654,0.));
#19748=DIRECTION('center_axis',(-0.994423866883654,-0.105456972136322,0.));
#19749=DIRECTION('ref_axis',(0.105456972136322,-0.994423866883654,0.));
#19750=DIRECTION('',(0.,0.,1.));
#19751=DIRECTION('center_axis',(0.693986442286823,-0.719988067902572,0.));
#19752=DIRECTION('ref_axis',(0.719988067902572,0.693986442286823,0.));
#19753=DIRECTION('center_axis',(-0.997628744921147,0.0688250485438065,0.));
#19754=DIRECTION('ref_axis',(-0.0688250485438065,-0.997628744921147,0.));
#19755=DIRECTION('',(-0.0688250485438065,-0.997628744921147,0.));
#19756=DIRECTION('',(0.,0.,1.));
#19757=DIRECTION('center_axis',(0.558418612916207,-0.829559312375396,0.));
#19758=DIRECTION('ref_axis',(0.829559312375396,0.558418612916207,0.));
#19759=DIRECTION('',(0.829559312375396,0.558418612916207,0.));
#19760=DIRECTION('center_axis',(0.,0.,1.));
#19761=DIRECTION('ref_axis',(0.5,0.866025403784439,0.));
#19762=DIRECTION('center_axis',(0.,0.,1.));
#19763=DIRECTION('ref_axis',(0.642787609686539,0.766044443118978,0.));
#19764=DIRECTION('',(0.91392481691896,0.405883516565584,0.));
#19765=DIRECTION('',(-0.241015854951086,-0.970521178368714,0.));
#19766=DIRECTION('center_axis',(-0.970521178368714,0.241015854951086,0.));
#19767=DIRECTION('ref_axis',(-0.241015854951086,-0.970521178368714,0.));
#19768=DIRECTION('',(0.,0.,1.));
#19769=DIRECTION('center_axis',(0.405883516565584,-0.91392481691896,0.));
#19770=DIRECTION('ref_axis',(0.91392481691896,0.405883516565584,0.));
#19771=DIRECTION('center_axis',(-0.91392481691896,0.405883516565585,0.));
#19772=DIRECTION('ref_axis',(-0.405883516565585,-0.91392481691896,0.));
#19773=DIRECTION('',(-0.405883516565584,-0.91392481691896,0.));
#19774=DIRECTION('',(0.,0.,1.));
#19775=DIRECTION('center_axis',(0.241015854951086,-0.970521178368714,0.));
#19776=DIRECTION('ref_axis',(0.970521178368714,0.241015854951086,0.));
#19777=DIRECTION('',(0.970521178368714,0.241015854951086,0.));
#19778=DIRECTION('center_axis',(0.,0.,1.));
#19779=DIRECTION('ref_axis',(0.766044443118978,0.642787609686539,0.));
#19780=DIRECTION('center_axis',(0.,0.,1.));
#19781=DIRECTION('ref_axis',(0.866025403784439,0.5,0.));
#19782=DIRECTION('',(0.997628744921147,0.0688250485438063,0.));
#19783=DIRECTION('',(-0.558418612916207,-0.829559312375396,0.));
#19784=DIRECTION('center_axis',(-0.829559312375396,0.558418612916207,0.));
#19785=DIRECTION('ref_axis',(-0.558418612916207,-0.829559312375396,0.));
#19786=DIRECTION('',(0.,0.,1.));
#19787=DIRECTION('center_axis',(0.0688250485438063,-0.997628744921147,0.));
#19788=DIRECTION('ref_axis',(0.997628744921147,0.0688250485438063,0.));
#19789=DIRECTION('center_axis',(-0.719988067902572,0.693986442286823,0.));
#19790=DIRECTION('ref_axis',(-0.693986442286823,-0.719988067902572,0.));
#19791=DIRECTION('',(-0.693986442286823,-0.719988067902572,0.));
#19792=DIRECTION('',(0.,0.,1.));
#19793=DIRECTION('center_axis',(-0.105456972136322,-0.994423866883654,0.));
#19794=DIRECTION('ref_axis',(0.994423866883654,-0.105456972136322,0.));
#19795=DIRECTION('',(0.994423866883654,-0.105456972136322,0.));
#19796=DIRECTION('center_axis',(0.,0.,1.));
#19797=DIRECTION('ref_axis',(0.939692620785908,0.342020143325669,0.));
#19798=DIRECTION('center_axis',(0.,0.,1.));
#19799=DIRECTION('ref_axis',(0.984807753012208,0.17364817766693,0.));
#19800=DIRECTION('',(0.961003922853658,-0.276534736081891,0.));
#19801=DIRECTION('',(-0.808467844782638,-0.588540350318069,0.));
#19802=DIRECTION('center_axis',(-0.58854035031807,0.808467844782638,0.));
#19803=DIRECTION('ref_axis',(-0.808467844782638,-0.58854035031807,0.));
#19804=DIRECTION('',(0.,0.,1.));
#19805=DIRECTION('center_axis',(-0.276534736081891,-0.961003922853658,0.));
#19806=DIRECTION('ref_axis',(0.961003922853658,-0.276534736081891,0.));
#19807=DIRECTION('center_axis',(-0.43921013200494,0.898384360919202,0.));
#19808=DIRECTION('ref_axis',(-0.898384360919202,-0.43921013200494,0.));
#19809=DIRECTION('',(-0.898384360919202,-0.43921013200494,0.));
#19810=DIRECTION('',(0.,0.,1.));
#19811=DIRECTION('center_axis',(-0.43921013200494,-0.898384360919202,0.));
#19812=DIRECTION('ref_axis',(0.898384360919202,-0.43921013200494,0.));
#19813=DIRECTION('',(0.898384360919202,-0.43921013200494,0.));
#19814=DIRECTION('center_axis',(0.,0.,1.));
#19815=DIRECTION('ref_axis',(1.,0.,0.));
#19816=DIRECTION('center_axis',(0.,0.,1.));
#19817=DIRECTION('ref_axis',(1.,0.,0.));
#19818=DIRECTION('center_axis',(0.,-1.,0.));
#19819=DIRECTION('ref_axis',(-1.,0.,0.));
#19820=DIRECTION('center_axis',(0.,0.,1.));
#19821=DIRECTION('ref_axis',(1.,0.,0.));
#19822=DIRECTION('center_axis',(0.,0.,1.));
#19823=DIRECTION('ref_axis',(1.,0.,0.));
#19824=DIRECTION('center_axis',(0.,0.,-1.));
#19825=DIRECTION('ref_axis',(1.,0.,0.));
#19826=DIRECTION('center_axis',(0.,0.,1.));
#19827=DIRECTION('ref_axis',(1.,0.,0.));
#19828=DIRECTION('center_axis',(0.,0.,1.));
#19829=DIRECTION('ref_axis',(1.,0.,0.));
#19830=DIRECTION('center_axis',(0.,0.,1.));
#19831=DIRECTION('ref_axis',(1.,0.,0.));
#19832=DIRECTION('center_axis',(0.,0.,1.));
#19833=DIRECTION('ref_axis',(1.,0.,0.));
#19834=DIRECTION('center_axis',(0.,0.,1.));
#19835=DIRECTION('ref_axis',(1.,0.,0.));
#19836=DIRECTION('center_axis',(0.,0.,1.));
#19837=DIRECTION('ref_axis',(1.,0.,0.));
#19838=DIRECTION('',(-0.707106781186551,8.65956056235498E-17,-0.707106781186544));
#19839=DIRECTION('center_axis',(0.,0.,1.));
#19840=DIRECTION('ref_axis',(1.,0.,0.));
#19841=DIRECTION('',(0.,0.,-1.));
#19842=DIRECTION('',(0.,0.,1.));
#19843=DIRECTION('center_axis',(0.,0.,-1.));
#19844=DIRECTION('ref_axis',(1.,0.,0.));
#19845=DIRECTION('center_axis',(0.,0.,1.));
#19846=DIRECTION('ref_axis',(1.,0.,0.));
#19847=DIRECTION('',(0.,0.,-1.));
#19848=DIRECTION('',(0.,0.,1.));
#19849=DIRECTION('center_axis',(0.,0.,-1.));
#19850=DIRECTION('ref_axis',(1.,0.,0.));
#19851=DIRECTION('center_axis',(0.,0.,1.));
#19852=DIRECTION('ref_axis',(1.,0.,0.));
#19853=DIRECTION('',(0.,0.,1.));
#19854=DIRECTION('center_axis',(0.,0.,-1.));
#19855=DIRECTION('ref_axis',(1.,0.,0.));
#19856=DIRECTION('',(0.,0.,-1.));
#19857=DIRECTION('center_axis',(0.,0.,1.));
#19858=DIRECTION('ref_axis',(1.,0.,0.));
#19859=DIRECTION('',(0.,0.,-1.));
#19860=DIRECTION('',(0.,0.,1.));
#19861=DIRECTION('center_axis',(0.,0.,-1.));
#19862=DIRECTION('ref_axis',(1.,0.,0.));
#19863=DIRECTION('center_axis',(0.,0.,1.));
#19864=DIRECTION('ref_axis',(1.,0.,0.));
#19865=DIRECTION('',(0.,0.,1.));
#19866=DIRECTION('center_axis',(0.,0.,-1.));
#19867=DIRECTION('ref_axis',(1.,0.,0.));
#19868=DIRECTION('',(0.,0.,-1.));
#19869=DIRECTION('center_axis',(0.,0.,1.));
#19870=DIRECTION('ref_axis',(1.,0.,0.));
#19871=DIRECTION('',(0.,0.,1.));
#19872=DIRECTION('center_axis',(0.,0.,-1.));
#19873=DIRECTION('ref_axis',(1.,0.,0.));
#19874=DIRECTION('',(0.,0.,-1.));
#19875=DIRECTION('center_axis',(0.,1.,0.));
#19876=DIRECTION('ref_axis',(-1.,0.,0.));
#19877=DIRECTION('',(-1.,0.,0.));
#19878=DIRECTION('',(0.,0.,1.));
#19879=DIRECTION('',(-1.,0.,0.));
#19880=DIRECTION('',(0.,0.,1.));
#19881=DIRECTION('center_axis',(0.866025403784438,0.500000000000001,0.));
#19882=DIRECTION('ref_axis',(-0.500000000000001,0.866025403784438,0.));
#19883=DIRECTION('',(-0.500000000000001,0.866025403784438,0.));
#19884=DIRECTION('',(0.,0.,1.));
#19885=DIRECTION('',(-0.500000000000001,0.866025403784438,0.));
#19886=DIRECTION('center_axis',(0.866025403784438,-0.500000000000001,0.));
#19887=DIRECTION('ref_axis',(0.500000000000001,0.866025403784438,0.));
#19888=DIRECTION('',(0.500000000000001,0.866025403784438,0.));
#19889=DIRECTION('',(0.,0.,1.));
#19890=DIRECTION('',(0.500000000000001,0.866025403784438,0.));
#19891=DIRECTION('center_axis',(0.,0.,1.));
#19892=DIRECTION('ref_axis',(1.,0.,0.));
#19893=DIRECTION('center_axis',(0.,0.,1.));
#19894=DIRECTION('ref_axis',(1.,0.,0.));
#19895=DIRECTION('center_axis',(0.,0.,1.));
#19896=DIRECTION('ref_axis',(1.,0.,0.));
#19897=DIRECTION('',(1.,0.,0.));
#19898=DIRECTION('center_axis',(0.,0.,1.));
#19899=DIRECTION('ref_axis',(1.,0.,0.));
#19900=DIRECTION('center_axis',(0.,0.,1.));
#19901=DIRECTION('ref_axis',(1.,0.,0.));
#19902=DIRECTION('',(0.500000000000001,-0.866025403784438,0.));
#19903=DIRECTION('center_axis',(0.,0.,1.));
#19904=DIRECTION('ref_axis',(1.,0.,0.));
#19905=DIRECTION('',(-0.500000000000001,-0.866025403784438,0.));
#19906=DIRECTION('center_axis',(0.,0.,-1.));
#19907=DIRECTION('ref_axis',(-1.,0.,0.));
#19908=DIRECTION('',(1.,0.,0.));
#19909=DIRECTION('center_axis',(0.,0.,1.));
#19910=DIRECTION('ref_axis',(1.,0.,0.));
#19911=DIRECTION('center_axis',(0.,0.,-1.));
#19912=DIRECTION('ref_axis',(-1.,0.,0.));
#19913=DIRECTION('center_axis',(0.,0.,1.));
#19914=DIRECTION('ref_axis',(1.,0.,0.));
#19915=DIRECTION('center_axis',(0.,0.,-1.));
#19916=DIRECTION('ref_axis',(-1.,0.,0.));
#19917=DIRECTION('center_axis',(0.,0.,1.));
#19918=DIRECTION('ref_axis',(1.,0.,0.));
#19919=DIRECTION('center_axis',(0.,0.,-1.));
#19920=DIRECTION('ref_axis',(-1.,0.,0.));
#19921=DIRECTION('center_axis',(0.,0.,1.));
#19922=DIRECTION('ref_axis',(1.,0.,0.));
#19923=DIRECTION('center_axis',(0.,0.,-1.));
#19924=DIRECTION('ref_axis',(-1.,0.,0.));
#19925=DIRECTION('',(-0.500000000000001,-0.866025403784438,0.));
#19926=DIRECTION('center_axis',(0.,0.,1.));
#19927=DIRECTION('ref_axis',(1.,0.,0.));
#19928=DIRECTION('center_axis',(0.,0.,-1.));
#19929=DIRECTION('ref_axis',(-1.,0.,0.));
#19930=DIRECTION('',(0.500000000000001,-0.866025403784438,0.));
#19931=DIRECTION('center_axis',(0.,0.,1.));
#19932=DIRECTION('ref_axis',(1.,0.,0.));
#19933=DIRECTION('center_axis',(0.,0.,-1.));
#19934=DIRECTION('ref_axis',(1.,0.,0.));
#19935=DIRECTION('',(-0.857167300702115,1.04972719113862E-16,-0.515038074910049));
#19936=DIRECTION('center_axis',(0.,-1.,0.));
#19937=DIRECTION('ref_axis',(1.,0.,0.));
#19938=DIRECTION('',(0.,0.,1.));
#19939=DIRECTION('center_axis',(-0.866025403784438,-0.500000000000001,0.));
#19940=DIRECTION('ref_axis',(0.500000000000001,-0.866025403784438,0.));
#19941=DIRECTION('',(0.,0.,1.));
#19942=DIRECTION('center_axis',(-0.866025403784438,0.500000000000001,0.));
#19943=DIRECTION('ref_axis',(-0.500000000000001,-0.866025403784438,0.));
#23034=CARTESIAN_POINT('',(0.,0.,0.));
#23035=CARTESIAN_POINT('Origin',(55.,21.,6.22095488139522));
#23036=CARTESIAN_POINT('',(55.1644483595783,22.9879598334805,8.16850613376992));
#23037=CARTESIAN_POINT('',(55.1644483516311,22.987959834138,8.01046478735112));
#23038=CARTESIAN_POINT('',(55.1644483516311,22.987959834138,6.22095488139522));
#23039=CARTESIAN_POINT('',(53.8619125385576,19.3617739799992,7.7));
#23040=CARTESIAN_POINT('Ctrl Pts',(55.1644483595783,22.9879598334805,8.16850613376992));
#23041=CARTESIAN_POINT('Ctrl Pts',(55.1739112702763,22.9871770409337,8.16795475044047));
#23042=CARTESIAN_POINT('Ctrl Pts',(55.1833696088008,22.9863265975055,8.16740313133717));
#23043=CARTESIAN_POINT('Ctrl Pts',(55.3237705246029,22.9726908763678,8.1592036975142));
#23044=CARTESIAN_POINT('Ctrl Pts',(55.4531201253634,22.9470521773363,8.15147670177632));
#23045=CARTESIAN_POINT('Ctrl Pts',(55.5938213859521,22.9043748946883,8.14234975210098));
#23046=CARTESIAN_POINT('Ctrl Pts',(55.6085936065288,22.8997056032264,8.14138272182667));
#23047=CARTESIAN_POINT('Ctrl Pts',(55.6324693111573,22.8918517677942,8.139804738193));
#23048=CARTESIAN_POINT('Ctrl Pts',(55.6416068997965,22.888772384845,8.13919722286266));
#23049=CARTESIAN_POINT('Ctrl Pts',(55.6578308337942,22.8831735755404,8.1381119927678));
#23050=CARTESIAN_POINT('Ctrl Pts',(55.6649259800132,22.8806800791425,8.13763514035216));
#23051=CARTESIAN_POINT('Ctrl Pts',(55.6798501285734,22.8753401715625,8.13662727724571));
#23052=CARTESIAN_POINT('Ctrl Pts',(55.6876757231185,22.8724847269786,8.13609597461454));
#23053=CARTESIAN_POINT('Ctrl Pts',(55.7083667015217,22.8647876918322,8.13468359012937));
#23054=CARTESIAN_POINT('Ctrl Pts',(55.7212001366586,22.8598620558134,8.13379972514799));
#23055=CARTESIAN_POINT('Ctrl Pts',(55.7820172652065,22.8357955597389,8.12957288800204));
#23056=CARTESIAN_POINT('Ctrl Pts',(55.8292925494817,22.8149295845626,8.12617250592043));
#23057=CARTESIAN_POINT('Ctrl Pts',(56.0330419639254,22.7153769234046,8.11099466761143));
#23058=CARTESIAN_POINT('Ctrl Pts',(56.1795621610039,22.6181191419544,8.09859647551919));
#23059=CARTESIAN_POINT('Ctrl Pts',(56.3221210645677,22.4937279297629,8.08555728451026));
#23060=CARTESIAN_POINT('Ctrl Pts',(56.3326694864003,22.4843245235456,8.08458654169387));
#23061=CARTESIAN_POINT('Ctrl Pts',(56.3804326360051,22.4408263606657,8.08016670917425));
#23062=CARTESIAN_POINT('Ctrl Pts',(56.416448451004,22.4054357351974,8.07676506186341));
#23063=CARTESIAN_POINT('Ctrl Pts',(56.4570253807462,22.362416797938,8.0728883373071));
#23064=CARTESIAN_POINT('Ctrl Pts',(56.462923946461,22.3560811276617,8.0723236423558));
#23065=CARTESIAN_POINT('Ctrl Pts',(56.4724145707644,22.3457532199429,8.07141348893154));
#23066=CARTESIAN_POINT('Ctrl Pts',(56.4760320040888,22.3417846033275,8.07106619941156));
#23067=CARTESIAN_POINT('Ctrl Pts',(56.4824368498612,22.3347007237273,8.07045071087391));
#23068=CARTESIAN_POINT('Ctrl Pts',(56.4852305607753,22.331591235476,8.07018204132472));
#23069=CARTESIAN_POINT('Ctrl Pts',(56.4912384529693,22.3248618314058,8.06960385814169));
#23070=CARTESIAN_POINT('Ctrl Pts',(56.4944492435359,22.3212389850583,8.06929459705603));
#23071=CARTESIAN_POINT('Ctrl Pts',(56.5034042461198,22.3110603373111,8.06843119675549));
#23072=CARTESIAN_POINT('Ctrl Pts',(56.5091188088655,22.3044784255482,8.06787922427727));
#23073=CARTESIAN_POINT('Ctrl Pts',(56.5431075755179,22.2648085964654,8.06458868855021));
#23074=CARTESIAN_POINT('Ctrl Pts',(56.5703381863521,22.2308372769387,8.06192074409987));
#23075=CARTESIAN_POINT('Ctrl Pts',(56.7338394295454,22.0125934054582,8.04550169557243));
#23076=CARTESIAN_POINT('Ctrl Pts',(56.8386154691083,21.8068819901909,8.03292315964913));
#23077=CARTESIAN_POINT('Ctrl Pts',(56.914070568179,21.5622110722724,8.01720752420272));
#23078=CARTESIAN_POINT('Ctrl Pts',(56.9214590319891,21.5364163595988,8.01554525244227));
#23079=CARTESIAN_POINT('Ctrl Pts',(56.9311627754301,21.4997608253042,8.01317197072088));
#23080=CARTESIAN_POINT('Ctrl Pts',(56.9339113127624,21.4890169466225,8.01247502441956));
#23081=CARTESIAN_POINT('Ctrl Pts',(56.9382344688724,21.4715112919375,8.01133706496191));
#23082=CARTESIAN_POINT('Ctrl Pts',(56.9398636507752,21.4647631323103,8.01089782654406));
#23083=CARTESIAN_POINT('Ctrl Pts',(56.9432045045168,21.4506014921009,8.00997478172884));
#23084=CARTESIAN_POINT('Ctrl Pts',(56.9449090490337,21.4431864612008,8.00949075318005));
#23085=CARTESIAN_POINT('Ctrl Pts',(56.948874412525,21.4254729776759,8.00833266945935));
#23086=CARTESIAN_POINT('Ctrl Pts',(56.9510960636413,21.4151660798481,8.00765736543105));
#23087=CARTESIAN_POINT('Ctrl Pts',(56.9583849172293,21.3799996627178,8.0053480608139));
#23088=CARTESIAN_POINT('Ctrl Pts',(56.9630593468725,21.3550621484496,8.00370157877714));
#23089=CARTESIAN_POINT('Ctrl Pts',(56.973140202337,21.2949741626493,7.99971130837033));
#23090=CARTESIAN_POINT('Ctrl Pts',(56.9780845687087,21.2597560258546,7.99735372741819));
#23091=CARTESIAN_POINT('Ctrl Pts',(57.0041004668181,21.0299892098894,7.98184970289821));
#23092=CARTESIAN_POINT('Ctrl Pts',(56.9973847445597,20.833415029745,7.96786928123027));
#23093=CARTESIAN_POINT('Ctrl Pts',(56.954586373688,20.5995026971139,7.95168749153061));
#23094=CARTESIAN_POINT('Ctrl Pts',(56.9456821482064,20.5582675526637,7.94885899209389));
#23095=CARTESIAN_POINT('Ctrl Pts',(56.9334936132035,20.5093910231311,7.94555921473854));
#23096=CARTESIAN_POINT('Ctrl Pts',(56.9314616967622,20.5014516673566,7.94502489923333));
#23097=CARTESIAN_POINT('Ctrl Pts',(56.9280566843323,20.4884805147866,7.9441549701788));
#23098=CARTESIAN_POINT('Ctrl Pts',(56.9267127048315,20.4834412750703,7.94381775601036));
#23099=CARTESIAN_POINT('Ctrl Pts',(56.9242574603283,20.4743782601909,7.94321270415758));
#23100=CARTESIAN_POINT('Ctrl Pts',(56.9231533304931,20.4703527069196,7.94294446972559));
#23101=CARTESIAN_POINT('Ctrl Pts',(56.9207027059227,20.4615266634482,7.94235747818033));
#23102=CARTESIAN_POINT('Ctrl Pts',(56.9193508503805,20.456727754098,7.94203903516486));
#23103=CARTESIAN_POINT('Ctrl Pts',(56.9154386730893,20.4430369206054,7.94113246439344));
#23104=CARTESIAN_POINT('Ctrl Pts',(56.9128344135364,20.43415753392,7.94054680931333));
#23105=CARTESIAN_POINT('Ctrl Pts',(56.8947940804951,20.3741960626433,7.93660563219028));
#23106=CARTESIAN_POINT('Ctrl Pts',(56.8773738696665,20.3237281313764,7.93335567538186));
#23107=CARTESIAN_POINT('Ctrl Pts',(56.7931413458539,20.1081593162929,7.91952579157411));
#23108=CARTESIAN_POINT('Ctrl Pts',(56.7064177778546,19.9517243446332,7.90955307986865));
#23109=CARTESIAN_POINT('Ctrl Pts',(56.564692136171,19.7613405832537,7.89534959861422));
#23110=CARTESIAN_POINT('Ctrl Pts',(56.5272122204425,19.7154142871462,7.89174323958466));
#23111=CARTESIAN_POINT('Ctrl Pts',(56.4778621090287,19.6601599609527,7.88713066327911));
#23112=CARTESIAN_POINT('Ctrl Pts',(56.467854701384,19.6492038271897,7.88620186051999));
#23113=CARTESIAN_POINT('Ctrl Pts',(56.4518053374027,19.6320219079677,7.88472198348949));
#23114=CARTESIAN_POINT('Ctrl Pts',(56.4458432700389,19.6257219958655,7.88417429990159));
#23115=CARTESIAN_POINT('Ctrl Pts',(56.4346491001832,19.6140469757009,7.88314969914366));
#23116=CARTESIAN_POINT('Ctrl Pts',(56.4294273823341,19.608662089085,7.88267323428618));
#23117=CARTESIAN_POINT('Ctrl Pts',(56.4177412857351,19.5967460486405,7.8816101074328));
#23118=CARTESIAN_POINT('Ctrl Pts',(56.4112619283098,19.5902298874123,7.88102279686199));
#23119=CARTESIAN_POINT('Ctrl Pts',(56.3921948510716,19.5713176811365,7.87930054058841));
#23120=CARTESIAN_POINT('Ctrl Pts',(56.3794874573028,19.5590440695089,7.8781603180321));
#23121=CARTESIAN_POINT('Ctrl Pts',(56.3503498330901,19.5316397885375,7.87556210552738));
#23122=CARTESIAN_POINT('Ctrl Pts',(56.3338253477606,19.5166132473141,7.8740999487099));
#23123=CARTESIAN_POINT('Ctrl Pts',(56.2787795574664,19.4682208556013,7.86926488891193));
#23124=CARTESIAN_POINT('Ctrl Pts',(56.2392341076601,19.4360554299076,7.86584641114681));
#23125=CARTESIAN_POINT('Ctrl Pts',(56.0973780387822,19.3294334807549,7.85377940760683));
#23126=CARTESIAN_POINT('Ctrl Pts',(55.989256610758,19.263222041386,7.84489643527489));
#23127=CARTESIAN_POINT('Ctrl Pts',(55.8022674540353,19.171870617062,7.83046817173561));
#23128=CARTESIAN_POINT('Ctrl Pts',(55.7267881096822,19.1405720628331,7.82487654362709));
#23129=CARTESIAN_POINT('Ctrl Pts',(55.6398027104851,19.1106119189392,7.81883720863747));
#23130=CARTESIAN_POINT('Ctrl Pts',(55.6299839383764,19.1073153782186,7.81816119356792));
#23131=CARTESIAN_POINT('Ctrl Pts',(55.6151402886258,19.1024601042568,7.81714824743538));
#23132=CARTESIAN_POINT('Ctrl Pts',(55.6101343707833,19.1008445872599,7.81680817867411));
#23133=CARTESIAN_POINT('Ctrl Pts',(55.6011501264652,19.097984368332,7.81620067919868));
#23134=CARTESIAN_POINT('Ctrl Pts',(55.5971743053158,19.0967323395754,7.81593283807526));
#23135=CARTESIAN_POINT('Ctrl Pts',(55.593161552592,19.0954824925416,7.81566350183841));
#23136=CARTESIAN_POINT('Ctrl Pts',(55.5931286308482,19.095472239384,7.81566129219574));
#23137=CARTESIAN_POINT('Ctrl Pts',(55.5930639609698,19.0954521004174,7.81565695181235));
#23138=CARTESIAN_POINT('Ctrl Pts',(55.5930322125785,19.0954422144629,7.81565482104972));
#23139=CARTESIAN_POINT('Ctrl Pts',(55.5929698361398,19.0954227931225,7.81565063483763));
#23140=CARTESIAN_POINT('Ctrl Pts',(55.5929392083847,19.0954132577672,7.81564857940348));
#23141=CARTESIAN_POINT('Ctrl Pts',(55.5928790246036,19.0953945223109,7.81564454057301));
#23142=CARTESIAN_POINT('Ctrl Pts',(55.5928494683373,19.0953853220795,7.81564255715656));
#23143=CARTESIAN_POINT('Ctrl Pts',(55.5927913806998,19.0953672421275,7.81563865920682));
#23144=CARTESIAN_POINT('Ctrl Pts',(55.592762849287,19.0953583623426,7.81563674466705));
#23145=CARTESIAN_POINT('Ctrl Pts',(55.5927067670439,19.0953409093402,7.81563298148622));
#23146=CARTESIAN_POINT('Ctrl Pts',(55.5926792163658,19.0953323361225,7.81563113285198));
#23147=CARTESIAN_POINT('Ctrl Pts',(55.5926250538063,19.0953154831107,7.81562749866834));
#23148=CARTESIAN_POINT('Ctrl Pts',(55.5925984421096,19.0953072033301,7.81562571312819));
#23149=CARTESIAN_POINT('Ctrl Pts',(55.5925461183382,19.095290924874,7.81562220249494));
#23150=CARTESIAN_POINT('Ctrl Pts',(55.5925204062322,19.0952829261479,7.81562047739684));
#23151=CARTESIAN_POINT('Ctrl Pts',(55.592469844534,19.0952671981364,7.81561708514935));
#23152=CARTESIAN_POINT('Ctrl Pts',(55.5924449948286,19.095259468778,7.81561541798968));
#23153=CARTESIAN_POINT('Ctrl Pts',(55.5923961217554,19.0952442681377,7.81561213918404));
#23154=CARTESIAN_POINT('Ctrl Pts',(55.5923720986674,19.095236796908,7.81561052755435));
#23155=CARTESIAN_POINT('Ctrl Pts',(55.5923248464771,19.0952221023601,7.81560735763085));
#23156=CARTESIAN_POINT('Ctrl Pts',(55.59230161689,19.0952148788587,7.81560579930222));
#23157=CARTESIAN_POINT('Ctrl Pts',(55.5922559190593,19.0952006695211,7.81560273378424));
#23158=CARTESIAN_POINT('Ctrl Pts',(55.5922334509298,19.0951936836903,7.8156012266004));
#23159=CARTESIAN_POINT('Ctrl Pts',(55.5921892456743,19.0951799401713,7.81559826133038));
#23160=CARTESIAN_POINT('Ctrl Pts',(55.5921675087154,19.0951731825071,7.81559680325341));
#23161=CARTESIAN_POINT('Ctrl Pts',(55.5921199766948,19.0951584064735,7.81559361495279));
#23162=CARTESIAN_POINT('Ctrl Pts',(55.592094181714,19.0951503882957,7.81559188474645));
#23163=CARTESIAN_POINT('Ctrl Pts',(55.5920427738835,19.0951344096993,7.815588436632));
#23164=CARTESIAN_POINT('Ctrl Pts',(55.5920171608995,19.0951264492309,7.81558671871432));
#23165=CARTESIAN_POINT('Ctrl Pts',(55.5919661138578,19.095110585033,7.81558329496049));
#23166=CARTESIAN_POINT('Ctrl Pts',(55.5919406797052,19.0951026812661,7.81558158911742));
#23167=CARTESIAN_POINT('Ctrl Pts',(55.5918899863674,19.0950869292176,7.8155781892456));
#23168=CARTESIAN_POINT('Ctrl Pts',(55.5918647275076,19.0950790810294,7.81557649523814));
#23169=CARTESIAN_POINT('Ctrl Pts',(55.59181438236,19.0950634393708,7.81557311887522));
#23170=CARTESIAN_POINT('Ctrl Pts',(55.5917892958867,19.0950556458353,7.81557143650681));
#23171=CARTESIAN_POINT('Ctrl Pts',(55.5917392920433,19.0950401123822,7.81556808318776));
#23172=CARTESIAN_POINT('Ctrl Pts',(55.5917143747504,19.0950323724812,7.81556641224178));
#23173=CARTESIAN_POINT('Ctrl Pts',(55.5868173968984,19.0935113605995,7.8152380299307));
#23174=CARTESIAN_POINT('Ctrl Pts',(55.581939485181,19.0920167646392,7.81491238772519));
#23175=CARTESIAN_POINT('Ctrl Pts',(55.5676795705694,19.087707289372,7.81396453357938));
#23176=CARTESIAN_POINT('Ctrl Pts',(55.5582823467525,19.0849427328924,7.8133450925289));
#23177=CARTESIAN_POINT('Ctrl Pts',(55.4871434054314,19.0645826143466,7.80869225079019));
#23178=CARTESIAN_POINT('Ctrl Pts',(55.4245982557927,19.0499058409691,7.80480788208925));
#23179=CARTESIAN_POINT('Ctrl Pts',(55.2234155882325,19.0128380098621,7.79265332231242));
#23180=CARTESIAN_POINT('Ctrl Pts',(55.0830832774369,19.0020442739689,7.78465341362658));
#23181=CARTESIAN_POINT('Ctrl Pts',(54.8684453297137,19.0082041953005,7.77190082410308));
#23182=CARTESIAN_POINT('Ctrl Pts',(54.7942994120393,19.0144918453275,7.76740648100607));
#23183=CARTESIAN_POINT('Ctrl Pts',(54.7063103746654,19.0269352108482,7.76188072368881));
#23184=CARTESIAN_POINT('Ctrl Pts',(54.6919609369275,19.0291245151652,7.76097351206504));
#23185=CARTESIAN_POINT('Ctrl Pts',(54.6683533421166,19.0329904541369,7.7594703781756));
#23186=CARTESIAN_POINT('Ctrl Pts',(54.6590807275695,19.0345763550609,7.75887727161705));
#23187=CARTESIAN_POINT('Ctrl Pts',(54.6423571214046,19.03755851135,7.7578025333055));
#23188=CARTESIAN_POINT('Ctrl Pts',(54.6349021715328,19.0389317711813,7.75732162766313));
#23189=CARTESIAN_POINT('Ctrl Pts',(54.6189487297594,19.0419646404841,7.75628852211697));
#23190=CARTESIAN_POINT('Ctrl Pts',(54.6104528786401,19.0436371563374,7.75573592648535));
#23191=CARTESIAN_POINT('Ctrl Pts',(54.587330318173,19.0483457140913,7.75422520699252));
#23192=CARTESIAN_POINT('Ctrl Pts',(54.5727266259799,19.0514907847362,7.75326367494978));
#23193=CARTESIAN_POINT('Ctrl Pts',(54.4937166405304,19.0694374055787,7.74802016063897));
#23194=CARTESIAN_POINT('Ctrl Pts',(54.4300474570642,19.0872670825043,7.74364307411907));
#23195=CARTESIAN_POINT('Ctrl Pts',(54.1876332328554,19.1683308247533,7.72637366107652));
#23196=CARTESIAN_POINT('Ctrl Pts',(54.0174481366244,19.2537222754074,7.7128318167165));
#23197=CARTESIAN_POINT('Ctrl Pts',(53.8619125385576,19.3617739799992,7.7));
#23198=CARTESIAN_POINT('',(56.1603489846691,19.3774656255483,7.7));
#23199=CARTESIAN_POINT('Origin',(55.,21.,7.7));
#23200=CARTESIAN_POINT('Ctrl Pts',(56.1603489846691,19.3774656255483,7.7));
#23201=CARTESIAN_POINT('Ctrl Pts',(56.2184119355306,19.4189891132105,7.70455633151969));
#23202=CARTESIAN_POINT('Ctrl Pts',(56.2742878120524,19.4636645528829,7.70911266303938));
#23203=CARTESIAN_POINT('Ctrl Pts',(56.327631526034,19.5112347083638,7.71366899455907));
#23204=CARTESIAN_POINT('Ctrl Pts',(56.3829325283937,19.5605503087251,7.71839250706531));
#23205=CARTESIAN_POINT('Ctrl Pts',(56.4355115089017,19.6129768999016,7.72311601957156));
#23206=CARTESIAN_POINT('Ctrl Pts',(56.4850212649274,19.6681819173726,7.72783953207781));
#23207=CARTESIAN_POINT('Ctrl Pts',(56.5327427796166,19.7213929865362,7.73239243618289));
#23208=CARTESIAN_POINT('Ctrl Pts',(56.5776126865276,19.777184823213,7.73694534028798));
#23209=CARTESIAN_POINT('Ctrl Pts',(56.6193586935831,19.8352232042074,7.74149824439307));
#23210=CARTESIAN_POINT('Ctrl Pts',(56.6611051744409,19.8932622439168,7.746051200172));
#23211=CARTESIAN_POINT('Ctrl Pts',(56.6997274177751,19.9535475074006,7.75060415595094));
#23212=CARTESIAN_POINT('Ctrl Pts',(56.7349954777785,20.0157143429938,7.75515711172987));
#23213=CARTESIAN_POINT('Ctrl Pts',(56.7702734473569,20.0778986461461,7.75971134679258));
#23214=CARTESIAN_POINT('Ctrl Pts',(56.8021951346799,20.141965174434,7.76426558185529));
#23215=CARTESIAN_POINT('Ctrl Pts',(56.8305763917255,20.207524362168,7.768819816918));
#23216=CARTESIAN_POINT('Ctrl Pts',(56.8589732786453,20.2731196540764,7.77337656004866));
#23217=CARTESIAN_POINT('Ctrl Pts',(56.8838256779872,20.3402088200512,7.77793330317931));
#23218=CARTESIAN_POINT('Ctrl Pts',(56.9049979603927,20.4083832884379,7.78249004630996));
#23219=CARTESIAN_POINT('Ctrl Pts',(56.9262029963242,20.4766632227434,7.78705383872332));
#23220=CARTESIAN_POINT('Ctrl Pts',(56.9437164171219,20.5460313730339,7.79161763113668));
#23221=CARTESIAN_POINT('Ctrl Pts',(56.9574528908856,20.6160654450776,7.79618142355004));
#23222=CARTESIAN_POINT('Ctrl Pts',(56.9712016619737,20.6861622138298,7.8007493016142));
#23223=CARTESIAN_POINT('Ctrl Pts',(56.9811666872574,20.7569256394431,7.80531717967836));
#23224=CARTESIAN_POINT('Ctrl Pts',(56.9873144028289,20.8279272630282,7.80988505774252));
#23225=CARTESIAN_POINT('Ctrl Pts',(56.9934735122458,20.8990604772048,7.81446140166627));
#23226=CARTESIAN_POINT('Ctrl Pts',(56.9958011727957,20.9704323143018,7.81903774559003));
#23227=CARTESIAN_POINT('Ctrl Pts',(56.9943158867061,21.041613778149,7.82361408951378));
#23228=CARTESIAN_POINT('Ctrl Pts',(56.9939459773054,21.0593414690047,7.82475382457885));
#23229=CARTESIAN_POINT('Ctrl Pts',(56.9933398192831,21.077057379685,7.82589355964391));
#23230=CARTESIAN_POINT('Ctrl Pts',(56.992498196117,21.0947549522225,7.82703329470898));
#23231=CARTESIAN_POINT('Ctrl Pts',(56.9892396630441,21.1632750782667,7.83144603493929));
#23232=CARTESIAN_POINT('Ctrl Pts',(56.9824346045893,21.2317892992464,7.83585877516959));
#23233=CARTESIAN_POINT('Ctrl Pts',(56.9720776952813,21.2998951921485,7.8402715153999));
#23234=CARTESIAN_POINT('Ctrl Pts',(56.9617380090342,21.3678878281029,7.84467691744743));
#23235=CARTESIAN_POINT('Ctrl Pts',(56.9478582607508,21.4354729937093,7.84908231949497));
#23236=CARTESIAN_POINT('Ctrl Pts',(56.9304850929434,21.5022498067926,7.8534877215425));
#23237=CARTESIAN_POINT('Ctrl Pts',(56.9131356262496,21.5689355204954,7.8578871135788));
#23238=CARTESIAN_POINT('Ctrl Pts',(56.8923023260374,21.6348145900977,7.8622865056151));
#23239=CARTESIAN_POINT('Ctrl Pts',(56.8680831432016,21.6994947695202,7.8666858976514));
#23240=CARTESIAN_POINT('Ctrl Pts',(56.8438819052752,21.7641270249492,7.87108203001159));
#23241=CARTESIAN_POINT('Ctrl Pts',(56.8162999323649,21.8275616842975,7.87547816237179));
#23242=CARTESIAN_POINT('Ctrl Pts',(56.7854849764184,21.8894217005921,7.87987429473198));
#23243=CARTESIAN_POINT('Ctrl Pts',(56.7546818822706,21.9512579047138,7.88426873486075));
#23244=CARTESIAN_POINT('Ctrl Pts',(56.7206484962793,22.0115202208583,7.88866317498952));
#23245=CARTESIAN_POINT('Ctrl Pts',(56.6835798897769,22.0698534092289,7.89305761511829));
#23246=CARTESIAN_POINT('Ctrl Pts',(56.6465123564219,22.128184908836,7.89745192802668));
#23247=CARTESIAN_POINT('Ctrl Pts',(56.6064100470769,22.1845869706907,7.90184624093507));
#23248=CARTESIAN_POINT('Ctrl Pts',(56.5635119754025,22.2387323622449,7.90624055384346));
#23249=CARTESIAN_POINT('Ctrl Pts',(56.5205704205432,22.2929326377131,7.9106393210015));
#23250=CARTESIAN_POINT('Ctrl Pts',(56.4748277577648,22.34487128408,7.91503808815953));
#23251=CARTESIAN_POINT('Ctrl Pts',(56.426563324315,22.3942541533807,7.91943685531758));
#23252=CARTESIAN_POINT('Ctrl Pts',(56.3782727050157,22.4436638153379,7.92383800902502));
#23253=CARTESIAN_POINT('Ctrl Pts',(56.3274579612184,22.4905146028582,7.92823916273246));
#23254=CARTESIAN_POINT('Ctrl Pts',(56.2744331730675,22.5345512861697,7.9326403164399));
#23255=CARTESIAN_POINT('Ctrl Pts',(56.2213135028848,22.5786667682871,7.93704934552828));
#23256=CARTESIAN_POINT('Ctrl Pts',(56.1659762959802,22.6199577967211,7.94145837461667));
#23257=CARTESIAN_POINT('Ctrl Pts',(56.1087656593053,22.6582117703252,7.94586740370505));
#23258=CARTESIAN_POINT('Ctrl Pts',(56.0733020212838,22.6819245823412,7.94860046560936));
#23259=CARTESIAN_POINT('Ctrl Pts',(56.037119055604,22.7044712965235,7.95133352751366));
#23260=CARTESIAN_POINT('Ctrl Pts',(56.0003030488091,22.7258103525716,7.95406658941796));
#23261=CARTESIAN_POINT('Ctrl Pts',(55.9402263670326,22.7606316108018,7.95852642372903));
#23262=CARTESIAN_POINT('Ctrl Pts',(55.878211896727,22.7923802153581,7.9629862580401));
#23263=CARTESIAN_POINT('Ctrl Pts',(55.814606302618,22.8208361085597,7.96744609235117));
#23264=CARTESIAN_POINT('Ctrl Pts',(55.751111477527,22.849242445879,7.9718981598695));
#23265=CARTESIAN_POINT('Ctrl Pts',(55.686031476172,22.874367267309,7.97635022738782));
#23266=CARTESIAN_POINT('Ctrl Pts',(55.6197385506428,22.8960357832454,7.98080229490615));
#23267=CARTESIAN_POINT('Ctrl Pts',(55.5535120650873,22.9176825826018,7.98524990048157));
#23268=CARTESIAN_POINT('Ctrl Pts',(55.4860755284922,22.9358797974142,7.98969750605699));
#23269=CARTESIAN_POINT('Ctrl Pts',(55.417821041808,22.9505007407131,7.99414511163241));
#23270=CARTESIAN_POINT('Ctrl Pts',(55.3496157056091,22.9651111553788,7.99858951445907));
#23271=CARTESIAN_POINT('Ctrl Pts',(55.2805940652508,22.9761503110027,8.00303391728573));
#23272=CARTESIAN_POINT('Ctrl Pts',(55.2111614840226,22.9835418801138,8.00747832011239));
#23273=CARTESIAN_POINT('Ctrl Pts',(55.1956094787083,22.9851974965415,8.00847380919197));
#23274=CARTESIAN_POINT('Ctrl Pts',(55.1800368963047,22.9866703158932,8.00946929827154));
#23275=CARTESIAN_POINT('Ctrl Pts',(55.1644483516311,22.987959834138,8.01046478735112));
#23276=CARTESIAN_POINT('Origin',(55.,21.,6.22095488139522));
#23277=CARTESIAN_POINT('',(55.1644483561882,22.987959833761,8.96685094802471));
#23278=CARTESIAN_POINT('',(55.1644479310503,22.9879598689293,8.81003518437327));
#23279=CARTESIAN_POINT('',(55.1644483516311,22.987959834138,6.22095488139522));
#23280=CARTESIAN_POINT('Ctrl Pts',(55.1644483561882,22.987959833761,8.96685094802472));
#23281=CARTESIAN_POINT('Ctrl Pts',(55.1865084564878,22.9861349743398,8.96536845462905));
#23282=CARTESIAN_POINT('Ctrl Pts',(55.2085395154997,22.9839428077344,8.96390036621413));
#23283=CARTESIAN_POINT('Ctrl Pts',(55.2395823717726,22.9803309980166,8.96185353255058));
#23284=CARTESIAN_POINT('Ctrl Pts',(55.2486253068872,22.9792160162485,8.96125989859017));
#23285=CARTESIAN_POINT('Ctrl Pts',(55.2625679963084,22.9773998336391,8.96034898609838));
#23286=CARTESIAN_POINT('Ctrl Pts',(55.2674731711851,22.9767423096468,8.96002935466431));
#23287=CARTESIAN_POINT('Ctrl Pts',(55.2765201775166,22.9754952936337,8.95944144062812));
#23288=CARTESIAN_POINT('Ctrl Pts',(55.2806625788646,22.9749110311965,8.95917287900392));
#23289=CARTESIAN_POINT('Ctrl Pts',(55.2900266624855,22.9735602219081,8.95856718687728));
#23290=CARTESIAN_POINT('Ctrl Pts',(55.2952471506301,22.9727859833341,8.95823049302025));
#23291=CARTESIAN_POINT('Ctrl Pts',(55.3087211275041,22.9707330060598,8.95736388279193));
#23292=CARTESIAN_POINT('Ctrl Pts',(55.316969866643,22.9694231198871,8.95683566485312));
#23293=CARTESIAN_POINT('Ctrl Pts',(55.3691079277055,22.9608076191609,8.95351023926098));
#23294=CARTESIAN_POINT('Ctrl Pts',(55.4127543858073,22.9520864922565,8.95078604867752));
#23295=CARTESIAN_POINT('Ctrl Pts',(55.4693998110486,22.9387827862763,8.94728607288447));
#23296=CARTESIAN_POINT('Ctrl Pts',(55.4826911878615,22.9355164958973,8.94646743070764));
#23297=CARTESIAN_POINT('Ctrl Pts',(55.6551105323159,22.8912587195686,8.93586958493547));
#23298=CARTESIAN_POINT('Ctrl Pts',(55.8086174884301,22.8308939233631,8.92662221527559));
#23299=CARTESIAN_POINT('Ctrl Pts',(56.0118357841249,22.7203787568067,8.91284248232438));
#23300=CARTESIAN_POINT('Ctrl Pts',(56.0690281228826,22.6854353060446,8.90877935135671));
#23301=CARTESIAN_POINT('Ctrl Pts',(56.1366164073965,22.639314249335,8.903685266579));
#23302=CARTESIAN_POINT('Ctrl Pts',(56.1487880083567,22.6308078239558,8.90275583833901));
#23303=CARTESIAN_POINT('Ctrl Pts',(56.1678252651308,22.6171842828034,8.90128241344744));
#23304=CARTESIAN_POINT('Ctrl Pts',(56.1747550454281,22.6121573849866,8.90074187727456));
#23305=CARTESIAN_POINT('Ctrl Pts',(56.187667139856,22.602663429206,8.89972671264464));
#23306=CARTESIAN_POINT('Ctrl Pts',(56.193657169235,22.5982070774024,8.89925250530754));
#23307=CARTESIAN_POINT('Ctrl Pts',(56.2069932677625,22.5881687366505,8.89818933239269));
#23308=CARTESIAN_POINT('Ctrl Pts',(56.2143258734256,22.5825692253111,8.89759968619538));
#23309=CARTESIAN_POINT('Ctrl Pts',(56.2328096587034,22.5682500710014,8.89610023816652));
#23310=CARTESIAN_POINT('Ctrl Pts',(56.2439072057028,22.5594623388304,8.89518775392164));
#23311=CARTESIAN_POINT('Ctrl Pts',(56.3093213635956,22.506520807602,8.88973489358598));
#23312=CARTESIAN_POINT('Ctrl Pts',(56.3613708453414,22.459655723815,8.88508546416893));
#23313=CARTESIAN_POINT('Ctrl Pts',(56.5282364015195,22.2927087169441,8.86908451838339));
#23314=CARTESIAN_POINT('Ctrl Pts',(56.6304864742761,22.161079785623,8.857293965576));
#23315=CARTESIAN_POINT('Ctrl Pts',(56.7330859240166,21.9882623150716,8.84353657859717));
#23316=CARTESIAN_POINT('Ctrl Pts',(56.7501370813457,21.9577419845985,8.84116824626649));
#23317=CARTESIAN_POINT('Ctrl Pts',(56.7730403932579,21.9140902218614,8.83788145016341));
#23318=CARTESIAN_POINT('Ctrl Pts',(56.7795656026522,21.9013209538791,8.83693181604444));
#23319=CARTESIAN_POINT('Ctrl Pts',(56.7907981239385,21.8787422730067,8.83527478665353));
#23320=CARTESIAN_POINT('Ctrl Pts',(56.7955638712028,21.8689627726656,8.834564277132));
#23321=CARTESIAN_POINT('Ctrl Pts',(56.8025380649138,21.8543490626825,8.833513756575));
#23322=CARTESIAN_POINT('Ctrl Pts',(56.804807490471,21.8495444192596,8.83317015962952));
#23323=CARTESIAN_POINT('Ctrl Pts',(56.8088301525623,21.8409390937834,8.83255803144846));
#23324=CARTESIAN_POINT('Ctrl Pts',(56.810590646736,21.8371419182502,8.83228906146702));
#23325=CARTESIAN_POINT('Ctrl Pts',(56.8143947258009,21.8288688376022,8.83170552282115));
#23326=CARTESIAN_POINT('Ctrl Pts',(56.8164337033289,21.8243909106942,8.83139123632787));
#23327=CARTESIAN_POINT('Ctrl Pts',(56.8220464623999,21.8119424553793,8.83052173699147));
#23328=CARTESIAN_POINT('Ctrl Pts',(56.8255845418527,21.8039558129589,8.82996865266857));
#23329=CARTESIAN_POINT('Ctrl Pts',(56.8442367451569,21.7610933736043,8.82702446763403));
#23330=CARTESIAN_POINT('Ctrl Pts',(56.85840527113,21.7258116710683,8.8246859470485));
#23331=CARTESIAN_POINT('Ctrl Pts',(56.9155278156353,21.5709046628101,8.81469396784404));
#23332=CARTESIAN_POINT('Ctrl Pts',(56.9480057108673,21.4477258939431,8.80743463040236));
#23333=CARTESIAN_POINT('Ctrl Pts',(56.9881871096727,21.2022947470752,8.79295922802081));
#23334=CARTESIAN_POINT('Ctrl Pts',(56.9968175632529,21.0807768319081,8.78578164015386));
#23335=CARTESIAN_POINT('Ctrl Pts',(56.9939888480958,20.9423762883097,8.77718580361414));
#23336=CARTESIAN_POINT('Ctrl Pts',(56.9934303699947,20.9255194584189,8.77613215667945));
#23337=CARTESIAN_POINT('Ctrl Pts',(56.9922465063731,20.899689055796,8.77450650512826));
#23338=CARTESIAN_POINT('Ctrl Pts',(56.9917740579242,20.8907089867084,8.77393928047882));
#23339=CARTESIAN_POINT('Ctrl Pts',(56.9908421045692,20.8750179116583,8.77294443357605));
#23340=CARTESIAN_POINT('Ctrl Pts',(56.9904093403938,20.8683054154788,8.77251765539606));
#23341=CARTESIAN_POINT('Ctrl Pts',(56.9893543670329,20.853137314105,8.77155051840636));
#23342=CARTESIAN_POINT('Ctrl Pts',(56.9887121853851,20.8446832714074,8.77100954128639));
#23343=CARTESIAN_POINT('Ctrl Pts',(56.9868277155012,20.8218070373187,8.76954031167875));
#23344=CARTESIAN_POINT('Ctrl Pts',(56.9854823201596,20.8073940784083,8.76860884724143));
#23345=CARTESIAN_POINT('Ctrl Pts',(56.9784364090486,20.739863793031,8.76421653125217));
#23346=CARTESIAN_POINT('Ctrl Pts',(56.9707608782783,20.6869790146462,8.76069441012519));
#23347=CARTESIAN_POINT('Ctrl Pts',(56.9273992381471,20.454355228825,8.74482515023841));
#23348=CARTESIAN_POINT('Ctrl Pts',(56.869169214372,20.2797331910237,8.73179941161804));
#23349=CARTESIAN_POINT('Ctrl Pts',(56.7641527851455,20.067436638048,8.71557049069498));
#23350=CARTESIAN_POINT('Ctrl Pts',(56.7384150534879,20.0202940697493,8.71194787633662));
#23351=CARTESIAN_POINT('Ctrl Pts',(56.7060472880574,19.9663096292685,8.70782426258264));
#23352=CARTESIAN_POINT('Ctrl Pts',(56.7012352521229,19.9584090262773,8.70722142853358));
#23353=CARTESIAN_POINT('Ctrl Pts',(56.6937491459621,19.9463083101455,8.70629946944603));
#23354=CARTESIAN_POINT('Ctrl Pts',(56.6911140980956,19.942084381791,8.70597790234971));
#23355=CARTESIAN_POINT('Ctrl Pts',(56.6862370694153,19.93433138924,8.70538820431591));
#23356=CARTESIAN_POINT('Ctrl Pts',(56.6839998169274,19.9307995232722,8.70511978089514));
#23357=CARTESIAN_POINT('Ctrl Pts',(56.6789336723095,19.9228571403148,8.70451661803648));
#23358=CARTESIAN_POINT('Ctrl Pts',(56.6760985026165,19.9184507282493,8.70418229946691));
#23359=CARTESIAN_POINT('Ctrl Pts',(56.6687663337754,19.9071531696018,8.70332581431172));
#23360=CARTESIAN_POINT('Ctrl Pts',(56.6642439454849,19.900278504851,8.7028052809941));
#23361=CARTESIAN_POINT('Ctrl Pts',(56.6362263645125,19.8582565167433,8.69962616446429));
#23362=CARTESIAN_POINT('Ctrl Pts',(56.6116593732559,19.8238326866816,8.69703343051772));
#23363=CARTESIAN_POINT('Ctrl Pts',(56.5690774512852,19.7680083447545,8.69280166471653));
#23364=CARTESIAN_POINT('Ctrl Pts',(56.5516750033045,19.7461609829284,8.69113821789112));
#23365=CARTESIAN_POINT('Ctrl Pts',(56.4246422639128,19.5933788839755,8.67939690273966));
#23366=CARTESIAN_POINT('Ctrl Pts',(56.2990602063877,19.4766372599477,8.66977820784346));
#23367=CARTESIAN_POINT('Ctrl Pts',(56.1186217146426,19.347632673179,8.65642364828826));
#23368=CARTESIAN_POINT('Ctrl Pts',(56.0759835428922,19.3195562894424,8.65330278979114));
#23369=CARTESIAN_POINT('Ctrl Pts',(56.0206186201192,19.2860711362976,8.64926811520142));
#23370=CARTESIAN_POINT('Ctrl Pts',(56.0088466723956,19.2791156650106,8.64841127130339));
#23371=CARTESIAN_POINT('Ctrl Pts',(55.9898131525822,19.2681321008778,8.64702707573648));
#23372=CARTESIAN_POINT('Ctrl Pts',(55.9825961793813,19.264027292288,8.64650250149506));
#23373=CARTESIAN_POINT('Ctrl Pts',(55.9688062295423,19.2562975041036,8.64550057955995));
#23374=CARTESIAN_POINT('Ctrl Pts',(55.9622379920794,19.2526643285652,8.64502353642583));
#23375=CARTESIAN_POINT('Ctrl Pts',(55.9471891964025,19.2444507733732,8.64393088639118));
#23376=CARTESIAN_POINT('Ctrl Pts',(55.9386956841478,19.2398946429085,8.64331443081922));
#23377=CARTESIAN_POINT('Ctrl Pts',(55.9164455232961,19.2281659638668,8.64169996408948));
#23378=CARTESIAN_POINT('Ctrl Pts',(55.9026378420401,19.2210921461991,8.64069851363044));
#23379=CARTESIAN_POINT('Ctrl Pts',(55.7885075455003,19.1642928918249,8.63242265650306));
#23380=CARTESIAN_POINT('Ctrl Pts',(55.6842605767762,19.1229425526894,8.6248578133751));
#23381=CARTESIAN_POINT('Ctrl Pts',(55.4948114204314,19.0656832433802,8.61117717891633));
#23382=CARTESIAN_POINT('Ctrl Pts',(55.4109899186735,19.0461560159091,8.60515076391878));
#23383=CARTESIAN_POINT('Ctrl Pts',(55.2489589085595,19.0192998970607,8.59374296508921));
#23384=CARTESIAN_POINT('Ctrl Pts',(55.1710495409836,19.0110560464908,8.58836297019318));
#23385=CARTESIAN_POINT('Ctrl Pts',(55.0776135567572,19.006702141134,8.58217487221943));
#23386=CARTESIAN_POINT('Ctrl Pts',(55.0623688232796,19.0061669121444,8.58117369327942));
#23387=CARTESIAN_POINT('Ctrl Pts',(55.0410293850822,19.0056627027973,8.57978545106758));
#23388=CARTESIAN_POINT('Ctrl Pts',(55.0349391409071,19.0055467104376,8.57939075261287));
#23389=CARTESIAN_POINT('Ctrl Pts',(55.0245533542877,19.0053964939698,8.57872034015849));
#23390=CARTESIAN_POINT('Ctrl Pts',(55.020258085147,19.0053482447256,8.57844385662053));
#23391=CARTESIAN_POINT('Ctrl Pts',(55.0119814393164,19.0052820103319,8.57791263653424));
#23392=CARTESIAN_POINT('Ctrl Pts',(55.0080001448542,19.0052620694554,8.57765778797978));
#23393=CARTESIAN_POINT('Ctrl Pts',(54.9984307094535,19.0052427901047,8.57704681857676));
#23394=CARTESIAN_POINT('Ctrl Pts',(54.9928425409804,19.0052550133715,8.5766913353187));
#23395=CARTESIAN_POINT('Ctrl Pts',(54.9724233002512,19.0053854860776,8.5753968994575));
#23396=CARTESIAN_POINT('Ctrl Pts',(54.9575931835433,19.0056456618568,8.57446545805293));
#23397=CARTESIAN_POINT('Ctrl Pts',(54.8041096731952,19.010051208765,8.56490274726291));
#23398=CARTESIAN_POINT('Ctrl Pts',(54.6662245513131,19.0284841901866,8.55694662923051));
#23399=CARTESIAN_POINT('Ctrl Pts',(54.3985642979242,19.0931791887636,8.54095999199972));
#23400=CARTESIAN_POINT('Ctrl Pts',(54.2694431651416,19.1388255619681,8.53296443385819));
#23401=CARTESIAN_POINT('Ctrl Pts',(54.129862678246,19.2049491047315,8.52338510605496));
#23402=CARTESIAN_POINT('Ctrl Pts',(54.1138227293572,19.2128132476175,8.52227006836565));
#23403=CARTESIAN_POINT('Ctrl Pts',(54.089683946122,19.2250529818988,8.52056934336464));
#23404=CARTESIAN_POINT('Ctrl Pts',(54.0815059385225,19.2292710852675,8.51998915452102));
#23405=CARTESIAN_POINT('Ctrl Pts',(54.0667457556547,19.2370139470255,8.51893458805065));
#23406=CARTESIAN_POINT('Ctrl Pts',(54.0601535936528,19.2405193841449,8.51846089863803));
#23407=CARTESIAN_POINT('Ctrl Pts',(54.0460253017488,19.2481342753807,8.51743978876543));
#23408=CARTESIAN_POINT('Ctrl Pts',(54.0384957294043,19.2522555175807,8.51689195613921));
#23409=CARTESIAN_POINT('Ctrl Pts',(54.0182646751908,19.2634991023865,8.51541001917457));
#23410=CARTESIAN_POINT('Ctrl Pts',(54.0056143958029,19.2707120347098,8.51447268823011));
#23411=CARTESIAN_POINT('Ctrl Pts',(53.944330844241,19.306549465321,8.50987850104922));
#23412=CARTESIAN_POINT('Ctrl Pts',(53.8968524391625,19.3370879490345,8.50615279584404));
#23413=CARTESIAN_POINT('Ctrl Pts',(53.692979707825,19.4807968217045,8.48939029214187));
#23414=CARTESIAN_POINT('Ctrl Pts',(53.5522288976417,19.6142799848005,8.47560681094763));
#23415=CARTESIAN_POINT('Ctrl Pts',(53.4071433362011,19.7985170455179,8.45967015303951));
#23416=CARTESIAN_POINT('Ctrl Pts',(53.3824631539231,19.831955152345,8.45688739156822));
#23417=CARTESIAN_POINT('Ctrl Pts',(53.3539277007352,19.8732576422887,8.45360256297839));
#23418=CARTESIAN_POINT('Ctrl Pts',(53.3490580594482,19.8804049524273,8.45303948186538));
#23419=CARTESIAN_POINT('Ctrl Pts',(53.3415307435403,19.8916089130415,8.4521654074708));
#23420=CARTESIAN_POINT('Ctrl Pts',(53.3388411872525,19.8956438634574,8.45185234616995));
#23421=CARTESIAN_POINT('Ctrl Pts',(53.3338542186678,19.9031848981677,8.45127052445996));
#23422=CARTESIAN_POINT('Ctrl Pts',(53.3315531628786,19.9066883863992,8.45100152943208));
#23423=CARTESIAN_POINT('Ctrl Pts',(53.3263075874079,19.9147302015091,8.45038705914323));
#23424=CARTESIAN_POINT('Ctrl Pts',(53.3233704771758,19.9192732665751,8.45004207716746));
#23425=CARTESIAN_POINT('Ctrl Pts',(53.3157041490186,19.9312378696055,8.4491390119709));
#23426=CARTESIAN_POINT('Ctrl Pts',(53.3110054361819,19.9386789481484,8.44858287802332));
#23427=CARTESIAN_POINT('Ctrl Pts',(53.277938754316,19.9918205165758,8.44464832241344));
#23428=CARTESIAN_POINT('Ctrl Pts',(53.2513775054864,20.0386253051174,8.44137712021863));
#23429=CARTESIAN_POINT('Ctrl Pts',(53.137338675478,20.2599825048624,8.42651664325599));
#23430=CARTESIAN_POINT('Ctrl Pts',(53.073892839478,20.4456956293377,8.41563826537016));
#23431=CARTESIAN_POINT('Ctrl Pts',(53.0306708516761,20.6796940777217,8.40123124119365));
#23432=CARTESIAN_POINT('Ctrl Pts',(53.0242624151752,20.7219464670555,8.39860884713311));
#23433=CARTESIAN_POINT('Ctrl Pts',(53.0176372123726,20.7776400830117,8.39511009818263));
#23434=CARTESIAN_POINT('Ctrl Pts',(53.01619203513,20.7909256133051,8.39427238761282));
#23435=CARTESIAN_POINT('Ctrl Pts',(53.0140727632987,20.8124145428847,8.3929120059279));
#23436=CARTESIAN_POINT('Ctrl Pts',(53.0133157431484,20.8206094944647,8.39239194698179));
#23437=CARTESIAN_POINT('Ctrl Pts',(53.0119644584749,20.8362968097598,8.39139389186064));
#23438=CARTESIAN_POINT('Ctrl Pts',(53.0113617830378,20.8437883219442,8.39091616877902));
#23439=CARTESIAN_POINT('Ctrl Pts',(53.0100739931629,20.8610134498793,8.38981513991193));
#23440=CARTESIAN_POINT('Ctrl Pts',(53.0094179387315,20.8707489823764,8.38919093381222));
#23441=CARTESIAN_POINT('Ctrl Pts',(53.0075917999732,20.9011741345993,8.38723401127514));
#23442=CARTESIAN_POINT('Ctrl Pts',(53.006672703119,20.9218768861661,8.3858934976464));
#23443=CARTESIAN_POINT('Ctrl Pts',(53.0028886157614,21.0533021562294,8.37732417736831));
#23444=CARTESIAN_POINT('Ctrl Pts',(53.0089276765414,21.1640696505946,8.36981793052127));
#23445=CARTESIAN_POINT('Ctrl Pts',(53.0377459093852,21.3720756965672,8.35528135071259));
#23446=CARTESIAN_POINT('Ctrl Pts',(53.0586890283821,21.4692470232919,8.34830564531651));
#23447=CARTESIAN_POINT('Ctrl Pts',(53.0940430860314,21.5890797735252,8.33967779543385));
#23448=CARTESIAN_POINT('Ctrl Pts',(53.1017831588605,21.6135630731477,8.33791422517428));
#23449=CARTESIAN_POINT('Ctrl Pts',(53.1240844565702,21.6796395610817,8.33316336334213));
#23450=CARTESIAN_POINT('Ctrl Pts',(53.1395556393487,21.7209136611738,8.33020517847966));
#23451=CARTESIAN_POINT('Ctrl Pts',(53.1595610012074,21.7693381215845,8.3267727273883));
#23452=CARTESIAN_POINT('Ctrl Pts',(53.1627875511733,21.7770117613453,8.32622996905585));
#23453=CARTESIAN_POINT('Ctrl Pts',(53.1681338931271,21.7895073580286,8.32534833023924));
#23454=CARTESIAN_POINT('Ctrl Pts',(53.1702248750348,21.7943414224981,8.32500779355331));
#23455=CARTESIAN_POINT('Ctrl Pts',(53.1740100218018,21.8029979090291,8.32439902175636));
#23456=CARTESIAN_POINT('Ctrl Pts',(53.1756970715198,21.8068233192643,8.324130367564));
#23457=CARTESIAN_POINT('Ctrl Pts',(53.1794091582221,21.8151693595066,8.3235450472189));
#23458=CARTESIAN_POINT('Ctrl Pts',(53.1814390063079,21.8196877523496,8.32322867879699));
#23459=CARTESIAN_POINT('Ctrl Pts',(53.1872589967608,21.8325148743381,8.32233188233438));
#23460=CARTESIAN_POINT('Ctrl Pts',(53.1910894539519,21.8408053310915,8.32175385719594));
#23461=CARTESIAN_POINT('Ctrl Pts',(53.2166556398915,21.8951560827101,8.31797306098169));
#23462=CARTESIAN_POINT('Ctrl Pts',(53.240093699518,21.9404000821336,8.31486657731594));
#23463=CARTESIAN_POINT('Ctrl Pts',(53.3421338799864,22.1201654740435,8.30249346811853));
#23464=CARTESIAN_POINT('Ctrl Pts',(53.434632553002,22.2461628856551,8.29371005804209));
#23465=CARTESIAN_POINT('Ctrl Pts',(53.5958793195042,22.4191492921025,8.27974011144415));
#23466=CARTESIAN_POINT('Ctrl Pts',(53.6544279274001,22.4747789993472,8.27488223774061));
#23467=CARTESIAN_POINT('Ctrl Pts',(53.7274147296392,22.5361542172549,8.26895633068329));
#23468=CARTESIAN_POINT('Ctrl Pts',(53.7387535513966,22.5454774108227,8.26803930739593));
#23469=CARTESIAN_POINT('Ctrl Pts',(53.7575113832154,22.560556870767,8.26652751982694));
#23470=CARTESIAN_POINT('Ctrl Pts',(53.7648700946963,22.5663875069428,8.26593574284831));
#23471=CARTESIAN_POINT('Ctrl Pts',(53.7781667366115,22.5767710749924,8.26486862037936));
#23472=CARTESIAN_POINT('Ctrl Pts',(53.7840896773369,22.5813429834177,8.26439403905699));
#23473=CARTESIAN_POINT('Ctrl Pts',(53.7967609098303,22.5910106092592,8.26338028831986));
#23474=CARTESIAN_POINT('Ctrl Pts',(53.8035161450404,22.5960969419428,8.26284076339189));
#23475=CARTESIAN_POINT('Ctrl Pts',(53.8218289661225,22.6097039338127,8.26138051155975));
#23476=CARTESIAN_POINT('Ctrl Pts',(53.8334463743195,22.6181428738318,8.26045664456695));
#23477=CARTESIAN_POINT('Ctrl Pts',(53.8937646222515,22.6609711655489,8.25567171050551));
#23478=CARTESIAN_POINT('Ctrl Pts',(53.9438938107748,22.6932868647718,8.25173301769435));
#23479=CARTESIAN_POINT('Ctrl Pts',(54.129584481805,22.8015360597188,8.23726755946039));
#23480=CARTESIAN_POINT('Ctrl Pts',(54.272447558802,22.8638164101038,8.22631508550302));
#23481=CARTESIAN_POINT('Ctrl Pts',(54.4265132078227,22.9105425813831,8.21517514585918));
#23482=CARTESIAN_POINT('Ctrl Pts',(54.4319752533222,22.9121736176193,8.21478112214838));
#23483=CARTESIAN_POINT('Ctrl Pts',(54.465706940801,22.9220890430145,8.21235367404621));
#23484=CARTESIAN_POINT('Ctrl Pts',(54.4941512941139,22.9297700843759,8.2103322016777));
#23485=CARTESIAN_POINT('Ctrl Pts',(54.56213677925,22.9465221141484,8.20557530596302));
#23486=CARTESIAN_POINT('Ctrl Pts',(54.6018073095801,22.955023185108,8.20285874755967));
#23487=CARTESIAN_POINT('Ctrl Pts',(54.6497128623326,22.9637700026662,8.19967006300534));
#23488=CARTESIAN_POINT('Ctrl Pts',(54.657722254699,22.9651818370479,8.19914000347872));
#23489=CARTESIAN_POINT('Ctrl Pts',(54.6708803510907,22.9674183600539,8.19827446874979));
#23490=CARTESIAN_POINT('Ctrl Pts',(54.6760239593531,22.9682719002622,8.19793744118423));
#23491=CARTESIAN_POINT('Ctrl Pts',(54.6853071788527,22.9697749993185,8.19733161783432));
#23492=CARTESIAN_POINT('Ctrl Pts',(54.6894455036847,22.9704316850051,8.19706243185619));
#23493=CARTESIAN_POINT('Ctrl Pts',(54.6985534617127,22.971847564879,8.1964719177826));
#23494=CARTESIAN_POINT('Ctrl Pts',(54.7035238972793,22.972601012982,8.1961509144526));
#23495=CARTESIAN_POINT('Ctrl Pts',(54.7178211360494,22.9747130131255,8.19523102984217));
#23496=CARTESIAN_POINT('Ctrl Pts',(54.7271549402624,22.976024285558,8.19463472956572));
#23497=CARTESIAN_POINT('Ctrl Pts',(54.7935071774651,22.9848667597959,8.19042356482895));
#23498=CARTESIAN_POINT('Ctrl Pts',(54.8508243690611,22.9899958099968,8.18693128718723));
#23499=CARTESIAN_POINT('Ctrl Pts',(54.9936931458039,22.996571355401,8.17841136970841));
#23500=CARTESIAN_POINT('Ctrl Pts',(55.0792561425175,22.9950071188978,8.17347009990951));
#23501=CARTESIAN_POINT('Ctrl Pts',(55.1644483595783,22.9879598334805,8.16850613376992));
#23502=CARTESIAN_POINT('',(53.0052503954397,21.0012560281401,8.22095488139522));
#23503=CARTESIAN_POINT('Ctrl Pts',(55.1644483516311,22.987959834138,8.01046478735112));
#23504=CARTESIAN_POINT('Ctrl Pts',(55.0948703834473,22.99371547466,8.01490805700561));
#23505=CARTESIAN_POINT('Ctrl Pts',(55.0249742386028,22.995815270762,8.01935132666011));
#23506=CARTESIAN_POINT('Ctrl Pts',(54.9551724962436,22.9942462379072,8.02379459631461));
#23507=CARTESIAN_POINT('Ctrl Pts',(54.8853627279582,22.9926770246423,8.02823837686401));
#23508=CARTESIAN_POINT('Ctrl Pts',(54.8156478716461,22.9874381586569,8.03268215741341));
#23509=CARTESIAN_POINT('Ctrl Pts',(54.7464386782799,22.9785687298215,8.03712593796281));
#23510=CARTESIAN_POINT('Ctrl Pts',(54.6771547819335,22.969689727507,8.04157451503756));
#23511=CARTESIAN_POINT('Ctrl Pts',(54.6083781223961,22.9571724063764,8.04602309211231));
#23512=CARTESIAN_POINT('Ctrl Pts',(54.5405115177318,22.9411073893947,8.05047166918706));
#23513=CARTESIAN_POINT('Ctrl Pts',(54.4726014940703,22.925032094502,8.05492309232662));
#23514=CARTESIAN_POINT('Ctrl Pts',(54.4056031520644,22.9054047244854,8.05937451546619));
#23515=CARTESIAN_POINT('Ctrl Pts',(54.3399037173856,22.8823656552803,8.06382593860575));
#23516=CARTESIAN_POINT('Ctrl Pts',(54.2740964660976,22.8592887776171,8.06828466679065));
#23517=CARTESIAN_POINT('Ctrl Pts',(54.2095928253016,22.8327892164037,8.07274339497555));
#23518=CARTESIAN_POINT('Ctrl Pts',(54.1467587511724,22.8030548892918,8.07720212316045));
#23519=CARTESIAN_POINT('Ctrl Pts',(54.1284491801205,22.7943904379972,8.07850137681595));
#23520=CARTESIAN_POINT('Ctrl Pts',(54.1102812013221,22.7854516086545,8.07980063047145));
#23521=CARTESIAN_POINT('Ctrl Pts',(54.0922634203053,22.776243751399,8.08109988412695));
#23522=CARTESIAN_POINT('Ctrl Pts',(54.0303847541435,22.744621104601,8.08556192543676));
#23523=CARTESIAN_POINT('Ctrl Pts',(53.9700429673079,22.709701070478,8.09002396674658));
#23524=CARTESIAN_POINT('Ctrl Pts',(53.9116108382143,22.6716568412828,8.09448600805639));
#23525=CARTESIAN_POINT('Ctrl Pts',(53.8532641469313,22.6336682392861,8.0989415250953));
#23526=CARTESIAN_POINT('Ctrl Pts',(53.7968219760873,22.5925647740467,8.1033970421342));
#23527=CARTESIAN_POINT('Ctrl Pts',(53.742633042301,22.548565754557,8.1078525591731));
#23528=CARTESIAN_POINT('Ctrl Pts',(53.6885053116059,22.5046164292727,8.11230304397763));
#23529=CARTESIAN_POINT('Ctrl Pts',(53.6366261398674,22.4577783514479,8.11675352878216));
#23530=CARTESIAN_POINT('Ctrl Pts',(53.5873142773744,22.4083133925337,8.12120401358668));
#23531=CARTESIAN_POINT('Ctrl Pts',(53.5380320620621,22.3588781728446,8.12565182267951));
#23532=CARTESIAN_POINT('Ctrl Pts',(53.4913144370052,22.306819550072,8.13009963177234));
#23533=CARTESIAN_POINT('Ctrl Pts',(53.4474449834977,22.2524378161145,8.13454744086518));
#23534=CARTESIAN_POINT('Ctrl Pts',(53.4035871544836,22.1980704921862,8.13899407138104));
#23535=CARTESIAN_POINT('Ctrl Pts',(53.3625763044683,22.141381658573,8.14344070189691));
#23536=CARTESIAN_POINT('Ctrl Pts',(53.3246560659812,22.0827050684496,8.14788733241278));
#23537=CARTESIAN_POINT('Ctrl Pts',(53.2867331258202,22.0240242978406,8.15233427973428));
#23538=CARTESIAN_POINT('Ctrl Pts',(53.2519014969672,21.9633559002514,8.15678122705579));
#23539=CARTESIAN_POINT('Ctrl Pts',(53.220360799391,21.9010615285072,8.1612281743773));
#23540=CARTESIAN_POINT('Ctrl Pts',(53.1887861866401,21.8387001726865,8.16567990342548));
#23541=CARTESIAN_POINT('Ctrl Pts',(53.1605097885676,21.7747097889159,8.17013163247367));
#23542=CARTESIAN_POINT('Ctrl Pts',(53.1356842295709,21.7094746441061,8.17458336152186));
#23543=CARTESIAN_POINT('Ctrl Pts',(53.1108438409058,21.644200530765,8.17903774983206));
#23544=CARTESIAN_POINT('Ctrl Pts',(53.0894585437783,21.5776806404973,8.18349213814226));
#23545=CARTESIAN_POINT('Ctrl Pts',(53.0716310834577,21.5103144953981,8.18794652645247));
#23546=CARTESIAN_POINT('Ctrl Pts',(53.0537726691785,21.4428313819352,8.19240864895187));
#23547=CARTESIAN_POINT('Ctrl Pts',(53.039484522774,21.3744995576203,8.19687077145126));
#23548=CARTESIAN_POINT('Ctrl Pts',(53.0288181401238,21.3057280454834,8.20133289395066));
#23549=CARTESIAN_POINT('Ctrl Pts',(53.0233996096131,21.2707920649357,8.20359965557908));
#23550=CARTESIAN_POINT('Ctrl Pts',(53.018914896146,21.2357426891999,8.20586641720751));
#23551=CARTESIAN_POINT('Ctrl Pts',(53.0153656007572,21.2006336558065,8.20813317883593));
#23552=CARTESIAN_POINT('Ctrl Pts',(53.0086735267431,21.1344367845124,8.21240707968903));
#23553=CARTESIAN_POINT('Ctrl Pts',(53.0052923566473,21.0678963361395,8.21668098054213));
#23554=CARTESIAN_POINT('Ctrl Pts',(53.0052503954397,21.0012560281401,8.22095488139522));
#23555=CARTESIAN_POINT('Ctrl Pts',(53.0052504499798,21.0013398486355,8.22235592323264));
#23556=CARTESIAN_POINT('Ctrl Pts',(53.0052354588656,20.979021269004,8.22369119184465));
#23557=CARTESIAN_POINT('Ctrl Pts',(53.0055950411512,20.9567032697669,8.22501509771246));
#23558=CARTESIAN_POINT('Ctrl Pts',(53.0118822235976,20.7656411471647,8.23628596927151));
#23559=CARTESIAN_POINT('Ctrl Pts',(53.038837182935,20.5982800528773,8.24580309326332));
#23560=CARTESIAN_POINT('Ctrl Pts',(53.0958551742049,20.4047321928301,8.25795760527897));
#23561=CARTESIAN_POINT('Ctrl Pts',(53.1059377588708,20.3733906086174,8.25996094695637));
#23562=CARTESIAN_POINT('Ctrl Pts',(53.1246729231539,20.3197445873193,8.26346098531721));
#23563=CARTESIAN_POINT('Ctrl Pts',(53.1329598296126,20.2973194202502,8.26494592515493));
#23564=CARTESIAN_POINT('Ctrl Pts',(53.1453892230824,20.2654576737732,8.26708961418652));
#23565=CARTESIAN_POINT('Ctrl Pts',(53.1492051088484,20.2558952846873,8.2677373991672));
#23566=CARTESIAN_POINT('Ctrl Pts',(53.1559520551253,20.2393608386296,8.26886537102514));
#23567=CARTESIAN_POINT('Ctrl Pts',(53.1588490825913,20.2323750567181,8.26934439606832));
#23568=CARTESIAN_POINT('Ctrl Pts',(53.1645014393616,20.2189612647145,8.27026901623429));
#23569=CARTESIAN_POINT('Ctrl Pts',(53.167250990435,20.2125309288626,8.2707144083219));
#23570=CARTESIAN_POINT('Ctrl Pts',(53.1738297883286,20.1973662910301,8.27176992170854));
#23571=CARTESIAN_POINT('Ctrl Pts',(53.1776879431349,20.1886447911613,8.27238102846664));
#23572=CARTESIAN_POINT('Ctrl Pts',(53.191458640716,20.1581093803898,8.27453512457026));
#23573=CARTESIAN_POINT('Ctrl Pts',(53.2017012092166,20.1364474311519,8.2760894431332));
#23574=CARTESIAN_POINT('Ctrl Pts',(53.2765002348601,19.985360127803,8.28712075167099));
#23575=CARTESIAN_POINT('Ctrl Pts',(53.354563967129,19.8631310456656,8.29708629822046));
#23576=CARTESIAN_POINT('Ctrl Pts',(53.4997175605774,19.6825125944605,8.31325773128512));
#23577=CARTESIAN_POINT('Ctrl Pts',(53.5586970386458,19.6182374923628,8.31935566144467));
#23578=CARTESIAN_POINT('Ctrl Pts',(53.6432006933683,19.5374650746013,8.32732090089623));
#23579=CARTESIAN_POINT('Ctrl Pts',(53.6651667349387,19.5173897631785,8.32932810551325));
#23580=CARTESIAN_POINT('Ctrl Pts',(53.6972128646045,19.4893918312796,8.33215790101528));
#23581=CARTESIAN_POINT('Ctrl Pts',(53.706932007257,19.481064008949,8.33300364016904));
#23582=CARTESIAN_POINT('Ctrl Pts',(53.7221350853931,19.4682889798934,8.33430645185761));
#23583=CARTESIAN_POINT('Ctrl Pts',(53.7275634236692,19.463776529334,8.33476771348039));
#23584=CARTESIAN_POINT('Ctrl Pts',(53.7377414858454,19.4554067067298,8.33562511388652));
#23585=CARTESIAN_POINT('Ctrl Pts',(53.7424852072569,19.4515422038009,8.33602173650106));
#23586=CARTESIAN_POINT('Ctrl Pts',(53.7505402179061,19.4450415673173,8.33669006891283));
#23587=CARTESIAN_POINT('Ctrl Pts',(53.7538422257107,19.4423940558081,8.33696258829237));
#23588=CARTESIAN_POINT('Ctrl Pts',(53.7602180910616,19.4373152142198,8.33748597499489));
#23589=CARTESIAN_POINT('Ctrl Pts',(53.7632906932421,19.4348824284845,8.33773695284236));
#23590=CARTESIAN_POINT('Ctrl Pts',(53.7713886425627,19.4285094740506,8.33839519886141));
#23591=CARTESIAN_POINT('Ctrl Pts',(53.776425825021,19.424584314608,8.33880141044685));
#23592=CARTESIAN_POINT('Ctrl Pts',(53.7941172548509,19.4109345324222,8.34021714740838));
#23593=CARTESIAN_POINT('Ctrl Pts',(53.8068696665272,19.4013373400012,8.34121818052374));
#23594=CARTESIAN_POINT('Ctrl Pts',(53.9035917225248,19.3303485384072,8.34867712024682));
#23595=CARTESIAN_POINT('Ctrl Pts',(53.9921440466086,19.275448154112,8.35476314360415));
#23596=CARTESIAN_POINT('Ctrl Pts',(54.1627020086377,19.1873527996347,8.36591987249285));
#23597=CARTESIAN_POINT('Ctrl Pts',(54.2434001979792,19.152213748393,8.37098979536434));
#23598=CARTESIAN_POINT('Ctrl Pts',(54.3996672731362,19.0961278703635,8.38077956062949));
#23599=CARTESIAN_POINT('Ctrl Pts',(54.4746627248512,19.0740853594523,8.38546620294678));
#23600=CARTESIAN_POINT('Ctrl Pts',(54.570635995411,19.0519007669188,8.39155807552668));
#23601=CARTESIAN_POINT('Ctrl Pts',(54.5905889723066,19.0476100202893,8.39282936918941));
#23602=CARTESIAN_POINT('Ctrl Pts',(54.6201307571847,19.0417300285119,8.39472013085657));
#23603=CARTESIAN_POINT('Ctrl Pts',(54.6296713868745,19.0399034116127,8.39533206023183));
#23604=CARTESIAN_POINT('Ctrl Pts',(54.6466281862664,19.0367851399428,8.39642212331452));
#23605=CARTESIAN_POINT('Ctrl Pts',(54.6540390914874,19.0354656346247,8.39689936416734));
#23606=CARTESIAN_POINT('Ctrl Pts',(54.6696255649875,19.032781406114,8.39790491411394));
#23607=CARTESIAN_POINT('Ctrl Pts',(54.6778025092209,19.0314256333667,8.39843349658196));
#23608=CARTESIAN_POINT('Ctrl Pts',(54.6993826216341,19.0279856133351,8.39983138818227));
#23609=CARTESIAN_POINT('Ctrl Pts',(54.7127988265832,19.0259870769582,8.40070338045249));
#23610=CARTESIAN_POINT('Ctrl Pts',(54.7701384370223,19.0180424274027,8.40444334849047));
#23611=CARTESIAN_POINT('Ctrl Pts',(54.8142301760946,19.0134247520525,8.40735248751739));
#23612=CARTESIAN_POINT('Ctrl Pts',(55.05030806839,18.9966284020374,8.42311611347497));
#23613=CARTESIAN_POINT('Ctrl Pts',(55.243134248663,19.0108065762286,8.43678591134482));
#23614=CARTESIAN_POINT('Ctrl Pts',(55.4839463341905,19.0640825457091,8.45368607612069));
#23615=CARTESIAN_POINT('Ctrl Pts',(55.5365074913047,19.077985088639,8.45735361782112));
#23616=CARTESIAN_POINT('Ctrl Pts',(55.597325338169,19.0967615813014,8.46152337226817));
#23617=CARTESIAN_POINT('Ctrl Pts',(55.6061916527687,19.0995669635042,8.46212937469842));
#23618=CARTESIAN_POINT('Ctrl Pts',(55.6197941343001,19.1039757943543,8.46305583931023));
#23619=CARTESIAN_POINT('Ctrl Pts',(55.624544291256,19.1055351713768,8.46337876016643));
#23620=CARTESIAN_POINT('Ctrl Pts',(55.6332646693485,19.1084342524079,8.46397038935791));
#23621=CARTESIAN_POINT('Ctrl Pts',(55.6372365277963,19.1097686048313,8.4642393956039));
#23622=CARTESIAN_POINT('Ctrl Pts',(55.6461688944084,19.1128008027511,8.46484333739955));
#23623=CARTESIAN_POINT('Ctrl Pts',(55.6511269202628,19.1145056920213,8.46517785503626));
#23624=CARTESIAN_POINT('Ctrl Pts',(55.6656898017097,19.1195776436002,8.46615848566965));
#23625=CARTESIAN_POINT('Ctrl Pts',(55.6752758479297,19.1229987506424,8.46680151697287));
#23626=CARTESIAN_POINT('Ctrl Pts',(55.7505634683038,19.1505191397754,8.47183541923421));
#23627=CARTESIAN_POINT('Ctrl Pts',(55.8149893950069,19.1779902543872,8.47604509441022));
#23628=CARTESIAN_POINT('Ctrl Pts',(56.0302021138878,19.2834629651191,8.4901952796307));
#23629=CARTESIAN_POINT('Ctrl Pts',(56.1724070251791,19.3772615734261,8.49976134008208));
#23630=CARTESIAN_POINT('Ctrl Pts',(56.3391834407498,19.5207606619325,8.5130153521124));
#23631=CARTESIAN_POINT('Ctrl Pts',(56.3760805099183,19.5550214225224,8.51609464217308));
#23632=CARTESIAN_POINT('Ctrl Pts',(56.4212583621677,19.6002723327611,8.52008236633211));
#23633=CARTESIAN_POINT('Ctrl Pts',(56.4307773185375,19.6100039119936,8.52093551795479));
#23634=CARTESIAN_POINT('Ctrl Pts',(56.4459317975964,19.6258175055055,8.52231523675366));
#23635=CARTESIAN_POINT('Ctrl Pts',(56.4516304125659,19.6318386668867,8.52283906160205));
#23636=CARTESIAN_POINT('Ctrl Pts',(56.4624198249165,19.6433820629601,8.52384053792747));
#23637=CARTESIAN_POINT('Ctrl Pts',(56.4675173021618,19.6488978807161,8.52431789137474));
#23638=CARTESIAN_POINT('Ctrl Pts',(56.4791036524311,19.6615780263406,8.52541264935526));
#23639=CARTESIAN_POINT('Ctrl Pts',(56.4855718039228,19.6687609515334,8.52603091313816));
#23640=CARTESIAN_POINT('Ctrl Pts',(56.502344177446,19.6876612464348,8.52765301605488));
#23641=CARTESIAN_POINT('Ctrl Pts',(56.5125634059593,19.6994528260736,8.52866034571494));
#23642=CARTESIAN_POINT('Ctrl Pts',(56.6013026288582,19.8043063555221,8.53757888215547));
#23643=CARTESIAN_POINT('Ctrl Pts',(56.6712729892373,19.904239787237,8.5458368146718));
#23644=CARTESIAN_POINT('Ctrl Pts',(56.790711489939,20.1131403271629,8.56252145612563));
#23645=CARTESIAN_POINT('Ctrl Pts',(56.8403846181662,20.2214417561895,8.5709033252617));
#23646=CARTESIAN_POINT('Ctrl Pts',(56.8952961378108,20.376346002623,8.58210457839388));
#23647=CARTESIAN_POINT('Ctrl Pts',(56.9090100793399,20.4196785325523,8.58515529264944));
#23648=CARTESIAN_POINT('Ctrl Pts',(56.923617085572,20.471981606668,8.58871024712029));
#23649=CARTESIAN_POINT('Ctrl Pts',(56.9259442255193,20.4805339637347,8.5892875159814));
#23650=CARTESIAN_POINT('Ctrl Pts',(56.9294679126777,20.4938329404382,8.59017864027216));
#23651=CARTESIAN_POINT('Ctrl Pts',(56.9307040877944,20.4985688034615,8.59049469500652));
#23652=CARTESIAN_POINT('Ctrl Pts',(56.9329648405286,20.5073622018794,8.5910790993988));
#23653=CARTESIAN_POINT('Ctrl Pts',(56.9339940742078,20.511418383159,8.59134770499359));
#23654=CARTESIAN_POINT('Ctrl Pts',(56.9363078023734,20.5206585981959,8.59195743154538));
#23655=CARTESIAN_POINT('Ctrl Pts',(56.9375842456032,20.5258445636657,8.59229808789103));
#23656=CARTESIAN_POINT('Ctrl Pts',(56.9408548516365,20.5393662344828,8.59318242827497));
#23657=CARTESIAN_POINT('Ctrl Pts',(56.9428161710456,20.5477098798375,8.59372429174151));
#23658=CARTESIAN_POINT('Ctrl Pts',(56.9555329374395,20.603417713735,8.59731825910798));
#23659=CARTESIAN_POINT('Ctrl Pts',(56.9646101457994,20.6511527400874,8.60028312388294));
#23660=CARTESIAN_POINT('Ctrl Pts',(56.9828747253291,20.7708790467991,8.60754180860352));
#23661=CARTESIAN_POINT('Ctrl Pts',(56.989894882159,20.8431300449526,8.6117655217173));
#23662=CARTESIAN_POINT('Ctrl Pts',(56.9976909662492,21.0272357279495,8.62246337546874));
#23663=CARTESIAN_POINT('Ctrl Pts',(56.9930308699611,21.1390575238036,8.6289105777023));
#23664=CARTESIAN_POINT('Ctrl Pts',(56.9718463871838,21.3068253484483,8.6390457916876));
#23665=CARTESIAN_POINT('Ctrl Pts',(56.9622056810899,21.3634114747572,8.64254291432021));
#23666=CARTESIAN_POINT('Ctrl Pts',(56.947158695099,21.4333608157624,8.64700117597994));
#23667=CARTESIAN_POINT('Ctrl Pts',(56.9440293846614,21.4471893510382,8.64788916234444));
#23668=CARTESIAN_POINT('Ctrl Pts',(56.9388100093969,21.4691630821336,8.64931124539091));
#23669=CARTESIAN_POINT('Ctrl Pts',(56.9368153569075,21.4773306190817,8.64984227415833));
#23670=CARTESIAN_POINT('Ctrl Pts',(56.932949860111,21.492735504625,8.65084858882708));
#23671=CARTESIAN_POINT('Ctrl Pts',(56.931089846383,21.499975441319,8.65132351777365));
#23672=CARTESIAN_POINT('Ctrl Pts',(56.9267921078319,21.5163221969054,8.65240041308718));
#23673=CARTESIAN_POINT('Ctrl Pts',(56.9243304417408,21.5254224812113,8.6530031454815));
#23674=CARTESIAN_POINT('Ctrl Pts',(56.9178297183122,21.5487957376671,8.654559671652));
#23675=CARTESIAN_POINT('Ctrl Pts',(56.9136958533978,21.563041518063,8.65551652052281));
#23676=CARTESIAN_POINT('Ctrl Pts',(56.8847508403948,21.6587863625304,8.66200386829715));
#23677=CARTESIAN_POINT('Ctrl Pts',(56.8549028676035,21.7386589775971,8.66769851550477));
#23678=CARTESIAN_POINT('Ctrl Pts',(56.7704463885792,21.9269491828465,8.68180497258093));
#23679=CARTESIAN_POINT('Ctrl Pts',(56.7108744673618,22.0327730985579,8.69032922898264));
#23680=CARTESIAN_POINT('Ctrl Pts',(56.6011321564454,22.191890848665,8.70372904869594));
#23681=CARTESIAN_POINT('Ctrl Pts',(56.5569956646777,22.2489974488875,8.70866978976218));
#23682=CARTESIAN_POINT('Ctrl Pts',(56.5002911599855,22.3146742295513,8.71440522798627));
#23683=CARTESIAN_POINT('Ctrl Pts',(56.4906016446421,22.3256502788447,8.71536558289372));
#23684=CARTESIAN_POINT('Ctrl Pts',(56.4767802436842,22.3409636541807,8.71670681956132));
#23685=CARTESIAN_POINT('Ctrl Pts',(56.4727486056412,22.3453902618937,8.71709469400604));
#23686=CARTESIAN_POINT('Ctrl Pts',(56.4658059340686,22.3529444853584,8.71775680220727));
#23687=CARTESIAN_POINT('Ctrl Pts',(56.4629046892727,22.3560810035931,8.71803176282822));
#23688=CARTESIAN_POINT('Ctrl Pts',(56.4568847852795,22.362547282515,8.71859869650468));
#23689=CARTESIAN_POINT('Ctrl Pts',(56.4537647637878,22.3658756851386,8.71889056223909));
#23690=CARTESIAN_POINT('Ctrl Pts',(56.445585643216,22.3745413015623,8.71965066097602));
#23691=CARTESIAN_POINT('Ctrl Pts',(56.4405083442694,22.3798613537975,8.72011752111943));
#23692=CARTESIAN_POINT('Ctrl Pts',(56.4196502942204,22.4014760582974,8.72201581206585));
#23693=CARTESIAN_POINT('Ctrl Pts',(56.403620870934,22.4175297717299,8.72342922169651));
#23694=CARTESIAN_POINT('Ctrl Pts',(56.287187640355,22.530227292239,8.73340821824288));
#23695=CARTESIAN_POINT('Ctrl Pts',(56.1771614556021,22.6163998289023,8.7413638884873));
#23696=CARTESIAN_POINT('Ctrl Pts',(55.9988968815992,22.728082497975,8.7535937769187));
#23697=CARTESIAN_POINT('Ctrl Pts',(55.9367912107991,22.7625224599454,8.75774512955749));
#23698=CARTESIAN_POINT('Ctrl Pts',(55.818387456376,22.8201529311676,8.76562069101969));
#23699=CARTESIAN_POINT('Ctrl Pts',(55.7626090740419,22.8442182710925,8.76931545442381));
#23700=CARTESIAN_POINT('Ctrl Pts',(55.6923237372138,22.8708083127928,8.77399643514121));
#23701=CARTESIAN_POINT('Ctrl Pts',(55.6787688702862,22.8757688300408,8.77490024145092));
#23702=CARTESIAN_POINT('Ctrl Pts',(55.6571763113675,22.8834061168609,8.77634217499607));
#23703=CARTESIAN_POINT('Ctrl Pts',(55.649173176725,22.8861796012813,8.77687709086558));
#23704=CARTESIAN_POINT('Ctrl Pts',(55.6340730904238,22.8913050452776,8.77788735158136));
#23705=CARTESIAN_POINT('Ctrl Pts',(55.6269800875571,22.8936682459199,8.77836231547541));
#23706=CARTESIAN_POINT('Ctrl Pts',(55.6109803514363,22.8988991877287,8.7794346985187));
#23707=CARTESIAN_POINT('Ctrl Pts',(55.6020664363841,22.9017442299764,8.78003285136743));
#23708=CARTESIAN_POINT('Ctrl Pts',(55.5792097578523,22.9088625609522,8.78156854137682));
#23709=CARTESIAN_POINT('Ctrl Pts',(55.5652397433671,22.9130458002811,8.78250898928305));
#23710=CARTESIAN_POINT('Ctrl Pts',(55.4759728459328,22.9387131177805,8.78853110534031));
#23711=CARTESIAN_POINT('Ctrl Pts',(55.3995210587367,22.9558984917152,8.79375032686555));
#23712=CARTESIAN_POINT('Ctrl Pts',(55.269895633711,22.9771191115937,8.80269640197856));
#23713=CARTESIAN_POINT('Ctrl Pts',(55.2172477843832,22.9835921617255,8.80635502660011));
#23714=CARTESIAN_POINT('Ctrl Pts',(55.1644479310504,22.9879598689293,8.81003518437327));
#23715=CARTESIAN_POINT('Origin',(55.,21.,6.22095488139522));
#23716=CARTESIAN_POINT('',(55.1644488239152,22.9879597950695,9.76988214123148));
#23717=CARTESIAN_POINT('',(55.1644483514339,22.9879598341543,9.61229346745724));
#23718=CARTESIAN_POINT('',(55.1644483516311,22.987959834138,6.22095488139522));
#23719=CARTESIAN_POINT('',(53.0052507447458,20.9982762938427,9.17962824983008));
#23720=CARTESIAN_POINT('Ctrl Pts',(55.1644488239152,22.9879597950695,9.76988214123148));
#23721=CARTESIAN_POINT('Ctrl Pts',(55.2474358169254,22.981094911064,9.76424197462399));
#23722=CARTESIAN_POINT('Ctrl Pts',(55.3299662031272,22.9690359088409,9.75847082587752));
#23723=CARTESIAN_POINT('Ctrl Pts',(55.5350448108733,22.9257940103328,9.74386339208412));
#23724=CARTESIAN_POINT('Ctrl Pts',(55.6557960150322,22.8880923220085,9.73500686785206));
#23725=CARTESIAN_POINT('Ctrl Pts',(55.7865152809458,22.8332110941054,9.72561977685455));
#23726=CARTESIAN_POINT('Ctrl Pts',(55.8007778150162,22.8270260341522,9.72459866881045));
#23727=CARTESIAN_POINT('Ctrl Pts',(55.8207325538242,22.8180939299511,9.72317587753889));
#23728=CARTESIAN_POINT('Ctrl Pts',(55.8264858081968,22.8154857957321,9.72276635504612));
#23729=CARTESIAN_POINT('Ctrl Pts',(55.8357772999726,22.8112203430816,9.72210621116057));
#23730=CARTESIAN_POINT('Ctrl Pts',(55.8393231710697,22.8095799074625,9.7218545756369));
#23731=CARTESIAN_POINT('Ctrl Pts',(55.8468201482237,22.8060847847211,9.72132320228721));
#23732=CARTESIAN_POINT('Ctrl Pts',(55.8507700316668,22.8042275263844,9.72104362977629));
#23733=CARTESIAN_POINT('Ctrl Pts',(55.8605365230152,22.7995960611537,9.72035324505411));
#23734=CARTESIAN_POINT('Ctrl Pts',(55.8663459031227,22.7968065754721,9.7199433668461));
#23735=CARTESIAN_POINT('Ctrl Pts',(55.8879724378284,22.7862929075207,9.71842006386957));
#23736=CARTESIAN_POINT('Ctrl Pts',(55.9037012002137,22.7783873573699,9.71731728546934));
#23737=CARTESIAN_POINT('Ctrl Pts',(55.9431738678502,22.7578887455393,9.71455756444242));
#23738=CARTESIAN_POINT('Ctrl Pts',(55.9667723176467,22.7450218381241,9.71291491478273));
#23739=CARTESIAN_POINT('Ctrl Pts',(56.1435284019199,22.6439599284703,9.70061187828319));
#23740=CARTESIAN_POINT('Ctrl Pts',(56.2846240314052,22.5362337799521,9.69072815261629));
#23741=CARTESIAN_POINT('Ctrl Pts',(56.4306772155898,22.3903490240591,9.67847587761321));
#23742=CARTESIAN_POINT('Ctrl Pts',(56.4511961516365,22.3689183049465,9.676701645126));
#23743=CARTESIAN_POINT('Ctrl Pts',(56.5023842136163,22.3130109556065,9.67212420401288));
#23744=CARTESIAN_POINT('Ctrl Pts',(56.532347538901,22.2779149461626,9.6692977715779));
#23745=CARTESIAN_POINT('Ctrl Pts',(56.5696233429099,22.2310560852789,9.66556445982336));
#23746=CARTESIAN_POINT('Ctrl Pts',(56.5780693846057,22.2202104433644,9.66470310064605));
#23747=CARTESIAN_POINT('Ctrl Pts',(56.5914455021725,22.2026628687031,9.66331336621481));
#23748=CARTESIAN_POINT('Ctrl Pts',(56.5964470156194,22.1960157545216,9.66278780918401));
#23749=CARTESIAN_POINT('Ctrl Pts',(56.6058798704214,22.1833147040329,9.66178516108847));
#23750=CARTESIAN_POINT('Ctrl Pts',(56.6103189311115,22.177266658233,9.66130838217501));
#23751=CARTESIAN_POINT('Ctrl Pts',(56.6203649879426,22.1634161695281,9.66021795587926));
#23752=CARTESIAN_POINT('Ctrl Pts',(56.6259499066247,22.1555980155208,9.65960347210462));
#23753=CARTESIAN_POINT('Ctrl Pts',(56.6429365338391,22.1314520320584,9.65770861135957));
#23754=CARTESIAN_POINT('Ctrl Pts',(56.6541501032143,22.1149939656289,9.65642114057298));
#23755=CARTESIAN_POINT('Ctrl Pts',(56.7457084598481,21.9761928106598,9.64559336508185));
#23756=CARTESIAN_POINT('Ctrl Pts',(56.812594561048,21.845538714214,9.63554515303679));
#23757=CARTESIAN_POINT('Ctrl Pts',(56.9089178011617,21.5921398840548,9.61664882556592));
#23758=CARTESIAN_POINT('Ctrl Pts',(56.942215883163,21.4715927667568,9.60789722510685));
#23759=CARTESIAN_POINT('Ctrl Pts',(56.9667614392938,21.3333476141695,9.59859970133848));
#23760=CARTESIAN_POINT('Ctrl Pts',(56.9693097130607,21.3179472931397,9.59757433448284));
#23761=CARTESIAN_POINT('Ctrl Pts',(56.9726366329678,21.2962639231247,9.5961466534224));
#23762=CARTESIAN_POINT('Ctrl Pts',(56.9735664740676,21.2900051257218,9.59573642979091));
#23763=CARTESIAN_POINT('Ctrl Pts',(56.9750225436277,21.279872816958,9.59507546040254));
#23764=CARTESIAN_POINT('Ctrl Pts',(56.9755671857392,21.2760020593865,9.59482369570737));
#23765=CARTESIAN_POINT('Ctrl Pts',(56.9766955732899,21.26780814571,9.59429234152571));
#23766=CARTESIAN_POINT('Ctrl Pts',(56.9772765219454,21.2634846273082,9.5940129159934));
#23767=CARTESIAN_POINT('Ctrl Pts',(56.9786790485502,21.2527808673986,9.59332339749371));
#23768=CARTESIAN_POINT('Ctrl Pts',(56.979483963707,21.2463984258503,9.59291423334154));
#23769=CARTESIAN_POINT('Ctrl Pts',(56.9823663404423,21.2226169178665,9.59139665701355));
#23770=CARTESIAN_POINT('Ctrl Pts',(56.9842454658417,21.2051940076959,9.59029878776543));
#23771=CARTESIAN_POINT('Ctrl Pts',(56.9884088527083,21.1611559738872,9.58755385706965));
#23772=CARTESIAN_POINT('Ctrl Pts',(56.9903886291186,21.1345149033365,9.5859208942389));
#23773=CARTESIAN_POINT('Ctrl Pts',(57.0012374766212,20.9341354214146,9.57379238754803));
#23774=CARTESIAN_POINT('Ctrl Pts',(56.987880697524,20.759934918808,9.56405313362454));
#23775=CARTESIAN_POINT('Ctrl Pts',(56.9458918179942,20.5601816403046,9.5519569544631));
#23776=CARTESIAN_POINT('Ctrl Pts',(56.9390276996911,20.53084477362,9.55015823917536));
#23777=CARTESIAN_POINT('Ctrl Pts',(56.9194413860788,20.4549283736556,9.54543142879155));
#23778=CARTESIAN_POINT('Ctrl Pts',(56.90568844675,20.4086377740589,9.54247720801513));
#23779=CARTESIAN_POINT('Ctrl Pts',(56.88580878461,20.349655503763,9.5385976273945));
#23780=CARTESIAN_POINT('Ctrl Pts',(56.8812078832709,20.3364643038237,9.53772243070247));
#23781=CARTESIAN_POINT('Ctrl Pts',(56.8736302293252,20.3154509883344,9.53631568562753));
#23782=CARTESIAN_POINT('Ctrl Pts',(56.8707420971984,20.3075972357615,9.53578708162576));
#23783=CARTESIAN_POINT('Ctrl Pts',(56.8654376013774,20.2934481009899,9.53482953734228));
#23784=CARTESIAN_POINT('Ctrl Pts',(56.8630385577829,20.2871463256661,9.53440118123162));
#23785=CARTESIAN_POINT('Ctrl Pts',(56.857308563916,20.2723213620472,9.53338896403459));
#23786=CARTESIAN_POINT('Ctrl Pts',(56.8539508457987,20.2638087487069,9.53280421193344));
#23787=CARTESIAN_POINT('Ctrl Pts',(56.843954889813,20.2389687435305,9.53108737416788));
#23788=CARTESIAN_POINT('Ctrl Pts',(56.8371588224166,20.2227062092671,9.52994999600638));
#23789=CARTESIAN_POINT('Ctrl Pts',(56.8212816287692,20.1860849763646,9.52735761091268));
#23790=CARTESIAN_POINT('Ctrl Pts',(56.8120730583125,20.1657844389894,9.52589841598972));
#23791=CARTESIAN_POINT('Ctrl Pts',(56.7807321222224,20.0996611701481,9.52107126168567));
#23792=CARTESIAN_POINT('Ctrl Pts',(56.7571878830396,20.0545334872926,9.5176574354516));
#23793=CARTESIAN_POINT('Ctrl Pts',(56.6700747495815,19.902079111676,9.50571436899782));
#23794=CARTESIAN_POINT('Ctrl Pts',(56.5981889535416,19.7998469853912,9.49695541440072));
#23795=CARTESIAN_POINT('Ctrl Pts',(56.4622906643107,19.6406259759884,9.48241776307868));
#23796=CARTESIAN_POINT('Ctrl Pts',(56.4032925020193,19.5798009732569,9.47660656345379));
#23797=CARTESIAN_POINT('Ctrl Pts',(56.3328967828005,19.5159103847815,9.47036380594232));
#23798=CARTESIAN_POINT('Ctrl Pts',(56.3251374133022,19.5089779791453,9.46968449539547));
#23799=CARTESIAN_POINT('Ctrl Pts',(56.3133527839832,19.4986139754389,9.46866643641604));
#23800=CARTESIAN_POINT('Ctrl Pts',(56.3093676817323,19.4951372801671,9.4683244905446));
#23801=CARTESIAN_POINT('Ctrl Pts',(56.302205113131,19.4889384821466,9.46771411850456));
#23802=CARTESIAN_POINT('Ctrl Pts',(56.2990328770418,19.4862104991774,9.46744526448588));
#23803=CARTESIAN_POINT('Ctrl Pts',(56.2920963941728,19.4802832916158,9.46686059499662));
#23804=CARTESIAN_POINT('Ctrl Pts',(56.2883288450662,19.4770880676076,9.46654507047809));
#23805=CARTESIAN_POINT('Ctrl Pts',(56.2776108833798,19.4680665008374,9.46565309748884));
#23806=CARTESIAN_POINT('Ctrl Pts',(56.2706324445029,19.4622734269091,9.46507901135552));
#23807=CARTESIAN_POINT('Ctrl Pts',(56.2252697957215,19.4251357884157,9.46138831049852));
#23808=CARTESIAN_POINT('Ctrl Pts',(56.18576485171,19.3951803885339,9.45836278077961));
#23809=CARTESIAN_POINT('Ctrl Pts',(56.026363813878,19.2834152898498,9.44669648244644));
#23810=CARTESIAN_POINT('Ctrl Pts',(55.8988040469977,19.2133151330815,9.43848216740319));
#23811=CARTESIAN_POINT('Ctrl Pts',(55.6799441041773,19.1224652253405,9.42455722871241));
#23812=CARTESIAN_POINT('Ctrl Pts',(55.5928087026705,19.093160864219,9.4190589646045));
#23813=CARTESIAN_POINT('Ctrl Pts',(55.4893983604155,19.0661583114225,9.41242120676643));
#23814=CARTESIAN_POINT('Ctrl Pts',(55.4747825213292,19.0625181369568,9.41148067931672));
#23815=CARTESIAN_POINT('Ctrl Pts',(55.4508811319091,19.0568520228991,9.409938154152));
#23816=CARTESIAN_POINT('Ctrl Pts',(55.4416196845429,19.0547262647087,9.40933936011487));
#23817=CARTESIAN_POINT('Ctrl Pts',(55.4250312350394,19.0510433260266,9.40826475000625));
#23818=CARTESIAN_POINT('Ctrl Pts',(55.4177099370897,19.0494610812033,9.40778974598518));
#23819=CARTESIAN_POINT('Ctrl Pts',(55.4021805079563,19.0461963752178,9.406780587133));
#23820=CARTESIAN_POINT('Ctrl Pts',(55.3939703598776,19.0445243245702,9.40624610997406));
#23821=CARTESIAN_POINT('Ctrl Pts',(55.3719955131262,19.0401930102414,9.40481289532779));
#23822=CARTESIAN_POINT('Ctrl Pts',(55.3582131057903,19.0376270861318,9.4039112105417));
#23823=CARTESIAN_POINT('Ctrl Pts',(55.290034822155,19.0256762374187,9.39943622337279));
#23824=CARTESIAN_POINT('Ctrl Pts',(55.2352973079836,19.0184075322534,9.39579680434988));
#23825=CARTESIAN_POINT('Ctrl Pts',(54.9702166105591,18.9943446939053,9.37793664448879));
#23826=CARTESIAN_POINT('Ctrl Pts',(54.758452837742,19.0087263861018,9.36277444052429));
#23827=CARTESIAN_POINT('Ctrl Pts',(54.526047721561,19.062177553013,9.34675778972842));
#23828=CARTESIAN_POINT('Ctrl Pts',(54.4993272457785,19.068908708993,9.34492908193437));
#23829=CARTESIAN_POINT('Ctrl Pts',(54.4651199828682,19.0782836907694,9.34261183692565));
#23830=CARTESIAN_POINT('Ctrl Pts',(54.4574990705697,19.0804211523044,9.3420971254225));
#23831=CARTESIAN_POINT('Ctrl Pts',(54.4453853740963,19.0838966232884,9.34128165065329));
#23832=CARTESIAN_POINT('Ctrl Pts',(54.4408843317689,19.0852051796202,9.34097923820133));
#23833=CARTESIAN_POINT('Ctrl Pts',(54.432331295327,19.087724473857,9.34040576365606));
#23834=CARTESIAN_POINT('Ctrl Pts',(54.4282785855041,19.0889322171496,9.34013454503861));
#23835=CARTESIAN_POINT('Ctrl Pts',(54.4187732929073,19.0917978212293,9.3394995799105));
#23836=CARTESIAN_POINT('Ctrl Pts',(54.4133239375802,19.0934661713425,9.33913644683079));
#23837=CARTESIAN_POINT('Ctrl Pts',(54.3955362568687,19.0989954541472,9.33795380122264));
#23838=CARTESIAN_POINT('Ctrl Pts',(54.3832280035083,19.1029530777621,9.33713970004766));
#23839=CARTESIAN_POINT('Ctrl Pts',(54.3539766718718,19.1126734099067,9.33521312505988));
#23840=CARTESIAN_POINT('Ctrl Pts',(54.3370706999954,19.1185450872518,9.33410624872874));
#23841=CARTESIAN_POINT('Ctrl Pts',(54.2746681863858,19.1411639326497,9.33003722157717));
#23842=CARTESIAN_POINT('Ctrl Pts',(54.2297050930297,19.1593413760665,9.32713821286093));
#23843=CARTESIAN_POINT('Ctrl Pts',(54.0322479865603,19.2476729732111,9.31437116845775));
#23844=CARTESIAN_POINT('Ctrl Pts',(53.8883145717822,19.3352622335131,9.30490591190842));
#23845=CARTESIAN_POINT('Ctrl Pts',(53.7173519639219,19.4714656912236,9.29175165587053));
#23846=CARTESIAN_POINT('Ctrl Pts',(53.6788829729788,19.5045896020782,9.28865025264508));
#23847=CARTESIAN_POINT('Ctrl Pts',(53.631310531202,19.5488215930287,9.28460274158093));
#23848=CARTESIAN_POINT('Ctrl Pts',(53.6210040864466,19.5586118202514,9.28371244538345));
#23849=CARTESIAN_POINT('Ctrl Pts',(53.604759610295,19.5743763663046,9.28228713331507));
#23850=CARTESIAN_POINT('Ctrl Pts',(53.5987531366276,19.5802797055828,9.28175520201736));
#23851=CARTESIAN_POINT('Ctrl Pts',(53.5880110719228,19.590971900264,9.28079488667754));
#23852=CARTESIAN_POINT('Ctrl Pts',(53.5832619840666,19.595747062939,9.28036711066229));
#23853=CARTESIAN_POINT('Ctrl Pts',(53.5735302105996,19.6056318859842,9.2794838011594));
#23854=CARTESIAN_POINT('Ctrl Pts',(53.5685505895157,19.6107444149851,9.27902814253846));
#23855=CARTESIAN_POINT('Ctrl Pts',(53.5540656858923,19.6257764851855,9.27769180155567));
#23856=CARTESIAN_POINT('Ctrl Pts',(53.5446354701373,19.635767476224,9.27680789832642));
#23857=CARTESIAN_POINT('Ctrl Pts',(53.4970643361312,19.6872220740788,9.27227656298673));
#23858=CARTESIAN_POINT('Ctrl Pts',(53.4605924361625,19.7301871011363,9.26855988781367));
#23859=CARTESIAN_POINT('Ctrl Pts',(53.3686124024927,19.8483375392624,9.25850428449512));
#23860=CARTESIAN_POINT('Ctrl Pts',(53.3164878807583,19.9259722658519,9.25205664760387));
#23861=CARTESIAN_POINT('Ctrl Pts',(53.2045285705031,20.1210205292247,9.23639150700404));
#23862=CARTESIAN_POINT('Ctrl Pts',(53.1504939919096,20.2412801941238,9.2271449203542));
#23863=CARTESIAN_POINT('Ctrl Pts',(53.1038361262805,20.3804653685814,9.21742896424449));
#23864=CARTESIAN_POINT('Ctrl Pts',(53.0991503163124,20.3949949508408,9.21642649266329));
#23865=CARTESIAN_POINT('Ctrl Pts',(53.0927757414616,20.4155665105,9.21502510022441));
#23866=CARTESIAN_POINT('Ctrl Pts',(53.0909480986891,20.4215644230553,9.21461864401671));
#23867=CARTESIAN_POINT('Ctrl Pts',(53.0879187286948,20.4316768998494,9.21393707138117));
#23868=CARTESIAN_POINT('Ctrl Pts',(53.0867019378591,20.4357868657837,9.2136610921622));
#23869=CARTESIAN_POINT('Ctrl Pts',(53.0842448293616,20.4441856246199,9.21309926909644));
#23870=CARTESIAN_POINT('Ctrl Pts',(53.0830056479758,20.4484747068629,9.21281349154791));
#23871=CARTESIAN_POINT('Ctrl Pts',(53.0798854177719,20.4594120879097,9.21208754622422));
#23872=CARTESIAN_POINT('Ctrl Pts',(53.0780244728101,20.4660661315871,9.21164853004105));
#23873=CARTESIAN_POINT('Ctrl Pts',(53.074059906336,20.4805312784615,9.21069959286802));
#23874=CARTESIAN_POINT('Ctrl Pts',(53.0719691400743,20.4883458147624,9.21019037325148));
#23875=CARTESIAN_POINT('Ctrl Pts',(53.0660136007062,20.511160455891,9.20871309087908));
#23876=CARTESIAN_POINT('Ctrl Pts',(53.0622758466901,20.5261934678134,9.20775147361118));
#23877=CARTESIAN_POINT('Ctrl Pts',(53.0233269900749,20.6910196695038,9.19732134383069));
#23878=CARTESIAN_POINT('Ctrl Pts',(53.0053837347156,20.8443743993901,9.188605506415));
#23879=CARTESIAN_POINT('Ctrl Pts',(53.0052507447458,20.9982762938427,9.17962824983008));
#23880=CARTESIAN_POINT('Ctrl Pts',(53.0052507434434,20.9982778017065,9.17962816187482));
#23881=CARTESIAN_POINT('Ctrl Pts',(53.0051828401937,21.0769272565001,9.1750404572398));
#23882=CARTESIAN_POINT('Ctrl Pts',(53.0097664109837,21.1555076732957,9.17040293054525));
#23883=CARTESIAN_POINT('Ctrl Pts',(53.0230355497044,21.2680305353932,9.1635329928163));
#23884=CARTESIAN_POINT('Ctrl Pts',(53.0279907401557,21.3023376729557,9.16140790578901));
#23885=CARTESIAN_POINT('Ctrl Pts',(53.0358351204672,21.3481726671077,9.1585194906103));
#23886=CARTESIAN_POINT('Ctrl Pts',(53.0379372937375,21.3598302479825,9.15778056533338));
#23887=CARTESIAN_POINT('Ctrl Pts',(53.0416739774596,21.3795448960094,9.15652332754926));
#23888=CARTESIAN_POINT('Ctrl Pts',(53.0432547111062,21.3876119319661,9.15600671209537));
#23889=CARTESIAN_POINT('Ctrl Pts',(53.0462742901041,21.4025325483763,9.15504706849639));
#23890=CARTESIAN_POINT('Ctrl Pts',(53.0476994550759,21.4093887910904,9.15460448058297));
#23891=CARTESIAN_POINT('Ctrl Pts',(53.0507238080268,21.4235634612059,9.15368605190557));
#23892=CARTESIAN_POINT('Ctrl Pts',(53.0523281760702,21.4308806586773,9.15321005217137));
#23893=CARTESIAN_POINT('Ctrl Pts',(53.0560626777143,21.4474658436589,9.15212677146438));
#23894=CARTESIAN_POINT('Ctrl Pts',(53.0582179352971,21.4567279302136,9.15151869424538));
#23895=CARTESIAN_POINT('Ctrl Pts',(53.0639635059175,21.4806431701988,9.14994037836016));
#23896=CARTESIAN_POINT('Ctrl Pts',(53.0676539226297,21.4952714205266,9.14896694714848));
#23897=CARTESIAN_POINT('Ctrl Pts',(53.0951880963049,21.5994172485215,9.14197780468443));
#23898=CARTESIAN_POINT('Ctrl Pts',(53.1250729235694,21.6872070146052,9.13576682073755));
#23899=CARTESIAN_POINT('Ctrl Pts',(53.1897511065282,21.8411649675577,9.12431160868321));
#23900=CARTESIAN_POINT('Ctrl Pts',(53.2223698334615,21.9080691297876,9.11912867220464));
#23901=CARTESIAN_POINT('Ctrl Pts',(53.2927277785203,22.0339879852313,9.10906759369945));
#23902=CARTESIAN_POINT('Ctrl Pts',(53.329992224216,22.0931534472244,9.10419720451516));
#23903=CARTESIAN_POINT('Ctrl Pts',(53.3987865316909,22.1906241492388,9.0960440760314));
#23904=CARTESIAN_POINT('Ctrl Pts',(53.4287807407972,22.2299355218696,9.09271710116968));
#23905=CARTESIAN_POINT('Ctrl Pts',(53.4659908337132,22.2751181167062,9.08888366975091));
#23906=CARTESIAN_POINT('Ctrl Pts',(53.4718226129579,22.2821014839455,9.08829090823107));
#23907=CARTESIAN_POINT('Ctrl Pts',(53.4808983220537,22.2928194451876,9.0873810520243));
#23908=CARTESIAN_POINT('Ctrl Pts',(53.4841086146754,22.2965821744037,9.08706161268604));
#23909=CARTESIAN_POINT('Ctrl Pts',(53.4900599664645,22.3035053349849,9.08647389584551));
#23910=CARTESIAN_POINT('Ctrl Pts',(53.492796956745,22.3066690668194,9.08620534050696));
#23911=CARTESIAN_POINT('Ctrl Pts',(53.4990113259303,22.3138068528042,9.08559946513332));
#23912=CARTESIAN_POINT('Ctrl Pts',(53.5024945385296,22.3177757170984,9.08526258312509));
#23913=CARTESIAN_POINT('Ctrl Pts',(53.5128631108908,22.3294957396674,9.08426762781139));
#23914=CARTESIAN_POINT('Ctrl Pts',(53.5197933103367,22.3372072447988,9.083612780022));
#23915=CARTESIAN_POINT('Ctrl Pts',(53.5816659592633,22.4049849305818,9.07785180140453));
#23916=CARTESIAN_POINT('Ctrl Pts',(53.6401844158498,22.4616973084398,9.07299206584844));
#23917=CARTESIAN_POINT('Ctrl Pts',(53.7823129006819,22.5834926657165,9.06200781416631));
#23918=CARTESIAN_POINT('Ctrl Pts',(53.8679585648431,22.6458109754695,9.05595091571441));
#23919=CARTESIAN_POINT('Ctrl Pts',(54.0136298890076,22.7350318370136,9.04593301661193));
#23920=CARTESIAN_POINT('Ctrl Pts',(54.0707435092103,22.7662793769604,9.04207055924135));
#23921=CARTESIAN_POINT('Ctrl Pts',(54.1647973677823,22.8119113274246,9.03572091598468));
#23922=CARTESIAN_POINT('Ctrl Pts',(54.2008177053333,22.8280846341323,9.03329202274851));
#23923=CARTESIAN_POINT('Ctrl Pts',(54.2487939292743,22.8479372118482,9.03004930153753));
#23924=CARTESIAN_POINT('Ctrl Pts',(54.2603395659209,22.85258871062,9.029268383939));
#23925=CARTESIAN_POINT('Ctrl Pts',(54.2784532929095,22.8596900384525,9.02804204657741));
#23926=CARTESIAN_POINT('Ctrl Pts',(54.2849921800722,22.8622138719923,9.0275991141178));
#23927=CARTESIAN_POINT('Ctrl Pts',(54.2985389715068,22.8673606983638,9.0266809252215));
#23928=CARTESIAN_POINT('Ctrl Pts',(54.3055485955028,22.8699788224949,9.02620551483901));
#23929=CARTESIAN_POINT('Ctrl Pts',(54.3214224244978,22.8758062023133,9.02512814548741));
#23930=CARTESIAN_POINT('Ctrl Pts',(54.3302949333851,22.8789921642515,9.02452542386294));
#23931=CARTESIAN_POINT('Ctrl Pts',(54.3531673676187,22.8870226738543,9.02297013373542));
#23932=CARTESIAN_POINT('Ctrl Pts',(54.3671990801259,22.8917742999904,9.02201452577132));
#23933=CARTESIAN_POINT('Ctrl Pts',(54.4615267196234,22.9225500590346,9.01557943611792));
#23934=CARTESIAN_POINT('Ctrl Pts',(54.5433412650726,22.9436078897621,9.00993908507125));
#23935=CARTESIAN_POINT('Ctrl Pts',(54.7756036005714,22.9879126892308,8.9937830938481));
#23936=CARTESIAN_POINT('Ctrl Pts',(54.927726568877,22.9992303610272,8.9830021449236));
#23937=CARTESIAN_POINT('Ctrl Pts',(55.1079515180691,22.9920281687318,8.9706680415368));
#23938=CARTESIAN_POINT('Ctrl Pts',(55.1362237077551,22.990294637996,8.96874771432807));
#23939=CARTESIAN_POINT('Ctrl Pts',(55.1644483561882,22.987959833761,8.96685094802472));
#23940=CARTESIAN_POINT('Ctrl Pts',(55.1644479310504,22.9879598689293,8.81003518437327));
#23941=CARTESIAN_POINT('Ctrl Pts',(55.0602828573514,22.9965766076901,8.81729550578455));
#23942=CARTESIAN_POINT('Ctrl Pts',(54.9555267627957,22.9969994905233,8.82464776415277));
#23943=CARTESIAN_POINT('Ctrl Pts',(54.8001413184913,22.9853714186208,8.83530728819776));
#23944=CARTESIAN_POINT('Ctrl Pts',(54.7493015405694,22.9795945148798,8.83875314450029));
#23945=CARTESIAN_POINT('Ctrl Pts',(54.6896973386332,22.9704881166276,8.84270234442929));
#23946=CARTESIAN_POINT('Ctrl Pts',(54.6806684719506,22.9690450838717,8.84329808716922));
#23947=CARTESIAN_POINT('Ctrl Pts',(54.6667607446777,22.9667241108439,8.84421158266041));
#23948=CARTESIAN_POINT('Ctrl Pts',(54.6618748415839,22.965890004045,8.84453170695718));
#23949=CARTESIAN_POINT('Ctrl Pts',(54.6528715016605,22.96431842232,8.84512007622143));
#23950=CARTESIAN_POINT('Ctrl Pts',(54.6487532950705,22.9635862118844,8.84538860362594));
#23951=CARTESIAN_POINT('Ctrl Pts',(54.6394532587541,22.9619024861104,8.8459936798834));
#23952=CARTESIAN_POINT('Ctrl Pts',(54.6342728862875,22.9609433947621,8.84632979607078));
#23953=CARTESIAN_POINT('Ctrl Pts',(54.620917803691,22.9584160778968,8.84719405592738));
#23954=CARTESIAN_POINT('Ctrl Pts',(54.6127489034824,22.9568171707334,8.84772051613693));
#23955=CARTESIAN_POINT('Ctrl Pts',(54.5614680601946,22.9464462139486,8.85101304504314));
#23956=CARTESIAN_POINT('Ctrl Pts',(54.5186426363149,22.9363003043483,8.85370774557413));
#23957=CARTESIAN_POINT('Ctrl Pts',(54.2892830923984,22.8738805644487,8.86801215552247));
#23958=CARTESIAN_POINT('Ctrl Pts',(54.1107798452838,22.7960643456084,8.8787848129137));
#23959=CARTESIAN_POINT('Ctrl Pts',(53.9006595602953,22.6653424175838,8.89365530736729));
#23960=CARTESIAN_POINT('Ctrl Pts',(53.8562045081614,22.6351286997452,8.89693644209995));
#23961=CARTESIAN_POINT('Ctrl Pts',(53.8018559420355,22.5948891945372,8.90115189208636));
#23962=CARTESIAN_POINT('Ctrl Pts',(53.7907729594592,22.5865026553504,8.9020226404251));
#23963=CARTESIAN_POINT('Ctrl Pts',(53.7731726779511,22.5728928821754,8.90342382966811));
#23964=CARTESIAN_POINT('Ctrl Pts',(53.7665988445046,22.5677432452763,8.90395136661294));
#23965=CARTESIAN_POINT('Ctrl Pts',(53.7541879416509,22.5578947416397,8.90495539464881));
#23966=CARTESIAN_POINT('Ctrl Pts',(53.7483446221371,22.5532039541899,8.90543155783345));
#23967=CARTESIAN_POINT('Ctrl Pts',(53.7351190720194,22.5424639023697,8.90651723595808));
#23968=CARTESIAN_POINT('Ctrl Pts',(53.7277535925301,22.5363943912707,8.90712756176496));
#23969=CARTESIAN_POINT('Ctrl Pts',(53.7087675593357,22.5205188384391,8.90871582505917));
#23970=CARTESIAN_POINT('Ctrl Pts',(53.6972152386696,22.5106325159566,8.90969702322558));
#23971=CARTESIAN_POINT('Ctrl Pts',(53.61295242649,22.4368360558758,8.91696538760889));
#23972=CARTESIAN_POINT('Ctrl Pts',(53.544877953502,22.3678500138841,8.92346660530846));
#23973=CARTESIAN_POINT('Ctrl Pts',(53.3908566855825,22.1872056370252,8.93978124369797));
#23974=CARTESIAN_POINT('Ctrl Pts',(53.3112009007468,22.0708663402775,8.94973433659892));
#23975=CARTESIAN_POINT('Ctrl Pts',(53.221210813,21.9040632106936,8.96268211225823));
#23976=CARTESIAN_POINT('Ctrl Pts',(53.1995704370656,21.8601601820237,8.96597427577031));
#23977=CARTESIAN_POINT('Ctrl Pts',(53.1758700770358,21.8072541502299,8.9697705611805));
#23978=CARTESIAN_POINT('Ctrl Pts',(53.1722313380716,21.7989812043107,8.97035933823313));
#23979=CARTESIAN_POINT('Ctrl Pts',(53.1666938807424,21.7861555577526,8.97126433156741));
#23980=CARTESIAN_POINT('Ctrl Pts',(53.1647556669086,21.7816201935892,8.97158285507234));
#23981=CARTESIAN_POINT('Ctrl Pts',(53.161204803451,21.773225247675,8.97216961544013));
#23982=CARTESIAN_POINT('Ctrl Pts',(53.1595874814217,21.769367805741,8.97243812449693));
#23983=CARTESIAN_POINT('Ctrl Pts',(53.1559506165795,21.7606165005101,8.97304480842484));
#23984=CARTESIAN_POINT('Ctrl Pts',(53.1539384181995,21.7557196749461,8.97338253902017));
#23985=CARTESIAN_POINT('Ctrl Pts',(53.1480173183783,21.7411454903343,8.97438270951778));
#23986=CARTESIAN_POINT('Ctrl Pts',(53.1441647733724,21.7314452225663,8.975041871926));
#23987=CARTESIAN_POINT('Ctrl Pts',(53.1081432205923,21.6386300482876,8.98129093449804));
#23988=CARTESIAN_POINT('Ctrl Pts',(53.0814979678095,21.5534659608479,8.98658486183109));
#23989=CARTESIAN_POINT('Ctrl Pts',(53.0239144387665,21.3142273391484,9.00097818624058));
#23990=CARTESIAN_POINT('Ctrl Pts',(53.0053248753638,21.1578692761744,9.00990128748095));
#23991=CARTESIAN_POINT('Ctrl Pts',(53.0052293593294,20.9570860933998,9.02204741246955));
#23992=CARTESIAN_POINT('Ctrl Pts',(53.0066552475153,20.9132372818238,9.02473792250262));
#23993=CARTESIAN_POINT('Ctrl Pts',(53.0104081689307,20.8560068112216,9.02831515112903));
#23994=CARTESIAN_POINT('Ctrl Pts',(53.0114278745639,20.8425497525654,9.02916102115691));
#23995=CARTESIAN_POINT('Ctrl Pts',(53.0132917939263,20.8208734678944,9.03053158129461));
#23996=CARTESIAN_POINT('Ctrl Pts',(53.0140506732978,20.8126471803633,9.03105359058605));
#23997=CARTESIAN_POINT('Ctrl Pts',(53.0155971192309,20.7969502583354,9.03205333699379));
#23998=CARTESIAN_POINT('Ctrl Pts',(53.0163758305301,20.789478878596,9.03253078768805));
#23999=CARTESIAN_POINT('Ctrl Pts',(53.0182574576288,20.772363720409,9.03362825038121));
#24000=CARTESIAN_POINT('Ctrl Pts',(53.0193885941512,20.7627232975127,9.03424914005485));
#24001=CARTESIAN_POINT('Ctrl Pts',(53.0231200578368,20.7328089729646,9.03618443642928));
#24002=CARTESIAN_POINT('Ctrl Pts',(53.0259616040053,20.7125670335537,9.03750638663736));
#24003=CARTESIAN_POINT('Ctrl Pts',(53.0412203424669,20.6148082734827,9.04395305057753));
#24004=CARTESIAN_POINT('Ctrl Pts',(53.0578937853662,20.5380355193413,9.04921004377207));
#24005=CARTESIAN_POINT('Ctrl Pts',(53.1026180129301,20.3782110807948,9.06055287102911));
#24006=CARTESIAN_POINT('Ctrl Pts',(53.131706174058,20.2956163725933,9.06665359953203));
#24007=CARTESIAN_POINT('Ctrl Pts',(53.2069383676496,20.1198169091956,9.07998962500898));
#24008=CARTESIAN_POINT('Ctrl Pts',(53.2551421990155,20.0277511130764,9.08720641913862));
#24009=CARTESIAN_POINT('Ctrl Pts',(53.3187703281887,19.9263386748042,9.095137869918));
#24010=CARTESIAN_POINT('Ctrl Pts',(53.3274073950845,19.9129324459384,9.09618578738727));
#24011=CARTESIAN_POINT('Ctrl Pts',(53.3397253454162,19.8943072902267,9.09763925968634));
#24012=CARTESIAN_POINT('Ctrl Pts',(53.3432716547882,19.8890006795793,9.09805310170421));
#24013=CARTESIAN_POINT('Ctrl Pts',(53.3490358974462,19.8804641837295,9.09871826494411));
#24014=CARTESIAN_POINT('Ctrl Pts',(53.351237947853,19.8772237053252,9.09897063046831));
#24015=CARTESIAN_POINT('Ctrl Pts',(53.3559043584173,19.8704000728906,9.09950173292386));
#24016=CARTESIAN_POINT('Ctrl Pts',(53.3583709140122,19.8668184529106,9.09978031321923));
#24017=CARTESIAN_POINT('Ctrl Pts',(53.3644798354237,19.858009657165,9.10046507889342));
#24018=CARTESIAN_POINT('Ctrl Pts',(53.368135606698,19.8527917554333,9.10087036319758));
#24019=CARTESIAN_POINT('Ctrl Pts',(53.3816959994845,19.8336329180438,9.10235757787664));
#24020=CARTESIAN_POINT('Ctrl Pts',(53.3917551078741,19.8198015331193,9.10342950350796));
#24021=CARTESIAN_POINT('Ctrl Pts',(53.4614684098847,19.726491766176,9.11066181109657));
#24022=CARTESIAN_POINT('Ctrl Pts',(53.5268191609118,19.6514282370647,9.11648802513467));
#24023=CARTESIAN_POINT('Ctrl Pts',(53.7150938578208,19.465271821967,9.13188635193029));
#24024=CARTESIAN_POINT('Ctrl Pts',(53.8466732065391,19.3640887318318,9.14137026587759));
#24025=CARTESIAN_POINT('Ctrl Pts',(54.0071731164936,19.2697526713335,9.15284991809959));
#24026=CARTESIAN_POINT('Ctrl Pts',(54.0252858912514,19.2594847329466,9.15414314593222));
#24027=CARTESIAN_POINT('Ctrl Pts',(54.053326964079,19.2441635297375,9.15614349624497));
#24028=CARTESIAN_POINT('Ctrl Pts',(54.0631427418637,19.2389065847947,9.15684339233716));
#24029=CARTESIAN_POINT('Ctrl Pts',(54.079183825811,19.2304876718798,9.15798687499016));
#24030=CARTESIAN_POINT('Ctrl Pts',(54.0853827165975,19.2272756759996,9.15842868861326));
#24031=CARTESIAN_POINT('Ctrl Pts',(54.0984192082412,19.2206073123949,9.15935775303313));
#24032=CARTESIAN_POINT('Ctrl Pts',(54.1052601029896,19.2171576696808,9.15984523032363));
#24033=CARTESIAN_POINT('Ctrl Pts',(54.1216447020866,19.2090134973813,9.16101275583091));
#24034=CARTESIAN_POINT('Ctrl Pts',(54.131206334138,19.2043557588323,9.16169407085541));
#24035=CARTESIAN_POINT('Ctrl Pts',(54.1639900314562,19.1887090489447,9.16403028173517));
#24036=CARTESIAN_POINT('Ctrl Pts',(54.1873861187847,19.1780927151107,9.16569790883912));
#24037=CARTESIAN_POINT('Ctrl Pts',(54.2441225484733,19.1536579360666,9.16974471321265));
#24038=CARTESIAN_POINT('Ctrl Pts',(54.2776446312157,19.1402870679403,9.17213804879462));
#24039=CARTESIAN_POINT('Ctrl Pts',(54.5030978819956,19.0573764559177,9.18825062367529));
#24040=CARTESIAN_POINT('Ctrl Pts',(54.7043218741102,19.0167578997439,9.20287874953262));
#24041=CARTESIAN_POINT('Ctrl Pts',(54.9419964826815,19.0058061787746,9.21895459278164));
#24042=CARTESIAN_POINT('Ctrl Pts',(54.9758475440011,19.0051089282962,9.22121179612446));
#24043=CARTESIAN_POINT('Ctrl Pts',(55.0181148569268,19.0053145138905,9.22397674756928));
#24044=CARTESIAN_POINT('Ctrl Pts',(55.0265273256589,19.005408652488,9.22452440895585));
#24045=CARTESIAN_POINT('Ctrl Pts',(55.0397845747207,19.0056408960003,9.22538303529213));
#24046=CARTESIAN_POINT('Ctrl Pts',(55.0446297622598,19.0057434383643,9.22569590737434));
#24047=CARTESIAN_POINT('Ctrl Pts',(55.0536265986851,19.0059666501789,9.22627507257861));
#24048=CARTESIAN_POINT('Ctrl Pts',(55.0577782077696,19.0060826267299,9.22654161280454));
#24049=CARTESIAN_POINT('Ctrl Pts',(55.0673205532176,19.0063790238281,9.22715262934781));
#24050=CARTESIAN_POINT('Ctrl Pts',(55.0727109370606,19.0065683420808,9.22749660650284));
#24051=CARTESIAN_POINT('Ctrl Pts',(55.0893840827649,19.0072216476622,9.22855710210797));
#24052=CARTESIAN_POINT('Ctrl Pts',(55.1006639554874,19.0077595883337,9.22926964201022));
#24053=CARTESIAN_POINT('Ctrl Pts',(55.2089600504383,19.0138464086931,9.23606858192566));
#24054=CARTESIAN_POINT('Ctrl Pts',(55.3054669931247,19.026382644399,9.2418063193963));
#24055=CARTESIAN_POINT('Ctrl Pts',(55.569411066746,19.0805043635134,9.25751740813453));
#24056=CARTESIAN_POINT('Ctrl Pts',(55.7329266713993,19.1368020982042,9.2673378305571));
#24057=CARTESIAN_POINT('Ctrl Pts',(55.9096594649216,19.2245627876558,9.27947415646563));
#24058=CARTESIAN_POINT('Ctrl Pts',(55.9319279169679,19.2361496925807,9.28103152929472));
#24059=CARTESIAN_POINT('Ctrl Pts',(55.9625446956151,19.2528221108306,9.28321503672277));
#24060=CARTESIAN_POINT('Ctrl Pts',(55.9710838239005,19.2575537113019,9.283828671662));
#24061=CARTESIAN_POINT('Ctrl Pts',(55.9857564375379,19.2658252814945,9.28489128324927));
#24062=CARTESIAN_POINT('Ctrl Pts',(55.9919064914131,19.2693356135167,9.28533919434151));
#24063=CARTESIAN_POINT('Ctrl Pts',(56.0046051289737,19.2766736723116,9.28626933447792));
#24064=CARTESIAN_POINT('Ctrl Pts',(56.0111508226025,19.2805061476687,9.28675172968762));
#24065=CARTESIAN_POINT('Ctrl Pts',(56.0264466318976,19.2895793200534,9.28788598116039));
#24066=CARTESIAN_POINT('Ctrl Pts',(56.0351786623749,19.2948499417669,9.28853891878499));
#24067=CARTESIAN_POINT('Ctrl Pts',(56.0635755020996,19.3122886870644,9.29068032205804));
#24068=CARTESIAN_POINT('Ctrl Pts',(56.0830685981246,19.3247314658245,9.29217882191706));
#24069=CARTESIAN_POINT('Ctrl Pts',(56.1855396128492,19.3926764901948,9.30021255750873));
#24070=CARTESIAN_POINT('Ctrl Pts',(56.2644679970332,19.4540024334536,9.30696572640259));
#24071=CARTESIAN_POINT('Ctrl Pts',(56.4146819816097,19.5899402971232,9.32095582761771));
#24072=CARTESIAN_POINT('Ctrl Pts',(56.4854495143307,19.6646976543961,9.32818029282559));
#24073=CARTESIAN_POINT('Ctrl Pts',(56.5952461737899,19.8002692940285,9.34024499217286));
#24074=CARTESIAN_POINT('Ctrl Pts',(56.6373235791965,19.8583617326098,9.34513336584363));
#24075=CARTESIAN_POINT('Ctrl Pts',(56.6817449859255,19.9272155372272,9.3505126760969));
#24076=CARTESIAN_POINT('Ctrl Pts',(56.6872373920234,19.9358746808047,9.35118199529146));
#24077=CARTESIAN_POINT('Ctrl Pts',(56.6954435004558,19.9490354347774,9.3521879943068));
#24078=CARTESIAN_POINT('Ctrl Pts',(56.6982064849786,19.9535058927523,9.35252776400843));
#24079=CARTESIAN_POINT('Ctrl Pts',(56.7031357264068,19.9615522456961,9.35313574879399));
#24080=CARTESIAN_POINT('Ctrl Pts',(56.7053084284988,19.9651240626677,9.35340437794755));
#24081=CARTESIAN_POINT('Ctrl Pts',(56.7100360130028,19.9729513004549,9.35399029717136));
#24082=CARTESIAN_POINT('Ctrl Pts',(56.7125862438962,19.9772094273434,9.35430728535708));
#24083=CARTESIAN_POINT('Ctrl Pts',(56.7198093019939,19.9893725465656,9.35520787173452));
#24084=CARTESIAN_POINT('Ctrl Pts',(56.724443547311,19.9973004713793,9.35578903394519));
#24085=CARTESIAN_POINT('Ctrl Pts',(56.7550141846342,20.0504373215417,9.359647385122));
#24086=CARTESIAN_POINT('Ctrl Pts',(56.7792273373102,20.0966201267629,9.36282367694648));
#24087=CARTESIAN_POINT('Ctrl Pts',(56.8730928926753,20.2941084295497,9.37589965084349));
#24088=CARTESIAN_POINT('Ctrl Pts',(56.9254674504142,20.4528783903085,9.38525702384606));
#24089=CARTESIAN_POINT('Ctrl Pts',(56.9708737014861,20.6845371791889,9.39928848378233));
#24090=CARTESIAN_POINT('Ctrl Pts',(56.9806682984673,20.7534001810688,9.4034961820481));
#24091=CARTESIAN_POINT('Ctrl Pts',(56.9881040195518,20.8366925274336,9.40869655404811));
#24092=CARTESIAN_POINT('Ctrl Pts',(56.9892101300842,20.850768751831,9.40957909534679));
#24093=CARTESIAN_POINT('Ctrl Pts',(56.9907908982071,20.8740474375635,9.41104522297326));
#24094=CARTESIAN_POINT('Ctrl Pts',(56.9913514034661,20.8832437081452,9.41162612101356));
#24095=CARTESIAN_POINT('Ctrl Pts',(56.9922505513398,20.8998950916761,9.41268115224679));
#24096=CARTESIAN_POINT('Ctrl Pts',(56.9926111063721,20.9073488895248,9.41315459065557));
#24097=CARTESIAN_POINT('Ctrl Pts',(56.9932956278294,20.9233615014235,9.41417423461002));
#24098=CARTESIAN_POINT('Ctrl Pts',(56.9936063114761,20.9319207046477,9.414720846234));
#24099=CARTESIAN_POINT('Ctrl Pts',(56.9943057091162,20.955350446462,9.41622158666618));
#24100=CARTESIAN_POINT('Ctrl Pts',(56.9945832108337,20.9702235124484,9.41717916670178));
#24101=CARTESIAN_POINT('Ctrl Pts',(56.9951983594208,21.0525634948495,9.42250881270515));
#24102=CARTESIAN_POINT('Ctrl Pts',(56.9922792850737,21.1200037188107,9.42698145556755));
#24103=CARTESIAN_POINT('Ctrl Pts',(56.9702222630708,21.3540497173227,9.44288238969973));
#24104=CARTESIAN_POINT('Ctrl Pts',(56.9335246377157,21.5182646825302,9.45477990699314));
#24105=CARTESIAN_POINT('Ctrl Pts',(56.8585773263293,21.726352881823,9.46994083902021));
#24106=CARTESIAN_POINT('Ctrl Pts',(56.8383963050628,21.7760143876414,9.47355864971153));
#24107=CARTESIAN_POINT('Ctrl Pts',(56.8126013935012,21.8328151662349,9.47764945802753));
#24108=CARTESIAN_POINT('Ctrl Pts',(56.8089117960508,21.8407990448001,9.47822333777473));
#24109=CARTESIAN_POINT('Ctrl Pts',(56.8028675354923,21.853654191791,9.47914523944525));
#24110=CARTESIAN_POINT('Ctrl Pts',(56.8005456969913,21.8585406364357,9.47949516971337));
#24111=CARTESIAN_POINT('Ctrl Pts',(56.796389314544,21.8671969610889,9.48011410321708));
#24112=CARTESIAN_POINT('Ctrl Pts',(56.7945627373398,21.870970563018,9.48038358664463));
#24113=CARTESIAN_POINT('Ctrl Pts',(56.7905975957533,21.8790968835913,9.4809631785986));
#24114=CARTESIAN_POINT('Ctrl Pts',(56.7884550541399,21.8834475656139,9.48127303670872));
#24115=CARTESIAN_POINT('Ctrl Pts',(56.7824443704109,21.8955414828093,9.48213325156417));
#24116=CARTESIAN_POINT('Ctrl Pts',(56.7785416088597,21.9032675312896,9.482681504577));
#24117=CARTESIAN_POINT('Ctrl Pts',(56.7555413856911,21.9480725402264,9.48585486500409));
#24118=CARTESIAN_POINT('Ctrl Pts',(56.7353335566076,21.9845735704633,9.48841581318161));
#24119=CARTESIAN_POINT('Ctrl Pts',(56.6140519481253,22.1882902985709,9.50272240661046));
#24120=CARTESIAN_POINT('Ctrl Pts',(56.4899865186897,22.3405789551896,9.51357470973993));
#24121=CARTESIAN_POINT('Ctrl Pts',(56.3057793110954,22.5089399864189,9.52855564836426));
#24122=CARTESIAN_POINT('Ctrl Pts',(56.2643431466358,22.5438248310436,9.53185864310612));
#24123=CARTESIAN_POINT('Ctrl Pts',(56.2101671787729,22.5857900182673,9.53612657646227));
#24124=CARTESIAN_POINT('Ctrl Pts',(56.1986976254285,22.5944775220362,9.53702734443431));
#24125=CARTESIAN_POINT('Ctrl Pts',(56.1802720054852,22.6081226613883,9.53847052018481));
#24126=CARTESIAN_POINT('Ctrl Pts',(56.1733762018089,22.6131611160572,9.53900977543551));
#24127=CARTESIAN_POINT('Ctrl Pts',(56.1603925859709,22.6225203656348,9.54002361770805));
#24128=CARTESIAN_POINT('Ctrl Pts',(56.1543124423563,22.6268515830938,9.54049779162503));
#24129=CARTESIAN_POINT('Ctrl Pts',(56.1406463943505,22.6364714724732,9.54156230616939));
#24130=CARTESIAN_POINT('Ctrl Pts',(56.133047775967,22.6417417000798,9.54215333693578));
#24131=CARTESIAN_POINT('Ctrl Pts',(56.1104648720599,22.6571732280104,9.543907498452));
#24132=CARTESIAN_POINT('Ctrl Pts',(56.0953789108245,22.6671833569129,9.54507627933058));
#24133=CARTESIAN_POINT('Ctrl Pts',(55.9759476215912,22.7441099185196,9.55430806931044));
#24134=CARTESIAN_POINT('Ctrl Pts',(55.8657252718189,22.8013614109527,9.56272876173517));
#24135=CARTESIAN_POINT('Ctrl Pts',(55.6246755141659,22.8993099311404,9.58078487022611));
#24136=CARTESIAN_POINT('Ctrl Pts',(55.4935003345567,22.9375391560412,9.59041185895706));
#24137=CARTESIAN_POINT('Ctrl Pts',(55.3335268172887,22.9668456738974,9.60132154369132));
#24138=CARTESIAN_POINT('Ctrl Pts',(55.3075121090441,22.9710805429602,9.60306913891539));
#24139=CARTESIAN_POINT('Ctrl Pts',(55.2737130777706,22.9758970902215,9.60529897098501));
#24140=CARTESIAN_POINT('Ctrl Pts',(55.2659999741732,22.9769502215919,9.60580509539952));
#24141=CARTESIAN_POINT('Ctrl Pts',(55.2536624194026,22.9785612530703,9.60661009217361));
#24142=CARTESIAN_POINT('Ctrl Pts',(55.249041931907,22.979148143117,9.60691054363731));
#24143=CARTESIAN_POINT('Ctrl Pts',(55.2402146710695,22.9802379713847,9.6074825339107));
#24144=CARTESIAN_POINT('Ctrl Pts',(55.2360083347193,22.9807436930951,9.60775421922156));
#24145=CARTESIAN_POINT('Ctrl Pts',(55.2260819607302,22.9819050576226,9.60839334167342));
#24146=CARTESIAN_POINT('Ctrl Pts',(55.2203605894581,22.9825493494483,9.60876014451398));
#24147=CARTESIAN_POINT('Ctrl Pts',(55.2014487809749,22.9845961559468,9.60996763573801));
#24148=CARTESIAN_POINT('Ctrl Pts',(55.1882468111938,22.9858919089266,9.61080259174365));
#24149=CARTESIAN_POINT('Ctrl Pts',(55.1715051708299,22.9873666187572,9.61185243912581));
#24150=CARTESIAN_POINT('Ctrl Pts',(55.1679771143424,22.9876679272289,9.61207317488924));
#24151=CARTESIAN_POINT('Ctrl Pts',(55.1644483514339,22.9879598341543,9.61229346745724));
#24152=CARTESIAN_POINT('Origin',(55.,21.,6.22095488139522));
#24153=CARTESIAN_POINT('',(55.1644484221209,22.9879598283069,10.5696416509586));
#24154=CARTESIAN_POINT('',(55.1644480736098,22.9879598571365,10.4094440176549));
#24155=CARTESIAN_POINT('',(55.1644483516311,22.987959834138,6.22095488139522));
#24156=CARTESIAN_POINT('Ctrl Pts',(55.1644484221208,22.9879598283069,10.5696416509586));
#24157=CARTESIAN_POINT('Ctrl Pts',(55.1795206323429,22.9867130218304,10.5687444671462));
#24158=CARTESIAN_POINT('Ctrl Pts',(55.1945828596467,22.9852944580563,10.5678435263383));
#24159=CARTESIAN_POINT('Ctrl Pts',(55.2696887042474,22.9773574861964,10.5633257816232));
#24160=CARTESIAN_POINT('Ctrl Pts',(55.3294208840686,22.9682874363899,10.5596505977628));
#24161=CARTESIAN_POINT('Ctrl Pts',(55.4027795667775,22.9537153912676,10.5549916129971));
#24162=CARTESIAN_POINT('Ctrl Pts',(55.416882237778,22.9507548262385,10.5540892908252));
#24163=CARTESIAN_POINT('Ctrl Pts',(55.4392160211955,22.9458130688504,10.5526491969457));
#24164=CARTESIAN_POINT('Ctrl Pts',(55.4474689046702,22.94393178583,10.5521146235002));
#24165=CARTESIAN_POINT('Ctrl Pts',(55.4629884365706,22.9402899708852,10.5511046811371));
#24166=CARTESIAN_POINT('Ctrl Pts',(55.4702576670761,22.9385409945568,10.5506296909739));
#24167=CARTESIAN_POINT('Ctrl Pts',(55.4866087990222,22.9345095317817,10.5495568096997));
#24168=CARTESIAN_POINT('Ctrl Pts',(55.495684756322,22.9322038891503,10.5489581815596));
#24169=CARTESIAN_POINT('Ctrl Pts',(55.5188760701109,22.9261382513339,10.5474204155609));
#24170=CARTESIAN_POINT('Ctrl Pts',(55.5329667740397,22.9222870072679,10.5464783523423));
#24171=CARTESIAN_POINT('Ctrl Pts',(55.6229356397672,22.8966316510767,10.5404124605316));
#24172=CARTESIAN_POINT('Ctrl Pts',(55.6974957710561,22.8704965375062,10.5351486458867));
#24173=CARTESIAN_POINT('Ctrl Pts',(55.915360154888,22.7792898405105,10.5190563825482));
#24174=CARTESIAN_POINT('Ctrl Pts',(56.0527105175792,22.7016316892603,10.5079004743152));
#24175=CARTESIAN_POINT('Ctrl Pts',(56.2207120192313,22.5784485813475,10.4936490590936));
#24176=CARTESIAN_POINT('Ctrl Pts',(56.2607416901066,22.546663875978,10.4902067664466));
#24177=CARTESIAN_POINT('Ctrl Pts',(56.3064438923021,22.5074201296362,10.486261242281));
#24178=CARTESIAN_POINT('Ctrl Pts',(56.3133369122406,22.5014184139045,10.4856657394375));
#24179=CARTESIAN_POINT('Ctrl Pts',(56.3239031081325,22.4920900356861,10.4847525803468));
#24180=CARTESIAN_POINT('Ctrl Pts',(56.3276054380052,22.4887968016458,10.4844325532266));
#24181=CARTESIAN_POINT('Ctrl Pts',(56.3344104174009,22.4826981810303,10.4838442841236));
#24182=CARTESIAN_POINT('Ctrl Pts',(56.3375164984436,22.4798968460925,10.4835757603014));
#24183=CARTESIAN_POINT('Ctrl Pts',(56.3445157414662,22.4735442815818,10.4829706188889));
#24184=CARTESIAN_POINT('Ctrl Pts',(56.3484036506588,22.4699873894902,10.4826344346083));
#24185=CARTESIAN_POINT('Ctrl Pts',(56.3583980814003,22.4607708697612,10.4817699709026));
#24186=CARTESIAN_POINT('Ctrl Pts',(56.3644834184551,22.4550882749749,10.4812433762019));
#24187=CARTESIAN_POINT('Ctrl Pts',(56.4025171414656,22.4191232954154,10.4779492019119));
#24188=CARTESIAN_POINT('Ctrl Pts',(56.4334940266845,22.3878259222307,10.4752530810785));
#24189=CARTESIAN_POINT('Ctrl Pts',(56.5950300672367,22.2134333008162,10.4609485298516));
#24190=CARTESIAN_POINT('Ctrl Pts',(56.7052575256727,22.0529248693865,10.4501768174887));
#24191=CARTESIAN_POINT('Ctrl Pts',(56.8143032085948,21.8307941653473,10.4353071999285));
#24192=CARTESIAN_POINT('Ctrl Pts',(56.8360223931457,21.7816239961098,10.4320259216238));
#24193=CARTESIAN_POINT('Ctrl Pts',(56.8608276689748,21.7187079973365,10.427810160613));
#24194=CARTESIAN_POINT('Ctrl Pts',(56.8657908748884,21.7057231714724,10.426939253867));
#24195=CARTESIAN_POINT('Ctrl Pts',(56.8735183803376,21.6848548813037,10.4255377824128));
#24196=CARTESIAN_POINT('Ctrl Pts',(56.8763696333598,21.6770039331303,10.4250101227268));
#24197=CARTESIAN_POINT('Ctrl Pts',(56.8816857318872,21.6620744277449,10.4240058426936));
#24198=CARTESIAN_POINT('Ctrl Pts',(56.8841601586861,21.6549994163107,10.4235295503243));
#24199=CARTESIAN_POINT('Ctrl Pts',(56.8896955994152,21.6388812496589,10.4224435509722));
#24200=CARTESIAN_POINT('Ctrl Pts',(56.8927316640792,21.6298297803117,10.4218330324798));
#24201=CARTESIAN_POINT('Ctrl Pts',(56.9004360851584,21.6063015862427,10.4202442081911));
#24202=CARTESIAN_POINT('Ctrl Pts',(56.9050039695012,21.591792854098,10.4192626389861));
#24203=CARTESIAN_POINT('Ctrl Pts',(56.9374546471015,21.484450704609,10.4119857704737));
#24204=CARTESIAN_POINT('Ctrl Pts',(56.9586996647495,21.3897609629342,10.4054758463642));
#24205=CARTESIAN_POINT('Ctrl Pts',(56.9936729643665,21.1549935069952,10.3891627511229));
#24206=CARTESIAN_POINT('Ctrl Pts',(56.9996371091365,21.0142836089884,10.3792213080346));
#24207=CARTESIAN_POINT('Ctrl Pts',(56.9876878621724,20.8253113976752,10.3662861095082));
#24208=CARTESIAN_POINT('Ctrl Pts',(56.9828076118112,20.7766303340642,10.3629954559046));
#24209=CARTESIAN_POINT('Ctrl Pts',(56.9749105119812,20.7192194297392,10.3592005228039));
#24210=CARTESIAN_POINT('Ctrl Pts',(56.9736179383067,20.7102734047097,10.358611674832));
#24211=CARTESIAN_POINT('Ctrl Pts',(56.9715259256716,20.6964585285444,10.3577065292089));
#24212=CARTESIAN_POINT('Ctrl Pts',(56.9707691772453,20.6915834767926,10.3573879242289));
#24213=CARTESIAN_POINT('Ctrl Pts',(56.9693371394543,20.6825786655285,10.356800976771));
#24214=CARTESIAN_POINT('Ctrl Pts',(56.9686669459429,20.6784482484599,10.3565323622129));
#24215=CARTESIAN_POINT('Ctrl Pts',(56.9671189111275,20.6690939561572,10.3559253875376));
#24216=CARTESIAN_POINT('Ctrl Pts',(56.9662332580555,20.6638714578548,10.3555874723663));
#24217=CARTESIAN_POINT('Ctrl Pts',(56.9635394435155,20.6483616751497,10.3545866156838));
#24218=CARTESIAN_POINT('Ctrl Pts',(56.9616712420815,20.6380848070395,10.3539269566416));
#24219=CARTESIAN_POINT('Ctrl Pts',(56.9428147412148,20.538794713725,10.3475835476879));
#24220=CARTESIAN_POINT('Ctrl Pts',(56.9198576660616,20.4510096883611,10.3422058741129));
#24221=CARTESIAN_POINT('Ctrl Pts',(56.876685017568,20.322426888312,10.3342765213955));
#24222=CARTESIAN_POINT('Ctrl Pts',(56.8609245646122,20.2802695960269,10.3316683798425));
#24223=CARTESIAN_POINT('Ctrl Pts',(56.7875311271255,20.1025264200261,10.3205118204389));
#24224=CARTESIAN_POINT('Ctrl Pts',(56.716411283723,19.9730379598587,10.3119351046345));
#24225=CARTESIAN_POINT('Ctrl Pts',(56.6216903735703,19.8383416063287,10.3017164801438));
#24226=CARTESIAN_POINT('Ctrl Pts',(56.611503261823,19.8242504099524,10.3006307288792));
#24227=CARTESIAN_POINT('Ctrl Pts',(56.5957049678437,19.8029886959157,10.2989658290496));
#24228=CARTESIAN_POINT('Ctrl Pts',(56.5902265806609,19.7957202051706,10.2983918315538));
#24229=CARTESIAN_POINT('Ctrl Pts',(56.5806065655438,19.7831368835164,10.2973895290677));
#24230=CARTESIAN_POINT('Ctrl Pts',(56.5764873660172,19.7778050309933,10.2969621109597));
#24231=CARTESIAN_POINT('Ctrl Pts',(56.5671715202991,19.7658721433801,10.2959993413764));
#24232=CARTESIAN_POINT('Ctrl Pts',(56.5619600509643,19.7592828943902,10.2954634058619));
#24233=CARTESIAN_POINT('Ctrl Pts',(56.5478777633252,19.7417069543017,10.2940221595638));
#24234=CARTESIAN_POINT('Ctrl Pts',(56.538931777746,19.7307813720725,10.29311384348));
#24235=CARTESIAN_POINT('Ctrl Pts',(56.4979618246229,19.6818154517599,10.2889856273645));
#24236=CARTESIAN_POINT('Ctrl Pts',(56.4646406759797,19.6448885296077,10.2857130586245));
#24237=CARTESIAN_POINT('Ctrl Pts',(56.4107092626002,19.5894360406048,10.280539297426));
#24238=CARTESIAN_POINT('Ctrl Pts',(56.3910324151128,19.5700279661225,10.2786752822605));
#24239=CARTESIAN_POINT('Ctrl Pts',(56.2532534487236,19.4396663285438,10.2657869899643));
#24240=CARTESIAN_POINT('Ctrl Pts',(56.1224320156335,19.3430680847122,10.2542856715688));
#24241=CARTESIAN_POINT('Ctrl Pts',(55.9364239473574,19.2379545658489,10.2396646000273));
#24242=CARTESIAN_POINT('Ctrl Pts',(55.8904946390295,19.2143028689359,10.2361843352079));
#24243=CARTESIAN_POINT('Ctrl Pts',(55.8353913880244,19.188582664532,10.2322012152433));
#24244=CARTESIAN_POINT('Ctrl Pts',(55.8270609777398,19.1847640149892,10.2316041123578));
#24245=CARTESIAN_POINT('Ctrl Pts',(55.8141812216076,19.1789670227817,10.2306890275811));
#24246=CARTESIAN_POINT('Ctrl Pts',(55.8096504479534,19.1769480755715,10.2303686594285));
#24247=CARTESIAN_POINT('Ctrl Pts',(55.8012855295126,19.1732579396096,10.2297800708355));
#24248=CARTESIAN_POINT('Ctrl Pts',(55.7974536788799,19.1715819171647,10.2295115662224));
#24249=CARTESIAN_POINT('Ctrl Pts',(55.7887880234012,19.1678240491753,10.2289068529175));
#24250=CARTESIAN_POINT('Ctrl Pts',(55.7839512425792,19.1657492779251,10.2285710748013));
#24251=CARTESIAN_POINT('Ctrl Pts',(55.7696382818747,19.1596765891433,10.2275824294941));
#24252=CARTESIAN_POINT('Ctrl Pts',(55.7601391582848,19.1557327167166,10.226932727311));
#24253=CARTESIAN_POINT('Ctrl Pts',(55.6477146370237,19.110072189154,10.2193141769951));
#24254=CARTESIAN_POINT('Ctrl Pts',(55.5414930669802,19.0769415107323,10.2128081317863));
#24255=CARTESIAN_POINT('Ctrl Pts',(55.4081136221418,19.0472779223273,10.204864708389));
#24256=CARTESIAN_POINT('Ctrl Pts',(55.3830710095716,19.0422112340185,10.2033831658793));
#24257=CARTESIAN_POINT('Ctrl Pts',(55.2133409011632,19.0112523695962,10.1933733896659));
#24258=CARTESIAN_POINT('Ctrl Pts',(55.0662933991303,19.0009429734723,10.1848118993532));
#24259=CARTESIAN_POINT('Ctrl Pts',(54.9023164468414,19.0075693860421,10.1746249037469));
#24260=CARTESIAN_POINT('Ctrl Pts',(54.8851863519837,19.0084830843205,10.1735535111708));
#24261=CARTESIAN_POINT('Ctrl Pts',(54.8590370273013,19.0102163518508,10.1719061401668));
#24262=CARTESIAN_POINT('Ctrl Pts',(54.8500077779817,19.0108766113974,10.1713351448596));
#24263=CARTESIAN_POINT('Ctrl Pts',(54.8342720875987,19.0121350267007,10.1703361425292));
#24264=CARTESIAN_POINT('Ctrl Pts',(54.8275635491583,19.0127057184144,10.1699090032749));
#24265=CARTESIAN_POINT('Ctrl Pts',(54.8124570060249,19.0140678913751,10.1689443045834));
#24266=CARTESIAN_POINT('Ctrl Pts',(54.8040609150552,19.0148786973984,10.1684061460766));
#24267=CARTESIAN_POINT('Ctrl Pts',(54.7814695203678,19.0172050551753,10.1669526448141));
#24268=CARTESIAN_POINT('Ctrl Pts',(54.767285140299,19.0188197607885,10.1660342073491));
#24269=CARTESIAN_POINT('Ctrl Pts',(54.7021219411451,19.0269471763794,10.1617872190869));
#24270=CARTESIAN_POINT('Ctrl Pts',(54.6513933994135,19.0352757387631,10.1584021969025));
#24271=CARTESIAN_POINT('Ctrl Pts',(54.576925039719,19.0504766652584,10.1533125699924));
#24272=CARTESIAN_POINT('Ctrl Pts',(54.552897539851,19.0558464650124,10.1516516808575));
#24273=CARTESIAN_POINT('Ctrl Pts',(54.3582897542213,19.1031368510996,10.1380509986044));
#24274=CARTESIAN_POINT('Ctrl Pts',(54.1938526201807,19.166970179225,10.1255320731254));
#24275=CARTESIAN_POINT('Ctrl Pts',(54.0164081440846,19.2644040326048,10.11178927966));
#24276=CARTESIAN_POINT('Ctrl Pts',(53.9931697346657,19.2777807156589,10.1099864901516));
#24277=CARTESIAN_POINT('Ctrl Pts',(53.955158792097,19.3006933354577,10.1070409938576));
#24278=CARTESIAN_POINT('Ctrl Pts',(53.9402305228355,19.3099630192671,10.1058850703593));
#24279=CARTESIAN_POINT('Ctrl Pts',(53.920000630192,19.3228982160019,10.1043218888375));
#24280=CARTESIAN_POINT('Ctrl Pts',(53.9145919133018,19.3263936183257,10.1039042757848));
#24281=CARTESIAN_POINT('Ctrl Pts',(53.9055466381482,19.3323014530859,10.1032065502335));
#24282=CARTESIAN_POINT('Ctrl Pts',(53.9019009354994,19.3346997116779,10.1029255156929));
#24283=CARTESIAN_POINT('Ctrl Pts',(53.8950055229073,19.3392682221652,10.102394366364));
#24284=CARTESIAN_POINT('Ctrl Pts',(53.8917542811157,19.3414360851828,10.1021440908646));
#24285=CARTESIAN_POINT('Ctrl Pts',(53.8832606969587,19.3471355635611,10.1014906435867));
#24286=CARTESIAN_POINT('Ctrl Pts',(53.8780286823287,19.3506826014594,10.1010884987161));
#24287=CARTESIAN_POINT('Ctrl Pts',(53.8599677074106,19.3630527319684,10.0997012668809));
#24288=CARTESIAN_POINT('Ctrl Pts',(53.8472248667372,19.3720013778125,10.0987242282678));
#24289=CARTESIAN_POINT('Ctrl Pts',(53.7329013840021,19.4543003992377,10.0899614386239));
#24290=CARTESIAN_POINT('Ctrl Pts',(53.6383232387173,19.5369308320924,10.0827211583798));
#24291=CARTESIAN_POINT('Ctrl Pts',(53.4813570455697,19.7025668355284,10.0694823491994));
#24292=CARTESIAN_POINT('Ctrl Pts',(53.4164842929297,19.7825907976671,10.0635136726485));
#24293=CARTESIAN_POINT('Ctrl Pts',(53.3381185465214,19.8961826723291,10.0552181243478));
#24294=CARTESIAN_POINT('Ctrl Pts',(53.318930495592,19.9256314558589,10.0530831176812));
#24295=CARTESIAN_POINT('Ctrl Pts',(53.2873491047164,19.9770198857956,10.0493716383957));
#24296=CARTESIAN_POINT('Ctrl Pts',(53.2745748685276,19.9987161090958,10.047808845111));
#24297=CARTESIAN_POINT('Ctrl Pts',(53.2570342330625,20.0298406051479,10.0455699812799));
#24298=CARTESIAN_POINT('Ctrl Pts',(53.2519264740627,20.0390744788529,10.0449061457732));
#24299=CARTESIAN_POINT('Ctrl Pts',(53.2432437327223,20.0550695963877,10.0437566828101));
#24300=CARTESIAN_POINT('Ctrl Pts',(53.2396338928623,20.061811737189,10.0432723058929));
#24301=CARTESIAN_POINT('Ctrl Pts',(53.2327939387063,20.0747652661179,10.0423418660736));
#24302=CARTESIAN_POINT('Ctrl Pts',(53.2295575732429,20.0809732390525,10.0418960331024));
#24303=CARTESIAN_POINT('Ctrl Pts',(53.222034574125,20.0955910183694,10.0408463627554));
#24304=CARTESIAN_POINT('Ctrl Pts',(53.2177748504954,20.1040144124698,10.0402415919609));
#24305=CARTESIAN_POINT('Ctrl Pts',(53.2032669627714,20.1332158833563,10.0381451522156));
#24306=CARTESIAN_POINT('Ctrl Pts',(53.1933214229174,20.1541414089725,10.0366430526732));
#24307=CARTESIAN_POINT('Ctrl Pts',(53.1179175798902,20.3201919967116,10.0247203447313));
#24308=CARTESIAN_POINT('Ctrl Pts',(53.0696946030046,20.4724821288948,10.013698302132));
#24309=CARTESIAN_POINT('Ctrl Pts',(53.0189524927518,20.7404309869774,9.99467756171033));
#24310=CARTESIAN_POINT('Ctrl Pts',(53.0073868960935,20.8536299421846,9.98677158445842));
#24311=CARTESIAN_POINT('Ctrl Pts',(53.0053397121424,20.9781466270934,9.97858796111114));
#24312=CARTESIAN_POINT('Ctrl Pts',(53.0052498563847,20.989086183223,9.97787341146361));
#24313=CARTESIAN_POINT('Ctrl Pts',(53.0052500701672,21.0053517588649,9.97681810964014));
#24314=CARTESIAN_POINT('Ctrl Pts',(53.005271467191,21.0106773538269,9.97647372476639));
#24315=CARTESIAN_POINT('Ctrl Pts',(53.0053477781925,21.0201891749405,9.97586074038109));
#24316=CARTESIAN_POINT('Ctrl Pts',(53.0053945424089,21.0243753639959,9.97559169711591));
#24317=CARTESIAN_POINT('Ctrl Pts',(53.0055248150456,21.0334727401625,9.97500861879199));
#24318=CARTESIAN_POINT('Ctrl Pts',(53.0056132834093,21.0383837683754,9.97469486200405));
#24319=CARTESIAN_POINT('Ctrl Pts',(53.0059138901869,21.0522306622226,9.97381291934913));
#24320=CARTESIAN_POINT('Ctrl Pts',(53.0061679540123,21.0611656352677,9.97324701239955));
#24321=CARTESIAN_POINT('Ctrl Pts',(53.0081287048847,21.116926820828,9.96973350786472));
#24322=CARTESIAN_POINT('Ctrl Pts',(53.0114249745165,21.1636865571769,9.96686720927864));
#24323=CARTESIAN_POINT('Ctrl Pts',(53.0289237777837,21.3287496035733,9.95689740860245));
#24324=CARTESIAN_POINT('Ctrl Pts',(53.0520686542674,21.4458535077955,9.95008391346948));
#24325=CARTESIAN_POINT('Ctrl Pts',(53.1191695401638,21.6751700030247,9.93617338895022));
#24326=CARTESIAN_POINT('Ctrl Pts',(53.1630945331575,21.7868611038043,9.92909871552594));
#24327=CARTESIAN_POINT('Ctrl Pts',(53.2237440030765,21.9078460916274,9.9206992918665));
#24328=CARTESIAN_POINT('Ctrl Pts',(53.2308827035187,21.9216799132677,9.91972774268353));
#24329=CARTESIAN_POINT('Ctrl Pts',(53.2427096524673,21.9439551883925,9.9181445034958));
#24330=CARTESIAN_POINT('Ctrl Pts',(53.2472986494408,21.9524488089649,9.91753630976153));
#24331=CARTESIAN_POINT('Ctrl Pts',(53.2555657261075,21.9674879814617,9.91645122619231));
#24332=CARTESIAN_POINT('Ctrl Pts',(53.2592194704208,21.9740467522273,9.91597521052456));
#24333=CARTESIAN_POINT('Ctrl Pts',(53.2669872538054,21.9878072549158,9.91497053167083));
#24334=CARTESIAN_POINT('Ctrl Pts',(53.2711093480965,21.995004252088,9.914441585486));
#24335=CARTESIAN_POINT('Ctrl Pts',(53.2821260186248,22.0139637249509,9.91303880089399));
#24336=CARTESIAN_POINT('Ctrl Pts',(53.2890964179815,22.025681416974,9.91216223075927));
#24337=CARTESIAN_POINT('Ctrl Pts',(53.3224969844937,22.0805420078166,9.9080120400027));
#24338=CARTESIAN_POINT('Ctrl Pts',(53.3504401813715,22.1227372973583,9.90468335658888));
#24339=CARTESIAN_POINT('Ctrl Pts',(53.4787493468056,22.3013441928268,9.88997482482784));
#24340=CARTESIAN_POINT('Ctrl Pts',(53.5946455249131,22.4257148737387,9.87801656279692));
#24341=CARTESIAN_POINT('Ctrl Pts',(53.778748061302,22.578761900371,9.86147012798136));
#24342=CARTESIAN_POINT('Ctrl Pts',(53.8350080032798,22.6207224563182,9.85669087045085));
#24343=CARTESIAN_POINT('Ctrl Pts',(53.9018666495572,22.6653032950413,9.85141571472648));
#24344=CARTESIAN_POINT('Ctrl Pts',(53.9104096301998,22.6709053702993,9.85074892228964));
#24345=CARTESIAN_POINT('Ctrl Pts',(53.923406096089,22.6792857620684,9.84974589911488));
#24346=CARTESIAN_POINT('Ctrl Pts',(53.9278279745852,22.6821124379992,9.84940660599922));
#24347=CARTESIAN_POINT('Ctrl Pts',(53.9357931019677,22.6871599586991,9.8487990462518));
#24348=CARTESIAN_POINT('Ctrl Pts',(53.9393322078173,22.689387132563,9.84853036912762));
#24349=CARTESIAN_POINT('Ctrl Pts',(53.9470949764504,22.6942382644822,9.84794383917477));
#24350=CARTESIAN_POINT('Ctrl Pts',(53.9513214480039,22.6968575607091,9.84762629166891));
#24351=CARTESIAN_POINT('Ctrl Pts',(53.9634128843393,22.7042886266924,9.84672279428538));
#24352=CARTESIAN_POINT('Ctrl Pts',(53.9713016001252,22.7090617839363,9.84613930428496));
#24353=CARTESIAN_POINT('Ctrl Pts',(54.0247096959407,22.7408731795927,9.84222706680628));
#24354=CARTESIAN_POINT('Ctrl Pts',(54.071261233634,22.766147218667,9.83900246623963));
#24355=CARTESIAN_POINT('Ctrl Pts',(54.2755937829782,22.866767682836,9.82539106138797));
#24356=CARTESIAN_POINT('Ctrl Pts',(54.4418937823907,22.9230473161335,9.81559329286339));
#24357=CARTESIAN_POINT('Ctrl Pts',(54.6736350687004,22.96882758614,9.8014815943344));
#24358=CARTESIAN_POINT('Ctrl Pts',(54.7343717481186,22.9779374731696,9.79775058576003));
#24359=CARTESIAN_POINT('Ctrl Pts',(54.8102854479758,22.9857640973899,9.79300114406748));
#24360=CARTESIAN_POINT('Ctrl Pts',(54.8251596057183,22.9871289538257,9.79206656556284));
#24361=CARTESIAN_POINT('Ctrl Pts',(54.8486871492846,22.9890216470555,9.79058138184153));
#24362=CARTESIAN_POINT('Ctrl Pts',(54.8573312479694,22.9896603515687,9.79003425405877));
#24363=CARTESIAN_POINT('Ctrl Pts',(54.8734196517449,22.9907437279569,9.78901309741248));
#24364=CARTESIAN_POINT('Ctrl Pts',(54.8808628446574,22.9912030310109,9.78853953585866));
#24365=CARTESIAN_POINT('Ctrl Pts',(54.8973816832914,22.9921294204338,9.78748596601456));
#24366=CARTESIAN_POINT('Ctrl Pts',(54.9064582550317,22.9925762429868,9.78690533354469));
#24367=CARTESIAN_POINT('Ctrl Pts',(54.932840624997,22.9936943393587,9.78521245670083));
#24368=CARTESIAN_POINT('Ctrl Pts',(54.9501521548108,22.9942022619015,9.78409514241426));
#24369=CARTESIAN_POINT('Ctrl Pts',(55.0332518502922,22.9955577134741,9.77869925214527));
#24370=CARTESIAN_POINT('Ctrl Pts',(55.0989923360642,22.9933745134514,9.77433085642924));
#24371=CARTESIAN_POINT('Ctrl Pts',(55.1644488239152,22.9879597950695,9.76988214123148));
#24372=CARTESIAN_POINT('',(53.0052507630248,20.9982552688642,9.82018160501716));
#24373=CARTESIAN_POINT('Ctrl Pts',(55.1644483514339,22.9879598341543,9.61229346745724));
#24374=CARTESIAN_POINT('Ctrl Pts',(55.1089206062989,22.9925532097293,9.6157599371205));
#24375=CARTESIAN_POINT('Ctrl Pts',(55.0532179574516,22.9948186209764,9.61911693483845));
#24376=CARTESIAN_POINT('Ctrl Pts',(54.828641597696,22.9945357235973,9.63242345076764));
#24377=CARTESIAN_POINT('Ctrl Pts',(54.6605077658855,22.972887588271,9.64192717472063));
#24378=CARTESIAN_POINT('Ctrl Pts',(54.4433596053057,22.9163151125312,9.655385059149));
#24379=CARTESIAN_POINT('Ctrl Pts',(54.3902270624372,22.9000758553173,9.65877059251745));
#24380=CARTESIAN_POINT('Ctrl Pts',(54.324178751614,22.8768332590493,9.66313075487158));
#24381=CARTESIAN_POINT('Ctrl Pts',(54.3105660854473,22.8718756107253,9.66403763047418));
#24382=CARTESIAN_POINT('Ctrl Pts',(54.2889951653645,22.8637524017234,9.66548837687345));
#24383=CARTESIAN_POINT('Ctrl Pts',(54.2810010440419,22.8606830432491,9.6660290373258));
#24384=CARTESIAN_POINT('Ctrl Pts',(54.2660774768651,22.85484257715,9.66704412518632));
#24385=CARTESIAN_POINT('Ctrl Pts',(54.2591433169166,22.8520838611207,9.66751812953735));
#24386=CARTESIAN_POINT('Ctrl Pts',(54.2438512023699,22.8459003606792,9.66856874639529));
#24387=CARTESIAN_POINT('Ctrl Pts',(54.2355007381463,22.8424576032854,9.66914595777952));
#24388=CARTESIAN_POINT('Ctrl Pts',(54.2112748962757,22.8322766442381,9.67083091807161));
#24389=CARTESIAN_POINT('Ctrl Pts',(54.1954634880096,22.8253892626325,9.67194370169674));
#24390=CARTESIAN_POINT('Ctrl Pts',(54.1597332848822,22.8092709348884,9.67448884756032));
#24391=CARTESIAN_POINT('Ctrl Pts',(54.1398738621292,22.7999145624565,9.67592536619496));
#24392=CARTESIAN_POINT('Ctrl Pts',(54.075498693003,22.7682767872788,9.68065495851626));
#24393=CARTESIAN_POINT('Ctrl Pts',(54.0316646955993,22.7446579972047,9.68399186181687));
#24394=CARTESIAN_POINT('Ctrl Pts',(53.8917238715625,22.6623553175447,9.69502423074494));
#24395=CARTESIAN_POINT('Ctrl Pts',(53.7996971950423,22.5971757649185,9.70290045213956));
#24396=CARTESIAN_POINT('Ctrl Pts',(53.6383817256847,22.4610701747593,9.7176004675061));
#24397=CARTESIAN_POINT('Ctrl Pts',(53.5678947914932,22.392052336322,9.72440856365455));
#24398=CARTESIAN_POINT('Ctrl Pts',(53.4958897048283,22.3102628852506,9.73156477600034));
#24399=CARTESIAN_POINT('Ctrl Pts',(53.4890509243693,22.3023707270529,9.73224659161516));
#24400=CARTESIAN_POINT('Ctrl Pts',(53.4788378960835,22.290395853582,9.73326759706016));
#24401=CARTESIAN_POINT('Ctrl Pts',(53.4754175403764,22.2863529572833,9.73361001206823));
#24402=CARTESIAN_POINT('Ctrl Pts',(53.4693241745386,22.2790920916492,9.73422081099481));
#24403=CARTESIAN_POINT('Ctrl Pts',(53.4666451578864,22.2758793010241,9.73448962624893));
#24404=CARTESIAN_POINT('Ctrl Pts',(53.4608297910738,22.2688604932783,9.73507373096043));
#24405=CARTESIAN_POINT('Ctrl Pts',(53.4576974469312,22.2650512714969,9.73538873269542));
#24406=CARTESIAN_POINT('Ctrl Pts',(53.4488667860125,22.2542308166217,9.73627800198762));
#24407=CARTESIAN_POINT('Ctrl Pts',(53.4432018427416,22.2471923243029,9.73684992900172));
#24408=CARTESIAN_POINT('Ctrl Pts',(53.4072078995929,22.2018437357967,9.74049501572245));
#24409=CARTESIAN_POINT('Ctrl Pts',(53.3782446198489,22.1624652273901,9.7434796563598));
#24410=CARTESIAN_POINT('Ctrl Pts',(53.3179491720982,22.0738406719841,9.74990688179934));
#24411=CARTESIAN_POINT('Ctrl Pts',(53.2872724473465,22.0242039986909,9.75332355518599));
#24412=CARTESIAN_POINT('Ctrl Pts',(53.2132284499993,21.8917417964281,9.76215722426305));
#24413=CARTESIAN_POINT('Ctrl Pts',(53.1734298107725,21.8070916795067,9.76753375079514));
#24414=CARTESIAN_POINT('Ctrl Pts',(53.1302470164264,21.6955133203145,9.77458230322623));
#24415=CARTESIAN_POINT('Ctrl Pts',(53.1212670338371,21.670878063763,9.77613578402236));
#24416=CARTESIAN_POINT('Ctrl Pts',(53.0925895358491,21.5871091488461,9.78142207023171));
#24417=CARTESIAN_POINT('Ctrl Pts',(53.0751798652793,21.5272363010452,9.7852081562648));
#24418=CARTESIAN_POINT('Ctrl Pts',(53.0570931710659,21.4520681206928,9.79001927144593));
#24419=CARTESIAN_POINT('Ctrl Pts',(53.0537489847629,21.4374465658683,9.79095770021957));
#24420=CARTESIAN_POINT('Ctrl Pts',(53.0487302609538,21.4143058255575,9.7924475560164));
#24421=CARTESIAN_POINT('Ctrl Pts',(53.0469458623405,21.405810846487,9.79299546702962));
#24422=CARTESIAN_POINT('Ctrl Pts',(53.0437322794341,21.3899996595754,9.79401720308837));
#24423=CARTESIAN_POINT('Ctrl Pts',(53.0422885452528,21.3826865381464,9.79449055457193));
#24424=CARTESIAN_POINT('Ctrl Pts',(53.0395434151779,21.3683591104237,9.79541948950454));
#24425=CARTESIAN_POINT('Ctrl Pts',(53.0382385893137,21.3613455694539,9.79587495579915));
#24426=CARTESIAN_POINT('Ctrl Pts',(53.035396065226,21.3455974512142,9.79689936333328));
#24427=CARTESIAN_POINT('Ctrl Pts',(53.0338789489189,21.336859358037,9.79746894882525));
#24428=CARTESIAN_POINT('Ctrl Pts',(53.0302122539574,21.3148713635623,9.79890528514081));
#24429=CARTESIAN_POINT('Ctrl Pts',(53.0281380792995,21.3016095010591,9.7997743925597));
#24430=CARTESIAN_POINT('Ctrl Pts',(53.0121645468032,21.1922597552295,9.8069645009715));
#24431=CARTESIAN_POINT('Ctrl Pts',(53.0051658710303,21.0953121951049,9.81350083438465));
#24432=CARTESIAN_POINT('Ctrl Pts',(53.0052507630248,20.9982552688642,9.82018160501716));
#24433=CARTESIAN_POINT('Ctrl Pts',(53.005250761363,20.9982571697515,9.82018147417241));
#24434=CARTESIAN_POINT('Ctrl Pts',(53.0053860238156,20.8434430824682,9.83083787131134));
#24435=CARTESIAN_POINT('Ctrl Pts',(53.0235426954589,20.6891709665941,9.84183516337205));
#24436=CARTESIAN_POINT('Ctrl Pts',(53.0643763109955,20.5174454261476,9.85374121521571));
#24437=CARTESIAN_POINT('Ctrl Pts',(53.0697377928547,20.4964268908962,9.85519157367019));
#24438=CARTESIAN_POINT('Ctrl Pts',(53.0793804526472,20.4610449399489,9.85761676212631));
#24439=CARTESIAN_POINT('Ctrl Pts',(53.0834825035105,20.4466350929466,9.85859983518176));
#24440=CARTESIAN_POINT('Ctrl Pts',(53.0894674436144,20.4264762700555,9.85996729988876));
#24441=CARTESIAN_POINT('Ctrl Pts',(53.0912145998974,20.4206879800285,9.86035903571322));
#24442=CARTESIAN_POINT('Ctrl Pts',(53.0942450750124,20.4108106469673,9.86102584278744));
#24443=CARTESIAN_POINT('Ctrl Pts',(53.0955152951957,20.4067176571241,9.86130166491522));
#24444=CARTESIAN_POINT('Ctrl Pts',(53.0979930902177,20.398823500335,9.86183265704579));
#24445=CARTESIAN_POINT('Ctrl Pts',(53.0991988795002,20.3950218437027,9.86208793311688));
#24446=CARTESIAN_POINT('Ctrl Pts',(53.1021317941633,20.3858701760786,9.86270145548229));
#24447=CARTESIAN_POINT('Ctrl Pts',(53.1038701622996,20.3805237633552,9.86305905073341));
#24448=CARTESIAN_POINT('Ctrl Pts',(53.1103601236829,20.3608469393985,9.86437233852564));
#24449=CARTESIAN_POINT('Ctrl Pts',(53.1152519030948,20.3465628258817,9.8653202186519));
#24450=CARTESIAN_POINT('Ctrl Pts',(53.1657864938792,20.2042914657335,9.87471913212622));
#24451=CARTESIAN_POINT('Ctrl Pts',(53.2242387153877,20.0812106073078,9.88252414508266));
#24452=CARTESIAN_POINT('Ctrl Pts',(53.3411262959643,19.8886266585373,9.89559882675533));
#24453=CARTESIAN_POINT('Ctrl Pts',(53.3925691237987,19.8154422408353,9.90080285863356));
#24454=CARTESIAN_POINT('Ctrl Pts',(53.4840972510739,19.7022214201233,9.90953560841896));
#24455=CARTESIAN_POINT('Ctrl Pts',(53.5212840302733,19.660004259427,9.91296507026975));
#24456=CARTESIAN_POINT('Ctrl Pts',(53.5697088256334,19.6095024649562,9.91732498794597));
#24457=CARTESIAN_POINT('Ctrl Pts',(53.5793175406992,19.5996866160219,9.91818519222063));
#24458=CARTESIAN_POINT('Ctrl Pts',(53.5940701712906,19.5849241055802,9.91949894094766));
#24459=CARTESIAN_POINT('Ctrl Pts',(53.5991406520325,19.5799043851572,9.91994925322498));
#24460=CARTESIAN_POINT('Ctrl Pts',(53.6095635406865,19.5696959817292,9.92087249906618));
#24461=CARTESIAN_POINT('Ctrl Pts',(53.614918316631,19.5645098885753,9.9213455346968));
#24462=CARTESIAN_POINT('Ctrl Pts',(53.6265685843059,19.5533524972712,9.92237202297392));
#24463=CARTESIAN_POINT('Ctrl Pts',(53.6328741996721,19.5473920374311,9.92292592979462));
#24464=CARTESIAN_POINT('Ctrl Pts',(53.6501741495146,19.5312514704063,9.92444122024709));
#24465=CARTESIAN_POINT('Ctrl Pts',(53.6612444418464,19.5211539616983,9.92540608458443));
#24466=CARTESIAN_POINT('Ctrl Pts',(53.7187789283916,19.4698506877642,9.93039739347665));
#24467=CARTESIAN_POINT('Ctrl Pts',(53.7670308384599,19.4307103486029,9.93450802850537));
#24468=CARTESIAN_POINT('Ctrl Pts',(53.9064253901271,19.3280399673356,9.94618629897363));
#24469=CARTESIAN_POINT('Ctrl Pts',(54.0011588937457,19.2697781889932,9.95391597867084));
#24470=CARTESIAN_POINT('Ctrl Pts',(54.1928137539631,19.1729154613862,9.96889323116746));
#24471=CARTESIAN_POINT('Ctrl Pts',(54.2889100932658,19.1334141071176,9.97611319234276));
#24472=CARTESIAN_POINT('Ctrl Pts',(54.4042529823624,19.0962097414256,9.98415504305193));
#24473=CARTESIAN_POINT('Ctrl Pts',(54.4209249920805,19.0910725412147,9.98530250060205));
#24474=CARTESIAN_POINT('Ctrl Pts',(54.4438229980657,19.0843445174885,9.98685610919408));
#24475=CARTESIAN_POINT('Ctrl Pts',(54.4499918846678,19.08256424854,9.98727245729615));
#24476=CARTESIAN_POINT('Ctrl Pts',(54.4603630901044,19.0796254095803,9.98796860420361));
#24477=CARTESIAN_POINT('Ctrl Pts',(54.4645607629922,19.0784507847483,9.98824931684867));
#24478=CARTESIAN_POINT('Ctrl Pts',(54.4725305573907,19.0762487600357,9.98878025381009));
#24479=CARTESIAN_POINT('Ctrl Pts',(54.4763018925294,19.0752186776087,9.98903063651271));
#24480=CARTESIAN_POINT('Ctrl Pts',(54.4861924097688,19.0725484554969,9.98968508874297));
#24481=CARTESIAN_POINT('Ctrl Pts',(54.4923164795569,19.0709263513597,9.99008812460039));
#24482=CARTESIAN_POINT('Ctrl Pts',(54.5136067372658,19.0653955333222,9.99148200599353));
#24483=CARTESIAN_POINT('Ctrl Pts',(54.5288116083312,19.0616361580112,9.99246469852505));
#24484=CARTESIAN_POINT('Ctrl Pts',(54.6645245657791,19.0297727230483,10.0011353315304));
#24485=CARTESIAN_POINT('Ctrl Pts',(54.7873775010952,19.0127557975032,10.0082920154952));
#24486=CARTESIAN_POINT('Ctrl Pts',(55.0148564092826,19.0025995962209,10.021502455981));
#24487=CARTESIAN_POINT('Ctrl Pts',(55.1188820686405,19.0060857456181,10.0275293599991));
#24488=CARTESIAN_POINT('Ctrl Pts',(55.2572868489808,19.0215964207877,10.0358993944882));
#24489=CARTESIAN_POINT('Ctrl Pts',(55.2923052708476,19.0264664535093,10.038046577975));
#24490=CARTESIAN_POINT('Ctrl Pts',(55.3521204360537,19.0364118887832,10.04177728671));
#24491=CARTESIAN_POINT('Ctrl Pts',(55.3769844281821,19.0410335063928,10.04334693439));
#24492=CARTESIAN_POINT('Ctrl Pts',(55.4121056169208,19.0482550804524,10.0455938145312));
#24493=CARTESIAN_POINT('Ctrl Pts',(55.4224409870032,19.0504659848866,10.0462586876158));
#24494=CARTESIAN_POINT('Ctrl Pts',(55.4402250100831,19.0544183361036,10.0474092695448));
#24495=CARTESIAN_POINT('Ctrl Pts',(55.4476821852852,19.0561207010941,10.0478937200156));
#24496=CARTESIAN_POINT('Ctrl Pts',(55.4619394883548,19.0594618279327,10.0488238271638));
#24497=CARTESIAN_POINT('Ctrl Pts',(55.468741161628,19.061093553186,10.049269251386));
#24498=CARTESIAN_POINT('Ctrl Pts',(55.4846819633904,19.0650065416677,10.0503172361939));
#24499=CARTESIAN_POINT('Ctrl Pts',(55.4938137320586,19.067316817889,10.0509207235476));
#24500=CARTESIAN_POINT('Ctrl Pts',(55.5252461387917,19.0755063169654,10.0530090419226));
#24501=CARTESIAN_POINT('Ctrl Pts',(55.5474602745024,19.0817073695127,10.054504199108));
#24502=CARTESIAN_POINT('Ctrl Pts',(55.7233456083865,19.1341094372841,10.0665011740046));
#24503=CARTESIAN_POINT('Ctrl Pts',(55.871011779508,19.1983076357173,10.0776153039086));
#24504=CARTESIAN_POINT('Ctrl Pts',(56.0984202367432,19.3317191182351,10.0960035705854));
#24505=CARTESIAN_POINT('Ctrl Pts',(56.1832943463724,19.3908055477882,10.1031885348333));
#24506=CARTESIAN_POINT('Ctrl Pts',(56.2766898483492,19.4672268303226,10.1111956422059));
#24507=CARTESIAN_POINT('Ctrl Pts',(56.290017170908,19.4784263714656,10.1123406075176));
#24508=CARTESIAN_POINT('Ctrl Pts',(56.3080535284524,19.4939904770871,10.113891418136));
#24509=CARTESIAN_POINT('Ctrl Pts',(56.3128901799333,19.4982050424308,10.11430741403));
#24510=CARTESIAN_POINT('Ctrl Pts',(56.3209780621825,19.505321602619,10.1150031372963));
#24511=CARTESIAN_POINT('Ctrl Pts',(56.3242402348248,19.5082110223118,10.1152837761466));
#24512=CARTESIAN_POINT('Ctrl Pts',(56.3304116666648,19.5137134695487,10.1158146973886));
#24513=CARTESIAN_POINT('Ctrl Pts',(56.3333227447129,19.5163243910901,10.1160651374702));
#24514=CARTESIAN_POINT('Ctrl Pts',(56.3409336061122,19.5231909992929,10.1167199678861));
#24515=CARTESIAN_POINT('Ctrl Pts',(56.3456208566869,19.5274606038387,10.1171233222225));
#24516=CARTESIAN_POINT('Ctrl Pts',(56.3618379487831,19.5423748070291,10.1185194321854));
#24517=CARTESIAN_POINT('Ctrl Pts',(56.3732628300936,19.5531333726073,10.1195040001479));
#24518=CARTESIAN_POINT('Ctrl Pts',(56.4724009843591,19.6487219579918,10.1280692486186));
#24519=CARTESIAN_POINT('Ctrl Pts',(56.5522979821094,19.7413116948731,10.1351336542516));
#24520=CARTESIAN_POINT('Ctrl Pts',(56.6257699388341,19.8441805304635,10.1424677671659));
#24521=CARTESIAN_POINT('Ctrl Pts',(56.628290257078,19.84773380728,10.1427204952594));
#24522=CARTESIAN_POINT('Ctrl Pts',(56.7164763606485,19.9729303034087,10.1516047806492));
#24523=CARTESIAN_POINT('Ctrl Pts',(56.7882650465273,20.103750213979,10.1602610192741));
#24524=CARTESIAN_POINT('Ctrl Pts',(56.8514337335229,20.2573553406565,10.170568456624));
#24525=CARTESIAN_POINT('Ctrl Pts',(56.8578163317679,20.2734696101186,10.1716507864361));
#24526=CARTESIAN_POINT('Ctrl Pts',(56.8672244962511,20.2981575335159,10.1733114085919));
#24527=CARTESIAN_POINT('Ctrl Pts',(56.8704028819254,20.3066723559293,10.1738845894396));
#24528=CARTESIAN_POINT('Ctrl Pts',(56.8758348960301,20.3215338178489,10.1748858809387));
#24529=CARTESIAN_POINT('Ctrl Pts',(56.8781147958007,20.3278707494368,10.1753131093524));
#24530=CARTESIAN_POINT('Ctrl Pts',(56.8831680989866,20.3421427737342,10.1762759943016));
#24531=CARTESIAN_POINT('Ctrl Pts',(56.8859235095907,20.3500840580524,10.1768122377103));
#24532=CARTESIAN_POINT('Ctrl Pts',(56.8931821649248,20.3714389023648,10.1782556309659));
#24533=CARTESIAN_POINT('Ctrl Pts',(56.8975929531165,20.3848831572668,10.1791658030527));
#24534=CARTESIAN_POINT('Ctrl Pts',(56.9169568341294,20.4460961521693,10.1833173060348));
#24535=CARTESIAN_POINT('Ctrl Pts',(56.9302505830606,20.4943668082178,10.1866120476153));
#24536=CARTESIAN_POINT('Ctrl Pts',(56.9475476726069,20.5678724988019,10.1916639267382));
#24537=CARTESIAN_POINT('Ctrl Pts',(56.9529056014151,20.5927706539171,10.1933808858098));
#24538=CARTESIAN_POINT('Ctrl Pts',(56.989144349417,20.7783827888683,10.2062191387137));
#24539=CARTESIAN_POINT('Ctrl Pts',(57.0006156252319,20.9422282127028,10.2178364601352));
#24540=CARTESIAN_POINT('Ctrl Pts',(56.9892082568408,21.1573607329815,10.2325809890999));
#24541=CARTESIAN_POINT('Ctrl Pts',(56.9844499091691,21.2089772267665,10.236073312663));
#24542=CARTESIAN_POINT('Ctrl Pts',(56.9764895322872,21.2694452965424,10.2400682320909));
#24543=CARTESIAN_POINT('Ctrl Pts',(56.9752300571101,21.2785280386805,10.2406657120262));
#24544=CARTESIAN_POINT('Ctrl Pts',(56.9731927657954,21.2925106459984,10.2415811928331));
#24545=CARTESIAN_POINT('Ctrl Pts',(56.9724592472064,21.2974166915605,10.2419015839529));
#24546=CARTESIAN_POINT('Ctrl Pts',(56.9710737601621,21.3064527294174,10.2424901071771));
#24547=CARTESIAN_POINT('Ctrl Pts',(56.9704271118367,21.3105833879984,10.2427585241096));
#24548=CARTESIAN_POINT('Ctrl Pts',(56.9689377565809,21.3199051886331,10.2433628991531));
#24549=CARTESIAN_POINT('Ctrl Pts',(56.9680875070261,21.325095040289,10.2436984279468));
#24550=CARTESIAN_POINT('Ctrl Pts',(56.965516168633,21.34041039792,10.2446859258761));
#24551=CARTESIAN_POINT('Ctrl Pts',(56.9637373611646,21.3505262260751,10.2453347399971));
#24552=CARTESIAN_POINT('Ctrl Pts',(56.9488027052193,21.4317733840827,10.2505214668697));
#24553=CARTESIAN_POINT('Ctrl Pts',(56.9318630101755,21.5021633286191,10.2548654909627));
#24554=CARTESIAN_POINT('Ctrl Pts',(56.8786112774649,21.680245449581,10.2658233392881));
#24555=CARTESIAN_POINT('Ctrl Pts',(56.8368634439123,21.7860332648842,10.2723111754453));
#24556=CARTESIAN_POINT('Ctrl Pts',(56.7569574689906,21.9468305989645,10.2828355271104));
#24557=CARTESIAN_POINT('Ctrl Pts',(56.7246563837557,22.0044635619656,10.2867526187784));
#24558=CARTESIAN_POINT('Ctrl Pts',(56.668289269915,22.0942757430114,10.2931910403408));
#24559=CARTESIAN_POINT('Ctrl Pts',(56.646005966302,22.1275160797707,10.295652300041));
#24560=CARTESIAN_POINT('Ctrl Pts',(56.6154237536345,22.1702956459808,10.2989366625541));
#24561=CARTESIAN_POINT('Ctrl Pts',(56.6080116293105,22.1804593984034,10.2997259214886));
#24562=CARTESIAN_POINT('Ctrl Pts',(56.5956929516429,22.1970198593235,10.3010270369599));
#24563=CARTESIAN_POINT('Ctrl Pts',(56.5908427997072,22.2034582348631,10.3015366958463));
#24564=CARTESIAN_POINT('Ctrl Pts',(56.5813561869833,22.2158937588734,10.3025286088321));
#24565=CARTESIAN_POINT('Ctrl Pts',(56.5767242963471,22.2218942317902,10.3030106776787));
#24566=CARTESIAN_POINT('Ctrl Pts',(56.5659073101299,22.2357433853213,10.3041313998706));
#24567=CARTESIAN_POINT('Ctrl Pts',(56.5596972558805,22.2435722263983,10.3047710386005));
#24568=CARTESIAN_POINT('Ctrl Pts',(56.5392652172734,22.2689365252606,10.3068636067134));
#24569=CARTESIAN_POINT('Ctrl Pts',(56.5248047170542,22.2862767274663,10.308326086989));
#24570=CARTESIAN_POINT('Ctrl Pts',(56.3985891068265,22.4325074486482,10.3209407610409));
#24571=CARTESIAN_POINT('Ctrl Pts',(56.2710389719548,22.5467920526852,10.3327966342144));
#24572=CARTESIAN_POINT('Ctrl Pts',(56.0700775949723,22.6850366821492,10.3497978511851));
#24573=CARTESIAN_POINT('Ctrl Pts',(56.007353180692,22.7232688886676,10.3548926440658));
#24574=CARTESIAN_POINT('Ctrl Pts',(55.9221315553986,22.7689668090524,10.3614291946561));
#24575=CARTESIAN_POINT('Ctrl Pts',(55.9014104289643,22.7796149907972,10.3629897304113));
#24576=CARTESIAN_POINT('Ctrl Pts',(55.8663168042062,22.7968786364347,10.3655791628008));
#24577=CARTESIAN_POINT('Ctrl Pts',(55.852043945182,22.8036903261181,10.3666177409116));
#24578=CARTESIAN_POINT('Ctrl Pts',(55.8320845941086,22.8129260750081,10.3680484395896));
#24579=CARTESIAN_POINT('Ctrl Pts',(55.8264660156571,22.8154943273445,10.3684488188394));
#24580=CARTESIAN_POINT('Ctrl Pts',(55.8169071174857,22.8198101280026,10.3691258669876));
#24581=CARTESIAN_POINT('Ctrl Pts',(55.8129729263791,22.8215710699437,10.3694033434984));
#24582=CARTESIAN_POINT('Ctrl Pts',(55.8054159079038,22.8249242277133,10.3699340377519));
#24583=CARTESIAN_POINT('Ctrl Pts',(55.8017940255722,22.8265184266309,10.3701873808363));
#24584=CARTESIAN_POINT('Ctrl Pts',(55.7921286757762,22.8307384141293,10.3708608393988));
#24585=CARTESIAN_POINT('Ctrl Pts',(55.7860768378138,22.8333450815236,10.3712798028832));
#24586=CARTESIAN_POINT('Ctrl Pts',(55.7641699528139,22.8426524690202,10.3727870034766));
#24587=CARTESIAN_POINT('Ctrl Pts',(55.7482407275905,22.8491781144444,10.3738652321395));
#24588=CARTESIAN_POINT('Ctrl Pts',(55.5978827768747,22.9085133556632,10.3838953973148));
#24589=CARTESIAN_POINT('Ctrl Pts',(55.4581569276992,22.9467899973822,10.3921391989112));
#24590=CARTESIAN_POINT('Ctrl Pts',(55.2653737834051,22.9776708571072,10.4034861834246));
#24591=CARTESIAN_POINT('Ctrl Pts',(55.2149845040072,22.9837793810589,10.4064469079153));
#24592=CARTESIAN_POINT('Ctrl Pts',(55.1644480736098,22.9879598571365,10.4094440176549));
#24593=CARTESIAN_POINT('Origin',(55.,21.,6.22095488139522));
#24594=CARTESIAN_POINT('',(55.1644483680005,22.9879598327838,11.3667309363937));
#24595=CARTESIAN_POINT('',(55.1644483504356,22.9879598342369,11.2090168340879));
#24596=CARTESIAN_POINT('',(55.1644483516311,22.987959834138,6.22095488139522));
#24597=CARTESIAN_POINT('',(53.0052507453988,21.0017244615935,10.7798738016618));
#24598=CARTESIAN_POINT('Ctrl Pts',(55.1644483680005,22.9879598327838,11.3667309363937));
#24599=CARTESIAN_POINT('Ctrl Pts',(55.2668183824715,22.9794915621808,11.3603918485463));
#24600=CARTESIAN_POINT('Ctrl Pts',(55.3684168750213,22.9631256322943,11.3544005539574));
#24601=CARTESIAN_POINT('Ctrl Pts',(55.6191159170458,22.9025732145644,11.3394236116951));
#24602=CARTESIAN_POINT('Ctrl Pts',(55.7651174048343,22.8486964255162,11.3304829507699));
#24603=CARTESIAN_POINT('Ctrl Pts',(55.924298641941,22.767837415238,11.3194830744304));
#24604=CARTESIAN_POINT('Ctrl Pts',(55.9450095793867,22.7568534171218,11.3180269037287));
#24605=CARTESIAN_POINT('Ctrl Pts',(55.9738224391431,22.7409156810808,11.3159634403282));
#24606=CARTESIAN_POINT('Ctrl Pts',(55.98209041941,22.7362649437039,11.3153668921521));
#24607=CARTESIAN_POINT('Ctrl Pts',(55.9964121464573,22.7280739491388,11.3143256730236));
#24608=CARTESIAN_POINT('Ctrl Pts',(56.0024810278712,22.7245603863059,11.3138819658548));
#24609=CARTESIAN_POINT('Ctrl Pts',(56.0151210062071,22.7171532382289,11.3129525566407));
#24610=CARTESIAN_POINT('Ctrl Pts',(56.0216885079963,22.7132537730195,11.3124666467453));
#24611=CARTESIAN_POINT('Ctrl Pts',(56.0372290606589,22.7039054090287,11.3113096003018));
#24612=CARTESIAN_POINT('Ctrl Pts',(56.0461817395778,22.698423247601,11.3106372566652));
#24613=CARTESIAN_POINT('Ctrl Pts',(56.0761793682199,22.6797270680567,11.3083645971277));
#24614=CARTESIAN_POINT('Ctrl Pts',(56.097019867477,22.6661909775211,11.3067524688492));
#24615=CARTESIAN_POINT('Ctrl Pts',(56.1462210109412,22.632911140739,11.3028644633317));
#24616=CARTESIAN_POINT('Ctrl Pts',(56.1743313645086,22.6128133826787,11.3005758487876));
#24617=CARTESIAN_POINT('Ctrl Pts',(56.281644685509,22.5317954150987,11.2915715975044));
#24618=CARTESIAN_POINT('Ctrl Pts',(56.3567406605626,22.4656947013413,11.2846754087921));
#24619=CARTESIAN_POINT('Ctrl Pts',(56.441722152327,22.3787440751148,11.2762046689164));
#24620=CARTESIAN_POINT('Ctrl Pts',(56.4566281366828,22.3629865939187,11.2746915864095));
#24621=CARTESIAN_POINT('Ctrl Pts',(56.4764066300199,22.3413831651284,11.2726486410622));
#24622=CARTESIAN_POINT('Ctrl Pts',(56.4815070414649,22.3357478127075,11.2721185519505));
#24623=CARTESIAN_POINT('Ctrl Pts',(56.5265587813653,22.2853954861329,11.267407818775));
#24624=CARTESIAN_POINT('Ctrl Pts',(56.5645088241818,22.2389253510599,11.2632379049449));
#24625=CARTESIAN_POINT('Ctrl Pts',(56.6298007217073,22.1511810155058,11.2557602316587));
#24626=CARTESIAN_POINT('Ctrl Pts',(56.657812784585,22.1104619749982,11.252432760538));
#24627=CARTESIAN_POINT('Ctrl Pts',(56.6888933541455,22.0614804497966,11.2486302821579));
#24628=CARTESIAN_POINT('Ctrl Pts',(56.6934536542744,22.0541898473052,11.2480693564371));
#24629=CARTESIAN_POINT('Ctrl Pts',(56.7007755854378,22.0423140673116,11.24716410446));
#24630=CARTESIAN_POINT('Ctrl Pts',(56.7035661016564,22.0377469565569,11.2468179776615));
#24631=CARTESIAN_POINT('Ctrl Pts',(56.7085076370482,22.0295857225005,11.2462031137966));
#24632=CARTESIAN_POINT('Ctrl Pts',(56.7106657467263,22.0259960087207,11.24593392164));
#24633=CARTESIAN_POINT('Ctrl Pts',(56.7153201603359,22.0181985294533,11.2453519171114));
#24634=CARTESIAN_POINT('Ctrl Pts',(56.7178122926903,22.0139883757513,11.2450393742355));
#24635=CARTESIAN_POINT('Ctrl Pts',(56.7247682594399,22.0021378711376,11.244164295987));
#24636=CARTESIAN_POINT('Ctrl Pts',(56.7291968481554,21.9944768115866,11.243603983246));
#24637=CARTESIAN_POINT('Ctrl Pts',(56.7558984918794,21.9475676854414,11.2402043981201));
#24638=CARTESIAN_POINT('Ctrl Pts',(56.7768872557064,21.9075992616797,11.2374404428493));
#24639=CARTESIAN_POINT('Ctrl Pts',(56.844431519403,21.767633247628,11.2280916919654));
#24640=CARTESIAN_POINT('Ctrl Pts',(56.8840445319404,21.664506016896,11.221758379718));
#24641=CARTESIAN_POINT('Ctrl Pts',(56.9515483192831,21.4331078739736,11.2077534366685));
#24642=CARTESIAN_POINT('Ctrl Pts',(56.9757305176247,21.3043116452713,11.2000726095537));
#24643=CARTESIAN_POINT('Ctrl Pts',(56.9884874826193,21.1586940409902,11.1909990067534));
#24644=CARTESIAN_POINT('Ctrl Pts',(56.9896569452038,21.143288124396,11.1900346392103));
#24645=CARTESIAN_POINT('Ctrl Pts',(56.991263920786,21.1182712409262,11.1884608183101));
#24646=CARTESIAN_POINT('Ctrl Pts',(56.9918110848332,21.1086677770637,11.187854792455));
#24647=CARTESIAN_POINT('Ctrl Pts',(56.9926613957655,21.0915665240527,11.1867721380226));
#24648=CARTESIAN_POINT('Ctrl Pts',(56.9929917363589,21.084070225366,11.1862963692656));
#24649=CARTESIAN_POINT('Ctrl Pts',(56.9935988669506,21.0682658059252,11.1852907234725));
#24650=CARTESIAN_POINT('Ctrl Pts',(56.9938660335417,21.0599574799825,11.1847605546401));
#24651=CARTESIAN_POINT('Ctrl Pts',(56.9944364732796,21.0379332592708,11.1833510470357));
#24652=CARTESIAN_POINT('Ctrl Pts',(56.9946501856733,21.0242156829173,11.1824689294788));
#24653=CARTESIAN_POINT('Ctrl Pts',(56.9949937782996,20.958925206455,11.1782495463655));
#24654=CARTESIAN_POINT('Ctrl Pts',(56.9932650387472,20.907366358009,11.1748549551963));
#24655=CARTESIAN_POINT('Ctrl Pts',(56.9769148115492,20.6815676758152,11.1597028598214));
#24656=CARTESIAN_POINT('Ctrl Pts',(56.9414194939986,20.5096282067382,11.1473262299537));
#24657=CARTESIAN_POINT('Ctrl Pts',(56.878786097787,20.3295961860727,11.1341886500161));
#24658=CARTESIAN_POINT('Ctrl Pts',(56.8734031328936,20.3146977337771,11.1331008172196));
#24659=CARTESIAN_POINT('Ctrl Pts',(56.8506395016987,20.2539681956921,11.1286677791383));
#24660=CARTESIAN_POINT('Ctrl Pts',(56.831748361077,20.2087169627035,11.1253671613535));
#24661=CARTESIAN_POINT('Ctrl Pts',(56.8076122310888,20.1564128912273,11.1215914335513));
#24662=CARTESIAN_POINT('Ctrl Pts',(56.8039666946028,20.1486449864166,11.1210317356633));
#24663=CARTESIAN_POINT('Ctrl Pts',(56.7979684552558,20.1360754772306,11.1201280687724));
#24664=CARTESIAN_POINT('Ctrl Pts',(56.7956464181313,20.13125948074,11.1197823092696));
#24665=CARTESIAN_POINT('Ctrl Pts',(56.7914709777949,20.1226877193273,11.119167842648));
#24666=CARTESIAN_POINT('Ctrl Pts',(56.789625086559,20.1189284065651,11.1188986828282));
#24667=CARTESIAN_POINT('Ctrl Pts',(56.7855953811288,20.1107864867254,11.1183164561528));
#24668=CARTESIAN_POINT('Ctrl Pts',(56.7834072693113,20.1064061043683,11.1180036606244));
#24669=CARTESIAN_POINT('Ctrl Pts',(56.7772112752573,20.0941157498714,11.1171271551517));
#24670=CARTESIAN_POINT('Ctrl Pts',(56.7731666872081,20.0862242628169,11.1165656794886));
#24671=CARTESIAN_POINT('Ctrl Pts',(56.7480564551115,20.038025683833,11.1131428660878));
#24672=CARTESIAN_POINT('Ctrl Pts',(56.72566825211,19.9984183702538,11.1103580455712));
#24673=CARTESIAN_POINT('Ctrl Pts',(56.6397739885888,19.8579067435847,11.1004545116726));
#24674=CARTESIAN_POINT('Ctrl Pts',(56.5686093605042,19.7619754974629,11.0936347196209));
#24675=CARTESIAN_POINT('Ctrl Pts',(56.4812645169098,19.6639502743727,11.0859932787979));
#24676=CARTESIAN_POINT('Ctrl Pts',(56.4731478469768,19.6550060013989,11.0852894235209));
#24677=CARTESIAN_POINT('Ctrl Pts',(56.3907885692442,19.5658890235545,11.0782048107881));
#24678=CARTESIAN_POINT('Ctrl Pts',(56.3101686723837,19.49188180673,11.0717182834002));
#24679=CARTESIAN_POINT('Ctrl Pts',(56.2116735057882,19.4153502894543,11.0639760452976));
#24680=CARTESIAN_POINT('Ctrl Pts',(56.1993347959456,19.4059914003176,11.0630094481628));
#24681=CARTESIAN_POINT('Ctrl Pts',(56.1791488569266,19.3910474614843,11.0614327028074));
#24682=CARTESIAN_POINT('Ctrl Pts',(56.1713678022771,19.3853738003672,11.0608260033716));
#24683=CARTESIAN_POINT('Ctrl Pts',(56.1574501912089,19.3753791393151,11.0597425950025));
#24684=CARTESIAN_POINT('Ctrl Pts',(56.1513297161945,19.371035983149,11.0592667503456));
#24685=CARTESIAN_POINT('Ctrl Pts',(56.1383834803816,19.3619586035276,11.0582614090146));
#24686=CARTESIAN_POINT('Ctrl Pts',(56.1315523792665,19.3572322822449,11.0577316232943));
#24687=CARTESIAN_POINT('Ctrl Pts',(56.1133834827024,19.3448286288575,11.0563242225301));
#24688=CARTESIAN_POINT('Ctrl Pts',(56.1019959754553,19.3372252401561,11.0554438434826));
#24689=CARTESIAN_POINT('Ctrl Pts',(56.0476065227738,19.3017137651208,11.0512462931027));
#24690=CARTESIAN_POINT('Ctrl Pts',(56.0036208964796,19.2753551482622,11.0478725155148));
#24691=CARTESIAN_POINT('Ctrl Pts',(55.8074107151989,19.1678243935281,11.0329008379241));
#24692=CARTESIAN_POINT('Ctrl Pts',(55.6460465504788,19.1049045773506,11.0207018788349));
#24693=CARTESIAN_POINT('Ctrl Pts',(55.4574400959387,19.058286000775,11.0072958427948));
#24694=CARTESIAN_POINT('Ctrl Pts',(55.4361496230854,19.0533931435388,11.0057956343937));
#24695=CARTESIAN_POINT('Ctrl Pts',(55.369807161911,19.0392898166312,11.0011690891197));
#24696=CARTESIAN_POINT('Ctrl Pts',(55.3245105118912,19.031285842289,10.9980785624643));
#24697=CARTESIAN_POINT('Ctrl Pts',(55.2706268478495,19.0236751947435,10.994512796268));
#24698=CARTESIAN_POINT('Ctrl Pts',(55.2622721737798,19.0225491309478,10.993963056626));
#24699=CARTESIAN_POINT('Ctrl Pts',(55.2486525781655,19.0208012837882,10.9930722560897));
#24700=CARTESIAN_POINT('Ctrl Pts',(55.2433919761061,19.0201474776072,10.9927294852665));
#24701=CARTESIAN_POINT('Ctrl Pts',(55.2339739705637,19.0190150794591,10.9921182319632));
#24702=CARTESIAN_POINT('Ctrl Pts',(55.2298176223591,19.0185285932384,10.9918493162519));
#24703=CARTESIAN_POINT('Ctrl Pts',(55.220761025863,19.0174974301263,10.9912651957709));
#24704=CARTESIAN_POINT('Ctrl Pts',(55.2158602871363,19.0169578401349,10.9909502776134));
#24705=CARTESIAN_POINT('Ctrl Pts',(55.2019838591642,19.0154820432115,10.9900617510789));
#24706=CARTESIAN_POINT('Ctrl Pts',(55.1930036091368,19.0145885528791,10.9894904762116));
#24707=CARTESIAN_POINT('Ctrl Pts',(55.1356207302212,19.0092722631872,10.9858622039911));
#24708=CARTESIAN_POINT('Ctrl Pts',(55.0870718107209,19.0065584359232,10.9828927767209));
#24709=CARTESIAN_POINT('Ctrl Pts',(54.9360303379903,19.0036451147226,10.973832597907));
#24710=CARTESIAN_POINT('Ctrl Pts',(54.8335858656606,19.0095643446713,10.9679356839063));
#24711=CARTESIAN_POINT('Ctrl Pts',(54.5984807913196,19.0414349979441,10.9541583559392));
#24712=CARTESIAN_POINT('Ctrl Pts',(54.4671159485836,19.0730277110291,10.9462568724126));
#24713=CARTESIAN_POINT('Ctrl Pts',(54.3253670049151,19.1227316039943,10.9369328001878));
#24714=CARTESIAN_POINT('Ctrl Pts',(54.3108462343836,19.1280135216724,10.9359683500865));
#24715=CARTESIAN_POINT('Ctrl Pts',(54.2873874432543,19.136856570102,10.9343944208915));
#24716=CARTESIAN_POINT('Ctrl Pts',(54.2784110753953,19.1403146731038,10.9337883700867));
#24717=CARTESIAN_POINT('Ctrl Pts',(54.2624778729155,19.1465855888969,10.9327056877423));
#24718=CARTESIAN_POINT('Ctrl Pts',(54.2555111909248,19.149373004122,10.9322299161883));
#24719=CARTESIAN_POINT('Ctrl Pts',(54.2484051403963,19.1522628007106,10.9317421544061));
#24720=CARTESIAN_POINT('Ctrl Pts',(54.2482498099747,19.1523259913029,10.9317314912612));
#24721=CARTESIAN_POINT('Ctrl Pts',(54.2479536870199,19.1524465017919,10.9317111606623));
#24722=CARTESIAN_POINT('Ctrl Pts',(54.2478128891772,19.1525038197812,10.9317014930595));
#24723=CARTESIAN_POINT('Ctrl Pts',(54.2475444218924,19.1526131470431,10.9316830573906));
#24724=CARTESIAN_POINT('Ctrl Pts',(54.2474167555492,19.1526651517185,10.9316742897144));
#24725=CARTESIAN_POINT('Ctrl Pts',(54.2471732977741,19.1527643532698,10.9316575683275));
#24726=CARTESIAN_POINT('Ctrl Pts',(54.2470575054225,19.1528115477855,10.9316496146988));
#24727=CARTESIAN_POINT('Ctrl Pts',(54.2468366611527,19.1529015834592,10.9316344439024));
#24728=CARTESIAN_POINT('Ctrl Pts',(54.2467316084176,19.1529444227057,10.9316272267979));
#24729=CARTESIAN_POINT('Ctrl Pts',(54.2465312209705,19.1530261582444,10.9316134591566));
#24730=CARTESIAN_POINT('Ctrl Pts',(54.2464358855569,19.1530650529796,10.9316069086695));
#24731=CARTESIAN_POINT('Ctrl Pts',(54.2462540108407,19.1531392702581,10.9315944112028));
#24732=CARTESIAN_POINT('Ctrl Pts',(54.2461674710736,19.1531745914762,10.9315884642718));
#24733=CARTESIAN_POINT('Ctrl Pts',(54.2460023565476,19.1532419965324,10.9315771170385));
#24734=CARTESIAN_POINT('Ctrl Pts',(54.2459237813517,19.1532740793035,10.9315717167723));
#24735=CARTESIAN_POINT('Ctrl Pts',(54.2457738460258,19.1533353100513,10.9315614115192));
#24736=CARTESIAN_POINT('Ctrl Pts',(54.2457024855702,19.1533644571365,10.9315565065644));
#24737=CARTESIAN_POINT('Ctrl Pts',(54.2455663028737,19.1534200899924,10.931547145569));
#24738=CARTESIAN_POINT('Ctrl Pts',(54.2455014803539,19.1534465750336,10.9315426895541));
#24739=CARTESIAN_POINT('Ctrl Pts',(54.2453777623816,19.1534971310502,10.9315341845574));
#24740=CARTESIAN_POINT('Ctrl Pts',(54.2453188666397,19.1535212014491,10.9315301355926));
#24741=CARTESIAN_POINT('Ctrl Pts',(54.245177769322,19.1535788751045,10.9315204350148));
#24742=CARTESIAN_POINT('Ctrl Pts',(54.2450955687962,19.1536124810498,10.9315147833082));
#24743=CARTESIAN_POINT('Ctrl Pts',(54.2449329009808,19.1536789970222,10.9315035983899));
#24744=CARTESIAN_POINT('Ctrl Pts',(54.2448524335574,19.1537119068374,10.9314980651832));
#24745=CARTESIAN_POINT('Ctrl Pts',(54.2446931859958,19.1537770485491,10.9314871141471));
#24746=CARTESIAN_POINT('Ctrl Pts',(54.2446144057922,19.1538092802182,10.9314816963266));
#24747=CARTESIAN_POINT('Ctrl Pts',(54.2444584883135,19.1538730830289,10.9314709730527));
#24748=CARTESIAN_POINT('Ctrl Pts',(54.2443813509234,19.1539046539752,10.9314656676041));
#24749=CARTESIAN_POINT('Ctrl Pts',(54.2442286757409,19.1539671523534,10.931455166132));
#24750=CARTESIAN_POINT('Ctrl Pts',(54.2441531379659,19.1539980795471,10.9314499701218));
#24751=CARTESIAN_POINT('Ctrl Pts',(54.2440036202437,19.1540593068339,10.9314396846898));
#24752=CARTESIAN_POINT('Ctrl Pts',(54.2439296402393,19.1540896067299,10.9314345952756));
#24753=CARTESIAN_POINT('Ctrl Pts',(54.2437831977011,19.1541495952941,10.931424520294));
#24754=CARTESIAN_POINT('Ctrl Pts',(54.2437107349883,19.1541792838251,10.9314195347254));
#24755=CARTESIAN_POINT('Ctrl Pts',(54.2355026579802,19.1575427606296,10.9308547738208));
#24756=CARTESIAN_POINT('Ctrl Pts',(54.2273892818791,19.1609302517248,10.9302931858881));
#24757=CARTESIAN_POINT('Ctrl Pts',(54.2044748184771,19.1706758780015,10.9286974669543));
#24758=CARTESIAN_POINT('Ctrl Pts',(54.1897282545356,19.1771597077648,10.9276590854953));
#24759=CARTESIAN_POINT('Ctrl Pts',(54.1566999366788,19.192161705036,10.9253069124052));
#24760=CARTESIAN_POINT('Ctrl Pts',(54.1384658094063,19.2007798670462,10.9239897958124));
#24761=CARTESIAN_POINT('Ctrl Pts',(53.9665274189338,19.2852576357964,10.911390175425));
#24762=CARTESIAN_POINT('Ctrl Pts',(53.8230966453887,19.3803446406582,10.8994091001011));
#24763=CARTESIAN_POINT('Ctrl Pts',(53.6230839921941,19.5536803982552,10.8809917275003));
#24764=CARTESIAN_POINT('Ctrl Pts',(53.556921678593,19.6196858246545,10.8745568848178));
#24765=CARTESIAN_POINT('Ctrl Pts',(53.4887599033793,19.697966961325,10.8677402494761));
#24766=CARTESIAN_POINT('Ctrl Pts',(53.4819625987441,19.7058983335307,10.8670582596291));
#24767=CARTESIAN_POINT('Ctrl Pts',(53.471812472039,19.7179319439403,10.8660369854317));
#24768=CARTESIAN_POINT('Ctrl Pts',(53.468413302882,19.7219945963467,10.8656944744065));
#24769=CARTESIAN_POINT('Ctrl Pts',(53.4623579488112,19.7292907513778,10.8650834987691));
#24770=CARTESIAN_POINT('Ctrl Pts',(53.4596957262742,19.732519105665,10.8648146026209));
#24771=CARTESIAN_POINT('Ctrl Pts',(53.4539169413917,19.7395718680027,10.8642303100145));
#24772=CARTESIAN_POINT('Ctrl Pts',(53.4508044060781,19.7433994616067,10.863915201531));
#24773=CARTESIAN_POINT('Ctrl Pts',(53.4420296808376,19.7542722047618,10.8630255943933));
#24774=CARTESIAN_POINT('Ctrl Pts',(53.4364010420819,19.7613444541075,10.8624534382661));
#24775=CARTESIAN_POINT('Ctrl Pts',(53.4006303502014,19.8069218623397,10.8588057787777));
#24776=CARTESIAN_POINT('Ctrl Pts',(53.3718620015992,19.8464895939911,10.8558189291558));
#24777=CARTESIAN_POINT('Ctrl Pts',(53.2788507577538,19.9848399916961,10.8458232836809));
#24778=CARTESIAN_POINT('Ctrl Pts',(53.2219117192847,20.0882377405094,10.8390848626177));
#24779=CARTESIAN_POINT('Ctrl Pts',(53.1529876377438,20.244749665733,10.8291263213151));
#24780=CARTESIAN_POINT('Ctrl Pts',(53.1335039572553,20.2942735210264,10.8260097617835));
#24781=CARTESIAN_POINT('Ctrl Pts',(53.1052921918637,20.3753589883507,10.8209036776332));
#24782=CARTESIAN_POINT('Ctrl Pts',(53.0953202619795,20.4064606013586,10.8189445623523));
#24783=CARTESIAN_POINT('Ctrl Pts',(53.0746973840322,20.4766655414888,10.814506264319));
#24784=CARTESIAN_POINT('Ctrl Pts',(53.0644658403725,20.5158757536743,10.8120163845285));
#24785=CARTESIAN_POINT('Ctrl Pts',(53.0525133445694,20.568149124727,10.8086699809758));
#24786=CARTESIAN_POINT('Ctrl Pts',(53.0497171011338,20.5809581728341,10.8078478853144));
#24787=CARTESIAN_POINT('Ctrl Pts',(53.0453818911083,20.6018009269637,10.8065063942485));
#24788=CARTESIAN_POINT('Ctrl Pts',(53.0437656848052,20.609818306175,10.8059894713785));
#24789=CARTESIAN_POINT('Ctrl Pts',(53.0407544461699,20.6252450600583,10.804992992783));
#24790=CARTESIAN_POINT('Ctrl Pts',(53.0393520246413,20.6326528625748,10.8045136818204));
#24791=CARTESIAN_POINT('Ctrl Pts',(53.0366633021752,20.6473092452745,10.8035636930044));
#24792=CARTESIAN_POINT('Ctrl Pts',(53.0353750658187,20.6545573519588,10.8030930851169));
#24793=CARTESIAN_POINT('Ctrl Pts',(53.0324989239059,20.6712762642178,10.8020056345429));
#24794=CARTESIAN_POINT('Ctrl Pts',(53.0309392386597,20.6807516770672,10.801387908206));
#24795=CARTESIAN_POINT('Ctrl Pts',(53.0270893902751,20.705242487661,10.7997874992393));
#24796=CARTESIAN_POINT('Ctrl Pts',(53.0249022367707,20.7202732233222,10.7988016081118));
#24797=CARTESIAN_POINT('Ctrl Pts',(53.0110638895879,20.8236460265885,10.7919949654859));
#24798=CARTESIAN_POINT('Ctrl Pts',(53.0051737349807,20.9126436292466,10.7859966396632));
#24799=CARTESIAN_POINT('Ctrl Pts',(53.0052507453988,21.0017244615935,10.7798738016618));
#24800=CARTESIAN_POINT('Ctrl Pts',(53.0052507436693,21.0017224598663,10.7798739392475));
#24801=CARTESIAN_POINT('Ctrl Pts',(53.0053401082293,21.1052139218134,10.7727606100826));
#24802=CARTESIAN_POINT('Ctrl Pts',(53.0134834815291,21.2085419252929,10.7654959353685));
#24803=CARTESIAN_POINT('Ctrl Pts',(53.0415117213874,21.3862523847116,10.7530068709339));
#24804=CARTESIAN_POINT('Ctrl Pts',(53.0577462375717,21.460998914051,10.7477591986531));
#24805=CARTESIAN_POINT('Ctrl Pts',(53.0822721918839,21.549158293487,10.7417069013195));
#24806=CARTESIAN_POINT('Ctrl Pts',(53.0864768818613,21.5636347101916,10.7407176746211));
#24807=CARTESIAN_POINT('Ctrl Pts',(53.092602145558,21.5838644838402,10.739343108748));
#24808=CARTESIAN_POINT('Ctrl Pts',(53.0943853379086,21.5896584372072,10.7389503270862));
#24809=CARTESIAN_POINT('Ctrl Pts',(53.0974753413965,21.5995380592557,10.7382822242631));
#24810=CARTESIAN_POINT('Ctrl Pts',(53.0987689608607,21.6036277812199,10.7380061457142));
#24811=CARTESIAN_POINT('Ctrl Pts',(53.101290137837,21.6115098606777,10.7374750396282));
#24812=CARTESIAN_POINT('Ctrl Pts',(53.1025158758534,21.6153027301032,10.7372199038554));
#24813=CARTESIAN_POINT('Ctrl Pts',(53.105494283013,21.6244254392014,10.7366072314572));
#24814=CARTESIAN_POINT('Ctrl Pts',(53.1072580977335,21.6297516447312,10.7362503414788));
#24815=CARTESIAN_POINT('Ctrl Pts',(53.1138234486359,21.6493003229001,10.7349432016805));
#24816=CARTESIAN_POINT('Ctrl Pts',(53.1187631524077,21.6634763350936,10.7340006673194));
#24817=CARTESIAN_POINT('Ctrl Pts',(53.1705796033817,21.8069465170489,10.724503332196));
#24818=CARTESIAN_POINT('Ctrl Pts',(53.2305556955158,21.9311389198942,10.7166110483166));
#24819=CARTESIAN_POINT('Ctrl Pts',(53.3502739136803,22.1249793055242,10.7033867006442));
#24820=CARTESIAN_POINT('Ctrl Pts',(53.4028586232198,22.1984624953458,10.6981264450733));
#24821=CARTESIAN_POINT('Ctrl Pts',(53.4946415376753,22.3099055752745,10.6894539529229));
#24822=CARTESIAN_POINT('Ctrl Pts',(53.5307317734994,22.3502617528428,10.686150040811));
#24823=CARTESIAN_POINT('Ctrl Pts',(53.5778654044065,22.3988369784169,10.6819314277818));
#24824=CARTESIAN_POINT('Ctrl Pts',(53.5874139943019,22.4084787759432,10.6810814875969));
#24825=CARTESIAN_POINT('Ctrl Pts',(53.6021234090578,22.4230317396734,10.6797788315187));
#24826=CARTESIAN_POINT('Ctrl Pts',(53.6072135283177,22.4280140537797,10.6793292459085));
#24827=CARTESIAN_POINT('Ctrl Pts',(53.6176347302153,22.4381058198931,10.6784111360838));
#24828=CARTESIAN_POINT('Ctrl Pts',(53.6229677138441,22.4432131404622,10.6779425300285));
#24829=CARTESIAN_POINT('Ctrl Pts',(53.6346476617258,22.4542751789837,10.6769188116558));
#24830=CARTESIAN_POINT('Ctrl Pts',(53.6410054621656,22.4602181843866,10.6763632098797));
#24831=CARTESIAN_POINT('Ctrl Pts',(53.6584935857218,22.4763522077062,10.6748392707228));
#24832=CARTESIAN_POINT('Ctrl Pts',(53.6697008082327,22.4864586574664,10.6738673878544));
#24833=CARTESIAN_POINT('Ctrl Pts',(53.7287419271851,22.5384982602923,10.6687707313523));
#24834=CARTESIAN_POINT('Ctrl Pts',(53.7784421657646,22.5782486980455,10.6645574323274));
#24835=CARTESIAN_POINT('Ctrl Pts',(53.9697094048945,22.7167720033435,10.6486115837678));
#24836=CARTESIAN_POINT('Ctrl Pts',(54.1219852859054,22.7994116425068,10.6363529486174));
#24837=CARTESIAN_POINT('Ctrl Pts',(54.3321809163916,22.8803790437716,10.6209278774489));
#24838=CARTESIAN_POINT('Ctrl Pts',(54.382120722739,22.8973755447677,10.6173718475456));
#24839=CARTESIAN_POINT('Ctrl Pts',(54.4415103701549,22.9149939255439,10.6133138458856));
#24840=CARTESIAN_POINT('Ctrl Pts',(54.4503590526472,22.9175524082494,10.6127136263765));
#24841=CARTESIAN_POINT('Ctrl Pts',(54.46400946534,22.921396995067,10.6117947917815));
#24842=CARTESIAN_POINT('Ctrl Pts',(54.4687986708469,22.9227265575506,10.6114737603378));
#24843=CARTESIAN_POINT('Ctrl Pts',(54.477626350717,22.9251417661823,10.6108845475352));
#24844=CARTESIAN_POINT('Ctrl Pts',(54.4816632509689,22.9262326091559,10.6106160774727));
#24845=CARTESIAN_POINT('Ctrl Pts',(54.4907766289446,22.9286644830695,10.6100121842035));
#24846=CARTESIAN_POINT('Ctrl Pts',(54.4958549792744,22.9299981682587,10.6096771863157));
#24847=CARTESIAN_POINT('Ctrl Pts',(54.5108401365037,22.9338704137622,10.6086929816708));
#24848=CARTESIAN_POINT('Ctrl Pts',(54.5207614454318,22.9363529036814,10.6080468977304));
#24849=CARTESIAN_POINT('Ctrl Pts',(54.5991804092406,22.9553350923326,10.6029805855274));
#24850=CARTESIAN_POINT('Ctrl Pts',(54.6684975544394,22.9682733786652,10.5987441951056));
#24851=CARTESIAN_POINT('Ctrl Pts',(54.8796520606731,22.9962105182464,10.5861740484261));
#24852=CARTESIAN_POINT('Ctrl Pts',(55.0224939943398,22.9997026117018,10.5780915871545));
#24853=CARTESIAN_POINT('Ctrl Pts',(55.1644484221208,22.9879598283069,10.5696416509586));
#24854=CARTESIAN_POINT('Ctrl Pts',(55.1644480736098,22.9879598571365,10.4094440176549));
#24855=CARTESIAN_POINT('Ctrl Pts',(55.0863476134817,22.9944204856899,10.4140758376681));
#24856=CARTESIAN_POINT('Ctrl Pts',(55.0078958510275,22.9962763510142,10.4187968915192));
#24857=CARTESIAN_POINT('Ctrl Pts',(54.9125225979619,22.9929033495909,10.424722003396));
#24858=CARTESIAN_POINT('Ctrl Pts',(54.8955568817554,22.9920862591188,10.4257829955949));
#24859=CARTESIAN_POINT('Ctrl Pts',(54.869604315938,22.9905039122646,10.4274175598496));
#24860=CARTESIAN_POINT('Ctrl Pts',(54.8606085078574,22.9898941848176,10.4279862681447));
#24861=CARTESIAN_POINT('Ctrl Pts',(54.8442555387887,22.9886743629352,10.4290240905391));
#24862=CARTESIAN_POINT('Ctrl Pts',(54.8368970046441,22.988084371827,10.4294925663439));
#24863=CARTESIAN_POINT('Ctrl Pts',(54.8208781677725,22.9867104836328,10.430515682826));
#24864=CARTESIAN_POINT('Ctrl Pts',(54.812219407468,22.9859107788805,10.4310708106726));
#24865=CARTESIAN_POINT('Ctrl Pts',(54.7885737291298,22.9835708890003,10.432592641983));
#24866=CARTESIAN_POINT('Ctrl Pts',(54.7735988359574,22.9819175139124,10.4335628761634));
#24867=CARTESIAN_POINT('Ctrl Pts',(54.6958225854969,22.9724372954723,10.4386367051597));
#24868=CARTESIAN_POINT('Ctrl Pts',(54.6334072132447,22.9617953627795,10.4428278850709));
#24869=CARTESIAN_POINT('Ctrl Pts',(54.4027392660803,22.9110737283502,10.4587716167255));
#24870=CARTESIAN_POINT('Ctrl Pts',(54.2394431953386,22.8521510858263,10.4710549008445));
#24871=CARTESIAN_POINT('Ctrl Pts',(54.038910143789,22.7487473094079,10.4865057328242));
#24872=CARTESIAN_POINT('Ctrl Pts',(53.9929928237833,22.7227154422734,10.490063854692));
#24873=CARTESIAN_POINT('Ctrl Pts',(53.9403320782204,22.6900344036017,10.4941237899967));
#24874=CARTESIAN_POINT('Ctrl Pts',(53.9325399620683,22.6851235756166,10.4947239675833));
#24875=CARTESIAN_POINT('Ctrl Pts',(53.9205964309163,22.6774803100883,10.4956426939913));
#24876=CARTESIAN_POINT('Ctrl Pts',(53.9164208693105,22.6747861130678,10.4959636591205));
#24877=CARTESIAN_POINT('Ctrl Pts',(53.9087511630472,22.6697966985182,10.4965527228833));
#24878=CARTESIAN_POINT('Ctrl Pts',(53.9052541812232,22.6675061113563,10.4968211102632));
#24879=CARTESIAN_POINT('Ctrl Pts',(53.8973831557249,22.6623150125175,10.497424777244));
#24880=CARTESIAN_POINT('Ctrl Pts',(53.8930133506873,22.6594082276171,10.4977596320673));
#24881=CARTESIAN_POINT('Ctrl Pts',(53.8801677358121,22.650790029003,10.4987432952975));
#24882=CARTESIAN_POINT('Ctrl Pts',(53.8717241377704,22.6450305799475,10.4993889850816));
#24883=CARTESIAN_POINT('Ctrl Pts',(53.8055331675151,22.5991317683604,10.5044468271993));
#24884=CARTESIAN_POINT('Ctrl Pts',(53.7498941574263,22.5560241305798,10.5086758136785));
#24885=CARTESIAN_POINT('Ctrl Pts',(53.5683572067163,22.3993369449524,10.5228293258379));
#24886=CARTESIAN_POINT('Ctrl Pts',(53.4547065097968,22.2727196755946,10.5323833857303));
#24887=CARTESIAN_POINT('Ctrl Pts',(53.3395478249205,22.1059071106663,10.5445940705102));
#24888=CARTESIAN_POINT('Ctrl Pts',(53.3213550154786,22.0780922029669,10.5466164820234));
#24889=CARTESIAN_POINT('Ctrl Pts',(53.2911753873372,22.0293334992437,10.5501487454425));
#24890=CARTESIAN_POINT('Ctrl Pts',(53.278857876023,22.0086023599044,10.5516466613861));
#24891=CARTESIAN_POINT('Ctrl Pts',(53.261784537033,21.978643003503,10.5538082858875));
#24892=CARTESIAN_POINT('Ctrl Pts',(53.2567199182606,21.9695925299296,10.5544608960713));
#24893=CARTESIAN_POINT('Ctrl Pts',(53.2480599138474,21.9538298959036,10.5555970129156));
#24894=CARTESIAN_POINT('Ctrl Pts',(53.2444319253344,21.9471358236188,10.5560793459627));
#24895=CARTESIAN_POINT('Ctrl Pts',(53.2375241102379,21.934214023006,10.5570101927488));
#24896=CARTESIAN_POINT('Ctrl Pts',(53.2342387413204,21.9279893738779,10.55745850101));
#24897=CARTESIAN_POINT('Ctrl Pts',(53.2265527933008,21.9132385381556,10.558520715992));
#24898=CARTESIAN_POINT('Ctrl Pts',(53.2221806833218,21.9046977917732,10.559135613073));
#24899=CARTESIAN_POINT('Ctrl Pts',(53.2070464692638,21.8746003146458,10.5613022719627));
#24900=CARTESIAN_POINT('Ctrl Pts',(53.1966138178407,21.8528811566704,10.5628654117797));
#24901=CARTESIAN_POINT('Ctrl Pts',(53.1291282369546,21.7056092602686,10.573466397367));
#24902=CARTESIAN_POINT('Ctrl Pts',(53.0848448398029,21.5746420688875,10.5829409461477));
#24903=CARTESIAN_POINT('Ctrl Pts',(53.0331408493616,21.3461132024955,10.599270808405));
#24904=CARTESIAN_POINT('Ctrl Pts',(53.018707549087,21.2506216440511,10.6060259627357));
#24905=CARTESIAN_POINT('Ctrl Pts',(53.0091279141836,21.1272759435081,10.6144291612223));
#24906=CARTESIAN_POINT('Ctrl Pts',(53.0075742506162,21.1000530517522,10.6162632944604));
#24907=CARTESIAN_POINT('Ctrl Pts',(53.005929789255,21.0550275790471,10.6192542956688));
#24908=CARTESIAN_POINT('Ctrl Pts',(53.0055183123431,21.0372409770852,10.6204248762878));
#24909=CARTESIAN_POINT('Ctrl Pts',(53.0052817470962,21.012981164723,10.6220044057902));
#24910=CARTESIAN_POINT('Ctrl Pts',(53.0052501351687,21.0065114263768,10.6224239878818));
#24911=CARTESIAN_POINT('Ctrl Pts',(53.0052499184983,20.9961071431697,10.623095952249));
#24912=CARTESIAN_POINT('Ctrl Pts',(53.0052614767333,20.9921727119171,10.623349418505));
#24913=CARTESIAN_POINT('Ctrl Pts',(53.0053102159789,20.9839068224652,10.6238805467052));
#24914=CARTESIAN_POINT('Ctrl Pts',(53.0053498648552,20.9795754134117,10.6241580626731));
#24915=CARTESIAN_POINT('Ctrl Pts',(53.00548163476,20.9689586256248,10.6248363973381));
#24916=CARTESIAN_POINT('Ctrl Pts',(53.0055893589523,20.9626734191028,10.6252363531352));
#24917=CARTESIAN_POINT('Ctrl Pts',(53.0060881023872,20.9398666868124,10.6266820980133));
#24918=CARTESIAN_POINT('Ctrl Pts',(53.0066547317768,20.9233491393244,10.6277185948844));
#24919=CARTESIAN_POINT('Ctrl Pts',(53.0085800783319,20.8821684737605,10.6302805963666));
#24920=CARTESIAN_POINT('Ctrl Pts',(53.0101917251743,20.8575194171634,10.6317942822705));
#24921=CARTESIAN_POINT('Ctrl Pts',(53.0190449357502,20.7522025049653,10.6382008516644));
#24922=CARTESIAN_POINT('Ctrl Pts',(53.030738186202,20.6719808779836,10.6429296916237));
#24923=CARTESIAN_POINT('Ctrl Pts',(53.0797404901348,20.4370561549053,10.6568724428793));
#24924=CARTESIAN_POINT('Ctrl Pts',(53.1306864232294,20.2858831203412,10.6660183651889));
#24925=CARTESIAN_POINT('Ctrl Pts',(53.2089979286368,20.1214349631584,10.6772432172742));
#24926=CARTESIAN_POINT('Ctrl Pts',(53.2193284645256,20.1006815042349,10.6786834597493));
#24927=CARTESIAN_POINT('Ctrl Pts',(53.2343712847124,20.0717371517246,10.6807278666122));
#24928=CARTESIAN_POINT('Ctrl Pts',(53.238783911721,20.063391991698,10.6813215498073));
#24929=CARTESIAN_POINT('Ctrl Pts',(53.2465713550007,20.0489140176549,10.6823590971529));
#24930=CARTESIAN_POINT('Ctrl Pts',(53.2499195531022,20.0427670156791,10.682802013815));
#24931=CARTESIAN_POINT('Ctrl Pts',(53.2569919885059,20.029943777177,10.6837310788419));
#24932=CARTESIAN_POINT('Ctrl Pts',(53.2607223837042,20.0232710845121,10.6842174417203));
#24933=CARTESIAN_POINT('Ctrl Pts',(53.2696895185394,20.007445519221,10.685377988833));
#24934=CARTESIAN_POINT('Ctrl Pts',(53.2749606201221,19.9983124786803,10.6860534009788));
#24935=CARTESIAN_POINT('Ctrl Pts',(53.2930441441609,19.9675459192176,10.6883481585971));
#24936=CARTESIAN_POINT('Ctrl Pts',(53.3061926523336,19.9461137177736,10.6899796339915));
#24937=CARTESIAN_POINT('Ctrl Pts',(53.3386517077019,19.8953822200822,10.6939229361675));
#24938=CARTESIAN_POINT('Ctrl Pts',(53.3583365981146,19.8663335527262,10.696247987536));
#24939=CARTESIAN_POINT('Ctrl Pts',(53.4385467685856,19.7544415188165,10.705472508389));
#24940=CARTESIAN_POINT('Ctrl Pts',(53.5046538440628,19.6758068028398,10.7125624110261));
#24941=CARTESIAN_POINT('Ctrl Pts',(53.6645774879033,19.5128954462777,10.7284739885947));
#24942=CARTESIAN_POINT('Ctrl Pts',(53.7609407657918,19.4316980676334,10.737294803976));
#24943=CARTESIAN_POINT('Ctrl Pts',(53.8770984665918,19.3512545577252,10.7466502190346));
#24944=CARTESIAN_POINT('Ctrl Pts',(53.889986342729,19.3425504219906,10.7476717215669));
#24945=CARTESIAN_POINT('Ctrl Pts',(53.9082507330908,19.3305237348263,10.7490948943379));
#24946=CARTESIAN_POINT('Ctrl Pts',(53.9135428641555,19.3270749101136,10.749504410973));
#24947=CARTESIAN_POINT('Ctrl Pts',(53.922133946302,19.3215341558295,10.7501644950792));
#24948=CARTESIAN_POINT('Ctrl Pts',(53.9254227638834,19.3194267097131,10.7504160768911));
#24949=CARTESIAN_POINT('Ctrl Pts',(53.9323981383867,19.3149857974539,10.7509472847016));
#24950=CARTESIAN_POINT('Ctrl Pts',(53.9360862023527,19.3126547390706,10.7512267457311));
#24951=CARTESIAN_POINT('Ctrl Pts',(53.9452370776753,19.3069128151169,10.7519167596891));
#24952=CARTESIAN_POINT('Ctrl Pts',(53.9507088712456,19.3035162341499,10.7523263801556));
#24953=CARTESIAN_POINT('Ctrl Pts',(53.9711795197516,19.2909461404471,10.7538481305647));
#24954=CARTESIAN_POINT('Ctrl Pts',(53.9862835180061,19.2819442326525,10.7549496402534));
#24955=CARTESIAN_POINT('Ctrl Pts',(54.0247353603372,19.2597107979409,10.757705668641));
#24956=CARTESIAN_POINT('Ctrl Pts',(54.0482353895762,19.2467481946488,10.7593459406939));
#24957=CARTESIAN_POINT('Ctrl Pts',(54.2278400653979,19.1523543101309,10.7716068696709));
#24958=CARTESIAN_POINT('Ctrl Pts',(54.3938566153392,19.0914331684165,10.7814557470698));
#24959=CARTESIAN_POINT('Ctrl Pts',(54.5886988562286,19.0479721222878,10.7932998580453));
#24960=CARTESIAN_POINT('Ctrl Pts',(54.6117578094609,19.0432554036462,10.7947045893341));
#24961=CARTESIAN_POINT('Ctrl Pts',(54.6859286022279,19.0294463978242,10.7992409975649));
#24962=CARTESIAN_POINT('Ctrl Pts',(54.7373105820563,19.0219413789412,10.8024114347813));
#24963=CARTESIAN_POINT('Ctrl Pts',(54.8031661041818,19.0149334711471,10.8065373944642));
#24964=CARTESIAN_POINT('Ctrl Pts',(54.8174241481265,19.0135713584646,10.8074343410588));
#24965=CARTESIAN_POINT('Ctrl Pts',(54.8401091413842,19.0116504895956,10.8088677273408));
#24966=CARTESIAN_POINT('Ctrl Pts',(54.8485272785639,19.0109914848589,10.8094010191624));
#24967=CARTESIAN_POINT('Ctrl Pts',(54.8636611837316,19.0099033760352,10.8103623356527));
#24968=CARTESIAN_POINT('Ctrl Pts',(54.8703754554391,19.0094547678672,10.8107897418362));
#24969=CARTESIAN_POINT('Ctrl Pts',(54.8861096975345,19.008483443738,10.8117935198066));
#24970=CARTESIAN_POINT('Ctrl Pts',(54.8951311463981,19.0079880236381,10.8123707375738));
#24971=CARTESIAN_POINT('Ctrl Pts',(54.9212099366469,19.0067335315421,10.8140443640473));
#24972=CARTESIAN_POINT('Ctrl Pts',(54.9382737175133,19.0061321697954,10.8151456688436));
#24973=CARTESIAN_POINT('Ctrl Pts',(55.0920123057643,19.0026894959832,10.825126572705));
#24974=CARTESIAN_POINT('Ctrl Pts',(55.2286080024636,19.0136866690473,10.8344493562165));
#24975=CARTESIAN_POINT('Ctrl Pts',(55.5007456387436,19.0640479904935,10.8537019886178));
#24976=CARTESIAN_POINT('Ctrl Pts',(55.6354489756893,19.1039866388751,10.8635831338431));
#24977=CARTESIAN_POINT('Ctrl Pts',(55.7785533594583,19.1633993384021,10.8738321707524));
#24978=CARTESIAN_POINT('Ctrl Pts',(55.7921813340977,19.1692362007036,10.874805246222));
#24979=CARTESIAN_POINT('Ctrl Pts',(55.8108518904856,19.1774803269982,10.876133052349));
#24980=CARTESIAN_POINT('Ctrl Pts',(55.8159509163856,19.1797574747733,10.8764951315042));
#24981=CARTESIAN_POINT('Ctrl Pts',(55.8246659663949,19.1836934640961,10.8771129522546));
#24982=CARTESIAN_POINT('Ctrl Pts',(55.8282866794595,19.1853417495832,10.877369323172));
#24983=CARTESIAN_POINT('Ctrl Pts',(55.8358043837662,19.188791280658,10.8779009532396));
#24984=CARTESIAN_POINT('Ctrl Pts',(55.8397005126308,19.1905942847442,10.8781760929409));
#24985=CARTESIAN_POINT('Ctrl Pts',(55.8491065557515,19.1949840252407,10.8788394746496));
#24986=CARTESIAN_POINT('Ctrl Pts',(55.8546105688266,19.1975834582037,10.8792269415692));
#24987=CARTESIAN_POINT('Ctrl Pts',(55.8738492984546,19.2067774560459,10.8805790792168));
#24988=CARTESIAN_POINT('Ctrl Pts',(55.88752069153,19.2135043398012,10.8815359643569));
#24989=CARTESIAN_POINT('Ctrl Pts',(55.9708022716576,19.2556743111458,10.8873487008874));
#24990=CARTESIAN_POINT('Ctrl Pts',(56.03836577675,19.2950283191704,10.8919953393839));
#24991=CARTESIAN_POINT('Ctrl Pts',(56.1754259180519,19.3860403935082,10.901634897512));
#24992=CARTESIAN_POINT('Ctrl Pts',(56.2442183467279,19.4384581811158,10.9066039699284));
#24993=CARTESIAN_POINT('Ctrl Pts',(56.3937031051243,19.568529355335,10.9181642785256));
#24994=CARTESIAN_POINT('Ctrl Pts',(56.4716848614971,19.648831879445,10.924790366076));
#24995=CARTESIAN_POINT('Ctrl Pts',(56.5523619595254,19.7472268968791,10.9326880476692));
#24996=CARTESIAN_POINT('Ctrl Pts',(56.5620551696402,19.7593341597923,10.9336560555268));
#24997=CARTESIAN_POINT('Ctrl Pts',(56.5775398276772,19.7791443598114,10.9352345587421));
#24998=CARTESIAN_POINT('Ctrl Pts',(56.5834184832331,19.7867785429692,10.9358415911659));
#24999=CARTESIAN_POINT('Ctrl Pts',(56.5937764231715,19.800433169683,10.9369252515318));
#25000=CARTESIAN_POINT('Ctrl Pts',(56.5982775089211,19.806436901786,10.9374010123231));
#25001=CARTESIAN_POINT('Ctrl Pts',(56.6076856961254,19.8191345749633,10.9384058216565));
#25002=CARTESIAN_POINT('Ctrl Pts',(56.6125850965443,19.8258340183158,10.938935156982));
#25003=CARTESIAN_POINT('Ctrl Pts',(56.6254418086082,19.843646547678,10.9403405295749));
#25004=CARTESIAN_POINT('Ctrl Pts',(56.6333268420728,19.8548110237147,10.9412193179625));
#25005=CARTESIAN_POINT('Ctrl Pts',(56.6700953906675,19.9080241458768,10.9453989241804));
#25006=CARTESIAN_POINT('Ctrl Pts',(56.6974714155697,19.9510863281705,10.9487557684769));
#25007=CARTESIAN_POINT('Ctrl Pts',(56.8091290265989,20.1425616553439,10.9635848454274));
#25008=CARTESIAN_POINT('Ctrl Pts',(56.8758127496346,20.3003868733724,10.9756441788885));
#25009=CARTESIAN_POINT('Ctrl Pts',(56.9291081246865,20.4917145876265,10.9893610976861));
#25010=CARTESIAN_POINT('Ctrl Pts',(56.9360557960598,20.5188552390742,10.9912845861484));
#25011=CARTESIAN_POINT('Ctrl Pts',(56.9520588174631,20.5873440709998,10.9960696396937));
#25012=CARTESIAN_POINT('Ctrl Pts',(56.9603748341308,20.6288536002443,10.9989075895413));
#25013=CARTESIAN_POINT('Ctrl Pts',(56.9687234437182,20.6787161823642,11.0022188847232));
#25014=CARTESIAN_POINT('Ctrl Pts',(56.9700322187786,20.6868413311199,11.0027553807396));
#25015=CARTESIAN_POINT('Ctrl Pts',(56.9720918586113,20.7001521822417,11.0036289888374));
#25016=CARTESIAN_POINT('Ctrl Pts',(56.9728726285275,20.7053330596342,11.003967706459));
#25017=CARTESIAN_POINT('Ctrl Pts',(56.9742395924999,20.7146527275148,11.004574584836));
#25018=CARTESIAN_POINT('Ctrl Pts',(56.9748331954837,20.7187903175542,11.0048431527432));
#25019=CARTESIAN_POINT('Ctrl Pts',(56.9761050487182,20.7278581893583,11.0054298469648));
#25020=CARTESIAN_POINT('Ctrl Pts',(56.9767778552583,20.7327891451811,11.0057476655489));
#25021=CARTESIAN_POINT('Ctrl Pts',(56.9786477208445,20.7468869396925,11.006652981277));
#25022=CARTESIAN_POINT('Ctrl Pts',(56.9797995377598,20.7560597970045,11.0072380021392));
#25023=CARTESIAN_POINT('Ctrl Pts',(56.9871926395632,20.81844238832,11.0111912567426));
#25024=CARTESIAN_POINT('Ctrl Pts',(56.9913524696098,20.8718820089326,11.0144528132427));
#25025=CARTESIAN_POINT('Ctrl Pts',(57.0001561044924,21.1072124255164,11.0285193119082));
#25026=CARTESIAN_POINT('Ctrl Pts',(56.9820603494715,21.2890739800174,11.0386942731503));
#25027=CARTESIAN_POINT('Ctrl Pts',(56.9268088989984,21.5190520585236,11.05288844851));
#25028=CARTESIAN_POINT('Ctrl Pts',(56.9118843180983,21.5715812439113,11.0562176579839));
#25029=CARTESIAN_POINT('Ctrl Pts',(56.8903172671782,21.637131278653,11.0605151860148));
#25030=CARTESIAN_POINT('Ctrl Pts',(56.8856606196969,21.65078387111,11.0614182105881));
#25031=CARTESIAN_POINT('Ctrl Pts',(56.8780090932287,21.6724451575695,11.0628641821008));
#25032=CARTESIAN_POINT('Ctrl Pts',(56.8751100279728,21.680487342646,11.0634039551801));
#25033=CARTESIAN_POINT('Ctrl Pts',(56.869583038705,21.6955160229821,11.0644182524494));
#25034=CARTESIAN_POINT('Ctrl Pts',(56.8669674127983,21.7025069066608,11.0648923598461));
#25035=CARTESIAN_POINT('Ctrl Pts',(56.8610277556968,21.718114581362,11.0659560465079));
#25036=CARTESIAN_POINT('Ctrl Pts',(56.8576830101499,21.7267232544089,11.0665463111358));
#25037=CARTESIAN_POINT('Ctrl Pts',(56.8476261626221,21.7520843150178,11.0682959698374));
#25038=CARTESIAN_POINT('Ctrl Pts',(56.8407465073948,21.7687688298116,11.0694609705695));
#25039=CARTESIAN_POINT('Ctrl Pts',(56.7772639891107,21.9169869625614,11.0799384066852));
#25040=CARTESIAN_POINT('Ctrl Pts',(56.7068878785158,22.0421377925879,11.0897388464372));
#25041=CARTESIAN_POINT('Ctrl Pts',(56.547423800954,22.2656108585438,11.1088617377864));
#25042=CARTESIAN_POINT('Ctrl Pts',(56.4607182777498,22.3647706876262,11.1180995522249));
#25043=CARTESIAN_POINT('Ctrl Pts',(56.353748000368,22.465137231911,11.1278080420744));
#25044=CARTESIAN_POINT('Ctrl Pts',(56.3424916816967,22.4754581916811,11.1288108648397));
#25045=CARTESIAN_POINT('Ctrl Pts',(56.3264479063178,22.4898331534217,11.1302125882075));
#25046=CARTESIAN_POINT('Ctrl Pts',(56.3217584911805,22.493995102659,11.1306190305018));
#25047=CARTESIAN_POINT('Ctrl Pts',(56.3138310536264,22.5009643195365,11.1313005276575));
#25048=CARTESIAN_POINT('Ctrl Pts',(56.3106034944305,22.5037833645686,11.1315764455293));
#25049=CARTESIAN_POINT('Ctrl Pts',(56.303996286329,22.509516864062,11.1321380929205));
#25050=CARTESIAN_POINT('Ctrl Pts',(56.3006159044407,22.5124304108679,11.1324237564703));
#25051=CARTESIAN_POINT('Ctrl Pts',(56.2919804104933,22.5198229693003,11.133149311327));
#25052=CARTESIAN_POINT('Ctrl Pts',(56.2867117158611,22.5242861288953,11.1335880528652));
#25053=CARTESIAN_POINT('Ctrl Pts',(56.2652445372956,22.5422805519496,11.1353603070656));
#25054=CARTESIAN_POINT('Ctrl Pts',(56.2488542677394,22.555582251938,11.1366781445922));
#25055=CARTESIAN_POINT('Ctrl Pts',(56.2051633484334,22.5899043289703,11.1401086818659));
#25056=CARTESIAN_POINT('Ctrl Pts',(56.177523094036,22.6104825703722,11.1421966643194));
#25057=CARTESIAN_POINT('Ctrl Pts',(56.0190128724598,22.7222298954607,11.1538016024108));
#25058=CARTESIAN_POINT('Ctrl Pts',(55.8781088547683,22.7981642090705,11.1627836695983));
#25059=CARTESIAN_POINT('Ctrl Pts',(55.6583655650443,22.8845290961288,11.1767608648133));
#25060=CARTESIAN_POINT('Ctrl Pts',(55.5855267523175,22.9084159776087,11.1813810449807));
#25061=CARTESIAN_POINT('Ctrl Pts',(55.4974697671304,22.9317769309693,11.1870433802224));
#25062=CARTESIAN_POINT('Ctrl Pts',(55.4833990876776,22.9353458566353,11.1879503269007));
#25063=CARTESIAN_POINT('Ctrl Pts',(55.4602180578158,22.9409569915671,11.1894486027284));
#25064=CARTESIAN_POINT('Ctrl Pts',(55.4511299429852,22.9430894147258,11.1900370313199));
#25065=CARTESIAN_POINT('Ctrl Pts',(55.4347409688124,22.9468137263359,11.1911001638077));
#25066=CARTESIAN_POINT('Ctrl Pts',(55.4274454558664,22.9484285398212,11.1915741232999));
#25067=CARTESIAN_POINT('Ctrl Pts',(55.4118517250784,22.95178831408,11.1925887719289));
#25068=CARTESIAN_POINT('Ctrl Pts',(55.4035511311414,22.9535214222837,11.1931298297066));
#25069=CARTESIAN_POINT('Ctrl Pts',(55.3810414865539,22.9580716992059,11.1945997901621));
#25070=CARTESIAN_POINT('Ctrl Pts',(55.3668126078206,22.9607870578116,11.1955319107423));
#25071=CARTESIAN_POINT('Ctrl Pts',(55.2920186946362,22.9742177046213,11.2004478621077));
#25072=CARTESIAN_POINT('Ctrl Pts',(55.2310173881768,22.9822815330329,11.2045146079987));
#25073=CARTESIAN_POINT('Ctrl Pts',(55.1679803510715,22.9876652899753,11.208777821554));
#25074=CARTESIAN_POINT('Ctrl Pts',(55.1662144135544,22.9878137416641,11.2088972999258));
#25075=CARTESIAN_POINT('Ctrl Pts',(55.1644483504356,22.9879598342368,11.2090168340879));
#25076=CARTESIAN_POINT('Origin',(55.,21.,6.22095488139522));
#25077=CARTESIAN_POINT('',(55.1644487484638,22.9879598013111,12.1688212129648));
#25078=CARTESIAN_POINT('',(55.1644483513162,22.987959834164,12.0120574026292));
#25079=CARTESIAN_POINT('',(55.1644483516311,22.987959834138,6.22095488139522));
#25080=CARTESIAN_POINT('Ctrl Pts',(55.1644487484638,22.9879598013111,12.1688212129648));
#25081=CARTESIAN_POINT('Ctrl Pts',(55.2631352750185,22.9797962178365,12.1619316809086));
#25082=CARTESIAN_POINT('Ctrl Pts',(55.3611348208292,22.9642908938561,12.1549763628138));
#25083=CARTESIAN_POINT('Ctrl Pts',(55.5057090792001,22.9302138419902,12.1448260486904));
#25084=CARTESIAN_POINT('Ctrl Pts',(55.553351071021,22.9170995415923,12.1415015513099));
#25085=CARTESIAN_POINT('Ctrl Pts',(55.6091024829877,22.8995009454316,12.1376729441441));
#25086=CARTESIAN_POINT('Ctrl Pts',(55.6177253683065,22.8967142782554,12.1370825731292));
#25087=CARTESIAN_POINT('Ctrl Pts',(55.6310177236848,22.8923183087989,12.1361755929473));
#25088=CARTESIAN_POINT('Ctrl Pts',(55.6357005759918,22.890750308313,12.1358566619738));
#25089=CARTESIAN_POINT('Ctrl Pts',(55.6443402171008,22.8878216953807,12.1352694131176));
#25090=CARTESIAN_POINT('Ctrl Pts',(55.6482985248752,22.8864660325937,12.1350008209137));
#25091=CARTESIAN_POINT('Ctrl Pts',(55.6572523894426,22.8833679537104,12.1343942734837));
#25092=CARTESIAN_POINT('Ctrl Pts',(55.6622452898147,22.8816181148588,12.1340567605018));
#25093=CARTESIAN_POINT('Ctrl Pts',(55.6770460037066,22.8763647664406,12.1330582074837));
#25094=CARTESIAN_POINT('Ctrl Pts',(55.6868335866626,22.8728042244651,12.1324004275954));
#25095=CARTESIAN_POINT('Ctrl Pts',(55.7928628133062,22.8332897124292,12.1252978816355));
#25096=CARTESIAN_POINT('Ctrl Pts',(55.8862314384353,22.7900230343139,12.1192479228581));
#25097=CARTESIAN_POINT('Ctrl Pts',(56.0857559881973,22.678105529276,12.1059244111246));
#25098=CARTESIAN_POINT('Ctrl Pts',(56.1895574207462,22.6061929755261,12.0987010950092));
#25099=CARTESIAN_POINT('Ctrl Pts',(56.3313802924731,22.4866055976501,12.0875975717351));
#25100=CARTESIAN_POINT('Ctrl Pts',(56.3751359904194,22.4462260064698,12.0839740466369));
#25101=CARTESIAN_POINT('Ctrl Pts',(56.4271163297072,22.3937619531715,12.0793730888262));
#25102=CARTESIAN_POINT('Ctrl Pts',(56.4371036760274,22.3834617479255,12.0784746479543));
#25103=CARTESIAN_POINT('Ctrl Pts',(56.4527958218823,22.3669247523332,12.0770393254238));
#25104=CARTESIAN_POINT('Ctrl Pts',(56.4585737132153,22.3607577661646,12.0765056051589));
#25105=CARTESIAN_POINT('Ctrl Pts',(56.469390617376,22.349064381777,12.0754963839202));
#25106=CARTESIAN_POINT('Ctrl Pts',(56.4744380910323,22.3435459820297,12.0750212555272));
#25107=CARTESIAN_POINT('Ctrl Pts',(56.4857497723439,22.3310384156323,12.0739468639525));
#25108=CARTESIAN_POINT('Ctrl Pts',(56.4919958899653,22.3240331979445,12.0733468550987));
#25109=CARTESIAN_POINT('Ctrl Pts',(56.5078824515922,22.3059607545082,12.0718031844183));
#25110=CARTESIAN_POINT('Ctrl Pts',(56.5174504700025,22.2948308893866,12.0708565590061));
#25111=CARTESIAN_POINT('Ctrl Pts',(56.5788809417828,22.2217566477893,12.0646662578256));
#25112=CARTESIAN_POINT('Ctrl Pts',(56.6270557590762,22.1568236325913,12.0592757245517));
#25113=CARTESIAN_POINT('Ctrl Pts',(56.7560623550808,21.9588811601491,12.0431619940139));
#25114=CARTESIAN_POINT('Ctrl Pts',(56.8254348750708,21.8191394523889,12.0321326866493));
#25115=CARTESIAN_POINT('Ctrl Pts',(56.8950347166383,21.6248679264221,12.018017251915));
#25116=CARTESIAN_POINT('Ctrl Pts',(56.9103582040815,21.57632371177,12.014589430937));
#25117=CARTESIAN_POINT('Ctrl Pts',(56.9262227503621,21.5184369164717,12.0106582468343));
#25118=CARTESIAN_POINT('Ctrl Pts',(56.9285755338481,21.5096148921415,12.0100633606266));
#25119=CARTESIAN_POINT('Ctrl Pts',(56.9321111481933,21.4959824649405,12.0091509437773));
#25120=CARTESIAN_POINT('Ctrl Pts',(56.9333367362451,21.4911834281402,12.0088310481817));
#25121=CARTESIAN_POINT('Ctrl Pts',(56.935564374119,21.4823231416446,12.0082429020439));
#25122=CARTESIAN_POINT('Ctrl Pts',(56.9365715195632,21.4782633265508,12.0079743705631));
#25123=CARTESIAN_POINT('Ctrl Pts',(56.9388191724453,21.4690794941811,12.0073690629039));
#25124=CARTESIAN_POINT('Ctrl Pts',(56.940052139632,21.4639537178982,12.0070327210953));
#25125=CARTESIAN_POINT('Ctrl Pts',(56.9431817507256,21.4507124391296,12.0061675805054));
#25126=CARTESIAN_POINT('Ctrl Pts',(56.9450479048463,21.44258973409,12.0056404708632));
#25127=CARTESIAN_POINT('Ctrl Pts',(56.9564835935697,21.3913446108047,12.0023362793467));
#25128=CARTESIAN_POINT('Ctrl Pts',(56.9646702776822,21.3479224306536,11.9996311563216));
#25129=CARTESIAN_POINT('Ctrl Pts',(57.0009287208087,21.1129916093255,11.9853285054397));
#25130=CARTESIAN_POINT('Ctrl Pts',(57.002459280579,20.9184382887348,11.9745642776035));
#25131=CARTESIAN_POINT('Ctrl Pts',(56.9685782559503,20.6734833533486,11.9597044830606));
#25132=CARTESIAN_POINT('Ctrl Pts',(56.9590718734489,20.6205924524478,11.9564240929527));
#25133=CARTESIAN_POINT('Ctrl Pts',(56.9444341814658,20.5545828035843,11.9522093335986));
#25134=CARTESIAN_POINT('Ctrl Pts',(56.9412833107636,20.5410448205084,11.9513385026714));
#25135=CARTESIAN_POINT('Ctrl Pts',(56.9360129961446,20.5194263800957,11.9499371244364));
#25136=CARTESIAN_POINT('Ctrl Pts',(56.9339837933855,20.5113242292975,11.949409481457));
#25137=CARTESIAN_POINT('Ctrl Pts',(56.930037186238,20.4959759906576,11.948405214584));
#25138=CARTESIAN_POINT('Ctrl Pts',(56.9281297031506,20.4887274820909,11.9479289185434));
#25139=CARTESIAN_POINT('Ctrl Pts',(56.9236996635051,20.4722705965353,11.9468428849412));
#25140=CARTESIAN_POINT('Ctrl Pts',(56.9211517703889,20.4630692888816,11.9462323356768));
#25141=CARTESIAN_POINT('Ctrl Pts',(56.9143732180348,20.4392557114714,11.9446433785994));
#25142=CARTESIAN_POINT('Ctrl Pts',(56.9100413479069,20.4246731337317,11.9436617064761));
#25143=CARTESIAN_POINT('Ctrl Pts',(56.8768638605763,20.3174928965863,11.9363810722413));
#25144=CARTESIAN_POINT('Ctrl Pts',(56.8414702849752,20.2270730508161,11.9298672252395));
#25145=CARTESIAN_POINT('Ctrl Pts',(56.7390874875415,20.012925949443,11.913553398416));
#25146=CARTESIAN_POINT('Ctrl Pts',(56.6653267350473,19.8930108129447,11.9036156675666));
#25147=CARTESIAN_POINT('Ctrl Pts',(56.5497295423518,19.7431162454355,11.8906845348243));
#25148=CARTESIAN_POINT('Ctrl Pts',(56.5184527152197,19.7055037017738,11.8873943900699));
#25149=CARTESIAN_POINT('Ctrl Pts',(56.4797918206915,19.6623433100878,11.8835999635599));
#25150=CARTESIAN_POINT('Ctrl Pts',(56.4737155448948,19.6556519227367,11.8830111386633));
#25151=CARTESIAN_POINT('Ctrl Pts',(56.4642526644052,19.6453723631457,11.8821060208406));
#25152=CARTESIAN_POINT('Ctrl Pts',(56.4608979710776,19.6417551696668,11.8817874208047));
#25153=CARTESIAN_POINT('Ctrl Pts',(56.4546730262615,19.6350928752721,11.8812004779104));
#25154=CARTESIAN_POINT('Ctrl Pts',(56.4518066300993,19.6320443787096,11.8809318630061));
#25155=CARTESIAN_POINT('Ctrl Pts',(56.4452898942278,19.625157193333,11.8803248818203));
#25156=CARTESIAN_POINT('Ctrl Pts',(56.4416338496469,19.6213240168501,11.8799869605258));
#25157=CARTESIAN_POINT('Ctrl Pts',(56.4307232213335,19.6099756364407,11.8789860687615));
#25158=CARTESIAN_POINT('Ctrl Pts',(56.4234246971968,19.6025026619261,11.8783263811014));
#25159=CARTESIAN_POINT('Ctrl Pts',(56.3520806048194,19.5305921082013,11.8719683946961));
#25160=CARTESIAN_POINT('Ctrl Pts',(56.2837531162298,19.470534778132,11.8665777618287));
#25161=CARTESIAN_POINT('Ctrl Pts',(56.1759874395737,19.388141999106,11.8586480939982));
#25162=CARTESIAN_POINT('Ctrl Pts',(56.1395085309533,19.3621498568731,11.8560524078389));
#25163=CARTESIAN_POINT('Ctrl Pts',(56.0180815137242,19.2816520487818,11.8476002153413));
#25164=CARTESIAN_POINT('Ctrl Pts',(55.929872459968,19.2323618024046,11.8417390465924));
#25165=CARTESIAN_POINT('Ctrl Pts',(55.8067839593314,19.1753534620842,11.8335813899607));
#25166=CARTESIAN_POINT('Ctrl Pts',(55.7748739955947,19.1615752852851,11.8314693778516));
#25167=CARTESIAN_POINT('Ctrl Pts',(55.7194552126707,19.1393455994197,11.8277944042415));
#25168=CARTESIAN_POINT('Ctrl Pts',(55.6961171861329,19.1304890002642,11.8262447550373));
#25169=CARTESIAN_POINT('Ctrl Pts',(55.6627193013234,19.1185268306655,11.8240214948683));
#25170=CARTESIAN_POINT('Ctrl Pts',(55.6527909697619,19.1150591249916,11.8233598839936));
#25171=CARTESIAN_POINT('Ctrl Pts',(55.6356022147318,19.1092076326856,11.8222130515602));
#25172=CARTESIAN_POINT('Ctrl Pts',(55.6283545910332,19.1067867375952,11.8217290650948));
#25173=CARTESIAN_POINT('Ctrl Pts',(55.6144331262706,19.1022253516083,11.8207985178666));
#25174=CARTESIAN_POINT('Ctrl Pts',(55.6077615511641,19.1000782706646,11.8203521822108));
#25175=CARTESIAN_POINT('Ctrl Pts',(55.592049001603,19.0951128054936,11.8193000155293));
#25176=CARTESIAN_POINT('Ctrl Pts',(55.5829990594267,19.092323576788,11.8186932399595));
#25177=CARTESIAN_POINT('Ctrl Pts',(55.5515695416394,19.0828814052565,11.8165831409066));
#25178=CARTESIAN_POINT('Ctrl Pts',(55.5290939720605,19.0765572123083,11.8150692063539));
#25179=CARTESIAN_POINT('Ctrl Pts',(55.3550051518577,19.0308540692414,11.8032999802397));
#25180=CARTESIAN_POINT('Ctrl Pts',(55.1993666428328,19.0090708120618,11.7924648842068));
#25181=CARTESIAN_POINT('Ctrl Pts',(54.9266520592972,19.0032154415543,11.7734384541342));
#25182=CARTESIAN_POINT('Ctrl Pts',(54.8104759586204,19.0108757590796,11.7653414698039));
#25183=CARTESIAN_POINT('Ctrl Pts',(54.6850157650914,19.0302468268437,11.757002340096));
#25184=CARTESIAN_POINT('Ctrl Pts',(54.6744274600482,19.0319692164764,11.7563018570637));
#25185=CARTESIAN_POINT('Ctrl Pts',(54.6586454189903,19.0346673240608,11.7552632279788));
#25186=CARTESIAN_POINT('Ctrl Pts',(54.6534410362598,19.0355783641739,11.7549216106729));
#25187=CARTESIAN_POINT('Ctrl Pts',(54.6441222428118,19.0372478284839,11.7543115881144));
#25188=CARTESIAN_POINT('Ctrl Pts',(54.6400065568597,19.0379985252868,11.754042757162));
#25189=CARTESIAN_POINT('Ctrl Pts',(54.6310323252322,19.0396646053923,11.7534578629229));
#25190=CARTESIAN_POINT('Ctrl Pts',(54.6261748188598,19.0405851027411,11.7531420923399));
#25191=CARTESIAN_POINT('Ctrl Pts',(54.6126437690227,19.0432013856596,11.7522646343666));
#25192=CARTESIAN_POINT('Ctrl Pts',(54.6039778708655,19.044936792102,11.751705138172));
#25193=CARTESIAN_POINT('Ctrl Pts',(54.55668379339,19.0547351275433,11.7486637735827));
#25194=CARTESIAN_POINT('Ctrl Pts',(54.5182869711783,19.0638859210863,11.7462386609306));
#25195=CARTESIAN_POINT('Ctrl Pts',(54.2887643883916,19.1258381876529,11.7318713474258));
#25196=CARTESIAN_POINT('Ctrl Pts',(54.1061075545412,19.2057563340643,11.7208729410609));
#25197=CARTESIAN_POINT('Ctrl Pts',(53.8923655121536,19.3401481864385,11.7057058333443));
#25198=CARTESIAN_POINT('Ctrl Pts',(53.8477022933176,19.3708372086715,11.7023986329782));
#25199=CARTESIAN_POINT('Ctrl Pts',(53.7931904249005,19.4116573287015,11.6981536438975));
#25200=CARTESIAN_POINT('Ctrl Pts',(53.7821229462194,19.4201274550495,11.6972805350793));
#25201=CARTESIAN_POINT('Ctrl Pts',(53.7645596536865,19.4338631567189,11.6958763563653));
#25202=CARTESIAN_POINT('Ctrl Pts',(53.7580064869741,19.4390549108523,11.6953482116631));
#25203=CARTESIAN_POINT('Ctrl Pts',(53.7456418386923,19.4489779750794,11.69434354872));
#25204=CARTESIAN_POINT('Ctrl Pts',(53.739823989157,19.4537011486096,11.6938673620792));
#25205=CARTESIAN_POINT('Ctrl Pts',(53.7266655285193,19.4645073193536,11.6927823525119));
#25206=CARTESIAN_POINT('Ctrl Pts',(53.719341678164,19.4706103485131,11.6921727236547));
#25207=CARTESIAN_POINT('Ctrl Pts',(53.7004814143636,19.4865572378919,11.6905877362977));
#25208=CARTESIAN_POINT('Ctrl Pts',(53.6890131821451,19.4964804321471,11.6896091403857));
#25209=CARTESIAN_POINT('Ctrl Pts',(53.6062910070647,19.5697240323046,11.6824399163084));
#25210=CARTESIAN_POINT('Ctrl Pts',(53.5395545496119,19.6379396451916,11.6760420244124));
#25211=CARTESIAN_POINT('Ctrl Pts',(53.386222364542,19.8189448489081,11.6597497655824));
#25212=CARTESIAN_POINT('Ctrl Pts',(53.3063122174673,19.9367085869422,11.6497020523071));
#25213=CARTESIAN_POINT('Ctrl Pts',(53.2164807616161,20.1052940678408,11.6366505789264));
#25214=CARTESIAN_POINT('Ctrl Pts',(53.1949916236563,20.1494794311572,11.6333454799807));
#25215=CARTESIAN_POINT('Ctrl Pts',(53.1714996054309,20.2026946978422,11.6295361693965));
#25216=CARTESIAN_POINT('Ctrl Pts',(53.1679016374288,20.2109974428874,11.6289466686373));
#25217=CARTESIAN_POINT('Ctrl Pts',(53.1624286361944,20.223866374661,11.6280407366684));
#25218=CARTESIAN_POINT('Ctrl Pts',(53.16051389935,20.2284153913823,11.6277219919289));
#25219=CARTESIAN_POINT('Ctrl Pts',(53.1570070772543,20.236834121825,11.6271349153711));
#25220=CARTESIAN_POINT('Ctrl Pts',(53.1554102933403,20.2407017150396,11.6268663105117));
#25221=CARTESIAN_POINT('Ctrl Pts',(53.1518206883696,20.2494743020717,11.626259519524));
#25222=CARTESIAN_POINT('Ctrl Pts',(53.1498352205134,20.2543822148745,11.6259217771807));
#25223=CARTESIAN_POINT('Ctrl Pts',(53.1439956610321,20.2689840764529,11.6249219107452));
#25224=CARTESIAN_POINT('Ctrl Pts',(53.140197976249,20.2787005959249,11.6242630595177));
#25225=CARTESIAN_POINT('Ctrl Pts',(53.1051685963822,20.3704408350954,11.6180992784536));
#25226=CARTESIAN_POINT('Ctrl Pts',(53.0793019958035,20.4544232310117,11.6128812400732));
#25227=CARTESIAN_POINT('Ctrl Pts',(53.0233811802809,20.6902999501212,11.5986941594621));
#25228=CARTESIAN_POINT('Ctrl Pts',(53.0053276029801,20.8443816608655,11.5899035048977));
#25229=CARTESIAN_POINT('Ctrl Pts',(53.0052267963372,21.0458823035609,11.5777423438057));
#25230=CARTESIAN_POINT('Ctrl Pts',(53.0068559918777,21.0927456276598,11.5748714783639));
#25231=CARTESIAN_POINT('Ctrl Pts',(53.0111010944751,21.1532965630707,11.571087290186));
#25232=CARTESIAN_POINT('Ctrl Pts',(53.0122112894115,21.1670769866418,11.5702210738776));
#25233=CARTESIAN_POINT('Ctrl Pts',(53.0142203551788,21.1891461151503,11.5688253687914));
#25234=CARTESIAN_POINT('Ctrl Pts',(53.0150281160256,21.1974428197599,11.5682987422623));
#25235=CARTESIAN_POINT('Ctrl Pts',(53.0166612389442,21.2131927550693,11.5672952700931));
#25236=CARTESIAN_POINT('Ctrl Pts',(53.0174766734884,21.2206468881253,11.5668187446811));
#25237=CARTESIAN_POINT('Ctrl Pts',(53.0194291890744,21.2376100560971,11.5657305989657));
#25238=CARTESIAN_POINT('Ctrl Pts',(53.0205927522274,21.247115798819,11.565118155073));
#25239=CARTESIAN_POINT('Ctrl Pts',(53.0243657875763,21.2762013682682,11.5632358170011));
#25240=CARTESIAN_POINT('Ctrl Pts',(53.0271976154137,21.295750641479,11.56195896434));
#25241=CARTESIAN_POINT('Ctrl Pts',(53.0502114716813,21.4395392708815,11.5524782485069));
#25242=CARTESIAN_POINT('Ctrl Pts',(53.0818186012838,21.5616403593145,11.5439076383811));
#25243=CARTESIAN_POINT('Ctrl Pts',(53.1750397041502,21.8187499082045,11.5249080522552));
#25244=CARTESIAN_POINT('Ctrl Pts',(53.2406323403614,21.9515579530286,11.5144672985571));
#25245=CARTESIAN_POINT('Ctrl Pts',(53.3278687800013,22.0877510381737,11.5037808844716));
#25246=CARTESIAN_POINT('Ctrl Pts',(53.3355754483629,22.0995071971577,11.5028589530587));
#25247=CARTESIAN_POINT('Ctrl Pts',(53.3464559242026,22.1157282503815,11.50158867378));
#25248=CARTESIAN_POINT('Ctrl Pts',(53.3495246000604,22.1202626902689,11.5012337768756));
#25249=CARTESIAN_POINT('Ctrl Pts',(53.3548392649776,22.1280466839637,11.5006249677821));
#25250=CARTESIAN_POINT('Ctrl Pts',(53.3570762882495,22.1313022775959,11.5003704657262));
#25251=CARTESIAN_POINT('Ctrl Pts',(53.3617795141683,22.1381036228022,11.4998390829897));
#25252=CARTESIAN_POINT('Ctrl Pts',(53.3642475806087,22.1416480365481,11.4995623393017));
#25253=CARTESIAN_POINT('Ctrl Pts',(53.3702968201381,22.150275519039,11.4988890798134));
#25254=CARTESIAN_POINT('Ctrl Pts',(53.3738903247223,22.1553499688855,11.4984933962833));
#25255=CARTESIAN_POINT('Ctrl Pts',(53.3868549564786,22.1734772345215,11.4970806984183));
#25256=CARTESIAN_POINT('Ctrl Pts',(53.3963602867035,22.186433925702,11.496072426503));
#25257=CARTESIAN_POINT('Ctrl Pts',(53.420324791419,22.2182855952533,11.493593579931));
#25258=CARTESIAN_POINT('Ctrl Pts',(53.4349677003432,22.2370398378151,11.4921338590358));
#25259=CARTESIAN_POINT('Ctrl Pts',(53.4977850239629,22.3145931696544,11.4860757324437));
#25260=CARTESIAN_POINT('Ctrl Pts',(53.5489675929747,22.3708799375397,11.4816234613602));
#25261=CARTESIAN_POINT('Ctrl Pts',(53.7220832589124,22.540670525554,11.46751839284));
#25262=CARTESIAN_POINT('Ctrl Pts',(53.8550317554083,22.6418826472947,11.4579769379792));
#25263=CARTESIAN_POINT('Ctrl Pts',(54.0189056430745,22.7369545132371,11.4462934852197));
#25264=CARTESIAN_POINT('Ctrl Pts',(54.0390081523801,22.748156663136,11.444862853427));
#25265=CARTESIAN_POINT('Ctrl Pts',(54.0673804807265,22.7633299115681,11.4428451775209));
#25266=CARTESIAN_POINT('Ctrl Pts',(54.0754912062399,22.7675958334768,11.4422685614604));
#25267=CARTESIAN_POINT('Ctrl Pts',(54.0904066352814,22.7753100191394,11.441208349367));
#25268=CARTESIAN_POINT('Ctrl Pts',(54.0972023069245,22.7787754428094,11.4407253669514));
#25269=CARTESIAN_POINT('Ctrl Pts',(54.1110209980808,22.7857226382097,11.4397432935432));
#25270=CARTESIAN_POINT('Ctrl Pts',(54.1180449924229,22.7892021596768,11.4392441346096));
#25271=CARTESIAN_POINT('Ctrl Pts',(54.135450481615,22.7976970324064,11.4380071849368));
#25272=CARTESIAN_POINT('Ctrl Pts',(54.1458551944191,22.8026638987656,11.437267728263));
#25273=CARTESIAN_POINT('Ctrl Pts',(54.1849348252037,22.820904930627,11.4344898729507));
#25274=CARTESIAN_POINT('Ctrl Pts',(54.2138795093055,22.8335867555719,11.4324313528172));
#25275=CARTESIAN_POINT('Ctrl Pts',(54.2870555953743,22.8635969719461,11.4272214950505));
#25276=CARTESIAN_POINT('Ctrl Pts',(54.3316258143947,22.8800422215631,11.4240429056687));
#25277=CARTESIAN_POINT('Ctrl Pts',(54.5558123335365,22.9537814554232,11.4080368618407));
#25278=CARTESIAN_POINT('Ctrl Pts',(54.7423048084404,22.9869941550036,11.3945496455318));
#25279=CARTESIAN_POINT('Ctrl Pts',(54.9611802109403,22.9946058451654,11.3797971648179));
#25280=CARTESIAN_POINT('Ctrl Pts',(54.9917110429182,22.9949664133274,11.3777663921631));
#25281=CARTESIAN_POINT('Ctrl Pts',(55.0304528559179,22.9945344431834,11.3752335181439));
#25282=CARTESIAN_POINT('Ctrl Pts',(55.0386652157354,22.9943921450433,11.3746991235355));
#25283=CARTESIAN_POINT('Ctrl Pts',(55.0516287285123,22.9940874182917,11.3738597793968));
#25284=CARTESIAN_POINT('Ctrl Pts',(55.0563804709015,22.9939587260137,11.3735530148023));
#25285=CARTESIAN_POINT('Ctrl Pts',(55.0649191732513,22.9936969231477,11.3730034334469));
#25286=CARTESIAN_POINT('Ctrl Pts',(55.0687061802393,22.9935700091809,11.3727602815624));
#25287=CARTESIAN_POINT('Ctrl Pts',(55.0778224251352,22.9932384890046,11.3721763571656));
#25288=CARTESIAN_POINT('Ctrl Pts',(55.0831512263136,22.9930233011828,11.3718361784439));
#25289=CARTESIAN_POINT('Ctrl Pts',(55.0994459130319,22.9922998216434,11.3707992986495));
#25290=CARTESIAN_POINT('Ctrl Pts',(55.1104087390921,22.9917223682492,11.3701063239169));
#25291=CARTESIAN_POINT('Ctrl Pts',(55.1357406157966,22.9901782406948,11.3685146017251));
#25292=CARTESIAN_POINT('Ctrl Pts',(55.1501020651774,22.9891465902058,11.3676193066293));
#25293=CARTESIAN_POINT('Ctrl Pts',(55.1644483680005,22.9879598327838,11.3667309363937));
#25294=CARTESIAN_POINT('',(53.0052509133734,21.0017010510026,11.4203138250391));
#25295=CARTESIAN_POINT('Ctrl Pts',(55.1644483504356,22.9879598342368,11.2090168340879));
#25296=CARTESIAN_POINT('Ctrl Pts',(55.0092635275445,23.0007970594652,11.2195203588896));
#25297=CARTESIAN_POINT('Ctrl Pts',(54.8531129331955,22.9954176987343,11.2305157839018));
#25298=CARTESIAN_POINT('Ctrl Pts',(54.6305636587255,22.9614701310944,11.2460703318392));
#25299=CARTESIAN_POINT('Ctrl Pts',(54.5625115666673,22.9474224762946,11.2508003530778));
#25300=CARTESIAN_POINT('Ctrl Pts',(54.4854643150143,22.9272738401728,11.2560279776748));
#25301=CARTESIAN_POINT('Ctrl Pts',(54.4756241844518,22.9246198172001,11.2566931689445));
#25302=CARTESIAN_POINT('Ctrl Pts',(54.4607540810592,22.9204866257303,11.257694208272));
#25303=CARTESIAN_POINT('Ctrl Pts',(54.4557090645972,22.9190629014876,11.2580331020069));
#25304=CARTESIAN_POINT('Ctrl Pts',(54.4466511940752,22.9164681407743,11.2586401657986));
#25305=CARTESIAN_POINT('Ctrl Pts',(54.4426363755956,22.9153043692301,11.2589087441613));
#25306=CARTESIAN_POINT('Ctrl Pts',(54.4338518252682,22.9127280389225,11.2594953090228));
#25307=CARTESIAN_POINT('Ctrl Pts',(54.4290837170337,22.9113102589005,11.2598129887718));
#25308=CARTESIAN_POINT('Ctrl Pts',(54.415479625998,22.9072096803969,11.2607175110254));
#25309=CARTESIAN_POINT('Ctrl Pts',(54.4066567611096,22.9044833003496,11.2613018840446));
#25310=CARTESIAN_POINT('Ctrl Pts',(54.3474294313881,22.8857297414347,11.2652115678339));
#25311=CARTESIAN_POINT('Ctrl Pts',(54.2976558442485,22.8677630411592,11.2684329772281));
#25312=CARTESIAN_POINT('Ctrl Pts',(54.0869222641937,22.7820766527148,11.2820281991051));
#25313=CARTESIAN_POINT('Ctrl Pts',(53.9345226912043,22.6953683437328,11.2918141232181));
#25314=CARTESIAN_POINT('Ctrl Pts',(53.7462401284685,22.5527105818578,11.3059240181889));
#25315=CARTESIAN_POINT('Ctrl Pts',(53.698884397953,22.5132485020501,11.3096683678554));
#25316=CARTESIAN_POINT('Ctrl Pts',(53.6424043636519,22.4615694097543,11.3144326163687));
#25317=CARTESIAN_POINT('Ctrl Pts',(53.631489121791,22.4513541981226,11.3153679983759));
#25318=CARTESIAN_POINT('Ctrl Pts',(53.6144273536599,22.4350230512437,11.3168540796457));
#25319=CARTESIAN_POINT('Ctrl Pts',(53.6082039736144,22.4289879401122,11.317401292947));
#25320=CARTESIAN_POINT('Ctrl Pts',(53.596702403059,22.4176879038426,11.3184223765349));
#25321=CARTESIAN_POINT('Ctrl Pts',(53.5914139873357,22.4124335668404,11.3188957780785));
#25322=CARTESIAN_POINT('Ctrl Pts',(53.5811203974231,22.4020910014361,11.319824986378));
#25323=CARTESIAN_POINT('Ctrl Pts',(53.5761128289944,22.3970053059946,11.3202806768769));
#25324=CARTESIAN_POINT('Ctrl Pts',(53.5615285935287,22.3820336534091,11.3216186867654));
#25325=CARTESIAN_POINT('Ctrl Pts',(53.5520269790321,22.3720754794033,11.3225042432158));
#25326=CARTESIAN_POINT('Ctrl Pts',(53.5039366997201,22.3206185538755,11.3270587020972));
#25327=CARTESIAN_POINT('Ctrl Pts',(53.4670293770656,22.2775910017095,11.3307976974811));
#25328=CARTESIAN_POINT('Ctrl Pts',(53.3753119724221,22.1609600345688,11.3407643108629));
#25329=CARTESIAN_POINT('Ctrl Pts',(53.3236629926683,22.0850486193954,11.3470932208943));
#25330=CARTESIAN_POINT('Ctrl Pts',(53.2104036821105,21.8910876756606,11.3627353059699));
#25331=CARTESIAN_POINT('Ctrl Pts',(53.1550175119223,21.7698944862666,11.3720849517102));
#25332=CARTESIAN_POINT('Ctrl Pts',(53.1071866309821,21.629695378185,11.3818884861442));
#25333=CARTESIAN_POINT('Ctrl Pts',(53.1024419563184,21.6152497246356,11.3828868498333));
#25334=CARTESIAN_POINT('Ctrl Pts',(53.0959778487469,21.594782633348,11.3842834524343));
#25335=CARTESIAN_POINT('Ctrl Pts',(53.0941210194638,21.5888056109612,11.3846891610648));
#25336=CARTESIAN_POINT('Ctrl Pts',(53.0910409042435,21.5787236629315,11.385369784152));
#25337=CARTESIAN_POINT('Ctrl Pts',(53.0898026629017,21.5746233913022,11.385645556742));
#25338=CARTESIAN_POINT('Ctrl Pts',(53.0873003698219,21.5662399050228,11.3862072539579));
#25339=CARTESIAN_POINT('Ctrl Pts',(53.0860374807261,21.5619563871821,11.3864931106972));
#25340=CARTESIAN_POINT('Ctrl Pts',(53.0828546444564,21.5510255171634,11.3872197525877));
#25341=CARTESIAN_POINT('Ctrl Pts',(53.0809548588042,21.5443722846421,11.387659381144));
#25342=CARTESIAN_POINT('Ctrl Pts',(53.0733688615912,21.5172720962352,11.3894398270361));
#25343=CARTESIAN_POINT('Ctrl Pts',(53.0679742709805,21.4967440319597,11.3907647861303));
#25344=CARTESIAN_POINT('Ctrl Pts',(53.0247486871252,21.3208856877327,11.4019445983941));
#25345=CARTESIAN_POINT('Ctrl Pts',(53.0053872115722,21.1616005945455,11.410976491796));
#25346=CARTESIAN_POINT('Ctrl Pts',(53.0052507266776,21.0017026683888,11.4203134044792));
#25347=CARTESIAN_POINT('Ctrl Pts',(53.0052507252816,21.0017010321814,11.4203135000222));
#25348=CARTESIAN_POINT('Ctrl Pts',(53.0051572374266,20.892070636593,11.4267151440213));
#25349=CARTESIAN_POINT('Ctrl Pts',(53.0141013025501,20.782630020886,11.4332260894532));
#25350=CARTESIAN_POINT('Ctrl Pts',(53.0339269391734,20.6627682253071,11.4407719853798));
#25351=CARTESIAN_POINT('Ctrl Pts',(53.0359691189056,20.6510712981564,11.4415126386308));
#25352=CARTESIAN_POINT('Ctrl Pts',(53.0396035524338,20.631298114834,11.44277226009));
#25353=CARTESIAN_POINT('Ctrl Pts',(53.0411416071494,20.623212121656,11.4432895198122));
#25354=CARTESIAN_POINT('Ctrl Pts',(53.0440806736763,20.6082651601016,11.4442497712183));
#25355=CARTESIAN_POINT('Ctrl Pts',(53.0454678583589,20.6014015791052,11.4446923184997));
#25356=CARTESIAN_POINT('Ctrl Pts',(53.0484128523122,20.5872152918814,11.4456104047392));
#25357=CARTESIAN_POINT('Ctrl Pts',(53.0499758028653,20.5798937772887,11.4460861012174));
#25358=CARTESIAN_POINT('Ctrl Pts',(53.0536121467205,20.5633172314747,11.4471674519151));
#25359=CARTESIAN_POINT('Ctrl Pts',(53.0557103950992,20.5540678943392,11.4477738927616));
#25360=CARTESIAN_POINT('Ctrl Pts',(53.0612989868218,20.5302222059878,11.4493454596257));
#25361=CARTESIAN_POINT('Ctrl Pts',(53.0648881893086,20.5156498643212,11.450313734171));
#25362=CARTESIAN_POINT('Ctrl Pts',(53.091192792144,20.4138145658406,11.457136938735));
#25363=CARTESIAN_POINT('Ctrl Pts',(53.1196346496169,20.3281515108074,11.4631764553428));
#25364=CARTESIAN_POINT('Ctrl Pts',(53.1825251391162,20.1744208185732,11.4745572760756));
#25365=CARTESIAN_POINT('Ctrl Pts',(53.2152720838552,20.1058294333342,11.4798479270736));
#25366=CARTESIAN_POINT('Ctrl Pts',(53.2864244833405,19.9763591665243,11.4901526226349));
#25367=CARTESIAN_POINT('Ctrl Pts',(53.3243741494522,19.915352353179,11.4951581753171));
#25368=CARTESIAN_POINT('Ctrl Pts',(53.3934021762447,19.8166848419255,11.5033830221403));
#25369=CARTESIAN_POINT('Ctrl Pts',(53.422722308933,19.7778759107242,11.506654072731));
#25370=CARTESIAN_POINT('Ctrl Pts',(53.4591542392526,19.7331519687879,11.5104316678307));
#25371=CARTESIAN_POINT('Ctrl Pts',(53.4649222964603,19.7261687536437,11.511021733257));
#25372=CARTESIAN_POINT('Ctrl Pts',(53.4739073949583,19.7154404289153,11.5119282878644));
#25373=CARTESIAN_POINT('Ctrl Pts',(53.4770910215909,19.7116676765717,11.5122470962951));
#25374=CARTESIAN_POINT('Ctrl Pts',(53.4829980803338,19.7047200170124,11.512834143463));
#25375=CARTESIAN_POINT('Ctrl Pts',(53.4857174769498,19.7015418760913,11.5131026561841));
#25376=CARTESIAN_POINT('Ctrl Pts',(53.4918983824786,19.694364120022,11.5137090480604));
#25377=CARTESIAN_POINT('Ctrl Pts',(53.4953658095081,19.6903697108674,11.5140464850665));
#25378=CARTESIAN_POINT('Ctrl Pts',(53.5057066714863,19.6785525176881,11.5150448788717));
#25379=CARTESIAN_POINT('Ctrl Pts',(53.5126256456882,19.6707695680026,11.5157025761111));
#25380=CARTESIAN_POINT('Ctrl Pts',(53.5770610906316,19.5994211719596,11.5217371214622));
#25381=CARTESIAN_POINT('Ctrl Pts',(53.638565949665,19.5395626240716,11.5268404176045));
#25382=CARTESIAN_POINT('Ctrl Pts',(53.8391085800137,19.3681059569576,11.5422946471397));
#25383=CARTESIAN_POINT('Ctrl Pts',(53.9893551535685,19.2710285685206,11.5523818863077));
#25384=CARTESIAN_POINT('Ctrl Pts',(54.16915330935,19.1863995117723,11.5645463391755));
#25385=CARTESIAN_POINT('Ctrl Pts',(54.1879490573907,19.177906101846,11.5658177993362));
#25386=CARTESIAN_POINT('Ctrl Pts',(54.2219127987131,19.1631884818063,11.5681171483211));
#25387=CARTESIAN_POINT('Ctrl Pts',(54.2370323758092,19.1568568624621,11.5691413814286));
#25388=CARTESIAN_POINT('Ctrl Pts',(54.2604387865059,19.147392320132,11.5707287269994));
#25389=CARTESIAN_POINT('Ctrl Pts',(54.2686715640999,19.1441269658812,11.571287374166));
#25390=CARTESIAN_POINT('Ctrl Pts',(54.2831974580241,19.1384772460299,11.5722737427874));
#25391=CARTESIAN_POINT('Ctrl Pts',(54.2894814474216,19.1360696814637,11.5727006783515));
#25392=CARTESIAN_POINT('Ctrl Pts',(54.3036764827762,19.1307133979278,11.5736656611751));
#25393=CARTESIAN_POINT('Ctrl Pts',(54.3115942699557,19.1277830284518,11.5742043115461));
#25394=CARTESIAN_POINT('Ctrl Pts',(54.3329887459804,19.1200190074,11.575660977536));
#25395=CARTESIAN_POINT('Ctrl Pts',(54.3464990615563,19.1152801133211,11.5765821124985));
#25396=CARTESIAN_POINT('Ctrl Pts',(54.409170894297,19.0940521415599,11.580861762251));
#25397=CARTESIAN_POINT('Ctrl Pts',(54.4589086552098,19.0793397987693,11.5842778208237));
#25398=CARTESIAN_POINT('Ctrl Pts',(54.532199090119,19.0607334095589,11.5893430901695));
#25399=CARTESIAN_POINT('Ctrl Pts',(54.5553407059858,19.0552967725533,11.590946829943));
#25400=CARTESIAN_POINT('Ctrl Pts',(54.7053313614505,19.0228767757062,11.6013664212854));
#25401=CARTESIAN_POINT('Ctrl Pts',(54.8344518759403,19.0079071029959,11.6104798798371));
#25402=CARTESIAN_POINT('Ctrl Pts',(55.0404094597709,19.004199294438,11.6247792474022));
#25403=CARTESIAN_POINT('Ctrl Pts',(55.1167485002965,19.0072065845438,11.6300204205694));
#25404=CARTESIAN_POINT('Ctrl Pts',(55.2077268579707,19.0160383040455,11.6360659171033));
#25405=CARTESIAN_POINT('Ctrl Pts',(55.2227030327147,19.0176635375024,11.6370544377176));
#25406=CARTESIAN_POINT('Ctrl Pts',(55.2436759833015,19.0201802374449,11.6384281269656));
#25407=CARTESIAN_POINT('Ctrl Pts',(55.2496888517483,19.0209295725825,11.6388207273027));
#25408=CARTESIAN_POINT('Ctrl Pts',(55.2599508322496,19.0222559535175,11.6394885552299));
#25409=CARTESIAN_POINT('Ctrl Pts',(55.2642016426041,19.0228193198432,11.6397645393504));
#25410=CARTESIAN_POINT('Ctrl Pts',(55.2723993964584,19.0239326906237,11.6402954868059));
#25411=CARTESIAN_POINT('Ctrl Pts',(55.2763465275944,19.0244808176728,11.6405505581848));
#25412=CARTESIAN_POINT('Ctrl Pts',(55.2858459433756,19.0258290027477,11.6411631035316));
#25413=CARTESIAN_POINT('Ctrl Pts',(55.2913965855073,19.0266406658925,11.6415199309805));
#25414=CARTESIAN_POINT('Ctrl Pts',(55.3117878759537,19.0297103708436,11.6428270313982));
#25415=CARTESIAN_POINT('Ctrl Pts',(55.3266067684547,19.0321125660015,11.6437695879997));
#25416=CARTESIAN_POINT('Ctrl Pts',(55.4768775293681,19.058216271204,11.6532657208826));
#25417=CARTESIAN_POINT('Ctrl Pts',(55.6095814847158,19.0957001803611,11.6611569658742));
#25418=CARTESIAN_POINT('Ctrl Pts',(55.865579536064,19.1975478202201,11.6771490845713));
#25419=CARTESIAN_POINT('Ctrl Pts',(55.9881162101072,19.261701667652,11.685219061316));
#25420=CARTESIAN_POINT('Ctrl Pts',(56.1178032133245,19.3477720475628,11.6948743816671));
#25421=CARTESIAN_POINT('Ctrl Pts',(56.1324282389952,19.3577614416785,11.6959799994203));
#25422=CARTESIAN_POINT('Ctrl Pts',(56.1544180683807,19.3732146676621,11.6976690260852));
#25423=CARTESIAN_POINT('Ctrl Pts',(56.1618816593078,19.3785368954701,11.6982470465856));
#25424=CARTESIAN_POINT('Ctrl Pts',(56.1747712690332,19.3878630649504,11.6992536944825));
#25425=CARTESIAN_POINT('Ctrl Pts',(56.1802142029615,19.3918434574956,11.6996814088273));
#25426=CARTESIAN_POINT('Ctrl Pts',(56.1923543429414,19.4008163145345,11.7006413785659));
#25427=CARTESIAN_POINT('Ctrl Pts',(56.1990405505272,19.40582338065,11.7011741974879));
#25428=CARTESIAN_POINT('Ctrl Pts',(56.2167769579273,19.4192802584887,11.7025987324203));
#25429=CARTESIAN_POINT('Ctrl Pts',(56.2277703923831,19.4278037928207,11.7034933348982));
#25430=CARTESIAN_POINT('Ctrl Pts',(56.2760815680787,19.4660766001242,11.7074774426777));
#25431=CARTESIAN_POINT('Ctrl Pts',(56.3124111099828,19.4970423819774,11.7106152424014));
#25432=CARTESIAN_POINT('Ctrl Pts',(56.3706333108814,19.5503902479971,11.7158890542039));
#25433=CARTESIAN_POINT('Ctrl Pts',(56.3931733144877,19.5720391942206,11.7179962023984));
#25434=CARTESIAN_POINT('Ctrl Pts',(56.5286298779206,19.7084017366175,11.7310645854318));
#25435=CARTESIAN_POINT('Ctrl Pts',(56.6278131568691,19.8358901568559,11.7424877818989));
#25436=CARTESIAN_POINT('Ctrl Pts',(56.7283783599356,20.0035409787108,11.755865466038));
#25437=CARTESIAN_POINT('Ctrl Pts',(56.7453864953543,20.0336415783008,11.7582068080424));
#25438=CARTESIAN_POINT('Ctrl Pts',(56.7715301444128,20.0828543706097,11.7619216174066));
#25439=CARTESIAN_POINT('Ctrl Pts',(56.7811582356661,20.101695717181,11.7633179043396));
#25440=CARTESIAN_POINT('Ctrl Pts',(56.7935316211003,20.1268908157473,11.7651474646895));
#25441=CARTESIAN_POINT('Ctrl Pts',(56.7965458499883,20.1331099632523,11.7655960729122));
#25442=CARTESIAN_POINT('Ctrl Pts',(56.8014537776446,20.1433718562911,11.766331220129));
#25443=CARTESIAN_POINT('Ctrl Pts',(56.8033663054284,20.1474054545164,11.7666188973632));
#25444=CARTESIAN_POINT('Ctrl Pts',(56.8070878394178,20.1553228670937,11.7671810074644));
#25445=CARTESIAN_POINT('Ctrl Pts',(56.8088978946037,20.1592061336748,11.7674555013033));
#25446=CARTESIAN_POINT('Ctrl Pts',(56.8133239418719,20.1687821618061,11.7681295035288));
#25447=CARTESIAN_POINT('Ctrl Pts',(56.8159256810885,20.1744815350345,11.7685281428671));
#25448=CARTESIAN_POINT('Ctrl Pts',(56.8247646701282,20.1940882348842,11.7698912518608));
#25449=CARTESIAN_POINT('Ctrl Pts',(56.8308695340691,20.2080551427808,11.7708480402085));
#25450=CARTESIAN_POINT('Ctrl Pts',(56.8882789174613,20.3436113255428,11.7800103280332));
#25451=CARTESIAN_POINT('Ctrl Pts',(56.9275653013854,20.4699571327537,11.7876076710108));
#25452=CARTESIAN_POINT('Ctrl Pts',(56.9829277273967,20.739923636688,11.8035981121753));
#25453=CARTESIAN_POINT('Ctrl Pts',(56.9964983245879,20.8832562912275,11.811973697707));
#25454=CARTESIAN_POINT('Ctrl Pts',(56.9943352706789,21.0442697577232,11.8219654479741));
#25455=CARTESIAN_POINT('Ctrl Pts',(56.9938708842138,21.0617401814132,11.823056653864));
#25456=CARTESIAN_POINT('Ctrl Pts',(56.9928149652987,21.0883132223465,11.8247281066979));
#25457=CARTESIAN_POINT('Ctrl Pts',(56.9923904433903,21.0974219061135,11.8253031374082));
#25458=CARTESIAN_POINT('Ctrl Pts',(56.9915436669917,21.1132553857507,11.8263064701525));
#25459=CARTESIAN_POINT('Ctrl Pts',(56.9911497618781,21.1199815981227,11.8267338781739));
#25460=CARTESIAN_POINT('Ctrl Pts',(56.990189162716,21.1350739491969,11.82769561595));
#25461=CARTESIAN_POINT('Ctrl Pts',(56.9896037802113,21.1434387303775,11.8282305235063));
#25462=CARTESIAN_POINT('Ctrl Pts',(56.9878960213922,21.165814788267,11.8296665569888));
#25463=CARTESIAN_POINT('Ctrl Pts',(56.9866782750849,21.1798181036466,11.8305706518607));
#25464=CARTESIAN_POINT('Ctrl Pts',(56.9805393109561,21.2427041586252,11.8346558233155));
#25465=CARTESIAN_POINT('Ctrl Pts',(56.9739615287026,21.2914042809144,11.8378882491754));
#25466=CARTESIAN_POINT('Ctrl Pts',(56.9607006026724,21.3681109454481,11.8430925321384));
#25467=CARTESIAN_POINT('Ctrl Pts',(56.9551972352366,21.3963031285349,11.8450296427212));
#25468=CARTESIAN_POINT('Ctrl Pts',(56.9119954546371,21.5947264549333,11.8588307755259));
#25469=CARTESIAN_POINT('Ctrl Pts',(56.8527350294271,21.7594667432054,11.871254645442));
#25470=CARTESIAN_POINT('Ctrl Pts',(56.7605705553206,21.9381542627826,11.8849025633339));
#25471=CARTESIAN_POINT('Ctrl Pts',(56.7478401449521,21.9616637006251,11.8866999293232));
#25472=CARTESIAN_POINT('Ctrl Pts',(56.725984260694,22.0001566094142,11.889637457561));
#25473=CARTESIAN_POINT('Ctrl Pts',(56.7171271470828,22.0152878030526,11.8907907534902));
#25474=CARTESIAN_POINT('Ctrl Pts',(56.7047486629335,22.0358093173544,11.8923509123996));
#25475=CARTESIAN_POINT('Ctrl Pts',(56.7013993069672,22.0413017558374,11.8927680817718));
#25476=CARTESIAN_POINT('Ctrl Pts',(56.6957346523005,22.0504906346733,11.8934652157797));
#25477=CARTESIAN_POINT('Ctrl Pts',(56.6934337184912,22.054195819914,11.8937460997775));
#25478=CARTESIAN_POINT('Ctrl Pts',(56.6890484365095,22.0612060160192,11.8942770731162));
#25479=CARTESIAN_POINT('Ctrl Pts',(56.6869665056987,22.0645124887026,11.8945273224618));
#25480=CARTESIAN_POINT('Ctrl Pts',(56.6814899121684,22.0731538668655,11.8951808954572));
#25481=CARTESIAN_POINT('Ctrl Pts',(56.6780795409149,22.0784788378371,11.8955831908399));
#25482=CARTESIAN_POINT('Ctrl Pts',(56.6661729861896,22.0968765745039,11.8969718918525));
#25483=CARTESIAN_POINT('Ctrl Pts',(56.6575486488922,22.1098662764253,11.8979502247717));
#25484=CARTESIAN_POINT('Ctrl Pts',(56.5784345056262,22.2260459841081,11.9066936838913));
#25485=CARTESIAN_POINT('Ctrl Pts',(56.4985351391853,22.3225148223572,11.9139163581989));
#25486=CARTESIAN_POINT('Ctrl Pts',(56.3063961347223,22.5145504697821,11.9296762693822));
#25487=CARTESIAN_POINT('Ctrl Pts',(56.1915700024885,22.6064519239246,11.938199231451));
#25488=CARTESIAN_POINT('Ctrl Pts',(56.0511479447294,22.6954351446342,11.9484888866744));
#25489=CARTESIAN_POINT('Ctrl Pts',(56.0344255130896,22.7056893464353,11.9497114961709));
#25490=CARTESIAN_POINT('Ctrl Pts',(56.0093424929474,22.7205657396226,11.9515426309291));
#25491=CARTESIAN_POINT('Ctrl Pts',(56.0010952054297,22.7253773839345,11.9521442725404));
#25492=CARTESIAN_POINT('Ctrl Pts',(55.9863144022977,22.7338591680085,11.9532219162576));
#25493=CARTESIAN_POINT('Ctrl Pts',(55.9797941094481,22.7375520755519,11.9536970868383));
#25494=CARTESIAN_POINT('Ctrl Pts',(55.9659664286467,22.7452810971178,11.9547044167121));
#25495=CARTESIAN_POINT('Ctrl Pts',(55.9586542191973,22.7493082443502,11.9552368851356));
#25496=CARTESIAN_POINT('Ctrl Pts',(55.9391117640425,22.7599117826715,11.9566594913001));
#25497=CARTESIAN_POINT('Ctrl Pts',(55.9268379356385,22.7664064688035,11.9575525017668));
#25498=CARTESIAN_POINT('Ctrl Pts',(55.8722927082063,22.7945440224227,11.9615197257005));
#25499=CARTESIAN_POINT('Ctrl Pts',(55.8293271081332,22.8147999152168,11.9646417322663));
#25500=CARTESIAN_POINT('Ctrl Pts',(55.7565710933529,22.8459769336753,11.9699271254088));
#25501=CARTESIAN_POINT('Ctrl Pts',(55.7271679174722,22.8577559886089,11.9720626557149));
#25502=CARTESIAN_POINT('Ctrl Pts',(55.5349972932419,22.9294792850819,11.9860100040474));
#25503=CARTESIAN_POINT('Ctrl Pts',(55.3653019640875,22.9686690743636,11.9983679866657));
#25504=CARTESIAN_POINT('Ctrl Pts',(55.183281523058,22.9863345084838,12.0107810213343));
#25505=CARTESIAN_POINT('Ctrl Pts',(55.1738677419974,22.987180641727,12.0114204197375));
#25506=CARTESIAN_POINT('Ctrl Pts',(55.1644483513162,22.987959834164,12.0120574026292));
#25507=CARTESIAN_POINT('Origin',(55.,21.,6.22095488139522));
#25508=CARTESIAN_POINT('',(55.1641804122445,22.9848227319589,12.9685061347694));
#25509=CARTESIAN_POINT('',(55.1644480621455,22.9879598580848,12.8106050954514));
#25510=CARTESIAN_POINT('',(55.1644483516311,22.987959834138,6.22095488139522));
#25511=CARTESIAN_POINT('',(53.0027029554326,20.9989116431895,12.3790451186048));
#25512=CARTESIAN_POINT('Ctrl Pts',(53.0027029554326,20.9989116431895,12.3790451186048));
#25513=CARTESIAN_POINT('Ctrl Pts',(53.0022880654464,20.9358127580545,12.3830871152256));
#25514=CARTESIAN_POINT('Ctrl Pts',(53.0336285294611,20.2121000156345,12.429473543416));
#25515=CARTESIAN_POINT('Ctrl Pts',(53.9157199028027,18.906273152354,12.5182044031761));
#25516=CARTESIAN_POINT('Ctrl Pts',(56.1713030095069,18.9536850922569,12.6452376978851));
#25517=CARTESIAN_POINT('Ctrl Pts',(57.3544922361658,20.8746135909814,12.7722709925941));
#25518=CARTESIAN_POINT('Ctrl Pts',(56.5295840241903,22.6014213230593,12.8800271382222));
#25519=CARTESIAN_POINT('Ctrl Pts',(55.5256092840336,22.9540479213118,12.9454388522806));
#25520=CARTESIAN_POINT('Ctrl Pts',(55.1641804122445,22.9848227319589,12.9685061347694));
#25521=CARTESIAN_POINT('Ctrl Pts',(53.0052503456376,20.9988257252519,12.37758152771));
#25522=CARTESIAN_POINT('Ctrl Pts',(53.0051430199567,21.1811406948336,12.3666360704211));
#25523=CARTESIAN_POINT('Ctrl Pts',(53.0300289413803,21.3626262549886,12.3564518925146));
#25524=CARTESIAN_POINT('Ctrl Pts',(53.0957203442371,21.5970592726417,12.3418950490065));
#25525=CARTESIAN_POINT('Ctrl Pts',(53.1148994162989,21.6550995822071,12.338178036601));
#25526=CARTESIAN_POINT('Ctrl Pts',(53.1418726252789,21.7256716310185,12.333472085354));
#25527=CARTESIAN_POINT('Ctrl Pts',(53.147181766391,21.7391219334858,12.3325666701201));
#25528=CARTESIAN_POINT('Ctrl Pts',(53.1558339602003,21.7603624242075,12.3311227740389));
#25529=CARTESIAN_POINT('Ctrl Pts',(53.1590813119202,21.7681912384199,12.3305875209643));
#25530=CARTESIAN_POINT('Ctrl Pts',(53.1652864303741,21.7828854058785,12.3295769999928));
#25531=CARTESIAN_POINT('Ctrl Pts',(53.1682330963473,21.789755309888,12.3291021157517));
#25532=CARTESIAN_POINT('Ctrl Pts',(53.1749512600266,21.805178263954,12.3280304173673));
#25533=CARTESIAN_POINT('Ctrl Pts',(53.1787443842762,21.8137216460812,12.3274328729792));
#25534=CARTESIAN_POINT('Ctrl Pts',(53.1885960385503,21.835496878911,12.3258997374109));
#25535=CARTESIAN_POINT('Ctrl Pts',(53.1947394942185,21.8486894802329,12.3249612506893));
#25536=CARTESIAN_POINT('Ctrl Pts',(53.2345047469547,21.9316965807568,12.3189940258471));
#25537=CARTESIAN_POINT('Ctrl Pts',(53.2720221886558,21.9995609300389,12.3138306352353));
#25538=CARTESIAN_POINT('Ctrl Pts',(53.3980946607118,22.1992064979579,12.2977554127866));
#25539=CARTESIAN_POINT('Ctrl Pts',(53.4984918082965,22.3227482439987,12.2864988986357));
#25540=CARTESIAN_POINT('Ctrl Pts',(53.6371566220555,22.4570064550637,12.273293655286));
#25541=CARTESIAN_POINT('Ctrl Pts',(53.6624755690758,22.4802832691831,12.2709649059374));
#25542=CARTESIAN_POINT('Ctrl Pts',(53.6990670340759,22.5122175747127,12.2677276379227));
#25543=CARTESIAN_POINT('Ctrl Pts',(53.7098484448114,22.5214261615813,12.2667889012373));
#25544=CARTESIAN_POINT('Ctrl Pts',(53.7288695699239,22.5373248197416,12.2651602551429));
#25545=CARTESIAN_POINT('Ctrl Pts',(53.7370660771486,22.5440654422756,12.2644671840838));
#25546=CARTESIAN_POINT('Ctrl Pts',(53.7494236672406,22.5540638062983,12.2634357688251));
#25547=CARTESIAN_POINT('Ctrl Pts',(53.7535443801015,22.5573708188114,12.2630940574513));
#25548=CARTESIAN_POINT('Ctrl Pts',(53.7608641446128,22.5631975166084,12.2624910566183));
#25549=CARTESIAN_POINT('Ctrl Pts',(53.7640578209501,22.565723818292,12.2622293007716));
#25550=CARTESIAN_POINT('Ctrl Pts',(53.7710471285791,22.5712178764809,12.2616593827586));
#25551=CARTESIAN_POINT('Ctrl Pts',(53.7748457799041,22.5741816647757,12.2613515004976));
#25552=CARTESIAN_POINT('Ctrl Pts',(53.7852075692985,22.582205926672,12.2605166176702));
#25553=CARTESIAN_POINT('Ctrl Pts',(53.7917916526752,22.5872393767951,12.2599914797352));
#25554=CARTESIAN_POINT('Ctrl Pts',(53.8242569793778,22.6117396467035,12.2574272292566));
#25555=CARTESIAN_POINT('Ctrl Pts',(53.8505798941841,22.6306164603011,12.2554259711973));
#25556=CARTESIAN_POINT('Ctrl Pts',(54.0473379179107,22.7645828929135,12.2409354831692));
#25557=CARTESIAN_POINT('Ctrl Pts',(54.2342093319486,22.8533491080173,12.2295753213666));
#25558=CARTESIAN_POINT('Ctrl Pts',(54.4838990902971,22.9276075138342,12.2139335296876));
#25559=CARTESIAN_POINT('Ctrl Pts',(54.5370451251463,22.9410571444666,12.2105889408114));
#25560=CARTESIAN_POINT('Ctrl Pts',(54.6043639199794,22.9551714260069,12.2063018116373));
#25561=CARTESIAN_POINT('Ctrl Pts',(54.6180832965096,22.9578975531699,12.2054255616982));
#25562=CARTESIAN_POINT('Ctrl Pts',(54.6400578522198,22.962024286006,12.2040175211832));
#25563=CARTESIAN_POINT('Ctrl Pts',(54.6482953090117,22.9635176229156,12.2034886846738));
#25564=CARTESIAN_POINT('Ctrl Pts',(54.6639215644729,22.966248959863,12.2024834715809));
#25565=CARTESIAN_POINT('Ctrl Pts',(54.6713084315377,22.9674972775839,12.2020074317473));
#25566=CARTESIAN_POINT('Ctrl Pts',(54.6880919877947,22.9702364003703,12.2009238146141));
#25567=CARTESIAN_POINT('Ctrl Pts',(54.6974926081884,22.9717016392285,12.2003154392419));
#25568=CARTESIAN_POINT('Ctrl Pts',(54.7218407252643,22.9753184637094,12.1987358533831));
#25569=CARTESIAN_POINT('Ctrl Pts',(54.7368025956508,22.9773676240688,12.1977614419176));
#25570=CARTESIAN_POINT('Ctrl Pts',(54.8441954606282,22.9908355852994,12.1907390709385));
#25571=CARTESIAN_POINT('Ctrl Pts',(54.9372894314649,22.9959369468908,12.1844936593506));
#25572=CARTESIAN_POINT('Ctrl Pts',(55.0751646497579,22.993836315959,12.1750325650663));
#25573=CARTESIAN_POINT('Ctrl Pts',(55.119876720263,22.9916469051696,12.1719328881632));
#25574=CARTESIAN_POINT('Ctrl Pts',(55.1644487484638,22.9879598013111,12.1688212129648));
#25575=CARTESIAN_POINT('Ctrl Pts',(55.1644483513162,22.987959834164,12.0120574026292));
#25576=CARTESIAN_POINT('Ctrl Pts',(55.1472821333312,22.9893798609661,12.0132182619184));
#25577=CARTESIAN_POINT('Ctrl Pts',(55.1300972845231,22.9905775594477,12.0143711020113));
#25578=CARTESIAN_POINT('Ctrl Pts',(55.0954212548586,22.9925432918177,12.0166759024132));
#25579=CARTESIAN_POINT('Ctrl Pts',(55.0779313521235,22.9933039759507,12.0178274312678));
#25580=CARTESIAN_POINT('Ctrl Pts',(55.054006748931,22.9940291292229,12.0193856079272));
#25581=CARTESIAN_POINT('Ctrl Pts',(55.0475794876185,22.9941928422897,12.019802528981));
#25582=CARTESIAN_POINT('Ctrl Pts',(55.0367917232815,22.9944154398785,12.0204993644048));
#25583=CARTESIAN_POINT('Ctrl Pts',(55.0324316603022,22.9944911045778,12.0207801964675));
#25584=CARTESIAN_POINT('Ctrl Pts',(55.0241637830745,22.994607466636,12.021311158452));
#25585=CARTESIAN_POINT('Ctrl Pts',(55.0202560514173,22.9946509788424,12.02156144789));
#25586=CARTESIAN_POINT('Ctrl Pts',(55.0100215272797,22.9947348597406,12.0222152855486));
#25587=CARTESIAN_POINT('Ctrl Pts',(55.003694564455,22.9947566128423,12.0226178038764));
#25588=CARTESIAN_POINT('Ctrl Pts',(54.9817553038484,22.994727659288,12.0240080647338));
#25589=CARTESIAN_POINT('Ctrl Pts',(54.9661433147736,22.9945237687374,12.0249877104127));
#25590=CARTESIAN_POINT('Ctrl Pts',(54.825889647723,22.9910447290102,12.0337145852198));
#25591=CARTESIAN_POINT('Ctrl Pts',(54.7017906309722,22.9762726086229,12.0409219973607));
#25592=CARTESIAN_POINT('Ctrl Pts',(54.4789042336405,22.9282515429392,12.0541494699615));
#25593=CARTESIAN_POINT('Ctrl Pts',(54.3797853415393,22.8986907346663,12.0601408996262));
#25594=CARTESIAN_POINT('Ctrl Pts',(54.2336163804897,22.8424250740349,12.0695551386846));
#25595=CARTESIAN_POINT('Ctrl Pts',(54.1846185782496,22.8212705399329,12.0728136520983));
#25596=CARTESIAN_POINT('Ctrl Pts',(54.1240302640645,22.7921765732984,12.0770035744064));
#25597=CARTESIAN_POINT('Ctrl Pts',(54.1115932251664,22.786044018273,12.0778723665361));
#25598=CARTESIAN_POINT('Ctrl Pts',(54.0917769643718,22.7760146664026,12.0792711390396));
#25599=CARTESIAN_POINT('Ctrl Pts',(54.0843563559767,22.7722002966523,12.079798233098));
#25600=CARTESIAN_POINT('Ctrl Pts',(54.0703162897619,22.764871645857,12.0808018921727));
#25601=CARTESIAN_POINT('Ctrl Pts',(54.0636922647943,22.7613663871871,12.0812781324664));
#25602=CARTESIAN_POINT('Ctrl Pts',(54.0486673785466,22.7533069097825,12.0823646454591));
#25603=CARTESIAN_POINT('Ctrl Pts',(54.0402792244526,22.7487295114629,12.0829757339127));
#25604=CARTESIAN_POINT('Ctrl Pts',(54.01859545913,22.7366937226092,12.0845673272026));
#25605=CARTESIAN_POINT('Ctrl Pts',(54.0053520827729,22.729142983772,12.0855511155753));
#25606=CARTESIAN_POINT('Ctrl Pts',(53.9092048496818,22.6728544070532,12.0927810882019));
#25607=CARTESIAN_POINT('Ctrl Pts',(53.8298476360918,22.6183369474405,12.0992383245163));
#25608=CARTESIAN_POINT('Ctrl Pts',(53.6445384740878,22.4702554054835,12.1155364253462));
#25609=CARTESIAN_POINT('Ctrl Pts',(53.5439956726429,22.3707574159044,12.1255220984236));
#25610=CARTESIAN_POINT('Ctrl Pts',(53.4238104694147,22.2235415691796,12.1385054764302));
#25611=CARTESIAN_POINT('Ctrl Pts',(53.3942355254379,22.1844613763546,12.1418019695838));
#25612=CARTESIAN_POINT('Ctrl Pts',(53.3609408221187,22.1369231764249,12.1456025885097));
#25613=CARTESIAN_POINT('Ctrl Pts',(53.3558046977686,22.1294826750636,12.1461915779772));
#25614=CARTESIAN_POINT('Ctrl Pts',(53.3479445483716,22.1179287459472,12.1470968365637));
#25615=CARTESIAN_POINT('Ctrl Pts',(53.3451849768813,22.1138398164948,12.1474154147054));
#25616=CARTESIAN_POINT('Ctrl Pts',(53.3401133638309,22.1062646230099,12.1480022489089));
#25617=CARTESIAN_POINT('Ctrl Pts',(53.3377971339463,22.1027813444625,12.1482707773721));
#25618=CARTESIAN_POINT('Ctrl Pts',(53.3325743898537,22.0948732448941,12.1488774708408));
#25619=CARTESIAN_POINT('Ctrl Pts',(53.3296745266765,22.0904441308392,12.1492151917903));
#25620=CARTESIAN_POINT('Ctrl Pts',(53.3211113419756,22.0772508150296,12.1502152117901));
#25621=CARTESIAN_POINT('Ctrl Pts',(53.3154990143388,22.0684535015435,12.1508742355331));
#25622=CARTESIAN_POINT('Ctrl Pts',(53.2629161331407,21.9845856670118,12.1570874647548));
#25623=CARTESIAN_POINT('Ctrl Pts',(53.2209181614938,21.9064994454913,12.1623495492353));
#25624=CARTESIAN_POINT('Ctrl Pts',(53.1070969862126,21.6562528897742,12.1784337506831));
#25625=CARTESIAN_POINT('Ctrl Pts',(53.0541010424324,21.4766798628353,12.1889940505051));
#25626=CARTESIAN_POINT('Ctrl Pts',(53.0234716469356,21.2699560697406,12.2018864856461));
#25627=CARTESIAN_POINT('Ctrl Pts',(53.0205338348667,21.2474959515836,12.2032950122899));
#25628=CARTESIAN_POINT('Ctrl Pts',(53.0168382884031,21.2149407027535,12.2053499169677));
#25629=CARTESIAN_POINT('Ctrl Pts',(53.0157738585393,21.2048816573873,12.2059866733096));
#25630=CARTESIAN_POINT('Ctrl Pts',(53.0140465266381,21.1872797183465,12.2071042769734));
#25631=CARTESIAN_POINT('Ctrl Pts',(53.0133499749683,21.179740275745,12.2075840586401));
#25632=CARTESIAN_POINT('Ctrl Pts',(53.0119987423176,21.1641458840986,12.2085787341071));
#25633=CARTESIAN_POINT('Ctrl Pts',(53.0113500551597,21.1560905683706,12.2090938066963));
#25634=CARTESIAN_POINT('Ctrl Pts',(53.0098098111806,21.1353927633548,12.2104206327715));
#25635=CARTESIAN_POINT('Ctrl Pts',(53.0089897726282,21.1227454693597,12.2112346092121));
#25636=CARTESIAN_POINT('Ctrl Pts',(53.0062447238034,21.0730836660248,12.2144439925563));
#25637=CARTESIAN_POINT('Ctrl Pts',(53.0052310952104,21.0360282642891,12.2168675498722));
#25638=CARTESIAN_POINT('Ctrl Pts',(53.0052817453659,20.9381172869696,12.2233515297983));
#25639=CARTESIAN_POINT('Ctrl Pts',(53.0080975985821,20.8773051181598,12.2274615491898));
#25640=CARTESIAN_POINT('Ctrl Pts',(53.0213795755411,20.7333595634598,12.2373681098823));
#25641=CARTESIAN_POINT('Ctrl Pts',(53.0343112535921,20.6505686492285,12.2432105029038));
#25642=CARTESIAN_POINT('Ctrl Pts',(53.0603629422339,20.5328904330271,12.2516151296792));
#25643=CARTESIAN_POINT('Ctrl Pts',(53.0693154290845,20.4971675755938,12.2541793133802));
#25644=CARTESIAN_POINT('Ctrl Pts',(53.0800301865641,20.4589345690755,12.2569268177156));
#25645=CARTESIAN_POINT('Ctrl Pts',(53.0808147055468,20.4561583955903,12.2571263364176));
#25646=CARTESIAN_POINT('Ctrl Pts',(53.1008998768015,20.3856678098868,12.2621926687645));
#25647=CARTESIAN_POINT('Ctrl Pts',(53.1237686827481,20.3190127898694,12.2669919913282));
#25648=CARTESIAN_POINT('Ctrl Pts',(53.1539423563909,20.2442201089912,12.2722863230984));
#25649=CARTESIAN_POINT('Ctrl Pts',(53.1578399335318,20.2347690758087,12.2729535925007));
#25650=CARTESIAN_POINT('Ctrl Pts',(53.163848401717,20.2205114372457,12.2739571302829));
#25651=CARTESIAN_POINT('Ctrl Pts',(53.1659058199693,20.2156826843363,12.2742964665259));
#25652=CARTESIAN_POINT('Ctrl Pts',(53.1696361114668,20.2070226522457,12.274903996813));
#25653=CARTESIAN_POINT('Ctrl Pts',(53.1713019827506,20.2031884782498,12.2751726020627));
#25654=CARTESIAN_POINT('Ctrl Pts',(53.1749742992301,20.1948084431792,12.275758844669));
#25655=CARTESIAN_POINT('Ctrl Pts',(53.176985676469,20.1902648401207,12.2760761777264));
#25656=CARTESIAN_POINT('Ctrl Pts',(53.1827729190191,20.1773226082435,12.27697871971));
#25657=CARTESIAN_POINT('Ctrl Pts',(53.1865900496132,20.1689424121296,12.2775614760752));
#25658=CARTESIAN_POINT('Ctrl Pts',(53.2126470393962,20.1127708617911,12.2814585011983));
#25659=CARTESIAN_POINT('Ctrl Pts',(53.2367178338558,20.0658462498892,12.2846695391328));
#25660=CARTESIAN_POINT('Ctrl Pts',(53.3473309939483,19.869762140052,12.2981261516832));
#25661=CARTESIAN_POINT('Ctrl Pts',(53.4511517904791,19.7312095847649,12.3077963019268));
#25662=CARTESIAN_POINT('Ctrl Pts',(53.6159919661092,19.562080601039,12.3218839798161));
#25663=CARTESIAN_POINT('Ctrl Pts',(53.6626392790816,19.5185967795252,12.3257533886522));
#25664=CARTESIAN_POINT('Ctrl Pts',(53.7228073859863,19.4676702435436,12.3306580584848));
#25665=CARTESIAN_POINT('Ctrl Pts',(53.7344402308553,19.4580486691212,12.3316024761219));
#25666=CARTESIAN_POINT('Ctrl Pts',(53.7529494332447,19.4430901821095,12.3330997518733));
#25667=CARTESIAN_POINT('Ctrl Pts',(53.7597535867706,19.4376645278051,12.333649034611));
#25668=CARTESIAN_POINT('Ctrl Pts',(53.7723944876453,19.4277192489391,12.3346675434637));
#25669=CARTESIAN_POINT('Ctrl Pts',(53.7782212625553,19.4231871485653,12.3351362618696));
#25670=CARTESIAN_POINT('Ctrl Pts',(53.7912142997399,19.4131963433191,12.3361798471587));
#25671=CARTESIAN_POINT('Ctrl Pts',(53.7983926208869,19.4077536572273,12.3367553311327));
#25672=CARTESIAN_POINT('Ctrl Pts',(53.8191804163547,19.3922127434899,12.3384189711184));
#25673=CARTESIAN_POINT('Ctrl Pts',(53.8328817630903,19.3822392812993,12.3395119333565));
#25674=CARTESIAN_POINT('Ctrl Pts',(53.9500018678375,19.2992476787905,12.3488271845166));
#25675=CARTESIAN_POINT('Ctrl Pts',(54.0600094596274,19.2360664316792,12.3574255488432));
#25676=CARTESIAN_POINT('Ctrl Pts',(54.3006826264698,19.1267773209753,12.3757719254443));
#25677=CARTESIAN_POINT('Ctrl Pts',(54.4316916344296,19.0829614577896,12.3855058729236));
#25678=CARTESIAN_POINT('Ctrl Pts',(54.5901272621266,19.0476593254977,12.3963733902617));
#25679=CARTESIAN_POINT('Ctrl Pts',(54.614177589219,19.0427644572554,12.3979984186275));
#25680=CARTESIAN_POINT('Ctrl Pts',(54.6457664046384,19.0369402561056,12.4000953967686));
#25681=CARTESIAN_POINT('Ctrl Pts',(54.653227332864,19.035608562437,12.4005879623897));
#25682=CARTESIAN_POINT('Ctrl Pts',(54.665240349757,19.033534946345,12.4013764904729));
#25683=CARTESIAN_POINT('Ctrl Pts',(54.6697876495554,19.0327662479148,12.4016739233768));
#25684=CARTESIAN_POINT('Ctrl Pts',(54.6785341099816,19.0313188839393,12.4022439481143));
#25685=CARTESIAN_POINT('Ctrl Pts',(54.6827327970208,19.0306378755094,12.402516663384));
#25686=CARTESIAN_POINT('Ctrl Pts',(54.6927242454305,19.0290500892357,12.4031634989931));
#25687=CARTESIAN_POINT('Ctrl Pts',(54.6985189418029,19.0281554032504,12.4035369403434));
#25688=CARTESIAN_POINT('Ctrl Pts',(54.7180413803295,19.025229260629,12.4047896036267));
#25689=CARTESIAN_POINT('Ctrl Pts',(54.7317867191033,19.0233154531785,12.4056624873672));
#25690=CARTESIAN_POINT('Ctrl Pts',(54.8097936684789,19.0132829965273,12.4105705016985));
#25691=CARTESIAN_POINT('Ctrl Pts',(54.8744071625643,19.0081538540431,12.4144607834168));
#25692=CARTESIAN_POINT('Ctrl Pts',(55.1091116861522,19.0009922317899,12.4283215340788));
#25693=CARTESIAN_POINT('Ctrl Pts',(55.2790223518195,19.0175554539421,12.4379057308322));
#25694=CARTESIAN_POINT('Ctrl Pts',(55.4926448469044,19.0664178955266,12.4511093268226));
#25695=CARTESIAN_POINT('Ctrl Pts',(55.5400880121583,19.0791296147358,12.4541127327729));
#25696=CARTESIAN_POINT('Ctrl Pts',(55.6004422960877,19.0977134522889,12.4580484706044));
#25697=CARTESIAN_POINT('Ctrl Pts',(55.6138290485315,19.1019907946169,12.4589287874954));
#25698=CARTESIAN_POINT('Ctrl Pts',(55.6351286874522,19.1090453692252,12.4603417288893));
#25699=CARTESIAN_POINT('Ctrl Pts',(55.6430713518842,19.1117317197546,12.4608713611555));
#25700=CARTESIAN_POINT('Ctrl Pts',(55.6573656860306,19.1166669662475,12.4618295953628));
#25701=CARTESIAN_POINT('Ctrl Pts',(55.6637233780522,19.1188981322652,12.4622576049433));
#25702=CARTESIAN_POINT('Ctrl Pts',(55.6786591233846,19.1242248212353,12.463267443325));
#25703=CARTESIAN_POINT('Ctrl Pts',(55.6872274373432,19.1273470231185,12.4638501513042));
#25704=CARTESIAN_POINT('Ctrl Pts',(55.7121565979709,19.1366250750634,12.4655555780946));
#25705=CARTESIAN_POINT('Ctrl Pts',(55.7284579654797,19.1429372409208,12.4666834844914));
#25706=CARTESIAN_POINT('Ctrl Pts',(55.8781738369404,19.2031843337904,12.4771631661521));
#25707=CARTESIAN_POINT('Ctrl Pts',(56.0054424064446,19.2711835986645,12.487009264057));
#25708=CARTESIAN_POINT('Ctrl Pts',(56.2330030922954,19.426450392841,12.5061977560865));
#25709=CARTESIAN_POINT('Ctrl Pts',(56.3341352727608,19.5112274444425,12.5154534160502));
#25710=CARTESIAN_POINT('Ctrl Pts',(56.4368506154463,19.6162656768939,12.525176922097));
#25711=CARTESIAN_POINT('Ctrl Pts',(56.4473932059313,19.6272970789773,12.5261788955187));
#25712=CARTESIAN_POINT('Ctrl Pts',(56.4620866817271,19.6430293364719,12.5275796435325));
#25713=CARTESIAN_POINT('Ctrl Pts',(56.4663432664172,19.6476301267194,12.5279859460844));
#25714=CARTESIAN_POINT('Ctrl Pts',(56.4734732139227,19.6554098727559,12.5286672767197));
#25715=CARTESIAN_POINT('Ctrl Pts',(56.4763581225468,19.6585781358597,12.5289431668842));
#25716=CARTESIAN_POINT('Ctrl Pts',(56.4822271517121,19.6650654871403,12.5295048235805));
#25717=CARTESIAN_POINT('Ctrl Pts',(56.4852103749431,19.6683853312566,12.5297905237785));
#25718=CARTESIAN_POINT('Ctrl Pts',(56.4927821118931,19.6768685467284,12.5305162849049));
#25719=CARTESIAN_POINT('Ctrl Pts',(56.4973550399905,19.6820458415373,12.5309551947706));
#25720=CARTESIAN_POINT('Ctrl Pts',(56.5158057323754,19.7031550006155,12.5327290007357));
#25721=CARTESIAN_POINT('Ctrl Pts',(56.529457440082,19.7192837962775,12.5340481871007));
#25722=CARTESIAN_POINT('Ctrl Pts',(56.5647197993602,19.7623126913729,12.5374830758078));
#25723=CARTESIAN_POINT('Ctrl Pts',(56.5858939361749,19.7895626313357,12.5395739828232));
#25724=CARTESIAN_POINT('Ctrl Pts',(56.7012832206323,19.9462917703661,12.5512191647472));
#25725=CARTESIAN_POINT('Ctrl Pts',(56.7803484695527,20.0861993479898,12.5602350253372));
#25726=CARTESIAN_POINT('Ctrl Pts',(56.8549736365081,20.2656495393253,12.5717442870465));
#25727=CARTESIAN_POINT('Ctrl Pts',(56.8672937415927,20.2975672900258,12.5737871581258));
#25728=CARTESIAN_POINT('Ctrl Pts',(56.8942489202137,20.3731296524752,12.5786322489278));
#25729=CARTESIAN_POINT('Ctrl Pts',(56.9082055420327,20.4169935575018,12.5814517602672));
#25730=CARTESIAN_POINT('Ctrl Pts',(56.9243405481291,20.4745196754187,12.5851769928329));
#25731=CARTESIAN_POINT('Ctrl Pts',(56.9279121800348,20.4877786339558,12.5860374369));
#25732=CARTESIAN_POINT('Ctrl Pts',(56.9334260126977,20.5091226884102,12.5874259467901));
#25733=CARTESIAN_POINT('Ctrl Pts',(56.9354550878136,20.5171850444797,12.587951202039));
#25734=CARTESIAN_POINT('Ctrl Pts',(56.9392187717076,20.5325447869017,12.5889534386144));
#25735=CARTESIAN_POINT('Ctrl Pts',(56.9409627410528,20.5398397495211,12.5894301090741));
#25736=CARTESIAN_POINT('Ctrl Pts',(56.9448470814285,20.5565028365895,12.5905205168217));
#25737=CARTESIAN_POINT('Ctrl Pts',(56.946960969867,20.5658768831708,12.5911350917431));
#25738=CARTESIAN_POINT('Ctrl Pts',(56.9532507468649,20.5947392086233,12.5930310729589));
#25739=CARTESIAN_POINT('Ctrl Pts',(56.9572022541346,20.6142746083907,12.5943195872321));
#25740=CARTESIAN_POINT('Ctrl Pts',(56.988165915428,20.7801027148525,12.6053048193061));
#25741=CARTESIAN_POINT('Ctrl Pts',(56.9990217609752,20.92890758912,12.6155277282375));
#25742=CARTESIAN_POINT('Ctrl Pts',(56.9884937645123,21.1996626274797,12.6344190490827));
#25743=CARTESIAN_POINT('Ctrl Pts',(56.9725237052528,21.3211358229798,12.6429852309299));
#25744=CARTESIAN_POINT('Ctrl Pts',(56.942065947612,21.455690119339,12.6521215862779));
#25745=CARTESIAN_POINT('Ctrl Pts',(56.9384222750827,21.4709487763316,12.6531521526536));
#25746=CARTESIAN_POINT('Ctrl Pts',(56.9330538267193,21.4923115395515,12.6545857315329));
#25747=CARTESIAN_POINT('Ctrl Pts',(56.9314794833029,21.4984523620172,12.6549967401416));
#25748=CARTESIAN_POINT('Ctrl Pts',(56.9288867564663,21.5083686977236,12.6556585813069));
#25749=CARTESIAN_POINT('Ctrl Pts',(56.9278865149936,21.5121488436463,12.6559104384413));
#25750=CARTESIAN_POINT('Ctrl Pts',(56.9257480022462,21.5201357382218,12.6564416101157));
#25751=CARTESIAN_POINT('Ctrl Pts',(56.924607048358,21.5243417439176,12.6567207625699));
#25752=CARTESIAN_POINT('Ctrl Pts',(56.9217522522921,21.5347307823527,12.6574089495316));
#25753=CARTESIAN_POINT('Ctrl Pts',(56.9200223274211,21.5409094135891,12.6578170625234));
#25754=CARTESIAN_POINT('Ctrl Pts',(56.9134867695878,21.5638254828419,12.6593267419904));
#25755=CARTESIAN_POINT('Ctrl Pts',(56.9084916810993,21.5805086945546,12.6604179054473));
#25756=CARTESIAN_POINT('Ctrl Pts',(56.8723459490667,21.6957197390413,12.6679120361855));
#25757=CARTESIAN_POINT('Ctrl Pts',(56.8337947479746,21.7917749090959,12.6739546209566));
#25758=CARTESIAN_POINT('Ctrl Pts',(56.7168825881373,22.0281278918137,12.6892776771497));
#25759=CARTESIAN_POINT('Ctrl Pts',(56.6287410221259,22.1627249469042,12.6984950768967));
#25760=CARTESIAN_POINT('Ctrl Pts',(56.5105750059554,22.3029671262384,12.7097978950417));
#25761=CARTESIAN_POINT('Ctrl Pts',(56.4953996876077,22.3203559695638,12.7112318489837));
#25762=CARTESIAN_POINT('Ctrl Pts',(56.473608954287,22.3444675493928,12.7132687675036));
#25763=CARTESIAN_POINT('Ctrl Pts',(56.4672419791969,22.3514130793825,12.7138613542192));
#25764=CARTESIAN_POINT('Ctrl Pts',(56.4560626666892,22.363436103517,12.7148975315937));
#25765=CARTESIAN_POINT('Ctrl Pts',(56.4512723458348,22.3685339140433,12.7153401811585));
#25766=CARTESIAN_POINT('Ctrl Pts',(56.4411885518834,22.3791525003565,12.7162692270472));
#25767=CARTESIAN_POINT('Ctrl Pts',(56.4358899519485,22.3846682290482,12.7167558406816));
#25768=CARTESIAN_POINT('Ctrl Pts',(56.4231963690036,22.3977307667788,12.7179179899864));
#25769=CARTESIAN_POINT('Ctrl Pts',(56.4157729474788,22.4052494992777,12.7185947625495));
#25770=CARTESIAN_POINT('Ctrl Pts',(56.3903945800356,22.4305484909044,12.7208990529384));
#25771=CARTESIAN_POINT('Ctrl Pts',(56.3721622572503,22.4480458264579,12.7225388378732));
#25772=CARTESIAN_POINT('Ctrl Pts',(56.3276634364322,22.4891556374522,12.7265058763382));
#25773=CARTESIAN_POINT('Ctrl Pts',(56.3010933190893,22.5124254143664,12.728846565667));
#25774=CARTESIAN_POINT('Ctrl Pts',(56.194082888121,22.6012364256864,12.7381666435083));
#25775=CARTESIAN_POINT('Ctrl Pts',(56.1092057846088,22.6611592559875,12.7453408391161));
#25776=CARTESIAN_POINT('Ctrl Pts',(55.913495595774,22.7776196881566,12.7612165740381));
#25777=CARTESIAN_POINT('Ctrl Pts',(55.8012362967081,22.8309647146541,12.7699119264545));
#25778=CARTESIAN_POINT('Ctrl Pts',(55.6700406827082,22.8789140543262,12.779162060202));
#25779=CARTESIAN_POINT('Ctrl Pts',(55.6552767042515,22.8841138546774,12.7801903058312));
#25780=CARTESIAN_POINT('Ctrl Pts',(55.6344543631186,22.8911730054278,12.7816212204077));
#25781=CARTESIAN_POINT('Ctrl Pts',(55.6284464640087,22.8931779419426,12.7820318470124));
#25782=CARTESIAN_POINT('Ctrl Pts',(55.6187150681843,22.8963740422706,12.7826932381613));
#25783=CARTESIAN_POINT('Ctrl Pts',(55.614997500106,22.8975829150014,12.7829450246593));
#25784=CARTESIAN_POINT('Ctrl Pts',(55.6071268653632,22.9001167160696,12.7834762047339));
#25785=CARTESIAN_POINT('Ctrl Pts',(55.6029729634754,22.9014389738646,12.7837554354888));
#25786=CARTESIAN_POINT('Ctrl Pts',(55.5926887186397,22.9046755340704,12.7844440868829));
#25787=CARTESIAN_POINT('Ctrl Pts',(55.586553338804,22.906573888092,12.7848525832263));
#25788=CARTESIAN_POINT('Ctrl Pts',(55.5637079491971,22.913521786356,12.7863653246141));
#25789=CARTESIAN_POINT('Ctrl Pts',(55.5469404736724,22.9183817258926,12.7874591117626));
#25790=CARTESIAN_POINT('Ctrl Pts',(55.504489668697,22.9300839508081,12.7901918895449));
#25791=CARTESIAN_POINT('Ctrl Pts',(55.4787287766821,22.9366343950759,12.7918169379439));
#25792=CARTESIAN_POINT('Ctrl Pts',(55.3578541463681,22.9648107347426,12.7993198089275));
#25793=CARTESIAN_POINT('Ctrl Pts',(55.2614624560589,22.9799346311093,12.804957572981));
#25794=CARTESIAN_POINT('Ctrl Pts',(55.1644480621455,22.9879598580848,12.8106050954514));
#25795=CARTESIAN_POINT('Origin',(55.,21.,6.22095488139522));
#25796=CARTESIAN_POINT('',(55.164448547645,22.9879598179233,13.7675726541794));
#25797=CARTESIAN_POINT('',(55.1644483515698,22.987959834143,13.6085666014869));
#25798=CARTESIAN_POINT('',(55.1644483516311,22.987959834138,6.22095488139522));
#25799=CARTESIAN_POINT('',(53.0046129860205,21.0017710049344,13.1790451186048));
#25800=CARTESIAN_POINT('Ctrl Pts',(55.164448547645,22.9879598179233,13.7675726541794));
#25801=CARTESIAN_POINT('Ctrl Pts',(55.2645411203093,22.9796799331608,13.7616912993627));
#25802=CARTESIAN_POINT('Ctrl Pts',(55.3639264204527,22.9638475460295,13.7559274711235));
#25803=CARTESIAN_POINT('Ctrl Pts',(55.5560482604016,22.9181326220663,13.7443471394518));
#25804=CARTESIAN_POINT('Ctrl Pts',(55.6485702217839,22.8888556037384,13.738558262633));
#25805=CARTESIAN_POINT('Ctrl Pts',(55.7527207671479,22.8473414357672,13.7315963732279));
#25806=CARTESIAN_POINT('Ctrl Pts',(55.7667853435036,22.8415480310159,13.7306467045588));
#25807=CARTESIAN_POINT('Ctrl Pts',(55.7895674137876,22.831857529926,13.7290921738092));
#25808=CARTESIAN_POINT('Ctrl Pts',(55.7983257700313,22.8280576223582,13.728490600419));
#25809=CARTESIAN_POINT('Ctrl Pts',(55.8139107996568,22.8211625275556,13.7274129097854));
#25810=CARTESIAN_POINT('Ctrl Pts',(55.8207479853913,22.8180914398187,13.726937622937));
#25811=CARTESIAN_POINT('Ctrl Pts',(55.8351675299038,22.8115166370394,13.7259298682735));
#25812=CARTESIAN_POINT('Ctrl Pts',(55.8427454973394,22.8080036926101,13.7253970900889));
#25813=CARTESIAN_POINT('Ctrl Pts',(55.862875685628,22.798517819093,13.7239732284081));
#25814=CARTESIAN_POINT('Ctrl Pts',(55.8753877317645,22.7924611843187,13.7230792645785));
#25815=CARTESIAN_POINT('Ctrl Pts',(55.9359533689449,22.7623581360577,13.7187073703467));
#25816=CARTESIAN_POINT('Ctrl Pts',(55.9830813035911,22.7365094724083,13.71516695115));
#25817=CARTESIAN_POINT('Ctrl Pts',(56.1950437690573,22.6088569416073,13.698581020333));
#25818=CARTESIAN_POINT('Ctrl Pts',(56.3455060137317,22.4853090060613,13.6847601643102));
#25819=CARTESIAN_POINT('Ctrl Pts',(56.5054234895833,22.3094530632374,13.6685684700548));
#25820=CARTESIAN_POINT('Ctrl Pts',(56.5339692678035,22.2758942584669,13.6656118533761));
#25821=CARTESIAN_POINT('Ctrl Pts',(56.5665649913327,22.2348971736623,13.6621806787774));
#25822=CARTESIAN_POINT('Ctrl Pts',(56.5717064772905,22.2283467167808,13.6616377456301));
#25823=CARTESIAN_POINT('Ctrl Pts',(56.5800345638026,22.2175985011034,13.6607557500721));
#25824=CARTESIAN_POINT('Ctrl Pts',(56.583245753735,22.213420049912,13.6604150319014));
#25825=CARTESIAN_POINT('Ctrl Pts',(56.5889760054388,22.2059022813359,13.6598059648329));
#25826=CARTESIAN_POINT('Ctrl Pts',(56.5915011470311,22.2025677353074,13.6595371961136));
#25827=CARTESIAN_POINT('Ctrl Pts',(56.5969945682994,22.1952658533723,13.6589516814145));
#25828=CARTESIAN_POINT('Ctrl Pts',(56.5999585567207,22.1912953997557,13.6586352329643));
#25829=CARTESIAN_POINT('Ctrl Pts',(56.6083468890952,22.1799709108016,13.6577380046858));
#25830=CARTESIAN_POINT('Ctrl Pts',(56.6137356205523,22.1725904743565,13.6571596314389));
#25831=CARTESIAN_POINT('Ctrl Pts',(56.6488984283103,22.1237297750284,13.6533704960579));
#25832=CARTESIAN_POINT('Ctrl Pts',(56.6771239571451,22.0811525585331,13.6502565086701));
#25833=CARTESIAN_POINT('Ctrl Pts',(56.7853332757802,21.903467222576,13.6378049017059));
#25834=CARTESIAN_POINT('Ctrl Pts',(56.8508732117771,21.7602254709168,13.6289568401826));
#25835=CARTESIAN_POINT('Ctrl Pts',(56.9231994099082,21.5353573016456,13.6149925111427));
#25836=CARTESIAN_POINT('Ctrl Pts',(56.9429392385478,21.4585720594319,13.61022030477));
#25837=CARTESIAN_POINT('Ctrl Pts',(56.9608513376461,21.3664740892523,13.6043896997356));
#25838=CARTESIAN_POINT('Ctrl Pts',(56.9634840924494,21.3520957643995,13.603476532278));
#25839=CARTESIAN_POINT('Ctrl Pts',(56.9675443121326,21.3284580456637,13.6019699787483));
#25840=CARTESIAN_POINT('Ctrl Pts',(56.9690650175664,21.319215068157,13.6013795478635));
#25841=CARTESIAN_POINT('Ctrl Pts',(56.9716823816857,21.3025756984959,13.6003141133066));
#25842=CARTESIAN_POINT('Ctrl Pts',(56.9728026682736,21.2951831586224,13.5998398665341));
#25843=CARTESIAN_POINT('Ctrl Pts',(56.9751022692204,21.279410459865,13.5988260305627));
#25844=CARTESIAN_POINT('Ctrl Pts',(56.976269865866,21.2710287670917,13.598286081175));
#25845=CARTESIAN_POINT('Ctrl Pts',(56.9792801976098,21.2483643520073,13.5968226960539));
#25846=CARTESIAN_POINT('Ctrl Pts',(56.9810216255651,21.2340689065069,13.5958960927018));
#25847=CARTESIAN_POINT('Ctrl Pts',(56.9892474423376,21.1598567864132,13.591066319055));
#25848=CARTESIAN_POINT('Ctrl Pts',(56.9931682239661,21.0996932028106,13.5870836882978));
#25849=CARTESIAN_POINT('Ctrl Pts',(56.9974820998487,20.8816054562162,13.572396861648));
#25850=CARTESIAN_POINT('Ctrl Pts',(56.9818532004351,20.7239594403078,13.5612518135231));
#25851=CARTESIAN_POINT('Ctrl Pts',(56.9326339654805,20.5010915443035,13.5454757457249));
#25852=CARTESIAN_POINT('Ctrl Pts',(56.9138219791016,20.4331919712266,13.5406772282269));
#25853=CARTESIAN_POINT('Ctrl Pts',(56.8882089224664,20.3567277663116,13.535383527226));
#25854=CARTESIAN_POINT('Ctrl Pts',(56.8848868385247,20.3470576456336,13.5347161465374));
#25855=CARTESIAN_POINT('Ctrl Pts',(56.8797466075484,20.3324613748682,13.53371241615));
#25856=CARTESIAN_POINT('Ctrl Pts',(56.8779831845906,20.3275163313815,13.533372997786));
#25857=CARTESIAN_POINT('Ctrl Pts',(56.8747801286319,20.318645086479,13.5327653058439));
#25858=CARTESIAN_POINT('Ctrl Pts',(56.8733476612475,20.3147164163798,13.5324966209533));
#25859=CARTESIAN_POINT('Ctrl Pts',(56.8701853895074,20.3061276206417,13.5319101815815));
#25860=CARTESIAN_POINT('Ctrl Pts',(56.8684505205586,20.3014694541491,13.5315927317315));
#25861=CARTESIAN_POINT('Ctrl Pts',(56.8634505970886,20.2881964392939,13.530689792387));
#25862=CARTESIAN_POINT('Ctrl Pts',(56.8601431977251,20.2795975232187,13.5301067580012));
#25863=CARTESIAN_POINT('Ctrl Pts',(56.8374909093142,20.2219000201297,13.5262057465217));
#25864=CARTESIAN_POINT('Ctrl Pts',(56.8162619274268,20.1735581620475,13.5229912321826));
#25865=CARTESIAN_POINT('Ctrl Pts',(56.7173495965792,19.9705993389065,13.5094966225792));
#25866=CARTESIAN_POINT('Ctrl Pts',(56.6216520662475,19.8256033890593,13.4997952314163));
#25867=CARTESIAN_POINT('Ctrl Pts',(56.4671157630676,19.6470079556063,13.485702268875));
#25868=CARTESIAN_POINT('Ctrl Pts',(56.4235500937784,19.6012433881567,13.4818672973344));
#25869=CARTESIAN_POINT('Ctrl Pts',(56.3670011222939,19.5472225626512,13.4770010929343));
#25870=CARTESIAN_POINT('Ctrl Pts',(56.3559946118949,19.5369439710868,13.4760589336283));
#25871=CARTESIAN_POINT('Ctrl Pts',(56.3384508103132,19.5209284644668,13.4745643572861));
#25872=CARTESIAN_POINT('Ctrl Pts',(56.3319904284758,19.5151078579814,13.4740154925577));
#25873=CARTESIAN_POINT('Ctrl Pts',(56.3199738578989,19.5044228177999,13.4729972276797));
#25874=CARTESIAN_POINT('Ctrl Pts',(56.3144282954451,19.4995466194561,13.4725283315439));
#25875=CARTESIAN_POINT('Ctrl Pts',(56.3020475114025,19.4887815384675,13.4714836863161));
#25876=CARTESIAN_POINT('Ctrl Pts',(56.2951991875691,19.4829080382095,13.4709073152875));
#25877=CARTESIAN_POINT('Ctrl Pts',(56.2753292331169,19.466099073045,13.469239059142));
#25878=CARTESIAN_POINT('Ctrl Pts',(56.2622075710119,19.4552836103294,13.4681423279872));
#25879=CARTESIAN_POINT('Ctrl Pts',(56.1472786880102,19.3629961990947,13.4585763892694));
#25880=CARTESIAN_POINT('Ctrl Pts',(56.0378671951796,19.2915358036076,13.4497066591063));
#25881=CARTESIAN_POINT('Ctrl Pts',(55.7913750942179,19.1630048509287,13.4303939641486));
#25882=CARTESIAN_POINT('Ctrl Pts',(55.653281178563,19.109482864558,13.4199547862178));
#25883=CARTESIAN_POINT('Ctrl Pts',(55.4969848235204,19.0681019115907,13.4092725816642));
#25884=CARTESIAN_POINT('Ctrl Pts',(55.483393327991,19.0646563468419,13.4083530199176));
#25885=CARTESIAN_POINT('Ctrl Pts',(55.4644507615683,19.0600662471987,13.4070854601013));
#25886=CARTESIAN_POINT('Ctrl Pts',(55.4591299901158,19.0588000800896,13.4067309485673));
#25887=CARTESIAN_POINT('Ctrl Pts',(55.4499590378488,19.0566575141207,13.4061226243678));
#25888=CARTESIAN_POINT('Ctrl Pts',(55.4461113729665,19.0557706419407,13.4058682239236));
#25889=CARTESIAN_POINT('Ctrl Pts',(55.4380481568352,19.0539372977985,13.405336854783));
#25890=CARTESIAN_POINT('Ctrl Pts',(55.4338321316845,19.0529930892277,13.4050600240247));
#25891=CARTESIAN_POINT('Ctrl Pts',(55.4235340745671,19.0507218768237,13.4043862224153));
#25892=CARTESIAN_POINT('Ctrl Pts',(55.4174487679122,19.0494096169434,13.4039900870259));
#25893=CARTESIAN_POINT('Ctrl Pts',(55.3955882942872,19.044802523895,13.4025739727095));
#25894=CARTESIAN_POINT('Ctrl Pts',(55.3797789792539,19.0416702945803,13.4015627920337));
#25895=CARTESIAN_POINT('Ctrl Pts',(55.3404503183141,19.0343724768612,13.3990754211655));
#25896=CARTESIAN_POINT('Ctrl Pts',(55.3168903358608,19.030436952471,13.3976101813319));
#25897=CARTESIAN_POINT('Ctrl Pts',(55.217588755629,19.015677445536,13.3915171113919));
#25898=CARTESIAN_POINT('Ctrl Pts',(55.1413225463487,19.0087916625203,13.3870371664692));
#25899=CARTESIAN_POINT('Ctrl Pts',(54.8992270124374,19.000917611299,13.3729491147946));
#25900=CARTESIAN_POINT('Ctrl Pts',(54.7336042631521,19.0161872791028,13.3634474873401));
#25901=CARTESIAN_POINT('Ctrl Pts',(54.5492380183973,19.0567105431483,13.3518073002083));
#25902=CARTESIAN_POINT('Ctrl Pts',(54.5267839703626,19.0620560385604,13.350372478579));
#25903=CARTESIAN_POINT('Ctrl Pts',(54.4955409989107,19.0700692082408,13.3483498687426));
#25904=CARTESIAN_POINT('Ctrl Pts',(54.486669523148,19.0724099082579,13.347772577724));
#25905=CARTESIAN_POINT('Ctrl Pts',(54.4704496661712,19.0768093594841,13.3467115170287));
#25906=CARTESIAN_POINT('Ctrl Pts',(54.4630963124641,19.0788492449834,13.3462283646628));
#25907=CARTESIAN_POINT('Ctrl Pts',(54.4482171297583,19.0830689593022,13.3452463529093));
#25908=CARTESIAN_POINT('Ctrl Pts',(54.4406920828997,19.0852510342944,13.3447474278921));
#25909=CARTESIAN_POINT('Ctrl Pts',(54.4221425392805,19.0907486157959,13.343511825711));
#25910=CARTESIAN_POINT('Ctrl Pts',(54.4111336269255,19.09411530295,13.3427734905921));
#25911=CARTESIAN_POINT('Ctrl Pts',(54.3707823148277,19.1068383129956,13.3400483718986));
#25912=CARTESIAN_POINT('Ctrl Pts',(54.3416298428973,19.116778125334,13.3380426185486));
#25913=CARTESIAN_POINT('Ctrl Pts',(54.2693437578541,19.1433083184868,13.3329733310149));
#25914=CARTESIAN_POINT('Ctrl Pts',(54.2265363500068,19.1607294980157,13.329884019296));
#25915=CARTESIAN_POINT('Ctrl Pts',(54.0393943892088,19.24457884342,13.3159919039293));
#25916=CARTESIAN_POINT('Ctrl Pts',(53.9026983484603,19.3266242818743,13.3047395987014));
#25917=CARTESIAN_POINT('Ctrl Pts',(53.7684112136017,19.4308153483634,13.2930527205901));
#25918=CARTESIAN_POINT('Ctrl Pts',(53.7596758235183,19.4377108609447,13.2922896292018));
#25919=CARTESIAN_POINT('Ctrl Pts',(53.7129732974139,19.475215359519,13.2881961525032));
#25920=CARTESIAN_POINT('Ctrl Pts',(53.6760771125373,19.5071386553002,13.2849126123578));
#25921=CARTESIAN_POINT('Ctrl Pts',(53.6341152775534,19.5462256329398,13.2811539025904));
#25922=CARTESIAN_POINT('Ctrl Pts',(53.627882871414,19.5521065035471,13.2805949866178));
#25923=CARTESIAN_POINT('Ctrl Pts',(53.6178261271116,19.5617192575264,13.2796923293008));
#25924=CARTESIAN_POINT('Ctrl Pts',(53.6139786255047,19.5654265929834,13.2793468038399));
#25925=CARTESIAN_POINT('Ctrl Pts',(53.6071421037555,19.5720672352561,13.2787325900828));
#25926=CARTESIAN_POINT('Ctrl Pts',(53.6041473864516,19.5749945326054,13.2784634506081));
#25927=CARTESIAN_POINT('Ctrl Pts',(53.5976693035084,19.5813667914921,13.277881081201));
#25928=CARTESIAN_POINT('Ctrl Pts',(53.5941894079656,19.5848151558281,13.277568123768));
#25929=CARTESIAN_POINT('Ctrl Pts',(53.5848808793864,19.594107557082,13.27673053662));
#25930=CARTESIAN_POINT('Ctrl Pts',(53.5790756796207,19.5999750830932,13.2762077107941));
#25931=CARTESIAN_POINT('Ctrl Pts',(53.5459595599289,19.6338649133974,13.2732212839489));
#25932=CARTESIAN_POINT('Ctrl Pts',(53.5194394031791,19.6626520747054,13.2708141453961));
#25933=CARTESIAN_POINT('Ctrl Pts',(53.4352379247601,19.7596287730261,13.2630453911727));
#25934=CARTESIAN_POINT('Ctrl Pts',(53.3812832193677,19.8309150428113,13.2578574645044));
#25935=CARTESIAN_POINT('Ctrl Pts',(53.2514589230141,20.0287462853698,13.2441260073103));
#25936=CARTESIAN_POINT('Ctrl Pts',(53.1845356700698,20.1604687335485,13.235602286656));
#25937=CARTESIAN_POINT('Ctrl Pts',(53.1243437241021,20.3206555887834,13.2250636790948));
#25938=CARTESIAN_POINT('Ctrl Pts',(53.1163631891268,20.3431076315202,13.2235840197377));
#25939=CARTESIAN_POINT('Ctrl Pts',(53.105749718957,20.3747523148721,13.221492630919));
#25940=CARTESIAN_POINT('Ctrl Pts',(53.1027775750157,20.3838296826005,13.2208920413586));
#25941=CARTESIAN_POINT('Ctrl Pts',(53.0977316217409,20.3996234632718,13.2198457581887));
#25942=CARTESIAN_POINT('Ctrl Pts',(53.0956278912612,20.4063301943173,13.2194010521076));
#25943=CARTESIAN_POINT('Ctrl Pts',(53.0913160256364,20.420335278548,13.2184714948271));
#25944=CARTESIAN_POINT('Ctrl Pts',(53.0891142070655,20.4276354422244,13.217986445817));
#25945=CARTESIAN_POINT('Ctrl Pts',(53.0840013824067,20.4449454713224,13.2168349997103));
#25946=CARTESIAN_POINT('Ctrl Pts',(53.0811269049094,20.4549658079226,13.2161674268173));
#25947=CARTESIAN_POINT('Ctrl Pts',(53.0752349704908,20.4761293919263,13.2147551392495));
#25948=CARTESIAN_POINT('Ctrl Pts',(53.0722354535064,20.4872771930133,13.2140098703492));
#25949=CARTESIAN_POINT('Ctrl Pts',(53.0599119346415,20.5347153789783,13.2108323710528));
#25950=CARTESIAN_POINT('Ctrl Pts',(53.051515171606,20.5712366130093,13.2083708237553));
#25951=CARTESIAN_POINT('Ctrl Pts',(53.0181619612568,20.7376369355591,13.1970814761549));
#25952=CARTESIAN_POINT('Ctrl Pts',(53.0051351486799,20.8695447645175,13.1878996406867));
#25953=CARTESIAN_POINT('Ctrl Pts',(53.0052507628146,21.0017444908055,13.1786788122144));
#25954=CARTESIAN_POINT('Ctrl Pts',(55.1641804122445,22.9848227319589,12.9685061347694));
#25955=CARTESIAN_POINT('Ctrl Pts',(54.8621371071006,23.010541002547,12.9877832838503));
#25956=CARTESIAN_POINT('Ctrl Pts',(53.8801469710629,22.883843418079,13.0494048645008));
#25957=CARTESIAN_POINT('Ctrl Pts',(53.0767306724305,21.9309683111089,13.1195845257793));
#25958=CARTESIAN_POINT('Ctrl Pts',(53.0033791829374,21.1357025185976,13.1704870379768));
#25959=CARTESIAN_POINT('Ctrl Pts',(53.0046129860205,21.0017710049344,13.1790451186048));
#25960=CARTESIAN_POINT('',(53.005250339812,20.9988356633973,13.0222599084274));
#25961=CARTESIAN_POINT('Ctrl Pts',(55.1644480621455,22.9879598580848,12.8106050954514));
#25962=CARTESIAN_POINT('Ctrl Pts',(55.090601741016,22.9940685751985,12.8149039292751));
#25963=CARTESIAN_POINT('Ctrl Pts',(55.0163945770778,22.9960643557173,12.819207547069));
#25964=CARTESIAN_POINT('Ctrl Pts',(54.8653052417656,22.9916821606349,12.8281542158983));
#25965=CARTESIAN_POINT('Ctrl Pts',(54.788643138605,22.9850105172829,12.8327915704553));
#25966=CARTESIAN_POINT('Ctrl Pts',(54.698187344796,22.9718386664432,12.8384728806987));
#25967=CARTESIAN_POINT('Ctrl Pts',(54.6838352499383,22.9695883932003,12.8393805159609));
#25968=CARTESIAN_POINT('Ctrl Pts',(54.6602999956822,22.9656344204189,12.8408796981102));
#25969=CARTESIAN_POINT('Ctrl Pts',(54.6511017927926,22.9640226077863,12.8414683383457));
#25970=CARTESIAN_POINT('Ctrl Pts',(54.6345643437187,22.9610048905017,12.8425317003339));
#25971=CARTESIAN_POINT('Ctrl Pts',(54.6272209950825,22.9596222111577,12.8430056762876));
#25972=CARTESIAN_POINT('Ctrl Pts',(54.6115636737461,22.9565829009106,12.844020193514));
#25973=CARTESIAN_POINT('Ctrl Pts',(54.6032521684792,22.9549144692834,12.8445611024148));
#25974=CARTESIAN_POINT('Ctrl Pts',(54.5807780843412,22.9502538494799,12.8460302401133));
#25975=CARTESIAN_POINT('Ctrl Pts',(54.5666372474109,22.947160444935,12.8469616806759));
#25976=CARTESIAN_POINT('Ctrl Pts',(54.4927395575319,22.9301499766266,12.8518672143673));
#25977=CARTESIAN_POINT('Ctrl Pts',(54.4336203302244,22.9136365419279,12.8559238019402));
#25978=CARTESIAN_POINT('Ctrl Pts',(54.2481250303717,22.852474174311,12.8690840573301));
#25979=CARTESIAN_POINT('Ctrl Pts',(54.1254507255302,22.7978132357945,12.8784709237588));
#25980=CARTESIAN_POINT('Ctrl Pts',(53.9287558225416,22.6852458593228,12.8942390354748));
#25981=CARTESIAN_POINT('Ctrl Pts',(53.8516106033083,22.6336534551344,12.9006271974587));
#25982=CARTESIAN_POINT('Ctrl Pts',(53.7700805012206,22.5704885809255,12.9074001721675));
#25983=CARTESIAN_POINT('Ctrl Pts',(53.7618851245166,22.564035780502,12.9080811877692));
#25984=CARTESIAN_POINT('Ctrl Pts',(53.7496077151996,22.5542119264665,12.9091012338966));
#25985=CARTESIAN_POINT('Ctrl Pts',(53.7454880200296,22.5508885427193,12.9094434808455));
#25986=CARTESIAN_POINT('Ctrl Pts',(53.7381363042508,22.5449094062738,12.9100541008262));
#25987=CARTESIAN_POINT('Ctrl Pts',(53.7348993744885,22.5422598576809,12.9103229040934));
#25988=CARTESIAN_POINT('Ctrl Pts',(53.7316519924108,22.5395846500704,12.9105925215664));
#25989=CARTESIAN_POINT('Ctrl Pts',(53.7316332785217,22.5395692329136,12.910594075306));
#25990=CARTESIAN_POINT('Ctrl Pts',(53.7315960294229,22.5395385446623,12.9105971679473));
#25991=CARTESIAN_POINT('Ctrl Pts',(53.7315774941997,22.5395232735675,12.9105987068499));
#25992=CARTESIAN_POINT('Ctrl Pts',(53.7315405989734,22.5394928746224,12.9106017701045));
#25993=CARTESIAN_POINT('Ctrl Pts',(53.7315222390771,22.5394777468706,12.9106032944475));
#25994=CARTESIAN_POINT('Ctrl Pts',(53.7314856927541,22.5394476332009,12.9106063287281));
#25995=CARTESIAN_POINT('Ctrl Pts',(53.731467505689,22.5394326467672,12.9106078387187));
#25996=CARTESIAN_POINT('Ctrl Pts',(53.7314313011027,22.5394028125293,12.9106108446205));
#25997=CARTESIAN_POINT('Ctrl Pts',(53.7314132836658,22.5393879648047,12.9106123405248));
#25998=CARTESIAN_POINT('Ctrl Pts',(53.7313774155591,22.5393584057268,12.9106153184846));
#25999=CARTESIAN_POINT('Ctrl Pts',(53.7313595648514,22.5393436943519,12.9106168005433));
#26000=CARTESIAN_POINT('Ctrl Pts',(53.7313240278797,22.539314406088,12.9106197510049));
#26001=CARTESIAN_POINT('Ctrl Pts',(53.7313063413379,22.5392998289793,12.910621219431));
#26002=CARTESIAN_POINT('Ctrl Pts',(53.7312711294452,22.5392708065953,12.9106241428974));
#26003=CARTESIAN_POINT('Ctrl Pts',(53.7312536042865,22.5392563614875,12.9106255979219));
#26004=CARTESIAN_POINT('Ctrl Pts',(53.7274443994663,22.5361165160902,12.9109418564666));
#26005=CARTESIAN_POINT('Ctrl Pts',(53.7236642322047,22.5329770763307,12.911255641436));
#26006=CARTESIAN_POINT('Ctrl Pts',(53.7131144443147,22.5241493730663,12.9121313096567));
#26007=CARTESIAN_POINT('Ctrl Pts',(53.7063708873993,22.5184299360731,12.9126909887021));
#26008=CARTESIAN_POINT('Ctrl Pts',(53.6910832320592,22.5052881914442,12.9139602410067));
#26009=CARTESIAN_POINT('Ctrl Pts',(53.6825637472879,22.497837567254,12.91466790002));
#26010=CARTESIAN_POINT('Ctrl Pts',(53.6554994430845,22.4737591978603,12.9169187743747));
#26011=CARTESIAN_POINT('Ctrl Pts',(53.6372017879249,22.4568558853423,12.9184448473533));
#26012=CARTESIAN_POINT('Ctrl Pts',(53.5599272144776,22.3827395887461,12.9249333092508));
#26013=CARTESIAN_POINT('Ctrl Pts',(53.5041954484117,22.3222515925881,12.9297273084609));
#26014=CARTESIAN_POINT('Ctrl Pts',(53.3531267341063,22.1364728151092,12.943635928764));
#26015=CARTESIAN_POINT('Ctrl Pts',(53.2686933083185,22.0031614696136,12.9526911323066));
#26016=CARTESIAN_POINT('Ctrl Pts',(53.1907305006437,21.8403061687681,12.9638167272644));
#26017=CARTESIAN_POINT('Ctrl Pts',(53.1810379143992,21.8191138132981,12.9652643729206));
#26018=CARTESIAN_POINT('Ctrl Pts',(53.1679354725549,21.7890859497488,12.9673175922319));
#26019=CARTESIAN_POINT('Ctrl Pts',(53.164213629488,21.7803880225348,12.9679125623885));
#26020=CARTESIAN_POINT('Ctrl Pts',(53.1578440262373,21.7652045474106,12.96895171878));
#26021=CARTESIAN_POINT('Ctrl Pts',(53.1551682731058,21.7587308669457,12.9693949500095));
#26022=CARTESIAN_POINT('Ctrl Pts',(53.1496454496203,21.7451670784589,12.9703240432325));
#26023=CARTESIAN_POINT('Ctrl Pts',(53.1468049104564,21.7380744504134,12.970810116477));
#26024=CARTESIAN_POINT('Ctrl Pts',(53.140149954041,21.7211768540245,12.9719688056827));
#26025=CARTESIAN_POINT('Ctrl Pts',(53.1363722537278,21.7113577612832,12.9726426391501));
#26026=CARTESIAN_POINT('Ctrl Pts',(53.1238815080677,21.6781090073821,12.9749263716007));
#26027=CARTESIAN_POINT('Ctrl Pts',(53.1155315404224,21.6545463714167,12.9765482428566));
#26028=CARTESIAN_POINT('Ctrl Pts',(53.09661454438,21.5977992390173,12.9804641541126));
#26029=CARTESIAN_POINT('Ctrl Pts',(53.086469734562,21.5644836598201,12.9827711773309));
#26030=CARTESIAN_POINT('Ctrl Pts',(53.0293411308842,21.3575853021602,12.9971487807717));
#26031=CARTESIAN_POINT('Ctrl Pts',(53.0051454168276,21.1785904584044,13.0099083080189));
#26032=CARTESIAN_POINT('Ctrl Pts',(53.005250339812,20.9988356633973,13.0222599084274));
#26033=CARTESIAN_POINT('Ctrl Pts',(53.005250341493,20.9988327870284,13.022260106073));
#26034=CARTESIAN_POINT('Ctrl Pts',(53.0052832483541,20.9425954493867,13.0261243745321));
#26035=CARTESIAN_POINT('Ctrl Pts',(53.0076943804446,20.886377919827,13.0299328038307));
#26036=CARTESIAN_POINT('Ctrl Pts',(53.0131339377996,20.8226581779702,13.0341353458906));
#26037=CARTESIAN_POINT('Ctrl Pts',(53.0138334265883,20.814988600084,13.0346392835011));
#26038=CARTESIAN_POINT('Ctrl Pts',(53.0150629882058,20.8023186858579,13.0354684241452));
#26039=CARTESIAN_POINT('Ctrl Pts',(53.0155675734077,20.7973160382515,13.0357949417051));
#26040=CARTESIAN_POINT('Ctrl Pts',(53.0165080685925,20.7883319547842,13.0363797059881));
#26041=CARTESIAN_POINT('Ctrl Pts',(53.0169370624376,20.7843498442502,13.0366383258122));
#26042=CARTESIAN_POINT('Ctrl Pts',(53.0177928782713,20.7766243440384,13.0371389169336));
#26043=CARTESIAN_POINT('Ctrl Pts',(53.0182183117154,20.7728808731764,13.0373809574812));
#26044=CARTESIAN_POINT('Ctrl Pts',(53.0192248823116,20.7642420810879,13.0379382983765));
#26045=CARTESIAN_POINT('Ctrl Pts',(53.0198135602627,20.7593477024161,13.0382531712955));
#26046=CARTESIAN_POINT('Ctrl Pts',(53.0215009771349,20.7457437489847,13.039126003131));
#26047=CARTESIAN_POINT('Ctrl Pts',(53.0226390905044,20.7370390428146,13.0396818069246));
#26048=CARTESIAN_POINT('Ctrl Pts',(53.0290947901409,20.6900773215935,13.0426671880341));
#26049=CARTESIAN_POINT('Ctrl Pts',(53.0354656066091,20.6519705646401,13.0450424377492));
#26050=CARTESIAN_POINT('Ctrl Pts',(53.0495626594614,20.5804840546944,13.0494494397717));
#26051=CARTESIAN_POINT('Ctrl Pts',(53.0570495575807,20.547072597816,13.0514887575308));
#26052=CARTESIAN_POINT('Ctrl Pts',(53.1067224903387,20.3493941805232,13.0635180167238));
#26053=CARTESIAN_POINT('Ctrl Pts',(53.168855121851,20.1908656192521,13.0730791772929));
#26054=CARTESIAN_POINT('Ctrl Pts',(53.2661973624452,20.0130590307908,13.0852919090766));
#26055=CARTESIAN_POINT('Ctrl Pts',(53.282818787009,19.9844151609859,13.0873072953921));
#26056=CARTESIAN_POINT('Ctrl Pts',(53.3127276386172,19.9357078542538,13.0908283502564));
#26057=CARTESIAN_POINT('Ctrl Pts',(53.3256795619821,19.9154462732187,13.0923221873717));
#26058=CARTESIAN_POINT('Ctrl Pts',(53.3447307802516,19.8867979982509,13.0944789539835));
#26059=CARTESIAN_POINT('Ctrl Pts',(53.3505344182689,19.8782165205656,13.095130854771));
#26060=CARTESIAN_POINT('Ctrl Pts',(53.360717896488,19.8634087406332,13.096266138423));
#26061=CARTESIAN_POINT('Ctrl Pts',(53.365067057254,19.8571615267812,13.0967483525425));
#26062=CARTESIAN_POINT('Ctrl Pts',(53.3735078478127,19.8451838155702,13.0976792571661));
#26063=CARTESIAN_POINT('Ctrl Pts',(53.3775942783783,19.8394497799298,13.0981277437932));
#26064=CARTESIAN_POINT('Ctrl Pts',(53.3873269454354,19.8259448704966,13.0991908299515));
#26065=CARTESIAN_POINT('Ctrl Pts',(53.3929990821886,19.8181929629423,13.099806423757));
#26066=CARTESIAN_POINT('Ctrl Pts',(53.4131327453762,19.7910899641035,13.1019779293358));
#26067=CARTESIAN_POINT('Ctrl Pts',(53.4278891263184,19.7719615337871,13.1035452859635));
#26068=CARTESIAN_POINT('Ctrl Pts',(53.5223694695506,19.6539827676595,13.1134368684278));
#26069=CARTESIAN_POINT('Ctrl Pts',(53.6110207396983,19.5626827732422,13.122125740282));
#26070=CARTESIAN_POINT('Ctrl Pts',(53.7878355780693,19.4123152725683,13.1382779259167));
#26071=CARTESIAN_POINT('Ctrl Pts',(53.873205136614,19.3506303448776,13.1456630274263));
#26072=CARTESIAN_POINT('Ctrl Pts',(53.9874312587432,19.2811203656088,13.1547582378884));
#26073=CARTESIAN_POINT('Ctrl Pts',(54.0121373886634,19.2668034484959,13.1566814138544));
#26074=CARTESIAN_POINT('Ctrl Pts',(54.048052790003,19.247008489948,13.1594059694709));
#26075=CARTESIAN_POINT('Ctrl Pts',(54.0590183732447,19.2410979786583,13.160228498306));
#26076=CARTESIAN_POINT('Ctrl Pts',(54.0785703756557,19.2307945261308,13.1616776950129));
#26077=CARTESIAN_POINT('Ctrl Pts',(54.0871345399095,19.2263604587876,13.1623066232983));
#26078=CARTESIAN_POINT('Ctrl Pts',(54.1002229380178,19.2197039007833,13.1632585446028));
#26079=CARTESIAN_POINT('Ctrl Pts',(54.1047238499272,19.2174362343456,13.1635842429479));
#26080=CARTESIAN_POINT('Ctrl Pts',(54.1092450032001,19.215179813442,13.1639097148136));
#26081=CARTESIAN_POINT('Ctrl Pts',(54.1092566390746,19.2151740063422,13.1639105524537));
#26082=CARTESIAN_POINT('Ctrl Pts',(54.1092799495246,19.2151623731131,13.1639122304973));
#26083=CARTESIAN_POINT('Ctrl Pts',(54.1092916235084,19.2151565472799,13.1639130708582));
#26084=CARTESIAN_POINT('Ctrl Pts',(54.1093150101449,19.2151448766025,13.1639147543411));
#26085=CARTESIAN_POINT('Ctrl Pts',(54.1093267230482,19.2151390316343,13.163915597481));
#26086=CARTESIAN_POINT('Ctrl Pts',(54.1093501874704,19.2151273227164,13.1639172865178));
#26087=CARTESIAN_POINT('Ctrl Pts',(54.1093619392379,19.2151214586436,13.1639181324324));
#26088=CARTESIAN_POINT('Ctrl Pts',(54.1093854819581,19.2151097112353,13.1639198270595));
#26089=CARTESIAN_POINT('Ctrl Pts',(54.109397272649,19.2151038280313,13.1639206757529));
#26090=CARTESIAN_POINT('Ctrl Pts',(54.1094208933249,19.215092042309,13.1639223759452));
#26091=CARTESIAN_POINT('Ctrl Pts',(54.1094327234841,19.2150861397048,13.1639232274564));
#26092=CARTESIAN_POINT('Ctrl Pts',(54.109456423472,19.2150743149978,13.1639249333111));
#26093=CARTESIAN_POINT('Ctrl Pts',(54.1094682930403,19.2150683930258,13.1639257876356));
#26094=CARTESIAN_POINT('Ctrl Pts',(54.1094920720285,19.2150565294954,13.1639274991297));
#26095=CARTESIAN_POINT('Ctrl Pts',(54.1095039814809,19.2150505879217,13.1639283563015));
#26096=CARTESIAN_POINT('Ctrl Pts',(54.1095278401604,19.215038685229,13.1639300734843));
#26097=CARTESIAN_POINT('Ctrl Pts',(54.1095397897401,19.2150327239352,13.1639309335206));
#26098=CARTESIAN_POINT('Ctrl Pts',(54.1095637293307,19.2150207814778,13.1639326564794));
#26099=CARTESIAN_POINT('Ctrl Pts',(54.1095757189013,19.2150148005349,13.1639335193702));
#26100=CARTESIAN_POINT('Ctrl Pts',(54.109599738599,19.21500281872,13.1639352480467));
#26101=CARTESIAN_POINT('Ctrl Pts',(54.1096117688505,19.2149968177868,13.1639361138414));
#26102=CARTESIAN_POINT('Ctrl Pts',(54.1096358701259,19.2149847958867,13.163937848341));
#26103=CARTESIAN_POINT('Ctrl Pts',(54.1096479410245,19.2149787749833,13.1639387170368));
#26104=CARTESIAN_POINT('Ctrl Pts',(54.1096721235327,19.2149667131764,13.1639404573342));
#26105=CARTESIAN_POINT('Ctrl Pts',(54.1096842355944,19.2149606720484,13.1639413289681));
#26106=CARTESIAN_POINT('Ctrl Pts',(54.1097085013314,19.2149485693452,13.1639430752063));
#26107=CARTESIAN_POINT('Ctrl Pts',(54.1097206541766,19.214942508185,13.1639439497508));
#26108=CARTESIAN_POINT('Ctrl Pts',(54.1097450011706,19.2149303655754,13.1639457017875));
#26109=CARTESIAN_POINT('Ctrl Pts',(54.1097571959602,19.2149242838073,13.1639465793258));
#26110=CARTESIAN_POINT('Ctrl Pts',(54.1097816271545,19.2149120998295,13.1639483373723));
#26111=CARTESIAN_POINT('Ctrl Pts',(54.1097938633632,19.2149059977185,13.1639492178664));
#26112=CARTESIAN_POINT('Ctrl Pts',(54.1098183779925,19.2148937727608,13.1639509818671));
#26113=CARTESIAN_POINT('Ctrl Pts',(54.1098306561082,19.214887650067,13.1639518653518));
#26114=CARTESIAN_POINT('Ctrl Pts',(54.1098552540844,19.2148753841795,13.1639536352999));
#26115=CARTESIAN_POINT('Ctrl Pts',(54.1098675747664,19.2148692405772,13.1639545218223));
#26116=CARTESIAN_POINT('Ctrl Pts',(54.1098922585294,19.2148569325499,13.1639562978928));
#26117=CARTESIAN_POINT('Ctrl Pts',(54.1099046212595,19.214850768301,13.1639571874156));
#26118=CARTESIAN_POINT('Ctrl Pts',(54.1099293896163,19.2148384187353,13.1639589695221));
#26119=CARTESIAN_POINT('Ctrl Pts',(54.1099417951073,19.2148322334875,13.1639598620961));
#26120=CARTESIAN_POINT('Ctrl Pts',(54.1099666493497,19.214819841746,13.1639616503311));
#26121=CARTESIAN_POINT('Ctrl Pts',(54.1099790976895,19.2148136354588,13.1639625459625));
#26122=CARTESIAN_POINT('Ctrl Pts',(54.1100040372026,19.2148012018548,13.1639643402812));
#26123=CARTESIAN_POINT('Ctrl Pts',(54.110016529122,19.2147949741672,13.1639652390222));
#26124=CARTESIAN_POINT('Ctrl Pts',(54.1100416959498,19.2147824278949,13.1639670496434));
#26125=CARTESIAN_POINT('Ctrl Pts',(54.1100543702003,19.2147761096431,13.1639679614759));
#26126=CARTESIAN_POINT('Ctrl Pts',(54.1100799207794,19.214763372741,13.1639697996523));
#26127=CARTESIAN_POINT('Ctrl Pts',(54.1100927975956,19.2147569538531,13.1639707260309));
#26128=CARTESIAN_POINT('Ctrl Pts',(54.1101187570107,19.2147440138486,13.1639725935647));
#26129=CARTESIAN_POINT('Ctrl Pts',(54.1101318392338,19.2147374929248,13.1639735346924));
#26130=CARTESIAN_POINT('Ctrl Pts',(54.1101582133024,19.2147243469516,13.1639754319994));
#26131=CARTESIAN_POINT('Ctrl Pts',(54.1101715048128,19.2147177220749,13.1639763881542));
#26132=CARTESIAN_POINT('Ctrl Pts',(54.1101983004707,19.2147043667105,13.1639783157306));
#26133=CARTESIAN_POINT('Ctrl Pts',(54.1102118052133,19.2146976359322,13.1639792871947));
#26134=CARTESIAN_POINT('Ctrl Pts',(54.1102390312302,19.2146840668417,13.1639812456685));
#26135=CARTESIAN_POINT('Ctrl Pts',(54.1102527523704,19.2146772286024,13.1639822326682));
#26136=CARTESIAN_POINT('Ctrl Pts',(54.1102804149144,19.2146634427487,13.1639842224803));
#26137=CARTESIAN_POINT('Ctrl Pts',(54.1102943566378,19.2146564949814,13.1639852253152));
#26138=CARTESIAN_POINT('Ctrl Pts',(54.1140503420512,19.2127847789558,13.1642553908185));
#26139=CARTESIAN_POINT('Ctrl Pts',(54.1177981900082,19.2109318040402,13.1645238039627));
#26140=CARTESIAN_POINT('Ctrl Pts',(54.1262722930752,19.2067752234782,13.1651280909973));
#26141=CARTESIAN_POINT('Ctrl Pts',(54.1310018377536,19.2044785157176,13.1654635361336));
#26142=CARTESIAN_POINT('Ctrl Pts',(54.1449914117077,19.1977532815708,13.166450557768));
#26143=CARTESIAN_POINT('Ctrl Pts',(54.154276771849,19.1933774184629,13.167098983782));
#26144=CARTESIAN_POINT('Ctrl Pts',(54.263067348875,19.1431308214525,13.1746230639566));
#26145=CARTESIAN_POINT('Ctrl Pts',(54.3661707748302,19.1054550760183,13.1810481740207));
#26146=CARTESIAN_POINT('Ctrl Pts',(54.5519249078212,19.0544538498031,13.1922498803867));
#26147=CARTESIAN_POINT('Ctrl Pts',(54.6332832254596,19.0374914989848,13.1970369974516));
#26148=CARTESIAN_POINT('Ctrl Pts',(54.8072545128356,19.0124190516006,13.207366522913));
#26149=CARTESIAN_POINT('Ctrl Pts',(54.8998488882186,19.0056090324894,13.2129210942788));
#26150=CARTESIAN_POINT('Ctrl Pts',(55.0086644953452,19.0052039187941,13.219684646704));
#26151=CARTESIAN_POINT('Ctrl Pts',(55.0247550198719,19.0053387144123,13.2206905906412));
#26152=CARTESIAN_POINT('Ctrl Pts',(55.0496673900674,19.005848893205,13.2222577949478));
#26153=CARTESIAN_POINT('Ctrl Pts',(55.0584915752964,19.006088212097,13.2228148043749));
#26154=CARTESIAN_POINT('Ctrl Pts',(55.0740228197196,19.0066126198482,13.2237986305679));
#26155=CARTESIAN_POINT('Ctrl Pts',(55.0807306168594,19.0068730118513,13.2242246681378));
#26156=CARTESIAN_POINT('Ctrl Pts',(55.096038938696,19.007544674986,13.2251996019708));
#26157=CARTESIAN_POINT('Ctrl Pts',(55.1046383246279,19.0079777819749,13.2257491736448));
#26158=CARTESIAN_POINT('Ctrl Pts',(55.1279035185684,19.0093005934133,13.227241303376));
#26159=CARTESIAN_POINT('Ctrl Pts',(55.1425625105737,19.0102966681302,13.2281871676294));
#26160=CARTESIAN_POINT('Ctrl Pts',(55.2152295265051,19.0160415192611,13.2329052064708));
#26161=CARTESIAN_POINT('Ctrl Pts',(55.2730161530937,19.023165147672,13.2367508705642));
#26162=CARTESIAN_POINT('Ctrl Pts',(55.4906129060613,19.0597120256788,13.2515965390692));
#26163=CARTESIAN_POINT('Ctrl Pts',(55.6469242984393,19.1060900625544,13.2630786513237));
#26164=CARTESIAN_POINT('Ctrl Pts',(55.8382349054426,19.1893299055669,13.2774802506528));
#26165=CARTESIAN_POINT('Ctrl Pts',(55.8799670652333,19.2092396918734,13.2806395635415));
#26166=CARTESIAN_POINT('Ctrl Pts',(55.9363493045465,19.2385863482564,13.2848993423019));
#26167=CARTESIAN_POINT('Ctrl Pts',(55.9516218893416,19.2467904013168,13.2860522784054));
#26168=CARTESIAN_POINT('Ctrl Pts',(55.9778189193548,19.2613060024839,13.2880258522527));
#26169=CARTESIAN_POINT('Ctrl Pts',(55.9887938198554,19.2675238941072,13.2888514023551));
#26170=CARTESIAN_POINT('Ctrl Pts',(56.0045909633503,19.2766728742632,13.2900370588755));
#26171=CARTESIAN_POINT('Ctrl Pts',(56.0094606496076,19.2795208270001,13.2904021880637));
#26172=CARTESIAN_POINT('Ctrl Pts',(56.0179516095673,19.2845350810716,13.2910381109667));
#26173=CARTESIAN_POINT('Ctrl Pts',(56.0215781800895,19.2866922661739,13.2913094830586));
#26174=CARTESIAN_POINT('Ctrl Pts',(56.0292415573486,19.2912836400187,13.2918823961385));
#26175=CARTESIAN_POINT('Ctrl Pts',(56.0332765905225,19.2937206351729,13.292183751429));
#26176=CARTESIAN_POINT('Ctrl Pts',(56.0441687524262,19.3003518630932,13.292996514063));
#26177=CARTESIAN_POINT('Ctrl Pts',(56.0510093183234,19.3045733307325,13.2935061799832));
#26178=CARTESIAN_POINT('Ctrl Pts',(56.0822056767484,19.3240866770757,13.295827864345));
#26179=CARTESIAN_POINT('Ctrl Pts',(56.1062558862837,19.3398636476524,13.2976103086756));
#26180=CARTESIAN_POINT('Ctrl Pts',(56.1697479361262,19.3835072968306,13.3023196929081));
#26181=CARTESIAN_POINT('Ctrl Pts',(56.208534479318,19.4122960216605,13.3052007942238));
#26182=CARTESIAN_POINT('Ctrl Pts',(56.3193986718867,19.5010025360307,13.3135683086431));
#26183=CARTESIAN_POINT('Ctrl Pts',(56.3883436705159,19.5646223057637,13.3189509452437));
#26184=CARTESIAN_POINT('Ctrl Pts',(56.5330695691188,19.71839045646,13.3312541330218));
#26185=CARTESIAN_POINT('Ctrl Pts',(56.6058524116594,19.8108583526604,13.3382029864829));
#26186=CARTESIAN_POINT('Ctrl Pts',(56.6792525413191,19.9232362432246,13.3465386255131));
#26187=CARTESIAN_POINT('Ctrl Pts',(56.6882531349711,19.9374038346139,13.3475872789823));
#26188=CARTESIAN_POINT('Ctrl Pts',(56.7017900608253,19.9593181602232,13.3492067612603));
#26189=CARTESIAN_POINT('Ctrl Pts',(56.7064548180056,19.9669849697998,13.3497728669576));
#26190=CARTESIAN_POINT('Ctrl Pts',(56.7148613019076,19.981013861301,13.350808002227));
#26191=CARTESIAN_POINT('Ctrl Pts',(56.7186197754489,19.9873657616486,13.3512764107289));
#26192=CARTESIAN_POINT('Ctrl Pts',(56.7267479490431,20.0012781483663,13.3523018347732));
#26193=CARTESIAN_POINT('Ctrl Pts',(56.7311034107354,20.0088467354677,13.3528593530363));
#26194=CARTESIAN_POINT('Ctrl Pts',(56.7429169693733,20.0296908429339,13.3543940075389));
#26195=CARTESIAN_POINT('Ctrl Pts',(56.7502728491137,20.0430233259223,13.3553747734436));
#26196=CARTESIAN_POINT('Ctrl Pts',(56.7885183637418,20.1142593160344,13.3606117043748));
#26197=CARTESIAN_POINT('Ctrl Pts',(56.8166858774398,20.1735707601373,13.3649623631607));
#26198=CARTESIAN_POINT('Ctrl Pts',(56.9073418831237,20.3916014067321,13.3809261323497));
#26199=CARTESIAN_POINT('Ctrl Pts',(56.9523400268486,20.5567635717114,13.3930374396775));
#26200=CARTESIAN_POINT('Ctrl Pts',(56.983013953433,20.7776446074142,13.4083065002408));
#26201=CARTESIAN_POINT('Ctrl Pts',(56.9881817291651,20.8299390005005,13.4118483705794));
#26202=CARTESIAN_POINT('Ctrl Pts',(56.9918218090702,20.8915652872133,13.4158922598772));
#26203=CARTESIAN_POINT('Ctrl Pts',(56.9923007584585,20.9007533289248,13.4164917781646));
#26204=CARTESIAN_POINT('Ctrl Pts',(56.9929403771028,20.9149065935751,13.4174097114755));
#26205=CARTESIAN_POINT('Ctrl Pts',(56.9931460909666,20.9198695072251,13.4177305364264));
#26206=CARTESIAN_POINT('Ctrl Pts',(56.9934908010687,20.9290108054948,13.4183194679463));
#26207=CARTESIAN_POINT('Ctrl Pts',(56.9936351996028,20.9331888393247,13.4185878623057));
#26208=CARTESIAN_POINT('Ctrl Pts',(56.9939313351666,20.9426156452687,13.4191917011256));
#26209=CARTESIAN_POINT('Ctrl Pts',(56.9940754830542,20.9478645712495,13.4195267197051));
#26210=CARTESIAN_POINT('Ctrl Pts',(56.9944394192318,20.963343868403,13.4205113140172));
#26211=CARTESIAN_POINT('Ctrl Pts',(56.994601221146,20.9735756156382,13.4211577623104));
#26212=CARTESIAN_POINT('Ctrl Pts',(56.9952581150675,21.0545000958836,13.4262393051825));
#26213=CARTESIAN_POINT('Ctrl Pts',(56.9920736128489,21.1251808464537,13.4304893071425));
#26214=CARTESIAN_POINT('Ctrl Pts',(56.9696684273553,21.3526281485193,13.4439755165884));
#26215=CARTESIAN_POINT('Ctrl Pts',(56.9356078270219,21.5073113846432,13.4528976476747));
#26216=CARTESIAN_POINT('Ctrl Pts',(56.8639215187066,21.7130399933706,13.4659330209543));
#26217=CARTESIAN_POINT('Ctrl Pts',(56.8416275793222,21.7687888285813,13.4695860806875));
#26218=CARTESIAN_POINT('Ctrl Pts',(56.8109200389748,21.8365422702239,13.4742200466229));
#26219=CARTESIAN_POINT('Ctrl Pts',(56.8048424048327,21.8495753256964,13.4751205423652));
#26220=CARTESIAN_POINT('Ctrl Pts',(56.794967852447,21.8701663543857,13.4765582917405));
#26221=CARTESIAN_POINT('Ctrl Pts',(56.7912627897613,21.8777680160913,13.4770923638655));
#26222=CARTESIAN_POINT('Ctrl Pts',(56.7841917587462,21.8920443988625,13.478101714479));
#26223=CARTESIAN_POINT('Ctrl Pts',(56.7808363789624,21.8987242237698,13.4785766169138));
#26224=CARTESIAN_POINT('Ctrl Pts',(56.7731907237404,21.9137341050365,13.4796497759987));
#26225=CARTESIAN_POINT('Ctrl Pts',(56.7688791648874,21.9220530638426,13.4802487726748));
#26226=CARTESIAN_POINT('Ctrl Pts',(56.7576855390496,21.9432831840286,13.4817884164241));
#26227=CARTESIAN_POINT('Ctrl Pts',(56.7507198385662,21.9561493854894,13.4827320022363));
#26228=CARTESIAN_POINT('Ctrl Pts',(56.7049303252074,22.0385481025204,13.4888442212116));
#26229=CARTESIAN_POINT('Ctrl Pts',(56.6621184314045,22.1057707903553,13.4941553937547));
#26230=CARTESIAN_POINT('Ctrl Pts',(56.5235323631449,22.2970747430652,13.5102563425561));
#26231=CARTESIAN_POINT('Ctrl Pts',(56.4170510976158,22.4126264327628,13.5213656216321));
#26232=CARTESIAN_POINT('Ctrl Pts',(56.2594299682373,22.5477292524502,13.5355667301343));
#26233=CARTESIAN_POINT('Ctrl Pts',(56.2194363826203,22.5794320450986,13.5390035230186));
#26234=CARTESIAN_POINT('Ctrl Pts',(56.1708974109203,22.6149644716734,13.5429434687467));
#26235=CARTESIAN_POINT('Ctrl Pts',(56.1634900548479,22.6203091963027,13.5435386128046));
#26236=CARTESIAN_POINT('Ctrl Pts',(56.1520097383602,22.6284734129521,13.5444512824076));
#26237=CARTESIAN_POINT('Ctrl Pts',(56.1479626676961,22.6313288475467,13.5447711757342));
#26238=CARTESIAN_POINT('Ctrl Pts',(56.140479278764,22.636567157975,13.5453592324038));
#26239=CARTESIAN_POINT('Ctrl Pts',(56.1370461214531,22.6389542904317,13.54562767717));
#26240=CARTESIAN_POINT('Ctrl Pts',(56.1292704196938,22.6443246752342,13.5462326762208));
#26241=CARTESIAN_POINT('Ctrl Pts',(56.1249235552974,22.6473015251171,13.5465687972025));
#26242=CARTESIAN_POINT('Ctrl Pts',(56.112031417964,22.6560555797976,13.5475596704936));
#26243=CARTESIAN_POINT('Ctrl Pts',(56.1034529160478,22.6617838700465,13.5482112355812));
#26244=CARTESIAN_POINT('Ctrl Pts',(56.0301246618068,22.7099305611676,13.5537185541613));
#26245=CARTESIAN_POINT('Ctrl Pts',(55.9629927620481,22.7486186594499,13.5583517761349));
#26246=CARTESIAN_POINT('Ctrl Pts',(55.7723940951098,22.844144479652,13.5708872392046));
#26247=CARTESIAN_POINT('Ctrl Pts',(55.6451218917195,22.892427085968,13.5786099493198));
#26248=CARTESIAN_POINT('Ctrl Pts',(55.4669421871161,22.939937473651,13.5895516940523));
#26249=CARTESIAN_POINT('Ctrl Pts',(55.4195145791887,22.9507433009584,13.5924729413793));
#26250=CARTESIAN_POINT('Ctrl Pts',(55.3505204937149,22.9638303124372,13.5967656717079));
#26251=CARTESIAN_POINT('Ctrl Pts',(55.3292357823367,22.9675105738819,13.5980957392484));
#26252=CARTESIAN_POINT('Ctrl Pts',(55.2909138089191,22.9734974424378,13.6005032883256));
#26253=CARTESIAN_POINT('Ctrl Pts',(55.273898367483,22.9759308325099,13.6015767797631));
#26254=CARTESIAN_POINT('Ctrl Pts',(55.2478705667101,22.9793104373928,13.6032266120576));
#26255=CARTESIAN_POINT('Ctrl Pts',(55.2388794025959,22.9804156765837,13.6037979447293));
#26256=CARTESIAN_POINT('Ctrl Pts',(55.2224768187164,22.9823186397565,13.6048429208506));
#26257=CARTESIAN_POINT('Ctrl Pts',(55.2150678240449,22.9831361408097,13.6053159328538));
#26258=CARTESIAN_POINT('Ctrl Pts',(55.1990150365473,22.9848163733298,13.6063430302337));
#26259=CARTESIAN_POINT('Ctrl Pts',(55.1903698705967,22.9856642034945,13.6068975739475));
#26260=CARTESIAN_POINT('Ctrl Pts',(55.1759645977854,22.986981987716,13.6078240185887));
#26261=CARTESIAN_POINT('Ctrl Pts',(55.1702074762722,22.9874834268497,13.6081949181193));
#26262=CARTESIAN_POINT('Ctrl Pts',(55.1644483515698,22.987959834143,13.6085666014869));
#26263=CARTESIAN_POINT('Origin',(55.,21.,6.22095488139522));
#26264=CARTESIAN_POINT('',(55.1644484406754,22.987959826772,14.5675833348156));
#26265=CARTESIAN_POINT('',(55.1644483421761,22.9879598349201,14.4110001919405));
#26266=CARTESIAN_POINT('',(55.1644483516311,22.987959834138,6.22095488139522));
#26267=CARTESIAN_POINT('Ctrl Pts',(55.1644484406754,22.987959826772,14.5675833348156));
#26268=CARTESIAN_POINT('Ctrl Pts',(55.2293615346116,22.9825900718436,14.5630733720583));
#26269=CARTESIAN_POINT('Ctrl Pts',(55.2939982819238,22.9740420031108,14.5586139385604));
#26270=CARTESIAN_POINT('Ctrl Pts',(55.3751010560904,22.9592408043298,14.5531448422678));
#26271=CARTESIAN_POINT('Ctrl Pts',(55.3920364515031,22.9559224935625,14.552009956185));
#26272=CARTESIAN_POINT('Ctrl Pts',(55.4151860566451,22.9510738046064,14.5504703915496));
#26273=CARTESIAN_POINT('Ctrl Pts',(55.4214385526315,22.9497328026498,14.5500557501661));
#26274=CARTESIAN_POINT('Ctrl Pts',(55.43193773831,22.9474281279609,14.5493615957564));
#26275=CARTESIAN_POINT('Ctrl Pts',(55.4361878758565,22.946480583372,14.5490811806471));
#26276=CARTESIAN_POINT('Ctrl Pts',(55.4442538435536,22.9446545750929,14.5485501571781));
#26277=CARTESIAN_POINT('Ctrl Pts',(55.4480702321122,22.9437787841427,14.5482993939904));
#26278=CARTESIAN_POINT('Ctrl Pts',(55.4580825811185,22.9414500795779,14.5476427384746));
#26279=CARTESIAN_POINT('Ctrl Pts',(55.4642742718268,22.9399787281806,14.5472378927992));
#26280=CARTESIAN_POINT('Ctrl Pts',(55.4858401365881,22.9347447999691,14.5458317697475));
#26281=CARTESIAN_POINT('Ctrl Pts',(55.5011769514433,22.9308287805037,14.5448388348704));
#26282=CARTESIAN_POINT('Ctrl Pts',(55.6310014348631,22.8960289245606,14.5364810806502));
#26283=CARTESIAN_POINT('Ctrl Pts',(55.742587527945,22.8551711386366,14.5296025934339));
#26284=CARTESIAN_POINT('Ctrl Pts',(55.9875662338876,22.7397982313336,14.513890277932));
#26285=CARTESIAN_POINT('Ctrl Pts',(56.1173483031017,22.6594307872944,14.5050753123241));
#26286=CARTESIAN_POINT('Ctrl Pts',(56.2523901496823,22.5527217865993,14.4944263653171));
#26287=CARTESIAN_POINT('Ctrl Pts',(56.267865183234,22.540111640693,14.493182518623));
#26288=CARTESIAN_POINT('Ctrl Pts',(56.2905112953748,22.5210853523676,14.4913255888369));
#26289=CARTESIAN_POINT('Ctrl Pts',(56.2978297073094,22.5148458991882,14.4907196788233));
#26290=CARTESIAN_POINT('Ctrl Pts',(56.310777131024,22.5036446308662,14.4896371539748));
#26291=CARTESIAN_POINT('Ctrl Pts',(56.3164238407634,22.4987034837169,14.4891613981939));
#26292=CARTESIAN_POINT('Ctrl Pts',(56.3282680018735,22.4882206807575,14.4881556996631));
#26293=CARTESIAN_POINT('Ctrl Pts',(56.3344589414928,22.4826719156494,14.4876254646428));
#26294=CARTESIAN_POINT('Ctrl Pts',(56.3507772020487,22.4678613200574,14.4862155930389));
#26295=CARTESIAN_POINT('Ctrl Pts',(56.3608437945503,22.4585335291695,14.4853331751132));
#26296=CARTESIAN_POINT('Ctrl Pts',(56.4041756821201,22.4175427032645,14.4814784554678));
#26297=CARTESIAN_POINT('Ctrl Pts',(56.4364358929736,22.3848422343479,14.4784616381259));
#26298=CARTESIAN_POINT('Ctrl Pts',(56.4877853061844,22.3290659028967,14.473405281233));
#26299=CARTESIAN_POINT('Ctrl Pts',(56.507535789191,22.3066204478637,14.4713928337083));
#26300=CARTESIAN_POINT('Ctrl Pts',(56.6323850999874,22.1581351113796,14.4582267516101));
#26301=CARTESIAN_POINT('Ctrl Pts',(56.7220795815213,22.0199954993894,14.446576766347));
#26302=CARTESIAN_POINT('Ctrl Pts',(56.8165251011663,21.8258049566556,14.4317971794872));
#26303=CARTESIAN_POINT('Ctrl Pts',(56.8373829237018,21.7782944802025,14.4283012406006));
#26304=CARTESIAN_POINT('Ctrl Pts',(56.8597239486326,21.721483576121,14.4243026149135));
#26305=CARTESIAN_POINT('Ctrl Pts',(56.8630223335183,21.7129232134842,14.4237048590337));
#26306=CARTESIAN_POINT('Ctrl Pts',(56.8680137869616,21.6996975621244,14.4227889884675));
#26307=CARTESIAN_POINT('Ctrl Pts',(56.8697486460658,21.6950483354103,14.4224684812275));
#26308=CARTESIAN_POINT('Ctrl Pts',(56.8729136602905,21.6864688448005,14.4218797620316));
#26309=CARTESIAN_POINT('Ctrl Pts',(56.8743487978127,21.6825405764626,14.421611264952));
#26310=CARTESIAN_POINT('Ctrl Pts',(56.8775611433769,21.6736611803479,14.4210067249144));
#26311=CARTESIAN_POINT('Ctrl Pts',(56.8793311248382,21.6687075278258,14.4206711114234));
#26312=CARTESIAN_POINT('Ctrl Pts',(56.8838419450751,21.6559237076198,14.4198090990724));
#26313=CARTESIAN_POINT('Ctrl Pts',(56.8865536024371,21.6480832469886,14.4192843689955));
#26314=CARTESIAN_POINT('Ctrl Pts',(56.903174106196,21.5990384876873,14.4160252745442));
#26315=CARTESIAN_POINT('Ctrl Pts',(56.9157824355719,21.5574020826099,14.4133606354269));
#26316=CARTESIAN_POINT('Ctrl Pts',(56.9337224113522,21.4903244510905,14.4091802714765));
#26317=CARTESIAN_POINT('Ctrl Pts',(56.9399352393888,21.4651363090738,14.4076353521036));
#26318=CARTESIAN_POINT('Ctrl Pts',(56.9834248014552,21.2727550623486,14.3959758257715));
#26319=CARTESIAN_POINT('Ctrl Pts',(56.9995168696397,21.1015117574379,14.3863301297046));
#26320=CARTESIAN_POINT('Ctrl Pts',(56.9923528933298,20.8965718969566,14.3739844318136));
#26321=CARTESIAN_POINT('Ctrl Pts',(56.9903170430279,20.8628675703426,14.3719308129874));
#26322=CARTESIAN_POINT('Ctrl Pts',(56.9853372349462,20.8049115592792,14.3683487216906));
#26323=CARTESIAN_POINT('Ctrl Pts',(56.9828013029156,20.780631934187,14.3668326541626));
#26324=CARTESIAN_POINT('Ctrl Pts',(56.9785476254048,20.7460600248567,14.3646493098096));
#26325=CARTESIAN_POINT('Ctrl Pts',(56.9771936474027,20.735724592471,14.3639934431612));
#26326=CARTESIAN_POINT('Ctrl Pts',(56.9747090961813,20.7178481139968,14.3628533859654));
#26327=CARTESIAN_POINT('Ctrl Pts',(56.9736161642502,20.7103019936299,14.362370390806));
#26328=CARTESIAN_POINT('Ctrl Pts',(56.9714325966813,20.6958117558236,14.3614394946268));
#26329=CARTESIAN_POINT('Ctrl Pts',(56.9703484658814,20.688866761547,14.3609918060667));
#26330=CARTESIAN_POINT('Ctrl Pts',(56.9677045116741,20.672497690729,14.3599329655641));
#26331=CARTESIAN_POINT('Ctrl Pts',(56.9661136674601,20.6630788679681,14.3593208392441));
#26332=CARTESIAN_POINT('Ctrl Pts',(56.9603176986663,20.6302027495763,14.3571739963814));
#26333=CARTESIAN_POINT('Ctrl Pts',(56.9557600525039,20.6068104509004,14.3556281751802));
#26334=CARTESIAN_POINT('Ctrl Pts',(56.9200435820043,20.4395206975094,14.3444371656428));
#26335=CARTESIAN_POINT('Ctrl Pts',(56.8734616531101,20.2994070383391,14.3342872673897));
#26336=CARTESIAN_POINT('Ctrl Pts',(56.7600139272689,20.0530191940997,14.315369679798));
#26337=CARTESIAN_POINT('Ctrl Pts',(56.6977146555525,19.9453943315695,14.3066909156322));
#26338=CARTESIAN_POINT('Ctrl Pts',(56.6192988289345,19.8350857411271,14.297792523091));
#26339=CARTESIAN_POINT('Ctrl Pts',(56.6127081750923,19.8259785845401,14.2970579804466));
#26340=CARTESIAN_POINT('Ctrl Pts',(56.6028471213512,19.8125920405279,14.2959790385747));
#26341=CARTESIAN_POINT('Ctrl Pts',(56.599635952795,19.8082695871904,14.2956307715026));
#26342=CARTESIAN_POINT('Ctrl Pts',(56.5938942436287,19.80060587421,14.2950135831801));
#26343=CARTESIAN_POINT('Ctrl Pts',(56.5913706390698,19.7972595379314,14.2947441929351));
#26344=CARTESIAN_POINT('Ctrl Pts',(56.5858922482519,19.7900425417683,14.2941634390148));
#26345=CARTESIAN_POINT('Ctrl Pts',(56.582933834471,19.7861747445749,14.2938523343598));
#26346=CARTESIAN_POINT('Ctrl Pts',(56.5747656760069,19.7755764345018,14.2930001248658));
#26347=CARTESIAN_POINT('Ctrl Pts',(56.5695269000432,19.7688682774435,14.2924610134989));
#26348=CARTESIAN_POINT('Ctrl Pts',(56.5425096231466,19.7347259021575,14.2897174163848));
#26349=CARTESIAN_POINT('Ctrl Pts',(56.5200527158194,19.707833381212,14.2875574002061));
#26350=CARTESIAN_POINT('Ctrl Pts',(56.3754349317021,19.5436427760545,14.2742754877038));
#26351=CARTESIAN_POINT('Ctrl Pts',(56.23549082531,19.4231758216685,14.2640300362258));
#26352=CARTESIAN_POINT('Ctrl Pts',(56.0413734813089,19.2980029808521,14.2503078465309));
#26353=CARTESIAN_POINT('Ctrl Pts',(56.0008387005034,19.2738557376337,14.2474710488413));
#26354=CARTESIAN_POINT('Ctrl Pts',(55.9319258589028,19.2360470216284,14.2426630404869));
#26355=CARTESIAN_POINT('Ctrl Pts',(55.9040111801154,19.2215794835117,14.2407194429367));
#26356=CARTESIAN_POINT('Ctrl Pts',(55.8654286420034,19.2027261639514,14.2380328638508));
#26357=CARTESIAN_POINT('Ctrl Pts',(55.8550465092259,19.1977637684414,14.2373099264706));
#26358=CARTESIAN_POINT('Ctrl Pts',(55.8375251066228,19.18957446161,14.2360895807494));
#26359=CARTESIAN_POINT('Ctrl Pts',(55.8304086246978,19.1862992398256,14.235593849275));
#26360=CARTESIAN_POINT('Ctrl Pts',(55.816321535393,19.1799162218973,14.2346123106265));
#26361=CARTESIAN_POINT('Ctrl Pts',(55.8093520159161,19.1768063404754,14.2341265853721));
#26362=CARTESIAN_POINT('Ctrl Pts',(55.7939618311549,19.1700446959976,14.2330536715362));
#26363=CARTESIAN_POINT('Ctrl Pts',(55.7855335000787,19.1664109185617,14.2324658818037));
#26364=CARTESIAN_POINT('Ctrl Pts',(55.7558045348668,19.1538362148956,14.2303916459095));
#26365=CARTESIAN_POINT('Ctrl Pts',(55.734374620603,19.1452075429938,14.2288947230466));
#26366=CARTESIAN_POINT('Ctrl Pts',(55.5581554401755,19.0777862042917,14.2165666668146));
#26367=CARTESIAN_POINT('Ctrl Pts',(55.396773262277,19.0381149531003,14.2050784366996));
#26368=CARTESIAN_POINT('Ctrl Pts',(55.1338435051142,19.0072737116295,14.1866196242322));
#26369=CARTESIAN_POINT('Ctrl Pts',(55.0345638587751,19.0030820164188,14.179727857552));
#26370=CARTESIAN_POINT('Ctrl Pts',(54.918294947748,19.006850752652,14.1720124026656));
#26371=CARTESIAN_POINT('Ctrl Pts',(54.9012208300879,19.0076239409862,14.1708885968169));
#26372=CARTESIAN_POINT('Ctrl Pts',(54.8777983722197,19.008986462254,14.1693614917557));
#26373=CARTESIAN_POINT('Ctrl Pts',(54.8714403617689,19.009386886553,14.1689484334336));
#26374=CARTESIAN_POINT('Ctrl Pts',(54.8607447558036,19.0101119485195,14.1682561789776));
#26375=CARTESIAN_POINT('Ctrl Pts',(54.8564061461445,19.0104203240992,14.1679760913621));
#26376=CARTESIAN_POINT('Ctrl Pts',(54.8481594220523,19.011033593326,14.1674451230392));
#26377=CARTESIAN_POINT('Ctrl Pts',(54.8442511564492,19.0113358186032,14.1671940906777));
#26378=CARTESIAN_POINT('Ctrl Pts',(54.8339767208445,19.0121608128636,14.1665356775679));
#26379=CARTESIAN_POINT('Ctrl Pts',(54.8276120634056,19.0127026480322,14.1661293543224));
#26380=CARTESIAN_POINT('Ctrl Pts',(54.8053459822788,19.0147059760209,14.1647129268298));
#26381=CARTESIAN_POINT('Ctrl Pts',(54.7894591131672,19.0163278695472,14.16371132743));
#26382=CARTESIAN_POINT('Ctrl Pts',(54.665653337191,19.0304714109176,14.1559644317481));
#26383=CARTESIAN_POINT('Ctrl Pts',(54.5588866492733,19.0516017423512,14.149625526924));
#26384=CARTESIAN_POINT('Ctrl Pts',(54.360472960126,19.1080273245364,14.1376452646986));
#26385=CARTESIAN_POINT('Ctrl Pts',(54.2686733373609,19.1415824685915,14.1320134376288));
#26386=CARTESIAN_POINT('Ctrl Pts',(54.1362696029225,19.2013149978459,14.1233875266458));
#26387=CARTESIAN_POINT('Ctrl Pts',(54.0935550761498,19.2224581406175,14.1205230394317));
#26388=CARTESIAN_POINT('Ctrl Pts',(54.0237757220257,19.2601675587828,14.1156724185072));
#26389=CARTESIAN_POINT('Ctrl Pts',(53.9962748283227,19.2758867869798,14.1137145592166));
#26390=CARTESIAN_POINT('Ctrl Pts',(53.9592814076733,19.2982169517958,14.111011359504));
#26391=CARTESIAN_POINT('Ctrl Pts',(53.9494539757162,19.3042660074488,14.1102863937447));
#26392=CARTESIAN_POINT('Ctrl Pts',(53.9330384161305,19.3145677056132,14.1090635897438));
#26393=CARTESIAN_POINT('Ctrl Pts',(53.9264217966929,19.3187745900851,14.108567443592));
#26394=CARTESIAN_POINT('Ctrl Pts',(53.9134185719142,19.3271501777982,14.1075858367425));
#26395=CARTESIAN_POINT('Ctrl Pts',(53.9070307280628,19.3313167180536,14.1071004623603));
#26396=CARTESIAN_POINT('Ctrl Pts',(53.8930256300361,19.340566612275,14.106029240816));
#26397=CARTESIAN_POINT('Ctrl Pts',(53.8854192054744,19.3456659732998,14.1054427994931));
#26398=CARTESIAN_POINT('Ctrl Pts',(53.8588569140426,19.3637397284104,14.1033783509854));
#26399=CARTESIAN_POINT('Ctrl Pts',(53.8400908819979,19.3769886063771,14.1018899976664));
#26400=CARTESIAN_POINT('Ctrl Pts',(53.6869026723977,19.4891537960387,14.0894861330886));
#26401=CARTESIAN_POINT('Ctrl Pts',(53.565177328456,19.6042411258448,14.0779015065588));
#26402=CARTESIAN_POINT('Ctrl Pts',(53.4111161175704,19.7916073675277,14.0609893622592));
#26403=CARTESIAN_POINT('Ctrl Pts',(53.3663779420761,19.8528098698243,14.0557260601564));
#26404=CARTESIAN_POINT('Ctrl Pts',(53.3123304914988,19.9363445991311,14.0489967717729));
#26405=CARTESIAN_POINT('Ctrl Pts',(53.2997903433196,19.9565066314446,14.0474055263903));
#26406=CARTESIAN_POINT('Ctrl Pts',(53.2793841668678,19.9906605675428,14.0447705210168));
#26407=CARTESIAN_POINT('Ctrl Pts',(53.2713218852945,20.0045317934763,14.0437166607207));
#26408=CARTESIAN_POINT('Ctrl Pts',(53.2603700039721,20.0239089936291,14.0422685500441));
#26409=CARTESIAN_POINT('Ctrl Pts',(53.2573377199747,20.0293330354462,14.0418657810728));
#26410=CARTESIAN_POINT('Ctrl Pts',(53.2522412663261,20.0385502517893,14.0411858289364));
#26411=CARTESIAN_POINT('Ctrl Pts',(53.2501639925456,20.0423360935244,14.0409078227035));
#26412=CARTESIAN_POINT('Ctrl Pts',(53.2462097238927,20.0495985904577,14.0403769925807));
#26413=CARTESIAN_POINT('Ctrl Pts',(53.2443307494997,20.0530741025088,14.0401240383948));
#26414=CARTESIAN_POINT('Ctrl Pts',(53.2398710626449,20.0613820276678,14.0395218849998));
#26415=CARTESIAN_POINT('Ctrl Pts',(53.2372998903166,20.0662195658938,14.039173284125));
#26416=CARTESIAN_POINT('Ctrl Pts',(53.2281937837549,20.0835239130664,14.0379332814178));
#26417=CARTESIAN_POINT('Ctrl Pts',(53.2217707317588,20.0960495689596,14.0370485869542));
#26418=CARTESIAN_POINT('Ctrl Pts',(53.1495873117757,20.2405625449687,14.0269764460843));
#26419=CARTESIAN_POINT('Ctrl Pts',(53.0985149168603,20.3794032890881,14.0185596558212));
#26420=CARTESIAN_POINT('Ctrl Pts',(53.0358849707252,20.633502202271,14.0033530664845));
#26421=CARTESIAN_POINT('Ctrl Pts',(53.0181304662096,20.7465096121793,13.9966554336261));
#26422=CARTESIAN_POINT('Ctrl Pts',(53.0081882054466,20.8882347119888,13.9879364266095));
#26423=CARTESIAN_POINT('Ctrl Pts',(53.0068201074395,20.9160982666301,13.986207993474));
#26424=CARTESIAN_POINT('Ctrl Pts',(53.0057282057485,20.954963390269,13.983773398809));
#26425=CARTESIAN_POINT('Ctrl Pts',(53.0055103953854,20.9659486429579,13.9830826298762));
#26426=CARTESIAN_POINT('Ctrl Pts',(53.0052939779079,20.984663977028,13.9819010725921));
#26427=CARTESIAN_POINT('Ctrl Pts',(53.0052495282842,20.9923933567165,13.9814117250838));
#26428=CARTESIAN_POINT('Ctrl Pts',(53.0052504850896,21.0079467540437,13.9804242028299));
#26429=CARTESIAN_POINT('Ctrl Pts',(53.0052969989434,21.0157706322548,13.9799260021873));
#26430=CARTESIAN_POINT('Ctrl Pts',(53.005525073187,21.0350518205792,13.9786945822042));
#26431=CARTESIAN_POINT('Ctrl Pts',(53.0057593299444,21.0465081135775,13.9779597296151));
#26432=CARTESIAN_POINT('Ctrl Pts',(53.0069957512948,21.0890416510443,13.9752192726415));
#26433=CARTESIAN_POINT('Ctrl Pts',(53.0086257496548,21.1200948186305,13.9731942427279));
#26434=CARTESIAN_POINT('Ctrl Pts',(53.0145009090126,21.1974351800298,13.9680873232751));
#26435=CARTESIAN_POINT('Ctrl Pts',(53.0196391357429,21.2436341148892,13.9649795394447));
#26436=CARTESIAN_POINT('Ctrl Pts',(53.0517891573737,21.462728906901,13.9499746503123));
#26437=CARTESIAN_POINT('Ctrl Pts',(53.0998547917015,21.6317282184606,13.9375165699183));
#26438=CARTESIAN_POINT('Ctrl Pts',(53.1867708802,21.8325587071409,13.9226114738475));
#26439=CARTESIAN_POINT('Ctrl Pts',(53.2055291435125,21.8722550351427,13.9196653436872));
#26440=CARTESIAN_POINT('Ctrl Pts',(53.2293838955418,21.918703093575,13.9162447344476));
#26441=CARTESIAN_POINT('Ctrl Pts',(53.2332306394897,21.9260792601345,13.9157023496882));
#26442=CARTESIAN_POINT('Ctrl Pts',(53.2395882595204,21.9380862487584,13.9148210639096));
#26443=CARTESIAN_POINT('Ctrl Pts',(53.2420714866698,21.9427314833475,13.9144805114628));
#26444=CARTESIAN_POINT('Ctrl Pts',(53.2465595692612,21.9510476920887,13.9138716201301));
#26445=CARTESIAN_POINT('Ctrl Pts',(53.2485575889342,21.9547222310737,13.9136028625064));
#26446=CARTESIAN_POINT('Ctrl Pts',(53.2529486906367,21.9627376869267,13.9130172317539));
#26447=CARTESIAN_POINT('Ctrl Pts',(53.2553463953839,21.9670759704211,13.9127006570518));
#26448=CARTESIAN_POINT('Ctrl Pts',(53.2622149024497,21.9793948094236,13.9118027094929));
#26449=CARTESIAN_POINT('Ctrl Pts',(53.2667245328025,21.9873537362153,13.9112237493036));
#26450=CARTESIAN_POINT('Ctrl Pts',(53.2968703177657,22.0397141511899,13.907420811812));
#26451=CARTESIAN_POINT('Ctrl Pts',(53.3241578300516,22.0831483053803,13.9042944216293));
#26452=CARTESIAN_POINT('Ctrl Pts',(53.4426792464745,22.2565790427975,13.8917241216521));
#26453=CARTESIAN_POINT('Ctrl Pts',(53.547601651041,22.3765116959438,13.8827796187527));
#26454=CARTESIAN_POINT('Ctrl Pts',(53.723119961459,22.5344654540417,13.8688065725319));
#26455=CARTESIAN_POINT('Ctrl Pts',(53.7835509224349,22.5828001909222,13.8641442462939));
#26456=CARTESIAN_POINT('Ctrl Pts',(53.8584978242574,22.6359131807713,13.8584351832116));
#26457=CARTESIAN_POINT('Ctrl Pts',(53.8704572934478,22.644193543578,13.857526390785));
#26458=CARTESIAN_POINT('Ctrl Pts',(53.8902473645466,22.657577747841,13.8560255946221));
#26459=CARTESIAN_POINT('Ctrl Pts',(53.8980253083639,22.6627587546711,13.8554365071666));
#26460=CARTESIAN_POINT('Ctrl Pts',(53.9120894218765,22.6719850515613,13.8543725325962));
#26461=CARTESIAN_POINT('Ctrl Pts',(53.918362504011,22.6760500480064,13.8538983935244));
#26462=CARTESIAN_POINT('Ctrl Pts',(53.93179794511,22.684649456512,13.8528837389246));
#26463=CARTESIAN_POINT('Ctrl Pts',(53.9389666380248,22.6891736507874,13.8523428568426));
#26464=CARTESIAN_POINT('Ctrl Pts',(53.9584465043738,22.7012945514631,13.8508743197494));
#26465=CARTESIAN_POINT('Ctrl Pts',(53.97081164561,22.7088031331847,13.8499434588304));
#26466=CARTESIAN_POINT('Ctrl Pts',(54.0359005741929,22.7473648487979,13.8450493659504));
#26467=CARTESIAN_POINT('Ctrl Pts',(54.0899459354064,22.7761114503358,13.8410041104192));
#26468=CARTESIAN_POINT('Ctrl Pts',(54.2655814463229,22.8594089502896,13.8279080141916));
#26469=CARTESIAN_POINT('Ctrl Pts',(54.3913452861554,22.9042857210874,13.8185776021681));
#26470=CARTESIAN_POINT('Ctrl Pts',(54.6114865635207,22.9587871522235,13.8027955105519));
#26471=CARTESIAN_POINT('Ctrl Pts',(54.7038324356323,22.9748617112744,13.7963407463093));
#26472=CARTESIAN_POINT('Ctrl Pts',(54.8073661275801,22.9854543180277,13.7895059596357));
#26473=CARTESIAN_POINT('Ctrl Pts',(54.8177652173258,22.9864357913348,13.7888239877174));
#26474=CARTESIAN_POINT('Ctrl Pts',(54.8334490828663,22.987791843322,13.7878027350285));
#26475=CARTESIAN_POINT('Ctrl Pts',(54.838728233377,22.9882271095721,13.7874602277789));
#26476=CARTESIAN_POINT('Ctrl Pts',(54.8481807600026,22.9889685745262,13.7868492561749));
#26477=CARTESIAN_POINT('Ctrl Pts',(54.8523534102309,22.9892826741466,13.7865803603094));
#26478=CARTESIAN_POINT('Ctrl Pts',(54.8614477196279,22.9899384829904,13.7859960651939));
#26479=CARTESIAN_POINT('Ctrl Pts',(54.8663696600848,22.9902750649114,13.7856809539383));
#26480=CARTESIAN_POINT('Ctrl Pts',(54.8803126365673,22.9911765853319,13.7847913310554));
#26481=CARTESIAN_POINT('Ctrl Pts',(54.8893364731645,22.9916984837372,13.7842191620866));
#26482=CARTESIAN_POINT('Ctrl Pts',(54.9472040080615,22.9946507778431,13.7805712188871));
#26483=CARTESIAN_POINT('Ctrl Pts',(54.9961239825301,22.9953458342757,13.7775841143064));
#26484=CARTESIAN_POINT('Ctrl Pts',(55.084908104999,22.9933413419167,13.7722594047859));
#26485=CARTESIAN_POINT('Ctrl Pts',(55.1247339702184,22.9912450978968,13.7699062491208));
#26486=CARTESIAN_POINT('Ctrl Pts',(55.164448547645,22.9879598179233,13.7675726541794));
#26487=CARTESIAN_POINT('Ctrl Pts',(55.1644483515698,22.987959834143,13.6085666014869));
#26488=CARTESIAN_POINT('Ctrl Pts',(55.1552326810296,22.9887221744091,13.6091613639964));
#26489=CARTESIAN_POINT('Ctrl Pts',(55.1460118811662,22.9894204182803,13.6097581340933));
#26490=CARTESIAN_POINT('Ctrl Pts',(55.0742147507976,22.9943554019005,13.614418225141));
#26491=CARTESIAN_POINT('Ctrl Pts',(55.0114812601815,22.9957023950593,13.6185707941191));
#26492=CARTESIAN_POINT('Ctrl Pts',(54.7753659584723,22.9896392050039,13.634509728283));
#26493=CARTESIAN_POINT('Ctrl Pts',(54.6032901096987,22.9625831772774,13.64683481341));
#26494=CARTESIAN_POINT('Ctrl Pts',(54.3862326369373,22.898711765279,13.6623297639935));
#26495=CARTESIAN_POINT('Ctrl Pts',(54.3361748130347,22.8817954064775,13.6658917594645));
#26496=CARTESIAN_POINT('Ctrl Pts',(54.2782394161307,22.8596166521722,13.6699555182529));
#26497=CARTESIAN_POINT('Ctrl Pts',(54.2696584792937,22.8562633715277,13.6705558523518));
#26498=CARTESIAN_POINT('Ctrl Pts',(54.256484684089,22.8510097881214,13.6714747670405));
#26499=CARTESIAN_POINT('Ctrl Pts',(54.2518753173202,22.8491516220113,13.6717957654537));
#26500=CARTESIAN_POINT('Ctrl Pts',(54.2434015411673,22.8456987322848,13.6723848606567));
#26501=CARTESIAN_POINT('Ctrl Pts',(54.2395352176559,22.8441090948444,13.6726532464198));
#26502=CARTESIAN_POINT('Ctrl Pts',(54.230826724131,22.8404965556407,13.6732568727682));
#26503=CARTESIAN_POINT('Ctrl Pts',(54.225987531244,22.8384666979214,13.6735916888372));
#26504=CARTESIAN_POINT('Ctrl Pts',(54.2117498002453,22.8324283296861,13.674575131744));
#26505=CARTESIAN_POINT('Ctrl Pts',(54.2023738168039,22.8283666052521,13.6752206420438));
#26506=CARTESIAN_POINT('Ctrl Pts',(54.1287945310834,22.7958179472095,13.6802728110162));
#26507=CARTESIAN_POINT('Ctrl Pts',(54.0660977685595,22.7640266351161,13.6844967638576));
#26508=CARTESIAN_POINT('Ctrl Pts',(53.8584294408312,22.6445419023461,13.6986382274644));
#26509=CARTESIAN_POINT('Ctrl Pts',(53.7230098718175,22.5417522544769,13.7081850348504));
#26510=CARTESIAN_POINT('Ctrl Pts',(53.5661867791288,22.3877158739902,13.7214250823952));
#26511=CARTESIAN_POINT('Ctrl Pts',(53.5315324342184,22.3509915076265,13.7245127345336));
#26512=CARTESIAN_POINT('Ctrl Pts',(53.4893441650268,22.3027402092431,13.7285096865559));
#26513=CARTESIAN_POINT('Ctrl Pts',(53.480483681854,22.2923943859438,13.7293633304094));
#26514=CARTESIAN_POINT('Ctrl Pts',(53.4664026205106,22.2756078380143,13.7307434813898));
#26515=CARTESIAN_POINT('Ctrl Pts',(53.4611149262075,22.269223780535,13.7312672390336));
#26516=CARTESIAN_POINT('Ctrl Pts',(53.4511154310859,22.2569966170398,13.7322683437077));
#26517=CARTESIAN_POINT('Ctrl Pts',(53.4463965083495,22.251159498735,13.732745391274));
#26518=CARTESIAN_POINT('Ctrl Pts',(53.4356833825343,22.2377537301119,13.7338391010312));
#26519=CARTESIAN_POINT('Ctrl Pts',(53.4297109962708,22.2301679622852,13.7344566193493));
#26520=CARTESIAN_POINT('Ctrl Pts',(53.4142489581222,22.2102329316568,13.73607604599));
#26521=CARTESIAN_POINT('Ctrl Pts',(53.4048485997373,22.1978155547022,13.737081429881));
#26522=CARTESIAN_POINT('Ctrl Pts',(53.3226756472774,22.0865864480545,13.746059602146));
#26523=CARTESIAN_POINT('Ctrl Pts',(53.2590334048429,21.9813830255535,13.7543850699677));
#26524=CARTESIAN_POINT('Ctrl Pts',(53.1539588892651,21.7649011003796,13.7710729524641));
#26525=CARTESIAN_POINT('Ctrl Pts',(53.1119661341389,21.6544237371343,13.7793849919054));
#26526=CARTESIAN_POINT('Ctrl Pts',(53.0677109457882,21.4973270302254,13.7905067833987));
#26527=CARTESIAN_POINT('Ctrl Pts',(53.0569256536497,21.4533629566357,13.7935447706254));
#26528=CARTESIAN_POINT('Ctrl Pts',(53.0458288627724,21.4004011883377,13.797086959804));
#26529=CARTESIAN_POINT('Ctrl Pts',(53.0440709507393,21.3917237629658,13.7976635808229));
#26530=CARTESIAN_POINT('Ctrl Pts',(53.0414313645827,21.378233260775,13.7985539290278));
#26531=CARTESIAN_POINT('Ctrl Pts',(53.0405095527251,21.3734282896132,13.798869849064));
#26532=CARTESIAN_POINT('Ctrl Pts',(53.0388316660343,21.3645049518832,13.799454260354));
#26533=CARTESIAN_POINT('Ctrl Pts',(53.0380708849644,21.3603876276639,13.7997230056433));
#26534=CARTESIAN_POINT('Ctrl Pts',(53.0363678689131,21.3510057239655,13.8003333387237));
#26535=CARTESIAN_POINT('Ctrl Pts',(53.0354338392054,21.3457397373156,13.8006744596697));
#26536=CARTESIAN_POINT('Ctrl Pts',(53.0330550521478,21.3320073783509,13.8015603803308));
#26537=CARTESIAN_POINT('Ctrl Pts',(53.0316437571322,21.3235352138146,13.8021033521161));
#26538=CARTESIAN_POINT('Ctrl Pts',(53.022513574026,21.2664534518167,13.8057390894018));
#26539=CARTESIAN_POINT('Ctrl Pts',(53.0165406409558,21.2175772625025,13.8087422989965));
#26540=CARTESIAN_POINT('Ctrl Pts',(53.0113077993132,21.1558603929747,13.8124527177128));
#26541=CARTESIAN_POINT('Ctrl Pts',(53.010354985019,21.1431846913762,13.8132104534635));
#26542=CARTESIAN_POINT('Ctrl Pts',(53.0067133644929,21.0876404008832,13.8165151117823));
#26543=CARTESIAN_POINT('Ctrl Pts',(53.0052883198242,21.0446991606966,13.8190292034624));
#26544=CARTESIAN_POINT('Ctrl Pts',(53.0051004112123,20.8297844890478,13.8315441383399));
#26545=CARTESIAN_POINT('Ctrl Pts',(53.0271841667994,20.6585476207796,13.8413745515307));
#26546=CARTESIAN_POINT('Ctrl Pts',(53.076088910496,20.4727416621568,13.8532305597303));
#26547=CARTESIAN_POINT('Ctrl Pts',(53.0815242033495,20.4532955032256,13.8544853664092));
#26548=CARTESIAN_POINT('Ctrl Pts',(53.0903655818648,20.4234202470756,13.8564363483584));
#26549=CARTESIAN_POINT('Ctrl Pts',(53.0935641790469,20.412930774688,13.857125810002));
#26550=CARTESIAN_POINT('Ctrl Pts',(53.0991396392622,20.3951728152262,13.8583008293405));
#26551=CARTESIAN_POINT('Ctrl Pts',(53.1014721284444,20.3878905712694,13.8587849274342));
#26552=CARTESIAN_POINT('Ctrl Pts',(53.1062716892927,20.3731972748331,13.8597663084676));
#26553=CARTESIAN_POINT('Ctrl Pts',(53.1087405330266,20.3657869468544,13.8602636425215));
#26554=CARTESIAN_POINT('Ctrl Pts',(53.1149202533105,20.3475952809971,13.8614905357406));
#26555=CARTESIAN_POINT('Ctrl Pts',(53.1186801341652,20.3368310002522,13.8622217027224));
#26556=CARTESIAN_POINT('Ctrl Pts',(53.132906339246,20.2971971768613,13.8649334539297));
#26557=CARTESIAN_POINT('Ctrl Pts',(53.1439461598869,20.2685394646035,13.8669329419791));
#26558=CARTESIAN_POINT('Ctrl Pts',(53.2234973797775,20.0754477484288,13.880678381433));
#26559=CARTESIAN_POINT('Ctrl Pts',(53.313099378693,19.9206017473992,13.8931710848395));
#26560=CARTESIAN_POINT('Ctrl Pts',(53.4743873775082,19.7120326738856,13.9114860782814));
#26561=CARTESIAN_POINT('Ctrl Pts',(53.5310578951989,19.6477550954853,13.917365365667));
#26562=CARTESIAN_POINT('Ctrl Pts',(53.5990632581276,19.5799604876498,13.9236711847041));
#26563=CARTESIAN_POINT('Ctrl Pts',(53.6064946750295,19.5726672105381,13.9243509776469));
#26564=CARTESIAN_POINT('Ctrl Pts',(53.6177867970575,19.5617572533241,13.9253695567141));
#26565=CARTESIAN_POINT('Ctrl Pts',(53.6216052007718,19.5580973279101,13.9257115459211));
#26566=CARTESIAN_POINT('Ctrl Pts',(53.6284693276917,19.5515702733502,13.9263218908697));
#26567=CARTESIAN_POINT('Ctrl Pts',(53.6315095429552,19.548697506328,13.9265906751643));
#26568=CARTESIAN_POINT('Ctrl Pts',(53.6381576682861,19.5424550104279,13.9271750663853));
#26569=CARTESIAN_POINT('Ctrl Pts',(53.6417690524902,19.5390891103235,13.927490383341));
#26570=CARTESIAN_POINT('Ctrl Pts',(53.652042123791,19.5295853728367,13.9283814416333));
#26571=CARTESIAN_POINT('Ctrl Pts',(53.6587332771765,19.5234793609788,13.9289548274795));
#26572=CARTESIAN_POINT('Ctrl Pts',(53.7021494038424,19.4843986633062,13.9326323213344));
#26573=CARTESIAN_POINT('Ctrl Pts',(53.7400492425903,19.4527480578743,13.9356460848332));
#26574=CARTESIAN_POINT('Ctrl Pts',(53.8927069438089,19.3345955237736,13.9472160842204));
#26575=CARTESIAN_POINT('Ctrl Pts',(54.015500190837,19.2591853037528,13.9553533038039));
#26576=CARTESIAN_POINT('Ctrl Pts',(54.2297343189642,19.1575986300446,13.9692766790851));
#26577=CARTESIAN_POINT('Ctrl Pts',(54.3168277822866,19.1235606991914,13.974864813304));
#26578=CARTESIAN_POINT('Ctrl Pts',(54.4203994448019,19.0912519878277,13.9816025438931));
#26579=CARTESIAN_POINT('Ctrl Pts',(54.4348711646708,19.0869173678614,13.982545814019));
#26580=CARTESIAN_POINT('Ctrl Pts',(54.458535085499,19.0801214020428,13.9840918503576));
#26581=CARTESIAN_POINT('Ctrl Pts',(54.4676982955756,19.0775606706726,13.9846913868545));
#26582=CARTESIAN_POINT('Ctrl Pts',(54.4841069239701,19.0731014576758,13.9857666952262));
#26583=CARTESIAN_POINT('Ctrl Pts',(54.4913454228148,19.0711780338986,13.9862416494695));
#26584=CARTESIAN_POINT('Ctrl Pts',(54.5066933086353,19.0671921758369,13.9872500322995));
#26585=CARTESIAN_POINT('Ctrl Pts',(54.5148051649436,19.0651399158058,13.9877837790261));
#26586=CARTESIAN_POINT('Ctrl Pts',(54.5364992177966,19.0597964299018,13.9892134206866));
#26587=CARTESIAN_POINT('Ctrl Pts',(54.5501032971806,19.056596848612,13.9901122386008));
#26588=CARTESIAN_POINT('Ctrl Pts',(54.6170985919839,19.0415811776925,13.9945507300544));
#26589=CARTESIAN_POINT('Ctrl Pts',(54.6709220207241,19.0318220364986,13.9981552318035));
#26590=CARTESIAN_POINT('Ctrl Pts',(54.9273535185751,18.9961389185671,14.0155214132644));
#26591=CARTESIAN_POINT('Ctrl Pts',(55.132709605493,18.9992247218774,14.0301570547956));
#26592=CARTESIAN_POINT('Ctrl Pts',(55.3672970428133,19.0390662407924,14.0462332392441));
#26593=CARTESIAN_POINT('Ctrl Pts',(55.4004488271056,19.045566735589,14.0484853227566));
#26594=CARTESIAN_POINT('Ctrl Pts',(55.4416269381479,19.054732956356,14.051244887526));
#26595=CARTESIAN_POINT('Ctrl Pts',(55.4498206740082,19.0566113124633,14.0517921066951));
#26596=CARTESIAN_POINT('Ctrl Pts',(55.4627174697789,19.059653748901,14.0526501789461));
#26597=CARTESIAN_POINT('Ctrl Pts',(55.4674284692655,19.0607832358589,14.0529629355441));
#26598=CARTESIAN_POINT('Ctrl Pts',(55.4761706788522,19.0629129350446,14.0535419873109));
#26599=CARTESIAN_POINT('Ctrl Pts',(55.4802028440518,19.0639085657922,14.0538085288544));
#26600=CARTESIAN_POINT('Ctrl Pts',(55.4894661563551,19.066226601598,14.0544196701416));
#26601=CARTESIAN_POINT('Ctrl Pts',(55.4946950644523,19.0675576413675,14.0547637698372));
#26602=CARTESIAN_POINT('Ctrl Pts',(55.5108604042022,19.0717425075797,14.0558250399915));
#26603=CARTESIAN_POINT('Ctrl Pts',(55.5217782558515,19.0746681388843,14.0565382233852));
#26604=CARTESIAN_POINT('Ctrl Pts',(55.6266881328798,19.1037385498565,14.0633618606612));
#26605=CARTESIAN_POINT('Ctrl Pts',(55.7186809901207,19.1366566748165,14.0691208891382));
#26606=CARTESIAN_POINT('Ctrl Pts',(55.9701957201019,19.2480712858742,14.0851595728427));
#26607=CARTESIAN_POINT('Ctrl Pts',(56.1221468237173,19.3412910896098,14.095279618973));
#26608=CARTESIAN_POINT('Ctrl Pts',(56.2763957593493,19.4669305917009,14.107564665743));
#26609=CARTESIAN_POINT('Ctrl Pts',(56.2928117331088,19.4807483051178,14.1088997106308));
#26610=CARTESIAN_POINT('Ctrl Pts',(56.3165053711697,19.5013539194377,14.1108693038057));
#26611=CARTESIAN_POINT('Ctrl Pts',(56.3239605762672,19.5079360423095,14.1114953867825));
#26612=CARTESIAN_POINT('Ctrl Pts',(56.3370050112589,19.5196275798027,14.1126022813778));
#26613=CARTESIAN_POINT('Ctrl Pts',(56.3426149906431,19.52471362545,14.1130821079201));
#26614=CARTESIAN_POINT('Ctrl Pts',(56.3541506291313,19.5352922079741,14.1140767102123));
#26615=CARTESIAN_POINT('Ctrl Pts',(56.3600721395892,19.5407890439186,14.1145916637942));
#26616=CARTESIAN_POINT('Ctrl Pts',(56.3751900100117,19.55499466679,14.1159178315714));
#26617=CARTESIAN_POINT('Ctrl Pts',(56.3843370051199,19.5637552365189,14.1167312644698));
#26618=CARTESIAN_POINT('Ctrl Pts',(56.4225850927655,19.6010923231142,14.1201801946861));
#26619=CARTESIAN_POINT('Ctrl Pts',(56.4508878262971,19.6304690051292,14.122850579856));
#26620=CARTESIAN_POINT('Ctrl Pts',(56.5238546648181,19.7110064881066,14.1300649916758));
#26621=CARTESIAN_POINT('Ctrl Pts',(56.5668377417068,19.7636120208499,14.1346710711252));
#26622=CARTESIAN_POINT('Ctrl Pts',(56.670247848153,19.9042447540744,14.1466873406498));
#26623=CARTESIAN_POINT('Ctrl Pts',(56.7264463350414,19.9951174387021,14.1541844714237));
#26624=CARTESIAN_POINT('Ctrl Pts',(56.7849357355886,20.1092159277828,14.1630662903404));
#26625=CARTESIAN_POINT('Ctrl Pts',(56.794453949625,20.1285489648467,14.1645534724135));
#26626=CARTESIAN_POINT('Ctrl Pts',(56.8133940903769,20.168646192926,14.1675969791084));
#26627=CARTESIAN_POINT('Ctrl Pts',(56.8227771721309,20.1894256788189,14.1691521091866));
#26628=CARTESIAN_POINT('Ctrl Pts',(56.8456655685474,20.2425221898798,14.1730628060774));
#26629=CARTESIAN_POINT('Ctrl Pts',(56.8586805661273,20.2750441852979,14.1753999733126));
#26630=CARTESIAN_POINT('Ctrl Pts',(56.8737856235143,20.3158747167406,14.1782483943594));
#26631=CARTESIAN_POINT('Ctrl Pts',(56.8766869178166,20.3238741353695,14.178802410939));
#26632=CARTESIAN_POINT('Ctrl Pts',(56.8811674762443,20.3364789476145,14.1796687766491));
#26633=CARTESIAN_POINT('Ctrl Pts',(56.8827811801762,20.3410718632183,14.1799830888593));
#26634=CARTESIAN_POINT('Ctrl Pts',(56.885752499689,20.3496288533142,14.1805660679371));
#26635=CARTESIAN_POINT('Ctrl Pts',(56.8871144282388,20.3535912641945,14.1808349776391));
#26636=CARTESIAN_POINT('Ctrl Pts',(56.8901974933762,20.3626539619936,14.1814476624666));
#26637=CARTESIAN_POINT('Ctrl Pts',(56.8919104760574,20.3677569388699,14.1817909562176));
#26638=CARTESIAN_POINT('Ctrl Pts',(56.8971354101909,20.3835334132539,14.1828472500474));
#26639=CARTESIAN_POINT('Ctrl Pts',(56.900577922197,20.3942299176702,14.1835563167646));
#26640=CARTESIAN_POINT('Ctrl Pts',(56.9379355574339,20.5137609590034,14.1914069741198));
#26641=CARTESIAN_POINT('Ctrl Pts',(56.9625567734565,20.6252985017048,14.1980668246599));
#26642=CARTESIAN_POINT('Ctrl Pts',(56.9982640914052,20.8951620098877,14.2138806702175));
#26643=CARTESIAN_POINT('Ctrl Pts',(57.0002854480263,21.0538730371714,14.2229844269306));
#26644=CARTESIAN_POINT('Ctrl Pts',(56.9810830727581,21.2342594280995,14.234163188077));
#26645=CARTESIAN_POINT('Ctrl Pts',(56.9782195767754,21.2573224764076,14.2356069528073));
#26646=CARTESIAN_POINT('Ctrl Pts',(56.9736258783564,21.2896856142171,14.2376555528477));
#26647=CARTESIAN_POINT('Ctrl Pts',(56.9722314020644,21.2990320293709,14.238249848864));
#26648=CARTESIAN_POINT('Ctrl Pts',(56.9696881184416,21.3152860753282,14.2392881622505));
#26649=CARTESIAN_POINT('Ctrl Pts',(56.968569242743,21.3221982739227,14.2397312285548));
#26650=CARTESIAN_POINT('Ctrl Pts',(56.9661530929869,21.3366422234673,14.2406603062273));
#26651=CARTESIAN_POINT('Ctrl Pts',(56.9648488830199,21.3441726832681,14.2411465305528));
#26652=CARTESIAN_POINT('Ctrl Pts',(56.9616442947634,21.3620637733453,14.2423061899184));
#26653=CARTESIAN_POINT('Ctrl Pts',(56.9597050775083,21.3724171280815,14.2429808478972));
#26654=CARTESIAN_POINT('Ctrl Pts',(56.9528729210201,21.4073617313167,14.2452703336611));
#26655=CARTESIAN_POINT('Ctrl Pts',(56.9475985272008,21.4318751064799,14.2468972158502));
#26656=CARTESIAN_POINT('Ctrl Pts',(56.9338669976195,21.4903143579195,14.2508274124513));
#26657=CARTESIAN_POINT('Ctrl Pts',(56.9249774460853,21.5241291057028,14.253143835649));
#26658=CARTESIAN_POINT('Ctrl Pts',(56.8867005629468,21.6555782990492,14.2623159788075));
#26659=CARTESIAN_POINT('Ctrl Pts',(56.8507372021531,21.751125433209,14.2693597588999));
#26660=CARTESIAN_POINT('Ctrl Pts',(56.7790310395837,21.9047937759995,14.2811779849764));
#26661=CARTESIAN_POINT('Ctrl Pts',(56.7473274725101,21.9645984917734,14.2859083468611));
#26662=CARTESIAN_POINT('Ctrl Pts',(56.7003912857594,22.0432010491635,14.2922275432127));
#26663=CARTESIAN_POINT('Ctrl Pts',(56.6877678910154,22.0635029699285,14.2938691794522));
#26664=CARTESIAN_POINT('Ctrl Pts',(56.6504508708863,22.1211805295448,14.2985512865359));
#26665=CARTESIAN_POINT('Ctrl Pts',(56.6248574781147,22.1579605905424,14.3015596788477));
#26666=CARTESIAN_POINT('Ctrl Pts',(56.5930382263116,22.2005526893131,14.3050428551924));
#26667=CARTESIAN_POINT('Ctrl Pts',(56.5879890641782,22.207223379591,14.3055883576664));
#26668=CARTESIAN_POINT('Ctrl Pts',(56.5796844998341,22.2180526793506,14.3064736253656));
#26669=CARTESIAN_POINT('Ctrl Pts',(56.5764543479728,22.2222303952221,14.306815067054));
#26670=CARTESIAN_POINT('Ctrl Pts',(56.5706363010165,22.2296937275913,14.3074248286645));
#26671=CARTESIAN_POINT('Ctrl Pts',(56.5680546379799,22.2329840660302,14.307693573564));
#26672=CARTESIAN_POINT('Ctrl Pts',(56.5623989964131,22.2401457064855,14.3082783358295));
#26673=CARTESIAN_POINT('Ctrl Pts',(56.5593209753191,22.244013703508,14.3085940603173));
#26674=CARTESIAN_POINT('Ctrl Pts',(56.5505430761194,22.2549606888105,14.3094874355758));
#26675=CARTESIAN_POINT('Ctrl Pts',(56.5448090650583,22.2620123301088,14.3100627114176));
#26676=CARTESIAN_POINT('Ctrl Pts',(56.5072131176887,22.3076073258052,14.313782881599));
#26677=CARTESIAN_POINT('Ctrl Pts',(56.4739566353184,22.3449836698419,14.3168349971958));
#26678=CARTESIAN_POINT('Ctrl Pts',(56.3364950593736,22.4882433787389,14.3287283432958));
#26679=CARTESIAN_POINT('Ctrl Pts',(56.2220103895296,22.5835984311233,14.337125201163));
#26680=CARTESIAN_POINT('Ctrl Pts',(56.0244248342823,22.713868832438,14.3510551936972));
#26681=CARTESIAN_POINT('Ctrl Pts',(55.9477315762915,22.7574397888886,14.3563404981603));
#26682=CARTESIAN_POINT('Ctrl Pts',(55.8549404295896,22.802311978598,14.3627426891505));
#26683=CARTESIAN_POINT('Ctrl Pts',(55.8413926171499,22.8086763256673,14.3636774326731));
#26684=CARTESIAN_POINT('Ctrl Pts',(55.8191564738538,22.8188182866302,14.3652122668273));
#26685=CARTESIAN_POINT('Ctrl Pts',(55.8105104337895,22.8226876090458,14.365809206426));
#26686=CARTESIAN_POINT('Ctrl Pts',(55.7949834026363,22.8295040259626,14.3668816454909));
#26687=CARTESIAN_POINT('Ctrl Pts',(55.7881127198565,22.8324742644264,14.3673563444551));
#26688=CARTESIAN_POINT('Ctrl Pts',(55.7735036196259,22.8386925094156,14.3683660824166));
#26689=CARTESIAN_POINT('Ctrl Pts',(55.765761115191,22.8419304831257,14.3689014509013));
#26690=CARTESIAN_POINT('Ctrl Pts',(55.7449670824066,22.8504729358417,14.3703400232282));
#26691=CARTESIAN_POINT('Ctrl Pts',(55.7318795975686,22.8556880874539,14.3712462143558));
#26692=CARTESIAN_POINT('Ctrl Pts',(55.666396575968,22.8809815423083,14.375785018258));
#26693=CARTESIAN_POINT('Ctrl Pts',(55.6132299796831,22.8989797040246,14.3794860583233));
#26694=CARTESIAN_POINT('Ctrl Pts',(55.4303683420704,22.9524024021443,14.3922770566148));
#26695=CARTESIAN_POINT('Ctrl Pts',(55.2980493655483,22.9769080689736,14.4016636059742));
#26696=CARTESIAN_POINT('Ctrl Pts',(55.1644483421759,22.9879598349201,14.4110001919405));
#26697=CARTESIAN_POINT('Origin',(55.,21.,6.22095488139522));
#26698=CARTESIAN_POINT('',(55.1642080971762,22.984919470593,15.3685782038315));
#26699=CARTESIAN_POINT('',(55.1646076307061,22.9900841388564,15.2105321270573));
#26700=CARTESIAN_POINT('',(55.1644483516311,22.987959834138,6.22095488139522));
#26701=CARTESIAN_POINT('',(53.0046263220794,20.9982271535794,14.7790451186048));
#26702=CARTESIAN_POINT('Ctrl Pts',(53.0046263220794,20.9982271535794,14.7790451186048));
#26703=CARTESIAN_POINT('Ctrl Pts',(53.0033880615454,20.8638533255282,14.7876313150491));
#26704=CARTESIAN_POINT('Ctrl Pts',(53.0770257042585,20.0681393313831,14.8385619430631));
#26705=CARTESIAN_POINT('Ctrl Pts',(54.1456767166442,18.8023905785495,14.9318370026467));
#26706=CARTESIAN_POINT('Ctrl Pts',(56.3832764285273,19.090575541161,15.0588702973557));
#26707=CARTESIAN_POINT('Ctrl Pts',(57.354408655632,21.1269461461278,15.1859035920647));
#26708=CARTESIAN_POINT('Ctrl Pts',(56.3918339859998,22.6873870777271,15.28913956089));
#26709=CARTESIAN_POINT('Ctrl Pts',(55.4549141389281,22.9618400383867,15.3500310981456));
#26710=CARTESIAN_POINT('Ctrl Pts',(55.1642080971762,22.984919470593,15.3685782038315));
#26711=CARTESIAN_POINT('Ctrl Pts',(53.0052508056195,20.9982072316684,14.7786858855498));
#26712=CARTESIAN_POINT('Ctrl Pts',(53.0051093009901,21.1556543710583,14.7695402577617));
#26713=CARTESIAN_POINT('Ctrl Pts',(53.0236076901605,21.312552534886,14.7604750581731));
#26714=CARTESIAN_POINT('Ctrl Pts',(53.0641633313545,21.4814866269597,14.749769145838));
#26715=CARTESIAN_POINT('Ctrl Pts',(53.0681602132696,21.4972805989829,14.7487594584664));
#26716=CARTESIAN_POINT('Ctrl Pts',(53.075878523736,21.5262816119864,14.7468882376772));
#26717=CARTESIAN_POINT('Ctrl Pts',(53.0795436455624,21.5395027028071,14.7460285268067));
#26718=CARTESIAN_POINT('Ctrl Pts',(53.0856479955576,21.5606719783708,14.7446408189508));
#26719=CARTESIAN_POINT('Ctrl Pts',(53.0880010821416,21.5686447036245,14.7441156253189));
#26720=CARTESIAN_POINT('Ctrl Pts',(53.092572889085,21.5837856479163,14.7431132553435));
#26721=CARTESIAN_POINT('Ctrl Pts',(53.0947823623488,21.5909565270189,14.7426363883998));
#26722=CARTESIAN_POINT('Ctrl Pts',(53.0999163811918,21.6072909736035,14.7415451769942));
#26723=CARTESIAN_POINT('Ctrl Pts',(53.1028668375154,21.6164461400038,14.7409299917306));
#26724=CARTESIAN_POINT('Ctrl Pts',(53.1107285025393,21.6402495273016,14.7393209935814));
#26725=CARTESIAN_POINT('Ctrl Pts',(53.1157438035436,21.6548624375776,14.7383237790047));
#26726=CARTESIAN_POINT('Ctrl Pts',(53.1648368827078,21.7926684031044,14.7288278777595));
#26727=CARTESIAN_POINT('Ctrl Pts',(53.2207570566107,21.9112791596017,14.7199246561726));
#26728=CARTESIAN_POINT('Ctrl Pts',(53.3255730378848,22.086609720519,14.7057310781512));
#26729=CARTESIAN_POINT('Ctrl Pts',(53.3667306207798,22.1475440924894,14.7005850891718));
#26730=CARTESIAN_POINT('Ctrl Pts',(53.4582853228461,22.2681559085178,14.6900858798536));
#26731=CARTESIAN_POINT('Ctrl Pts',(53.5090192190398,22.3274346080632,14.6847479978984));
#26732=CARTESIAN_POINT('Ctrl Pts',(53.5705907605057,22.3913782638125,14.6789119312165));
#26733=CARTESIAN_POINT('Ctrl Pts',(53.5781465600205,22.3990986579342,14.6782059539672));
#26734=CARTESIAN_POINT('Ctrl Pts',(53.5888524565059,22.4098614614895,14.6772203570995));
#26735=CARTESIAN_POINT('Ctrl Pts',(53.5919502573058,22.4129552905459,14.6769368753826));
#26736=CARTESIAN_POINT('Ctrl Pts',(53.5981365333277,22.4190930860855,14.6763741957952));
#26737=CARTESIAN_POINT('Ctrl Pts',(53.601224810976,22.4221372430092,14.6760949834341));
#26738=CARTESIAN_POINT('Ctrl Pts',(53.6071324196211,22.4279225917131,14.6755641205512));
#26739=CARTESIAN_POINT('Ctrl Pts',(53.609949954986,22.4306655435169,14.6753123270914));
#26740=CARTESIAN_POINT('Ctrl Pts',(53.6174129771987,22.4378881507121,14.6746489899062));
#26741=CARTESIAN_POINT('Ctrl Pts',(53.6220721708681,22.4423536702372,14.6742385342098));
#26742=CARTESIAN_POINT('Ctrl Pts',(53.6386194410553,22.4580597404909,14.6727933379997));
#26743=CARTESIAN_POINT('Ctrl Pts',(53.6506244218265,22.469176920175,14.671767562946));
#26744=CARTESIAN_POINT('Ctrl Pts',(53.7567534380884,22.5650589808827,14.6628811330546));
#26745=CARTESIAN_POINT('Ctrl Pts',(53.8586295358653,22.6408394260659,14.6555717324402));
#26746=CARTESIAN_POINT('Ctrl Pts',(54.0534641712264,22.7587804738662,14.6423584557538));
#26747=CARTESIAN_POINT('Ctrl Pts',(54.1437573468979,22.8044626034304,14.6364893593641));
#26748=CARTESIAN_POINT('Ctrl Pts',(54.2692546348302,22.8564074377094,14.6283215275186));
#26749=CARTESIAN_POINT('Ctrl Pts',(54.3017335613391,22.8688662710383,14.6262078070782));
#26750=CARTESIAN_POINT('Ctrl Pts',(54.3578366913226,22.8887206223258,14.6225450979));
#26751=CARTESIAN_POINT('Ctrl Pts',(54.3813037084655,22.8965374024671,14.621009708445));
#26752=CARTESIAN_POINT('Ctrl Pts',(54.4150430480052,22.9070830223147,14.6187947846496));
#26753=CARTESIAN_POINT('Ctrl Pts',(54.425201842738,22.9101694587418,14.6181269312347));
#26754=CARTESIAN_POINT('Ctrl Pts',(54.442730913073,22.9153426313239,14.6169727086636));
#26755=CARTESIAN_POINT('Ctrl Pts',(54.4500895295623,22.917468305461,14.6164876180453));
#26756=CARTESIAN_POINT('Ctrl Pts',(54.4641843143264,22.9214520395255,14.6155573354789));
#26757=CARTESIAN_POINT('Ctrl Pts',(54.4709183735436,22.9233171916543,14.6151123820768));
#26758=CARTESIAN_POINT('Ctrl Pts',(54.4867195398463,22.9276044225198,14.6140671024935));
#26759=CARTESIAN_POINT('Ctrl Pts',(54.4957941554183,22.9299979538326,14.6134658624168));
#26760=CARTESIAN_POINT('Ctrl Pts',(54.5270237474313,22.9379998244758,14.6113933377087));
#26761=CARTESIAN_POINT('Ctrl Pts',(54.5492573440115,22.9432912394195,14.6099119345449));
#26762=CARTESIAN_POINT('Ctrl Pts',(54.7307005610402,22.9831919782937,14.5977703076172));
#26763=CARTESIAN_POINT('Ctrl Pts',(54.8934838760922,22.9985510965638,14.586476208462));
#26764=CARTESIAN_POINT('Ctrl Pts',(55.0923963267766,22.9929364532975,14.5725991760173));
#26765=CARTESIAN_POINT('Ctrl Pts',(55.128464834068,22.9909364704228,14.5700833654849));
#26766=CARTESIAN_POINT('Ctrl Pts',(55.1644484406754,22.987959826772,14.5675833348156));
#26767=CARTESIAN_POINT('',(53.008286603288,21.0001954942154,14.6208388173789));
#26768=CARTESIAN_POINT('Ctrl Pts',(55.1644483421759,22.9879598349201,14.4110001919405));
#26769=CARTESIAN_POINT('Ctrl Pts',(55.1025335197272,22.9930815631004,14.4153270529764));
#26770=CARTESIAN_POINT('Ctrl Pts',(55.0403429528252,22.9953139133895,14.4196373367823));
#26771=CARTESIAN_POINT('Ctrl Pts',(54.9391576233513,22.9942017486132,14.4265037334952));
#26772=CARTESIAN_POINT('Ctrl Pts',(54.9002566347636,22.9926349756726,14.4291080060147));
#26773=CARTESIAN_POINT('Ctrl Pts',(54.8526457235039,22.9893194070754,14.4322325079126));
#26774=CARTESIAN_POINT('Ctrl Pts',(54.843871854374,22.9886500434199,14.4328056692727));
#26775=CARTESIAN_POINT('Ctrl Pts',(54.8301851532795,22.9875147363219,14.4336953604483));
#26776=CARTESIAN_POINT('Ctrl Pts',(54.8252692631919,22.9870885939376,14.4340140251934));
#26777=CARTESIAN_POINT('Ctrl Pts',(54.8161889224585,22.9862674915272,14.4346009394302));
#26778=CARTESIAN_POINT('Ctrl Pts',(54.8120241578351,22.9858776758514,14.4348694619184));
#26779=CARTESIAN_POINT('Ctrl Pts',(54.8025929498459,22.9849649937103,14.4354760417209));
#26780=CARTESIAN_POINT('Ctrl Pts',(54.7973273504136,22.9844342690985,14.4358136556978));
#26781=CARTESIAN_POINT('Ctrl Pts',(54.7813468556045,22.9827593098309,14.4368352573577));
#26782=CARTESIAN_POINT('Ctrl Pts',(54.7706388539653,22.9815491806167,14.4375156758485));
#26783=CARTESIAN_POINT('Ctrl Pts',(54.7458760669907,22.9785472741259,14.4390807163507));
#26784=CARTESIAN_POINT('Ctrl Pts',(54.731829359033,22.9766923942108,14.4399621628217));
#26785=CARTESIAN_POINT('Ctrl Pts',(54.6837955439313,22.969828023617,14.4429583091842));
#26786=CARTESIAN_POINT('Ctrl Pts',(54.6499171229389,22.9640901080659,14.445040543394));
#26787=CARTESIAN_POINT('Ctrl Pts',(54.4609054062164,22.9270310622953,14.4565672192785));
#26788=CARTESIAN_POINT('Ctrl Pts',(54.309777818485,22.8782096791687,14.4654836054982));
#26789=CARTESIAN_POINT('Ctrl Pts',(54.0952420959614,22.7794685099114,14.4794549762261));
#26790=CARTESIAN_POINT('Ctrl Pts',(54.0264587439206,22.7427881013267,14.4841503144741));
#26791=CARTESIAN_POINT('Ctrl Pts',(53.9464756337429,22.6939200656817,14.4899755749277));
#26792=CARTESIAN_POINT('Ctrl Pts',(53.9330497691615,22.6854957612994,14.4909662574186));
#26793=CARTESIAN_POINT('Ctrl Pts',(53.912358916783,22.6721666288084,14.4925138332816));
#26794=CARTESIAN_POINT('Ctrl Pts',(53.9050232677481,22.6673722776486,14.4930666325735));
#26795=CARTESIAN_POINT('Ctrl Pts',(53.8919639779343,22.6587137862896,14.4940582822601));
#26796=CARTESIAN_POINT('Ctrl Pts',(53.8862283289142,22.6548679445042,14.4944964415168));
#26797=CARTESIAN_POINT('Ctrl Pts',(53.8802595549919,22.6508207025449,14.4949551911354));
#26798=CARTESIAN_POINT('Ctrl Pts',(53.8800063257327,22.6506489105012,14.4949746591452));
#26799=CARTESIAN_POINT('Ctrl Pts',(53.8795253008057,22.6503224190407,14.495011649832));
#26800=CARTESIAN_POINT('Ctrl Pts',(53.8792974976222,22.6501677307131,14.4950291720878));
#26801=CARTESIAN_POINT('Ctrl Pts',(53.8788616430457,22.649871634506,14.4950627054653));
#26802=CARTESIAN_POINT('Ctrl Pts',(53.8786535863363,22.6497302344156,14.4950787162922));
#26803=CARTESIAN_POINT('Ctrl Pts',(53.8782531247459,22.6494579608178,14.4951095403133));
#26804=CARTESIAN_POINT('Ctrl Pts',(53.8780607159613,22.6493270929619,14.4951243532949));
#26805=CARTESIAN_POINT('Ctrl Pts',(53.8776884852326,22.6490738229802,14.4951530161208));
#26806=CARTESIAN_POINT('Ctrl Pts',(53.8775086604149,22.6489514251107,14.4951668658026));
#26807=CARTESIAN_POINT('Ctrl Pts',(53.8771592385969,22.6487135072958,14.4951937826131));
#26808=CARTESIAN_POINT('Ctrl Pts',(53.8769896393652,22.648597990571,14.4952068496208));
#26809=CARTESIAN_POINT('Ctrl Pts',(53.8766588068039,22.6483725805295,14.495232343694));
#26810=CARTESIAN_POINT('Ctrl Pts',(53.8764975717951,22.6482626897404,14.4952447706619));
#26811=CARTESIAN_POINT('Ctrl Pts',(53.8761819658174,22.6480475185686,14.4952690997552));
#26812=CARTESIAN_POINT('Ctrl Pts',(53.8760275934384,22.647942240099,14.4952810018115));
#26813=CARTESIAN_POINT('Ctrl Pts',(53.875724476518,22.6477354588122,14.4953043758796));
#26814=CARTESIAN_POINT('Ctrl Pts',(53.8755757309428,22.6476339575533,14.4953158478311));
#26815=CARTESIAN_POINT('Ctrl Pts',(53.8752828315722,22.6474340302458,14.4953384411914));
#26816=CARTESIAN_POINT('Ctrl Pts',(53.8751386769664,22.6473356054281,14.4953495625522));
#26817=CARTESIAN_POINT('Ctrl Pts',(53.8748540759329,22.6471412328596,14.495371522582));
#26818=CARTESIAN_POINT('Ctrl Pts',(53.8747136288809,22.6470452860819,14.4953823612124));
#26819=CARTESIAN_POINT('Ctrl Pts',(53.8744356769868,22.6468553503576,14.4954038146436));
#26820=CARTESIAN_POINT('Ctrl Pts',(53.874298171582,22.6467613621098,14.4954144294208));
#26821=CARTESIAN_POINT('Ctrl Pts',(53.8740254277067,22.6465748849939,14.4954354870817));
#26822=CARTESIAN_POINT('Ctrl Pts',(53.8738901889127,22.6464823967223,14.4954459299397));
#26823=CARTESIAN_POINT('Ctrl Pts',(53.873621374154,22.6462985087565,14.4954666902657));
#26824=CARTESIAN_POINT('Ctrl Pts',(53.8734877978484,22.6462071094185,14.4954770077237));
#26825=CARTESIAN_POINT('Ctrl Pts',(53.8732217582993,22.6460250248098,14.4954975596111));
#26826=CARTESIAN_POINT('Ctrl Pts',(53.8730892949882,22.6459343398811,14.4955077940219));
#26827=CARTESIAN_POINT('Ctrl Pts',(53.8651859058975,22.6405222458142,14.4961185142975));
#26828=CARTESIAN_POINT('Ctrl Pts',(53.857452866986,22.6351459601498,14.4967210803998));
#26829=CARTESIAN_POINT('Ctrl Pts',(53.8328907857349,22.6178102131982,14.4986512397652));
#26830=CARTESIAN_POINT('Ctrl Pts',(53.8162096629667,22.6056444776907,14.4999867032378));
#26831=CARTESIAN_POINT('Ctrl Pts',(53.7358047920365,22.5450702047642,14.5065473137775));
#26832=CARTESIAN_POINT('Ctrl Pts',(53.6748522179466,22.4931215575001,14.5119100962587));
#26833=CARTESIAN_POINT('Ctrl Pts',(53.519837697439,22.3440210519825,14.526622370619));
#26834=CARTESIAN_POINT('Ctrl Pts',(53.4322504196806,22.2407378132037,14.5361592718706));
#26835=CARTESIAN_POINT('Ctrl Pts',(53.3473020019213,22.1170680822263,14.5464974362038));
#26836=CARTESIAN_POINT('Ctrl Pts',(53.3389631226623,22.104630382423,14.5475256766446));
#26837=CARTESIAN_POINT('Ctrl Pts',(53.3037601590698,22.0508239224615,14.5519215548976));
#26838=CARTESIAN_POINT('Ctrl Pts',(53.2782930410174,22.0085566723762,14.5552436711169));
#26839=CARTESIAN_POINT('Ctrl Pts',(53.250258121056,21.9578646940406,14.5590407028151));
#26840=CARTESIAN_POINT('Ctrl Pts',(53.2461476171676,21.9503174420168,14.5596012747505));
#26841=CARTESIAN_POINT('Ctrl Pts',(53.2395576314333,21.9380292361754,14.560506017031));
#26842=CARTESIAN_POINT('Ctrl Pts',(53.2370482726526,21.9333045535219,14.5608519853716));
#26843=CARTESIAN_POINT('Ctrl Pts',(53.2326087691644,21.9248639531808,14.5614666056552));
#26844=CARTESIAN_POINT('Ctrl Pts',(53.2306712912535,21.9211520049568,14.5617357120715));
#26845=CARTESIAN_POINT('Ctrl Pts',(53.2264957827786,21.9130905102161,14.5623175688376));
#26846=CARTESIAN_POINT('Ctrl Pts',(53.2242620610533,21.9087388303437,14.5626300496195));
#26847=CARTESIAN_POINT('Ctrl Pts',(53.2180327110184,21.8964922953067,14.5635050410681));
#26848=CARTESIAN_POINT('Ctrl Pts',(53.2140735127537,21.8885788899191,14.5640653290017));
#26849=CARTESIAN_POINT('Ctrl Pts',(53.1902325619024,21.8401239507384,14.5674665658638));
#26850=CARTESIAN_POINT('Ctrl Pts',(53.1716777679201,21.7989398953987,14.5702321044402));
#26851=CARTESIAN_POINT('Ctrl Pts',(53.1144998916092,21.6595770000029,14.5792934216638));
#26852=CARTESIAN_POINT('Ctrl Pts',(53.0822639643949,21.5589671205267,14.5853631052236));
#26853=CARTESIAN_POINT('Ctrl Pts',(53.0297027811058,21.335270770168,14.598705662906));
#26854=CARTESIAN_POINT('Ctrl Pts',(53.0126463155418,21.2118908127092,14.605980964456));
#26855=CARTESIAN_POINT('Ctrl Pts',(53.0063349151494,21.0685313378505,14.6148170626009));
#26856=CARTESIAN_POINT('Ctrl Pts',(53.0057671401622,21.0493181132451,14.6160086110643));
#26857=CARTESIAN_POINT('Ctrl Pts',(53.005326135664,21.0200959110041,14.6178333923284));
#26858=CARTESIAN_POINT('Ctrl Pts',(53.0052504320197,21.0100908251943,14.6184603853498));
#26859=CARTESIAN_POINT('Ctrl Pts',(53.0052500018438,21.0000857659472,14.6190897100634));
#26860=CARTESIAN_POINT('Ctrl Pts',(53.0084881004496,21.0002027753601,14.6209548813952));
#26861=CARTESIAN_POINT('Ctrl Pts',(53.0088012939876,20.6548595780746,14.6429136572615));
#26862=CARTESIAN_POINT('Ctrl Pts',(53.2585703182277,19.6431460319286,14.7072168646974));
#26863=CARTESIAN_POINT('Ctrl Pts',(54.8687658122962,18.6458264387637,14.813864503703));
#26864=CARTESIAN_POINT('Ctrl Pts',(56.9069018544316,19.6132480805813,14.940897798412));
#26865=CARTESIAN_POINT('Ctrl Pts',(57.199161840635,21.8503192148488,15.0679310931209));
#26866=CARTESIAN_POINT('Ctrl Pts',(55.981387458458,22.8822711615308,15.1578092026694));
#26867=CARTESIAN_POINT('Ctrl Pts',(55.2454399918933,22.9840771000814,15.2053428806482));
#26868=CARTESIAN_POINT('Ctrl Pts',(55.1646076307061,22.9900841388564,15.2105321270573));
#26869=CARTESIAN_POINT('Origin',(55.,21.,6.22095488139522));
#26870=CARTESIAN_POINT('',(55.1644483516311,22.987959834138,16.1684645359809));
#26871=CARTESIAN_POINT('',(55.1644482585673,22.9879598418364,16.0088160704683));
#26872=CARTESIAN_POINT('',(55.1644483516311,22.987959834138,6.22095488139522));
#26873=CARTESIAN_POINT('',(53.0052502923665,21.0010799982591,15.5790451544755));
#26874=CARTESIAN_POINT('Ctrl Pts',(53.0052502923665,21.0010799982591,15.5790451544755));
#26875=CARTESIAN_POINT('Ctrl Pts',(53.0052131657774,20.9325074313172,15.5834434861452));
#26876=CARTESIAN_POINT('Ctrl Pts',(53.0087162052572,20.8637923838756,15.5878418178149));
#26877=CARTESIAN_POINT('Ctrl Pts',(53.0157771547505,20.7953362198876,15.5922401494845));
#26878=CARTESIAN_POINT('Ctrl Pts',(53.022827440247,20.7269834437393,15.5966318384506));
#26879=CARTESIAN_POINT('Ctrl Pts',(53.0334249181497,20.6588892708525,15.6010235274166));
#26880=CARTESIAN_POINT('Ctrl Pts',(53.0475353187344,20.5914547382354,15.6054152163827));
#26881=CARTESIAN_POINT('Ctrl Pts',(53.061633981611,20.5240763008969,15.6098032521312));
#26882=CARTESIAN_POINT('Ctrl Pts',(53.0792396735167,20.4573569060938,15.6141912878797));
#26883=CARTESIAN_POINT('Ctrl Pts',(53.1002665442361,20.3916905725279,15.6185793236282));
#26884=CARTESIAN_POINT('Ctrl Pts',(53.1212834799863,20.3260552655952,15.6229652860773));
#26885=CARTESIAN_POINT('Ctrl Pts',(53.1457182362593,20.2614725111638,15.6273512485263));
#26886=CARTESIAN_POINT('Ctrl Pts',(53.1734347757927,20.1983223564196,15.6317372109753));
#26887=CARTESIAN_POINT('Ctrl Pts',(53.2011481786548,20.1351793483568,15.6361226770665));
#26888=CARTESIAN_POINT('Ctrl Pts',(53.2321424242669,20.0734690776151,15.6405081431577));
#26889=CARTESIAN_POINT('Ctrl Pts',(53.2662336402944,20.0135509275928,15.6448936092488));
#26890=CARTESIAN_POINT('Ctrl Pts',(53.3003564985035,19.9535771638022,15.6492831457643));
#26891=CARTESIAN_POINT('Ctrl Pts',(53.3375818183001,19.8953992801179,15.6536726822798));
#26892=CARTESIAN_POINT('Ctrl Pts',(53.3776806739743,19.8393503685851,15.6580622187953));
#26893=CARTESIAN_POINT('Ctrl Pts',(53.4177985411012,19.7832748834453,15.6624538364541));
#26894=CARTESIAN_POINT('Ctrl Pts',(53.4607923417108,19.7293307723388,15.6668454541129));
#26895=CARTESIAN_POINT('Ctrl Pts',(53.5063926899687,19.677818179704,15.6712370717717));
#26896=CARTESIAN_POINT('Ctrl Pts',(53.5520741810312,19.6262139238168,15.6756365040238));
#26897=CARTESIAN_POINT('Ctrl Pts',(53.6003711274293,19.5770501834321,15.6800359362758));
#26898=CARTESIAN_POINT('Ctrl Pts',(53.6509777244895,19.5305897568492,15.6844353685279));
#26899=CARTESIAN_POINT('Ctrl Pts',(53.6877926491778,19.496791058557,15.6876358359855));
#26900=CARTESIAN_POINT('Ctrl Pts',(53.7258291234092,19.4644221954192,15.690836303443));
#26901=CARTESIAN_POINT('Ctrl Pts',(53.7649596425576,19.4335700213579,15.6940367709006));
#26902=CARTESIAN_POINT('Ctrl Pts',(53.819423624556,19.3906282897056,15.6984913553475));
#26903=CARTESIAN_POINT('Ctrl Pts',(53.8762374044059,19.3504456850435,15.7029459397944));
#26904=CARTESIAN_POINT('Ctrl Pts',(53.935089962567,19.3132889474855,15.7074005242413));
#26905=CARTESIAN_POINT('Ctrl Pts',(53.9938542289503,19.276187953204,15.711848425832));
#26906=CARTESIAN_POINT('Ctrl Pts',(54.0546507925009,19.2421040753733,15.7162963274228));
#26907=CARTESIAN_POINT('Ctrl Pts',(54.1171366007932,19.211263076682,15.7207442290135));
#26908=CARTESIAN_POINT('Ctrl Pts',(54.1795489420745,19.1804583389603,15.7251869010322));
#26909=CARTESIAN_POINT('Ctrl Pts',(54.2436461466312,19.1528891232233,15.7296295730509));
#26910=CARTESIAN_POINT('Ctrl Pts',(54.3090588417498,19.128736288404,15.7340722450696));
#26911=CARTESIAN_POINT('Ctrl Pts',(54.3744304090047,19.1045986395436,15.7385121237833));
#26912=CARTESIAN_POINT('Ctrl Pts',(54.4411153679474,19.0838732794765,15.742952002497));
#26913=CARTESIAN_POINT('Ctrl Pts',(54.5087239574729,19.0666931406166,15.7473918812107));
#26914=CARTESIAN_POINT('Ctrl Pts',(54.5763129955656,19.0495179700061,15.7518304759752));
#26915=CARTESIAN_POINT('Ctrl Pts',(54.6448246598927,19.0358861057982,15.7562690707398));
#26916=CARTESIAN_POINT('Ctrl Pts',(54.7138553196154,19.0258802507478,15.7607076655043));
#26917=CARTESIAN_POINT('Ctrl Pts',(54.7828894559218,19.0158738917736,15.7651464838093));
#26918=CARTESIAN_POINT('Ctrl Pts',(54.8524421548205,19.0094939723416,15.7695853021143));
#26919=CARTESIAN_POINT('Ctrl Pts',(54.9221026877489,19.0067715707315,15.7740241204193));
#26920=CARTESIAN_POINT('Ctrl Pts',(54.9918369190813,19.0040462889159,15.7784676348386));
#26921=CARTESIAN_POINT('Ctrl Pts',(55.0616787221389,19.0049862673432,15.7829111492579));
#26922=CARTESIAN_POINT('Ctrl Pts',(55.1312163458724,19.0095704400618,15.7873546636772));
#26923=CARTESIAN_POINT('Ctrl Pts',(55.2007946366043,19.0141572936966,15.791800776753));
#26924=CARTESIAN_POINT('Ctrl Pts',(55.2700679078115,19.0223925257482,15.7962468898287));
#26925=CARTESIAN_POINT('Ctrl Pts',(55.3386312988932,19.0342033660854,15.8006930029045));
#26926=CARTESIAN_POINT('Ctrl Pts',(55.4073138594396,19.0460347347468,15.8051468437327));
#26927=CARTESIAN_POINT('Ctrl Pts',(55.4752835997395,19.0614540089214,15.8096006845609));
#26928=CARTESIAN_POINT('Ctrl Pts',(55.5421483674747,19.0803378656273,15.8140545253892));
#26929=CARTESIAN_POINT('Ctrl Pts',(55.577256078285,19.0902529375354,15.816393038796));
#26930=CARTESIAN_POINT('Ctrl Pts',(55.6120594570637,19.1011223144444,15.8187315522028));
#26931=CARTESIAN_POINT('Ctrl Pts',(55.646504023642,19.112922865934,15.8210700656096));
#26932=CARTESIAN_POINT('Ctrl Pts',(55.7121167458579,19.135401485461,15.8255246500565));
#26933=CARTESIAN_POINT('Ctrl Pts',(55.7766852636897,19.1613505471637,15.8299792345034));
#26934=CARTESIAN_POINT('Ctrl Pts',(55.8398168110724,19.1906533537378,15.8344338189503));
#26935=CARTESIAN_POINT('Ctrl Pts',(55.9028536472525,19.2199121996589,15.838881720541));
#26936=CARTESIAN_POINT('Ctrl Pts',(55.9644573513741,19.2525145999698,15.8433296221317));
#26937=CARTESIAN_POINT('Ctrl Pts',(56.0242522191242,19.2882947233478,15.8477775237224));
#26938=CARTESIAN_POINT('Ctrl Pts',(56.0839767837076,19.324032778634,15.8522201957412));
#26939=CARTESIAN_POINT('Ctrl Pts',(56.1418963179344,19.3629408863146,15.8566628677599));
#26940=CARTESIAN_POINT('Ctrl Pts',(56.1976585757808,19.4048067520332,15.8611055397786));
#26941=CARTESIAN_POINT('Ctrl Pts',(56.2533857734214,19.4466462948244,15.8655454184923));
#26942=CARTESIAN_POINT('Ctrl Pts',(56.3069579949739,19.4914396132661,15.8699852972059));
#26943=CARTESIAN_POINT('Ctrl Pts',(56.3580522089396,19.5389312951493,15.8744251759196));
#26944=CARTESIAN_POINT('Ctrl Pts',(56.4091316471927,19.5864092431203,15.8788637706842));
#26945=CARTESIAN_POINT('Ctrl Pts',(56.457734142166,19.6365836723948,15.8833023654487));
#26946=CARTESIAN_POINT('Ctrl Pts',(56.5035713466246,19.6891602813046,15.8877409602132));
#26947=CARTESIAN_POINT('Ctrl Pts',(56.5494108595773,19.7417395381245,15.8921797785182));
#26948=CARTESIAN_POINT('Ctrl Pts',(56.5924844857156,19.796720844287,15.8966185968233));
#26949=CARTESIAN_POINT('Ctrl Pts',(56.6325434059738,19.8537759424478,15.9010574151283));
#26950=CARTESIAN_POINT('Ctrl Pts',(56.6726447071665,19.9108914029041,15.9055009295476));
#26951=CARTESIAN_POINT('Ctrl Pts',(56.709724654796,19.9700846330709,15.9099444439669));
#26952=CARTESIAN_POINT('Ctrl Pts',(56.7435776888094,20.0309982427332,15.9143879583862));
#26953=CARTESIAN_POINT('Ctrl Pts',(56.7774505207568,20.0919474758975,15.9188340714619));
#26954=CARTESIAN_POINT('Ctrl Pts',(56.8080924678627,20.1546186513152,15.9232801845377));
#26955=CARTESIAN_POINT('Ctrl Pts',(56.8353451499069,20.2186321332349,15.9277262976134));
#26956=CARTESIAN_POINT('Ctrl Pts',(56.8626451996131,20.2827568764597,15.9321801384416));
#26957=CARTESIAN_POINT('Ctrl Pts',(56.886544057494,20.3482281236182,15.9366339792699));
#26958=CARTESIAN_POINT('Ctrl Pts',(56.9069327103309,20.4146495060479,15.9410878200981));
#26959=CARTESIAN_POINT('Ctrl Pts',(56.917637883651,20.4495244149868,15.9434263335049));
#26960=CARTESIAN_POINT('Ctrl Pts',(56.927376200681,20.4846610583987,15.9457648469118));
#26961=CARTESIAN_POINT('Ctrl Pts',(56.9361375560808,20.5200011182998,15.9481033603186));
#26962=CARTESIAN_POINT('Ctrl Pts',(56.9528268756218,20.5873196466979,15.9525579447655));
#26963=CARTESIAN_POINT('Ctrl Pts',(56.9660340164727,20.655642547169,15.9570125292124));
#26964=CARTESIAN_POINT('Ctrl Pts',(56.9756440654991,20.7245765279461,15.9614671136593));
#26965=CARTESIAN_POINT('Ctrl Pts',(56.9852396973388,20.7934070925945,15.96591501525));
#26966=CARTESIAN_POINT('Ctrl Pts',(56.9912488810164,20.8628464371986,15.9703629168407));
#26967=CARTESIAN_POINT('Ctrl Pts',(56.9936072387921,20.9324889643411,15.9748108184314));
#26968=CARTESIAN_POINT('Ctrl Pts',(56.9959628237542,21.0020496100382,15.9792534904501));
#26969=CARTESIAN_POINT('Ctrl Pts',(56.9946760916894,21.0718124770158,15.9836961624689));
#26970=CARTESIAN_POINT('Ctrl Pts',(56.9897344243389,21.1413664850692,15.9881388344876));
#26971=CARTESIAN_POINT('Ctrl Pts',(56.9847958640339,21.2108767614316,15.9925787132013));
#26972=CARTESIAN_POINT('Ctrl Pts',(56.9762069618547,21.2801779523193,15.9970185919149));
#26973=CARTESIAN_POINT('Ctrl Pts',(56.9640071694412,21.3488601451638,16.0014584706286));
#26974=CARTESIAN_POINT('Ctrl Pts',(56.9518109050323,21.4175224761049,16.0058970653932));
#26975=CARTESIAN_POINT('Ctrl Pts',(56.9360059089185,21.4855656827349,16.0103356601577));
#26976=CARTESIAN_POINT('Ctrl Pts',(56.9166831156036,21.5525879087167,16.0147742549222));
#26977=CARTESIAN_POINT('Ctrl Pts',(56.8973593491372,21.6196135101313,16.0192130732272));
#26978=CARTESIAN_POINT('Ctrl Pts',(56.8745175716195,21.6856175592179,16.0236518915322));
#26979=CARTESIAN_POINT('Ctrl Pts',(56.8482986813516,21.7502130010964,16.0280907098372));
#26980=CARTESIAN_POINT('Ctrl Pts',(56.822052052416,21.81487678269,16.0325342242565));
#26981=CARTESIAN_POINT('Ctrl Pts',(56.7924213639965,21.8781285282594,16.0369777386758));
#26982=CARTESIAN_POINT('Ctrl Pts',(56.7595954488438,21.9396017341982,16.0414212530951));
#26983=CARTESIAN_POINT('Ctrl Pts',(56.7267503364369,22.001110890902,16.0458673661709));
#26984=CARTESIAN_POINT('Ctrl Pts',(56.6907065309271,22.0608390185728,16.0503134792466));
#26985=CARTESIAN_POINT('Ctrl Pts',(56.6516971384873,22.1184471937526,16.0547595923223));
#26986=CARTESIAN_POINT('Ctrl Pts',(56.612619944144,22.1761554972268,16.0592134331506));
#26987=CARTESIAN_POINT('Ctrl Pts',(56.5705671690884,22.2317361028605,16.0636672739788));
#26988=CARTESIAN_POINT('Ctrl Pts',(56.525812746943,22.2848824941473,16.068121114807));
#26989=CARTESIAN_POINT('Ctrl Pts',(56.502314193618,22.3127872966186,16.0704596282139));
#26990=CARTESIAN_POINT('Ctrl Pts',(56.478071471137,22.3400216303825,16.0727981416207));
#26991=CARTESIAN_POINT('Ctrl Pts',(56.4531281009969,22.3665453832907,16.0751366550276));
#26992=CARTESIAN_POINT('Ctrl Pts',(56.4056260482042,22.4170571106084,16.0795901104623));
#26993=CARTESIAN_POINT('Ctrl Pts',(56.3553933595571,22.4651887889572,16.0840435658969));
#26994=CARTESIAN_POINT('Ctrl Pts',(56.3026979752753,22.5106308442878,16.0884970213315));
#26995=CARTESIAN_POINT('Ctrl Pts',(56.2500754348441,22.5560100824602,16.0929443204994));
#26996=CARTESIAN_POINT('Ctrl Pts',(56.1949973185801,22.5987067557146,16.0973916196673));
#26997=CARTESIAN_POINT('Ctrl Pts',(56.1377693807795,22.6384469471608,16.1018389188352));
#26998=CARTESIAN_POINT('Ctrl Pts',(56.0806011129274,22.6781457026359,16.1062815809304));
#26999=CARTESIAN_POINT('Ctrl Pts',(56.0212878714928,22.714893815648,16.1107242430255));
#27000=CARTESIAN_POINT('Ctrl Pts',(55.9601682043401,22.7484577724024,16.1151669051206));
#27001=CARTESIAN_POINT('Ctrl Pts',(55.8990649478455,22.7820127172193,16.119608374359));
#27002=CARTESIAN_POINT('Ctrl Pts',(55.8361566447006,22.8123849462518,16.1240498435973));
#27003=CARTESIAN_POINT('Ctrl Pts',(55.7718094973695,22.839385131578,16.1284913128357));
#27004=CARTESIAN_POINT('Ctrl Pts',(55.7075011255453,22.8663690466278,16.1329301056505));
#27005=CARTESIAN_POINT('Ctrl Pts',(55.6417560895648,22.889984779647,16.1373688984653));
#27006=CARTESIAN_POINT('Ctrl Pts',(55.5749614015851,22.9100908222352,16.1418076912801));
#27007=CARTESIAN_POINT('Ctrl Pts',(55.5081063016138,22.930215049594,16.1462504987302));
#27008=CARTESIAN_POINT('Ctrl Pts',(55.4402001196311,22.9468230912987,16.1506933061804));
#27009=CARTESIAN_POINT('Ctrl Pts',(55.3716455595063,22.9598232421826,16.1551361136305));
#27010=CARTESIAN_POINT('Ctrl Pts',(55.3030909993815,22.9728233930666,16.1595789210806));
#27011=CARTESIAN_POINT('Ctrl Pts',(55.2338885481216,22.9822155903893,16.1640217285307));
#27012=CARTESIAN_POINT('Ctrl Pts',(55.1644483516311,22.987959834138,16.1684645359809));
#27013=CARTESIAN_POINT('Ctrl Pts',(55.1642080971762,22.984919470593,15.3685782038315));
#27014=CARTESIAN_POINT('Ctrl Pts',(54.791210469995,23.0145321109006,15.3923755297153));
#27015=CARTESIAN_POINT('Ctrl Pts',(53.7301334665886,22.8199335201067,15.4585172871686));
#27016=CARTESIAN_POINT('Ctrl Pts',(53.033386236972,21.787011120162,15.5286729254264));
#27017=CARTESIAN_POINT('Ctrl Pts',(53.0022835510889,21.0637411429413,15.5750312378004));
#27018=CARTESIAN_POINT('Ctrl Pts',(53.0026935992604,21.0010819424674,15.5790451186048));
#27019=CARTESIAN_POINT('',(53.0049939673739,20.9981913424498,15.420954726227));
#27020=CARTESIAN_POINT('Ctrl Pts',(55.1646076307061,22.9900841388564,15.2105321270573));
#27021=CARTESIAN_POINT('Ctrl Pts',(54.5858451071959,23.0330947458601,15.2476873122178));
#27022=CARTESIAN_POINT('Ctrl Pts',(53.4459374565242,22.6200279605996,15.3178281786077));
#27023=CARTESIAN_POINT('Ctrl Pts',(53.0097639809454,21.5146609743285,15.3879690449977));
#27024=CARTESIAN_POINT('Ctrl Pts',(53.0049939673739,20.9981913424498,15.420954726227));
#27025=CARTESIAN_POINT('Ctrl Pts',(53.0052508126406,20.9981994364738,15.421102452815));
#27026=CARTESIAN_POINT('Ctrl Pts',(53.0053510647738,20.8871353955393,15.4288471065411));
#27027=CARTESIAN_POINT('Ctrl Pts',(53.0147268740369,20.7762621275074,15.4366195681347));
#27028=CARTESIAN_POINT('Ctrl Pts',(53.0358535934502,20.6515856253841,15.4450663374528));
#27029=CARTESIAN_POINT('Ctrl Pts',(53.0385958981777,20.6364650443494,15.4460855343218));
#27030=CARTESIAN_POINT('Ctrl Pts',(53.0430393883581,20.6134803797667,15.447625344939));
#27031=CARTESIAN_POINT('Ctrl Pts',(53.044613804336,20.6055927444684,15.4481520552864));
#27032=CARTESIAN_POINT('Ctrl Pts',(53.0472783225556,20.5926520778961,15.4490131476044));
#27033=CARTESIAN_POINT('Ctrl Pts',(53.0483404165262,20.5875934640958,15.4493489897642));
#27034=CARTESIAN_POINT('Ctrl Pts',(53.0504417930872,20.5777748266234,15.4499992860299));
#27035=CARTESIAN_POINT('Ctrl Pts',(53.0514788748356,20.5730143735494,15.4503138585225));
#27036=CARTESIAN_POINT('Ctrl Pts',(53.0534401713326,20.5641675232971,15.450897067657));
#27037=CARTESIAN_POINT('Ctrl Pts',(53.0543598103192,20.5600802719784,15.4511659489515));
#27038=CARTESIAN_POINT('Ctrl Pts',(53.0564891954052,20.5507537121437,15.4517782449666));
#27039=CARTESIAN_POINT('Ctrl Pts',(53.057707252214,20.5455163828505,15.4521211807054));
#27040=CARTESIAN_POINT('Ctrl Pts',(53.0609480313193,20.531832879904,15.4530149642999));
#27041=CARTESIAN_POINT('Ctrl Pts',(53.0630047877747,20.5233947714788,15.4535639306557));
#27042=CARTESIAN_POINT('Ctrl Pts',(53.0775106488955,20.4655279175796,15.4573152138641));
#27043=CARTESIAN_POINT('Ctrl Pts',(53.0917964143046,20.4165741158235,15.4604214481491));
#27044=CARTESIAN_POINT('Ctrl Pts',(53.1265071875482,20.3126226641734,15.4669770490478));
#27045=CARTESIAN_POINT('Ctrl Pts',(53.1475131868166,20.2578704837039,15.4704052142044));
#27046=CARTESIAN_POINT('Ctrl Pts',(53.199646474455,20.1380571884916,15.4780054269643));
#27047=CARTESIAN_POINT('Ctrl Pts',(53.2319496750776,20.0736004266553,15.482163236072));
#27048=CARTESIAN_POINT('Ctrl Pts',(53.3095873765614,19.9376058068315,15.4913240550353));
#27049=CARTESIAN_POINT('Ctrl Pts',(53.3561278307007,19.8669252611186,15.4963407569303));
#27050=CARTESIAN_POINT('Ctrl Pts',(53.424769591956,19.7758482276004,15.5033274168221));
#27051=CARTESIAN_POINT('Ctrl Pts',(53.4430508267868,19.7526798599785,15.5051535362483));
#27052=CARTESIAN_POINT('Ctrl Pts',(53.4673484216776,19.7232535144209,15.5075414701357));
#27053=CARTESIAN_POINT('Ctrl Pts',(53.4729015951414,19.7166166172613,15.5080846876073));
#27054=CARTESIAN_POINT('Ctrl Pts',(53.4839058463224,19.7036373901723,15.5091563130192));
#27055=CARTESIAN_POINT('Ctrl Pts',(53.4893539751192,19.6972927869107,15.5096845944947));
#27056=CARTESIAN_POINT('Ctrl Pts',(53.4997573297919,19.6853306111869,15.5106891903622));
#27057=CARTESIAN_POINT('Ctrl Pts',(53.5047046289526,19.6797063121373,15.5111651711632));
#27058=CARTESIAN_POINT('Ctrl Pts',(53.5160128131169,19.6669957742144,15.5122492577886));
#27059=CARTESIAN_POINT('Ctrl Pts',(53.5223929602089,19.6599269917066,15.5128581656974));
#27060=CARTESIAN_POINT('Ctrl Pts',(53.5390432124855,19.6417430860713,15.5144403536542));
#27061=CARTESIAN_POINT('Ctrl Pts',(53.5493894799272,19.63069883615,15.515416853504));
#27062=CARTESIAN_POINT('Ctrl Pts',(53.6251179301101,19.5516831335772,15.52251811737));
#27063=CARTESIAN_POINT('Ctrl Pts',(53.6951126523438,19.4883165584853,15.5288455890199));
#27064=CARTESIAN_POINT('Ctrl Pts',(53.8796696204105,19.3436337221625,15.5449443628457));
#27065=CARTESIAN_POINT('Ctrl Pts',(53.9988289071187,19.2690051793327,15.5548666078106));
#27066=CARTESIAN_POINT('Ctrl Pts',(54.1559900269391,19.1922728174744,15.5668354460668));
#27067=CARTESIAN_POINT('Ctrl Pts',(54.1875491778496,19.1778709304201,15.5691849132651));
#27068=CARTESIAN_POINT('Ctrl Pts',(54.2325937796785,19.1587182072989,15.5724480395552));
#27069=CARTESIAN_POINT('Ctrl Pts',(54.2457778625774,19.1532785969797,15.5733924161728));
#27070=CARTESIAN_POINT('Ctrl Pts',(54.26886377943,19.1440420773241,15.5750260999898));
#27071=CARTESIAN_POINT('Ctrl Pts',(54.2787395059834,19.140181918746,15.5757186584927));
#27072=CARTESIAN_POINT('Ctrl Pts',(54.2936749708942,19.1344809050779,15.5767560703827));
#27073=CARTESIAN_POINT('Ctrl Pts',(54.2987119649171,19.1325815590081,15.5771042384922));
#27074=CARTESIAN_POINT('Ctrl Pts',(54.3076475988664,19.1292533696836,15.577718804945));
#27075=CARTESIAN_POINT('Ctrl Pts',(54.3115430694272,19.1278162862421,15.5779856856377));
#27076=CARTESIAN_POINT('Ctrl Pts',(54.3200012351053,19.1247259420911,15.5785628963511));
#27077=CARTESIAN_POINT('Ctrl Pts',(54.3245654795197,19.1230771666686,15.5788729602611));
#27078=CARTESIAN_POINT('Ctrl Pts',(54.3370865803329,19.1186056664744,15.5797198085754));
#27079=CARTESIAN_POINT('Ctrl Pts',(54.3450555206016,19.1158167352598,15.5802546396508));
#27080=CARTESIAN_POINT('Ctrl Pts',(54.3854046404801,19.1019824655199,15.5829429356349));
#27081=CARTESIAN_POINT('Ctrl Pts',(54.4180495829951,19.0917201314812,15.5850540264259));
#27082=CARTESIAN_POINT('Ctrl Pts',(54.6467879518315,19.0262301317743,15.5995096514263));
#27083=CARTESIAN_POINT('Ctrl Pts',(54.8500772925075,19.0004829399303,15.6107753321542));
#27084=CARTESIAN_POINT('Ctrl Pts',(55.0898157958883,19.0069466924209,15.6251774586414));
#27085=CARTESIAN_POINT('Ctrl Pts',(55.1258346128224,19.0088963392613,15.627366717883));
#27086=CARTESIAN_POINT('Ctrl Pts',(55.1873749884919,19.0139039163861,15.6311640848457));
#27087=CARTESIAN_POINT('Ctrl Pts',(55.2129271045245,19.016480654527,15.6327576236345));
#27088=CARTESIAN_POINT('Ctrl Pts',(55.2489789875215,19.0208208512984,15.6350328265464));
#27089=CARTESIAN_POINT('Ctrl Pts',(55.259525994957,19.0221762237738,15.6357016962004));
#27090=CARTESIAN_POINT('Ctrl Pts',(55.2776517809216,19.0246530079171,15.636857015901));
#27091=CARTESIAN_POINT('Ctrl Pts',(55.2852359360596,19.0257338809846,15.6373421796931));
#27092=CARTESIAN_POINT('Ctrl Pts',(55.2997195491981,19.0278832446124,15.6382721448998));
#27093=CARTESIAN_POINT('Ctrl Pts',(55.3066200054796,19.0289443246694,15.6387167053303));
#27094=CARTESIAN_POINT('Ctrl Pts',(55.3245121673585,19.0317918240676,15.6398733577671));
#27095=CARTESIAN_POINT('Ctrl Pts',(55.3354946183994,19.0336340820527,15.6405872072601));
#27096=CARTESIAN_POINT('Ctrl Pts',(55.366969499728,19.0391852114591,15.6426444666741));
#27097=CARTESIAN_POINT('Ctrl Pts',(55.3874195375099,19.0431230758806,15.6439950729244));
#27098=CARTESIAN_POINT('Ctrl Pts',(55.5695746424837,19.0811660688116,15.656154097486));
#27099=CARTESIAN_POINT('Ctrl Pts',(55.726490755741,19.1349185502859,15.66761913074));
#27100=CARTESIAN_POINT('Ctrl Pts',(55.9643466985291,19.2510120140521,15.6860743573232));
#27101=CARTESIAN_POINT('Ctrl Pts',(56.0503650492637,19.3012767270346,15.6929849056846));
#27102=CARTESIAN_POINT('Ctrl Pts',(56.1463660861621,19.3674666680496,15.7007189508597));
#27103=CARTESIAN_POINT('Ctrl Pts',(56.1603267673647,19.3773595211226,15.7018440168585));
#27104=CARTESIAN_POINT('Ctrl Pts',(56.1793102119633,19.3911819276813,15.7033724649419));
#27105=CARTESIAN_POINT('Ctrl Pts',(56.1844435239027,19.3949574126409,15.7037856299161));
#27106=CARTESIAN_POINT('Ctrl Pts',(56.1930497245641,19.4013509359045,15.7044779539706));
#27107=CARTESIAN_POINT('Ctrl Pts',(56.1965322703681,19.403955826883,15.7047580055549));
#27108=CARTESIAN_POINT('Ctrl Pts',(56.2031360869384,19.4089291437047,15.7052888202313));
#27109=CARTESIAN_POINT('Ctrl Pts',(56.2062589321402,19.4112954010498,15.7055397353665));
#27110=CARTESIAN_POINT('Ctrl Pts',(56.2144500535848,19.4175400925288,15.7061976760657));
#27111=CARTESIAN_POINT('Ctrl Pts',(56.2195067747011,19.4214337136054,15.7066036464607));
#27112=CARTESIAN_POINT('Ctrl Pts',(56.2371288197154,19.4351377148775,15.7080180300434));
#27113=CARTESIAN_POINT('Ctrl Pts',(56.2495955400678,19.4450746924914,15.7090179690062));
#27114=CARTESIAN_POINT('Ctrl Pts',(56.3425424270726,19.5210007662374,15.7164795315619));
#27115=CARTESIAN_POINT('Ctrl Pts',(56.4178772283359,19.5930569827258,15.7225686810504));
#27116=CARTESIAN_POINT('Ctrl Pts',(56.5459493232423,19.736344009908,15.733737998096));
#27117=CARTESIAN_POINT('Ctrl Pts',(56.6002325990108,19.8058304624465,15.7388172137825));
#27118=CARTESIAN_POINT('Ctrl Pts',(56.693438013054,19.9429584678914,15.7485954786565));
#27119=CARTESIAN_POINT('Ctrl Pts',(56.7333325504978,20.0097346900497,15.7532599707987));
#27120=CARTESIAN_POINT('Ctrl Pts',(56.7786199567316,20.096699307806,15.7593239639879));
#27121=CARTESIAN_POINT('Ctrl Pts',(56.7877358534907,20.1148776572217,15.7605907246089));
#27122=CARTESIAN_POINT('Ctrl Pts',(56.8007815396024,20.1419165237639,15.7624752277464));
#27123=CARTESIAN_POINT('Ctrl Pts',(56.8049274160698,20.1506717813744,15.763085476846));
#27124=CARTESIAN_POINT('Ctrl Pts',(56.8121738857521,20.1662675657669,15.7641727507067));
#27125=CARTESIAN_POINT('Ctrl Pts',(56.8152999499695,20.1730961040024,15.7646488870201));
#27126=CARTESIAN_POINT('Ctrl Pts',(56.821788261661,20.187483214042,15.7656523060847));
#27127=CARTESIAN_POINT('Ctrl Pts',(56.8251421917617,20.1950453588913,15.7661798627511));
#27128=CARTESIAN_POINT('Ctrl Pts',(56.8338631098235,20.2150432450993,15.7675754555429));
#27129=CARTESIAN_POINT('Ctrl Pts',(56.8391505714553,20.2275129948412,15.7684461747148));
#27130=CARTESIAN_POINT('Ctrl Pts',(56.8611862392841,20.2809899762186,15.7721830428967));
#27131=CARTESIAN_POINT('Ctrl Pts',(56.8766919126076,20.3224923753097,15.7750904201147));
#27132=CARTESIAN_POINT('Ctrl Pts',(56.9008850360456,20.3944711901988,15.7801485536937));
#27133=CARTESIAN_POINT('Ctrl Pts',(56.9102518419404,20.4247028664337,15.7822775480933));
#27134=CARTESIAN_POINT('Ctrl Pts',(56.9637764852852,20.6132078173788,15.7955749725531));
#27135=CARTESIAN_POINT('Ctrl Pts',(56.9889509824335,20.7761897219217,15.8072399424666));
#27136=CARTESIAN_POINT('Ctrl Pts',(56.9954095805707,20.9922599737663,15.8220352273783));
#27137=CARTESIAN_POINT('Ctrl Pts',(56.9949360426966,21.0441647537622,15.8255325184685));
#27138=CARTESIAN_POINT('Ctrl Pts',(56.9919973395273,21.1051584314049,15.8295323510324));
#27139=CARTESIAN_POINT('Ctrl Pts',(56.991492720431,21.1143173155307,15.8301300373187));
#27140=CARTESIAN_POINT('Ctrl Pts',(56.9906178405321,21.1284242523775,15.8310457664564));
#27141=CARTESIAN_POINT('Ctrl Pts',(56.9902922745852,21.133374805227,15.8313662015449));
#27142=CARTESIAN_POINT('Ctrl Pts',(56.9896583126334,21.1424950594003,15.8319547660829));
#27143=CARTESIAN_POINT('Ctrl Pts',(56.9893552788833,21.1466649854575,15.8322231806606));
#27144=CARTESIAN_POINT('Ctrl Pts',(56.9886415322621,21.1560771170274,15.8328275010635));
#27145=CARTESIAN_POINT('Ctrl Pts',(56.9882232021661,21.1613186604016,15.8331629779209));
#27146=CARTESIAN_POINT('Ctrl Pts',(56.9869268873471,21.1767894595909,15.8341501801768));
#27147=CARTESIAN_POINT('Ctrl Pts',(56.985990634628,21.1870138456729,15.834798753373));
#27148=CARTESIAN_POINT('Ctrl Pts',(56.9778388503983,21.2690552478096,15.8399752858079));
#27149=CARTESIAN_POINT('Ctrl Pts',(56.9668082552577,21.3404482004662,15.8443102160548));
#27150=CARTESIAN_POINT('Ctrl Pts',(56.9273018802228,21.5280300268974,15.8556123745615));
#27151=CARTESIAN_POINT('Ctrl Pts',(56.8922156163492,21.642518338818,15.8624316182027));
#27152=CARTESIAN_POINT('Ctrl Pts',(56.8235955137034,21.8108016259018,15.8731077873845));
#27153=CARTESIAN_POINT('Ctrl Pts',(56.7974176398596,21.8672881821525,15.8768088409536));
#27154=CARTESIAN_POINT('Ctrl Pts',(56.7568188653363,21.9451290613063,15.8821466575709));
#27155=CARTESIAN_POINT('Ctrl Pts',(56.7445590247577,21.9675718010639,15.8837145451998));
#27156=CARTESIAN_POINT('Ctrl Pts',(56.7221218777678,22.0068316089218,15.8865133001155));
#27157=CARTESIAN_POINT('Ctrl Pts',(56.7121209576025,22.0237457859437,15.8877379710291));
#27158=CARTESIAN_POINT('Ctrl Pts',(56.6968880429045,22.0486609687559,15.8895716007625));
#27159=CARTESIAN_POINT('Ctrl Pts',(56.6918455731269,22.0567768965679,15.8901736480195));
#27160=CARTESIAN_POINT('Ctrl Pts',(56.682744427713,22.0711932210145,15.8912517426868));
#27161=CARTESIAN_POINT('Ctrl Pts',(56.6787081609313,22.077507602602,15.8917269558936));
#27162=CARTESIAN_POINT('Ctrl Pts',(56.6701028680966,22.0908041057353,15.8927340874224));
#27163=CARTESIAN_POINT('Ctrl Pts',(56.6655254325671,22.0977805869562,15.8932663131576));
#27164=CARTESIAN_POINT('Ctrl Pts',(56.6532233680654,22.1162761371856,15.8946875839482));
#27165=CARTESIAN_POINT('Ctrl Pts',(56.6454222554634,22.1277435454362,15.8955794922305));
#27166=CARTESIAN_POINT('Ctrl Pts',(56.6104754159754,22.1779797876132,15.8995350519953));
#27167=CARTESIAN_POINT('Ctrl Pts',(56.5820764511271,22.2158539887533,15.9026461518083));
#27168=CARTESIAN_POINT('Ctrl Pts',(56.5322868832193,22.277554746381,15.9079395564349));
#27169=CARTESIAN_POINT('Ctrl Pts',(56.5116201375564,22.3019422460328,15.910094705495));
#27170=CARTESIAN_POINT('Ctrl Pts',(56.3835366004,22.4459229836597,15.9231987164374));
#27171=CARTESIAN_POINT('Ctrl Pts',(56.2625848720434,22.5526552544748,15.9346065389171));
#27172=CARTESIAN_POINT('Ctrl Pts',(56.1016783652932,22.6632876981583,15.947968312459));
#27173=CARTESIAN_POINT('Ctrl Pts',(56.0727039430594,22.6821200072393,15.9503084949259));
#27174=CARTESIAN_POINT('Ctrl Pts',(56.0252272170605,22.7112521738022,15.9540216769226));
#27175=CARTESIAN_POINT('Ctrl Pts',(56.0070254402028,22.7220263350432,15.9554174729121));
#27176=CARTESIAN_POINT('Ctrl Pts',(55.9826532764748,22.7359342871923,15.9572464948717));
#27177=CARTESIAN_POINT('Ctrl Pts',(55.9766338002893,22.7393279549175,15.957695044553));
#27178=CARTESIAN_POINT('Ctrl Pts',(55.9666969727923,22.7448623013406,15.9584301207717));
#27179=CARTESIAN_POINT('Ctrl Pts',(55.9627899149645,22.7470211986254,15.958717785127));
#27180=CARTESIAN_POINT('Ctrl Pts',(55.955118585176,22.7512265437838,15.9592798909439));
#27181=CARTESIAN_POINT('Ctrl Pts',(55.9513549238789,22.7532740027557,15.9595543932637));
#27182=CARTESIAN_POINT('Ctrl Pts',(55.9420710718735,22.7582857893503,15.9602284482935));
#27183=CARTESIAN_POINT('Ctrl Pts',(55.9365433956169,22.7612362965137,15.9606271316407));
#27184=CARTESIAN_POINT('Ctrl Pts',(55.9175182367484,22.7712764572299,15.9619905488729));
#27185=CARTESIAN_POINT('Ctrl Pts',(55.9039530359682,22.7782375951068,15.962947596788));
#27186=CARTESIAN_POINT('Ctrl Pts',(55.7722955602515,22.8439031476453,15.9721043985158));
#27187=CARTESIAN_POINT('Ctrl Pts',(55.648718233845,22.8909241010592,15.9796968742609));
#27188=CARTESIAN_POINT('Ctrl Pts',(55.4045043574775,22.9570558279542,15.9943773613061));
#27189=CARTESIAN_POINT('Ctrl Pts',(55.2850325860818,22.9779848502632,16.0014269554212));
#27190=CARTESIAN_POINT('Ctrl Pts',(55.1644482585673,22.9879598418364,16.0088160704683));
#27191=CARTESIAN_POINT('Origin',(55.,21.,6.22095488139522));
#27192=CARTESIAN_POINT('',(55.164448352281,22.9879598340842,16.9667227887628));
#27193=CARTESIAN_POINT('',(55.1644482145651,22.9879598454763,16.809768216174));
#27194=CARTESIAN_POINT('',(55.1644483516311,22.987959834138,6.22095488139522));
#27195=CARTESIAN_POINT('',(53.0052503038905,21.0011010772302,16.3790451185582));
#27196=CARTESIAN_POINT('Ctrl Pts',(55.164448352281,22.9879598340842,16.9667227887628));
#27197=CARTESIAN_POINT('Ctrl Pts',(55.1692009938859,22.9875666852552,16.9664083972774));
#27198=CARTESIAN_POINT('Ctrl Pts',(55.1739524101488,22.9871564778586,16.9660947938768));
#27199=CARTESIAN_POINT('Ctrl Pts',(55.1875134282772,22.9859366901065,16.9652018433256));
#27200=CARTESIAN_POINT('Ctrl Pts',(55.1963191738424,22.9850855426879,16.9646245499614));
#27201=CARTESIAN_POINT('Ctrl Pts',(55.2105165670934,22.9836178515125,16.9636981958022));
#27202=CARTESIAN_POINT('Ctrl Pts',(55.2159117548901,22.9830378517935,16.9633471983118));
#27203=CARTESIAN_POINT('Ctrl Pts',(55.225473779728,22.9819704175264,16.9627270217624));
#27204=CARTESIAN_POINT('Ctrl Pts',(55.2296415139441,22.9814918464494,16.9624573560035));
#27205=CARTESIAN_POINT('Ctrl Pts',(55.238615882347,22.9804326453078,16.9618780937649));
#27206=CARTESIAN_POINT('Ctrl Pts',(55.2434219164473,22.9798476642679,16.9615687434008));
#27207=CARTESIAN_POINT('Ctrl Pts',(55.2567731786842,22.978173223809,16.9607116378098));
#27208=CARTESIAN_POINT('Ctrl Pts',(55.2653136733424,22.9770458846017,16.9601659608864));
#27209=CARTESIAN_POINT('Ctrl Pts',(55.3144452030712,22.9702364501159,16.9570403652911));
#27210=CARTESIAN_POINT('Ctrl Pts',(55.3548639020246,22.9633592665141,16.9545223625556));
#27211=CARTESIAN_POINT('Ctrl Pts',(55.4901309344792,22.9360293465946,16.9461892884863));
#27212=CARTESIAN_POINT('Ctrl Pts',(55.5836963506633,22.9099056232083,16.9405775967386));
#27213=CARTESIAN_POINT('Ctrl Pts',(55.8040647442482,22.83066124531,16.9269913086181));
#27214=CARTESIAN_POINT('Ctrl Pts',(55.9279867779923,22.7710661630308,16.9190152345749));
#27215=CARTESIAN_POINT('Ctrl Pts',(56.0653447613261,22.6866087935056,16.9090877407181));
#27216=CARTESIAN_POINT('Ctrl Pts',(56.0856486198404,22.6736115675758,16.9075910366386));
#27217=CARTESIAN_POINT('Ctrl Pts',(56.1137002628937,22.6549294302224,16.9054794049525));
#27218=CARTESIAN_POINT('Ctrl Pts',(56.1216506054828,22.6495513355606,16.9048759086679));
#27219=CARTESIAN_POINT('Ctrl Pts',(56.1353649035642,22.6401291629907,16.9038259767214));
#27220=CARTESIAN_POINT('Ctrl Pts',(56.1411468822823,22.6361115263113,16.9033805457489));
#27221=CARTESIAN_POINT('Ctrl Pts',(56.153138781588,22.6276844038495,16.9024508471324));
#27222=CARTESIAN_POINT('Ctrl Pts',(56.159344950756,22.6232698021744,16.9019663887765));
#27223=CARTESIAN_POINT('Ctrl Pts',(56.1739440513228,22.6127586720863,16.9008188336992));
#27224=CARTESIAN_POINT('Ctrl Pts',(56.1823149433281,22.6066320481306,16.9001545828806));
#27225=CARTESIAN_POINT('Ctrl Pts',(56.2099860704517,22.5860462890327,16.8979376195425));
#27226=CARTESIAN_POINT('Ctrl Pts',(56.2290712406905,22.5713029378016,16.8963738688555));
#27227=CARTESIAN_POINT('Ctrl Pts',(56.2738118004669,22.5354268408576,16.8926228891196));
#27228=CARTESIAN_POINT('Ctrl Pts',(56.2992148486119,22.5139922888557,16.8904240795533));
#27229=CARTESIAN_POINT('Ctrl Pts',(56.4508703444832,22.3794002869036,16.8768655771366));
#27230=CARTESIAN_POINT('Ctrl Pts',(56.5627958792803,22.2511685191208,16.8648934034886));
#27231=CARTESIAN_POINT('Ctrl Pts',(56.6962548256279,22.0519908726685,16.8483220833582));
#27232=CARTESIAN_POINT('Ctrl Pts',(56.7322621149789,21.991582272053,16.8435328520369));
#27233=CARTESIAN_POINT('Ctrl Pts',(56.7697706705476,21.9203498178749,16.8382480931461));
#27234=CARTESIAN_POINT('Ctrl Pts',(56.7744629825528,21.9112700740082,16.8375809970704));
#27235=CARTESIAN_POINT('Ctrl Pts',(56.7814593753626,21.8974729014788,16.8365776088219));
#27236=CARTESIAN_POINT('Ctrl Pts',(56.783814876006,21.8927819468527,16.8362382510271));
#27237=CARTESIAN_POINT('Ctrl Pts',(56.788013564466,21.88433734614,16.8356306229828));
#27238=CARTESIAN_POINT('Ctrl Pts',(56.7898634820035,21.880587170739,16.8353619418176));
#27239=CARTESIAN_POINT('Ctrl Pts',(56.7938869304648,21.8723657250095,16.8347754585405));
#27240=CARTESIAN_POINT('Ctrl Pts',(56.7960555401853,21.8678921449888,16.8344579613945));
#27241=CARTESIAN_POINT('Ctrl Pts',(56.8021966100727,21.8551022632328,16.83355475198));
#27242=CARTESIAN_POINT('Ctrl Pts',(56.8061282537045,21.8467663437419,16.8329714971264));
#27243=CARTESIAN_POINT('Ctrl Pts',(56.832217227101,21.7904436923842,16.82906506185));
#27244=CARTESIAN_POINT('Ctrl Pts',(56.8525196391284,21.7416153109182,16.8258456744038));
#27245=CARTESIAN_POINT('Ctrl Pts',(56.9311791830559,21.5289652230822,16.8122949692424));
#27246=CARTESIAN_POINT('Ctrl Pts',(56.9699222991364,21.3587072633161,16.8025473092958));
#27247=CARTESIAN_POINT('Ctrl Pts',(56.9918956429076,21.1235369204037,16.7884454381991));
#27248=CARTESIAN_POINT('Ctrl Pts',(56.9947818396309,21.0612688575145,16.7846604075312));
#27249=CARTESIAN_POINT('Ctrl Pts',(56.994742004622,20.983971465127,16.7798503057266));
#27250=CARTESIAN_POINT('Ctrl Pts',(56.9945650682515,20.9689718180639,16.7789117796303));
#27251=CARTESIAN_POINT('Ctrl Pts',(56.9940186576918,20.9452959064464,16.7774217045518));
#27252=CARTESIAN_POINT('Ctrl Pts',(56.9937616681672,20.9366174174814,16.7768736719055));
#27253=CARTESIAN_POINT('Ctrl Pts',(56.9931786696285,20.9204892840428,16.7758516686435));
#27254=CARTESIAN_POINT('Ctrl Pts',(56.9928675281707,20.913039228937,16.7753781715842));
#27255=CARTESIAN_POINT('Ctrl Pts',(56.9920853600501,20.8965314350179,16.7743258091181));
#27256=CARTESIAN_POINT('Ctrl Pts',(56.991594314281,20.8874748539177,16.7737463267742));
#27257=CARTESIAN_POINT('Ctrl Pts',(56.9899911584643,20.8612205040897,16.7720601110615));
#27258=CARTESIAN_POINT('Ctrl Pts',(56.9887179430646,20.8440337496564,16.7709483688317));
#27259=CARTESIAN_POINT('Ctrl Pts',(56.9742301474694,20.6777435705585,16.7601123378514));
#27260=CARTESIAN_POINT('Ctrl Pts',(56.9444969341449,20.5305870650988,16.749849142564));
#27261=CARTESIAN_POINT('Ctrl Pts',(56.8599975006504,20.2683728634241,16.7306477137786));
#27262=CARTESIAN_POINT('Ctrl Pts',(56.8101381590583,20.1524893418869,16.7218164502821));
#27263=CARTESIAN_POINT('Ctrl Pts',(56.7422183842659,20.0284319769945,16.7124517881987));
#27264=CARTESIAN_POINT('Ctrl Pts',(56.7345920591683,20.0148808468637,16.7114304245822));
#27265=CARTESIAN_POINT('Ctrl Pts',(56.7236453030853,19.9959510269611,16.7100073399107));
#27266=CARTESIAN_POINT('Ctrl Pts',(56.7204568096393,19.9904972313567,16.7095977753863));
#27267=CARTESIAN_POINT('Ctrl Pts',(56.7152544960523,19.9816951139194,16.7089375820725));
#27268=CARTESIAN_POINT('Ctrl Pts',(56.7132566850449,19.978337453443,16.7086859388631));
#27269=CARTESIAN_POINT('Ctrl Pts',(56.7090062536041,19.9712414098123,16.7081545671353));
#27270=CARTESIAN_POINT('Ctrl Pts',(56.706751203372,19.9675045074013,16.7078750038496));
#27271=CARTESIAN_POINT('Ctrl Pts',(56.7011366164711,19.9582690875789,16.7071846723091));
#27272=CARTESIAN_POINT('Ctrl Pts',(56.697762633779,19.9527793337171,16.7067748377424));
#27273=CARTESIAN_POINT('Ctrl Pts',(56.6850753347306,19.9323585117788,16.7052518831588));
#27274=CARTESIAN_POINT('Ctrl Pts',(56.6755908484767,19.9175340236898,16.7041494032243));
#27275=CARTESIAN_POINT('Ctrl Pts',(56.6511350026874,19.8804007616584,16.7013905816269));
#27276=CARTESIAN_POINT('Ctrl Pts',(56.6359065034463,19.8582647826906,16.6997485210992));
#27277=CARTESIAN_POINT('Ctrl Pts',(56.5172455584056,19.6930314137088,16.6874562583192));
#27278=CARTESIAN_POINT('Ctrl Pts',(56.3956665757374,19.5639194193307,16.6775814557249));
#27279=CARTESIAN_POINT('Ctrl Pts',(56.2368861875563,19.4347752909524,16.6654349612381));
#27280=CARTESIAN_POINT('Ctrl Pts',(56.2147340674437,19.4175219162812,16.6637567420029));
#27281=CARTESIAN_POINT('Ctrl Pts',(56.1540501191195,19.372282822589,16.6591911215947));
#27282=CARTESIAN_POINT('Ctrl Pts',(56.114870265604,19.3452013337919,16.6562763333413));
#27283=CARTESIAN_POINT('Ctrl Pts',(56.0630498502284,19.3120586974552,16.6524418759761));
#27284=CARTESIAN_POINT('Ctrl Pts',(56.0512606494066,19.30469122092,16.6515709118317));
#27285=CARTESIAN_POINT('Ctrl Pts',(56.0322663016953,19.2930953114743,16.6501693698176));
#27286=CARTESIAN_POINT('Ctrl Pts',(56.0251097901661,19.2887877840569,16.6496416974955));
#27287=CARTESIAN_POINT('Ctrl Pts',(56.0114806703002,19.2807005512516,16.6486374075272));
#27288=CARTESIAN_POINT('Ctrl Pts',(56.005013385158,19.2769121223814,16.6481611179534));
#27289=CARTESIAN_POINT('Ctrl Pts',(55.9902604337306,19.2683813999167,16.6470751445737));
#27290=CARTESIAN_POINT('Ctrl Pts',(55.9819618142033,19.2636619876952,16.6464646494043));
#27291=CARTESIAN_POINT('Ctrl Pts',(55.9565240021682,19.249436229654,16.6445942311671));
#27292=CARTESIAN_POINT('Ctrl Pts',(55.9392787230937,19.2401229828121,16.6433274772234));
#27293=CARTESIAN_POINT('Ctrl Pts',(55.7994760401723,19.1672632845178,16.6330652475449));
#27294=CARTESIAN_POINT('Ctrl Pts',(55.6707831660314,19.1163539614051,16.6236218065157));
#27295=CARTESIAN_POINT('Ctrl Pts',(55.4086661765892,19.042954192605,16.6046687614064));
#27296=CARTESIAN_POINT('Ctrl Pts',(55.2761091690908,19.0198975414158,16.5952240105739));
#27297=CARTESIAN_POINT('Ctrl Pts',(55.1271090824598,19.0092461877652,16.5853385427881));
#27298=CARTESIAN_POINT('Ctrl Pts',(55.1119729223528,19.0083374889978,16.5843429435877));
#27299=CARTESIAN_POINT('Ctrl Pts',(55.0912016265966,19.0073280377456,16.5829898176994));
#27300=CARTESIAN_POINT('Ctrl Pts',(55.0855747022773,19.0070784616458,16.5826245776483));
#27301=CARTESIAN_POINT('Ctrl Pts',(55.0759581087713,19.0066927324711,16.5820027127483));
#27302=CARTESIAN_POINT('Ctrl Pts',(55.0719689887494,19.0065447177287,16.5817454413407));
#27303=CARTESIAN_POINT('Ctrl Pts',(55.0636967529413,19.0062626430168,16.5812134022792));
#27304=CARTESIAN_POINT('Ctrl Pts',(55.0594136292264,19.0061304089862,16.5809387470931));
#27305=CARTESIAN_POINT('Ctrl Pts',(55.0490936678046,19.0058450811369,16.5802788886029));
#27306=CARTESIAN_POINT('Ctrl Pts',(55.043056432992,19.0057055948272,16.5798944391587));
#27307=CARTESIAN_POINT('Ctrl Pts',(55.0220921888015,19.0053164734428,16.578564609522));
#27308=CARTESIAN_POINT('Ctrl Pts',(55.0071626477137,19.0052069872387,16.5776266750933));
#27309=CARTESIAN_POINT('Ctrl Pts',(54.917293458193,19.0055569260401,16.5720279247323));
#27310=CARTESIAN_POINT('Ctrl Pts',(54.8424214330629,19.0100716007706,16.5675600042198));
#27311=CARTESIAN_POINT('Ctrl Pts',(54.7379279784377,19.0223091880352,16.5613862278743));
#27312=CARTESIAN_POINT('Ctrl Pts',(54.7079656367682,19.0265110379746,16.559623328537));
#27313=CARTESIAN_POINT('Ctrl Pts',(54.5182033169,19.057539366651,16.5484468153891));
#27314=CARTESIAN_POINT('Ctrl Pts',(54.3620974008528,19.1030668153155,16.5391392346602));
#27315=CARTESIAN_POINT('Ctrl Pts',(54.1921499278254,19.1760121731134,16.5277389116158));
#27316=CARTESIAN_POINT('Ctrl Pts',(54.1712374394313,19.1854185378954,16.5263140528486));
#27317=CARTESIAN_POINT('Ctrl Pts',(54.1419890983342,19.1991854120023,16.5242878696667));
#27318=CARTESIAN_POINT('Ctrl Pts',(54.1335143178166,19.2032478063324,16.5236967738899));
#27319=CARTESIAN_POINT('Ctrl Pts',(54.1187861915353,19.210436182173,16.5226623690225));
#27320=CARTESIAN_POINT('Ctrl Pts',(54.1125199362212,19.2135354555224,16.5222199918878));
#27321=CARTESIAN_POINT('Ctrl Pts',(54.0995617657419,19.2200295355763,16.5213003891382));
#27322=CARTESIAN_POINT('Ctrl Pts',(54.0928724652831,19.2234292861906,16.5208229959894));
#27323=CARTESIAN_POINT('Ctrl Pts',(54.0770816103596,19.2315672204121,16.5196896267859));
#27324=CARTESIAN_POINT('Ctrl Pts',(54.0679971897672,19.2363380128089,16.5190325107134));
#27325=CARTESIAN_POINT('Ctrl Pts',(54.048796528662,19.2466112446011,16.517632631883));
#27326=CARTESIAN_POINT('Ctrl Pts',(54.0386903527454,19.2521316055534,16.5168892502653));
#27327=CARTESIAN_POINT('Ctrl Pts',(54.0112721417145,19.2674181523139,16.5148542450719));
#27328=CARTESIAN_POINT('Ctrl Pts',(53.9940577480851,19.2773558767347,16.5135565783449));
#27329=CARTESIAN_POINT('Ctrl Pts',(53.9399395243347,19.3096856762955,16.5094122072797));
#27330=CARTESIAN_POINT('Ctrl Pts',(53.9036145453936,19.3330179339152,16.5065329230525));
#27331=CARTESIAN_POINT('Ctrl Pts',(53.7407008959973,19.4452898824258,16.4931670650648));
#27332=CARTESIAN_POINT('Ctrl Pts',(53.6239757863481,19.5475863994228,16.4822395871003));
#27333=CARTESIAN_POINT('Ctrl Pts',(53.5026158694608,19.6818344082034,16.4697438130851));
#27334=CARTESIAN_POINT('Ctrl Pts',(53.485359817934,19.7016991986294,16.4679370865997));
#27335=CARTESIAN_POINT('Ctrl Pts',(53.4407229885164,19.755185824174,16.4631938762394));
#27336=CARTESIAN_POINT('Ctrl Pts',(53.4140347933791,19.7893711831262,16.4602846732763));
#27337=CARTESIAN_POINT('Ctrl Pts',(53.3835952187077,19.8310980181733,16.4569013550973));
#27338=CARTESIAN_POINT('Ctrl Pts',(53.3787521612786,19.8378245781031,16.4563609742489));
#27339=CARTESIAN_POINT('Ctrl Pts',(53.3709054811579,19.8488674021876,16.4554822826097));
#27340=CARTESIAN_POINT('Ctrl Pts',(53.3678768066826,19.8531656211811,16.4551423361829));
#27341=CARTESIAN_POINT('Ctrl Pts',(53.3624697575195,19.8609039735684,16.4545340864696));
#27342=CARTESIAN_POINT('Ctrl Pts',(53.3600851843463,19.8643396410598,16.4542653684119));
#27343=CARTESIAN_POINT('Ctrl Pts',(53.3548937345172,19.8718698744083,16.4536793087167));
#27344=CARTESIAN_POINT('Ctrl Pts',(53.3520913359052,19.8759674199143,16.4533622688072));
#27345=CARTESIAN_POINT('Ctrl Pts',(53.3441490531959,19.8876738267091,16.452461669025));
#27346=CARTESIAN_POINT('Ctrl Pts',(53.3390462886722,19.8953078934184,16.4518805443269));
#27347=CARTESIAN_POINT('Ctrl Pts',(53.3053656082326,19.9464573615876,16.4480260052497));
#27348=CARTESIAN_POINT('Ctrl Pts',(53.2784452242897,19.9910460821894,16.4448532469008));
#27349=CARTESIAN_POINT('Ctrl Pts',(53.1674216491063,20.1923470796031,16.4311052411632));
#27350=CARTESIAN_POINT('Ctrl Pts',(53.1027473074923,20.3588393303913,16.4211498793913));
#27351=CARTESIAN_POINT('Ctrl Pts',(53.0492599558051,20.5803090361699,16.4075228954763));
#27352=CARTESIAN_POINT('Ctrl Pts',(53.0393547499554,20.6293292144935,16.4044897790563));
#27353=CARTESIAN_POINT('Ctrl Pts',(53.0279513405126,20.6991940287121,16.4001139789896));
#27354=CARTESIAN_POINT('Ctrl Pts',(53.0249222454511,20.7197715922117,16.3988188233113));
#27355=CARTESIAN_POINT('Ctrl Pts',(53.0209567938934,20.7499818078036,16.396906556824));
#27356=CARTESIAN_POINT('Ctrl Pts',(53.0197678201504,20.7595803322233,16.3962973910627));
#27357=CARTESIAN_POINT('Ctrl Pts',(53.0177772108139,20.7766681747287,16.395209930527));
#27358=CARTESIAN_POINT('Ctrl Pts',(53.0169480952719,20.7841541504632,16.3947325093959));
#27359=CARTESIAN_POINT('Ctrl Pts',(53.0154314506239,20.7985947534022,16.393809520598));
#27360=CARTESIAN_POINT('Ctrl Pts',(53.0147380335559,20.8055486614254,16.3933641455118));
#27361=CARTESIAN_POINT('Ctrl Pts',(53.0133242675411,20.8205231379393,16.3924030695235));
#27362=CARTESIAN_POINT('Ctrl Pts',(53.0126159195606,20.8285446891409,16.3918869994485));
#27363=CARTESIAN_POINT('Ctrl Pts',(53.0110196869293,20.8479620823592,16.3906346898616));
#27364=CARTESIAN_POINT('Ctrl Pts',(53.0101811533913,20.8593615883424,16.3898969205667));
#27365=CARTESIAN_POINT('Ctrl Pts',(53.0066214187238,20.9141919281727,16.3863356068006));
#27366=CARTESIAN_POINT('Ctrl Pts',(53.005224130425,20.9576934333355,16.383471389899));
#27367=CARTESIAN_POINT('Ctrl Pts',(53.0052503625455,21.0012026534312,16.3805665413763));
#27368=CARTESIAN_POINT('Ctrl Pts',(55.1644483516311,22.987959834138,16.1684645359809));
#27369=CARTESIAN_POINT('Ctrl Pts',(55.0949564505043,22.9937083550063,16.1729106515113));
#27370=CARTESIAN_POINT('Ctrl Pts',(55.0252269405976,22.9958034934844,16.1773567670417));
#27371=CARTESIAN_POINT('Ctrl Pts',(54.9556709906544,22.9942573809392,16.1818028825721));
#27372=CARTESIAN_POINT('Ctrl Pts',(54.8859941619893,22.992708581462,16.1862567248428));
#27373=CARTESIAN_POINT('Ctrl Pts',(54.8164919833358,22.9875059359452,16.1907105671135));
#27374=CARTESIAN_POINT('Ctrl Pts',(54.7475705257622,22.978713451472,16.1951644093842));
#27375=CARTESIAN_POINT('Ctrl Pts',(54.7114345318024,22.9741034914247,16.1974995895017));
#27376=CARTESIAN_POINT('Ctrl Pts',(54.6754580112511,22.9685075475329,16.1998347696191));
#27377=CARTESIAN_POINT('Ctrl Pts',(54.639698020522,22.9619403778108,16.2021699497366));
#27378=CARTESIAN_POINT('Ctrl Pts',(54.5714823409985,22.9494128593185,16.2066245341835));
#27379=CARTESIAN_POINT('Ctrl Pts',(54.5037861158996,22.9332986294088,16.2110791186304));
#27380=CARTESIAN_POINT('Ctrl Pts',(54.4370150511099,22.9136550132726,16.2155337030772));
#27381=CARTESIAN_POINT('Ctrl Pts',(54.3703441575992,22.8940408668798,16.219981604668));
#27382=CARTESIAN_POINT('Ctrl Pts',(54.3045961353565,22.8709079803606,16.2244295062587));
#27383=CARTESIAN_POINT('Ctrl Pts',(54.240167082901,22.8443647959644,16.2288774078494));
#27384=CARTESIAN_POINT('Ctrl Pts',(54.1758137822046,22.8178528194291,16.2333200798681));
#27385=CARTESIAN_POINT('Ctrl Pts',(54.1127768216026,22.7879386942306,16.2377627518869));
#27386=CARTESIAN_POINT('Ctrl Pts',(54.0514359710254,22.7547802840913,16.2422054239056));
#27387=CARTESIAN_POINT('Ctrl Pts',(53.9901336881627,22.7216427221157,16.2466453026193));
#27388=CARTESIAN_POINT('Ctrl Pts',(53.9305258293109,22.6852651539973,16.2510851813329));
#27389=CARTESIAN_POINT('Ctrl Pts',(53.8729696481371,22.6458524078665,16.2555250600466));
#27390=CARTESIAN_POINT('Ctrl Pts',(53.8154301113842,22.6064510593356,16.2599636548112));
#27391=CARTESIAN_POINT('Ctrl Pts',(53.7599414780685,22.5640165516394,16.2644022495757));
#27392=CARTESIAN_POINT('Ctrl Pts',(53.706832450642,22.5187973043785,16.2688408443403));
#27393=CARTESIAN_POINT('Ctrl Pts',(53.6537207484914,22.4735757797456,16.2732796626453));
#27394=CARTESIAN_POINT('Ctrl Pts',(53.6029892612418,22.425569556217,16.2777184809502));
#27395=CARTESIAN_POINT('Ctrl Pts',(53.5549326198038,22.3750664817357,16.2821572992552));
#27396=CARTESIAN_POINT('Ctrl Pts',(53.5068251361222,22.3245099767703,16.2866008136745));
#27397=CARTESIAN_POINT('Ctrl Pts',(53.4613984845393,22.2714517037136,16.2910443280939));
#27398=CARTESIAN_POINT('Ctrl Pts',(53.4189088213326,22.2162147208615,16.2954878425132));
#27399=CARTESIAN_POINT('Ctrl Pts',(53.3763943093178,22.1609454343129,16.2999339555889));
#27400=CARTESIAN_POINT('Ctrl Pts',(53.3368204821056,22.103495305066,16.3043800686647));
#27401=CARTESIAN_POINT('Ctrl Pts',(53.3004001250256,22.0442163700532,16.3088261817404));
#27402=CARTESIAN_POINT('Ctrl Pts',(53.2639164660232,21.9848344028122,16.3132800225686));
#27403=CARTESIAN_POINT('Ctrl Pts',(53.2305974519699,21.9236177146054,16.3177338633969));
#27404=CARTESIAN_POINT('Ctrl Pts',(53.2006095188318,21.8609421924736,16.3221877042251));
#27405=CARTESIAN_POINT('Ctrl Pts',(53.1848641910595,21.8280340679049,16.3245262176319));
#27406=CARTESIAN_POINT('Ctrl Pts',(53.1700363772471,21.7947240924266,16.3268647310387));
#27407=CARTESIAN_POINT('Ctrl Pts',(53.1561446966371,21.7610684481441,16.3292032444456));
#27408=CARTESIAN_POINT('Ctrl Pts',(53.1265894763852,21.6894644423068,16.3341785444644));
#27409=CARTESIAN_POINT('Ctrl Pts',(53.1011757332561,21.6160560788944,16.3391538444832));
#27410=CARTESIAN_POINT('Ctrl Pts',(53.0801012621631,21.5413098917924,16.3441291445021));
#27411=CARTESIAN_POINT('Ctrl Pts',(53.0591002696496,21.4668243159117,16.3490870975623));
#27412=CARTESIAN_POINT('Ctrl Pts',(53.042408496276,21.3910104768948,16.3540450506225));
#27413=CARTESIAN_POINT('Ctrl Pts',(53.0301750919772,21.314352340906,16.3590030036827));
#27414=CARTESIAN_POINT('Ctrl Pts',(53.0180122992591,21.2381366780028,16.3639323392875));
#27415=CARTESIAN_POINT('Ctrl Pts',(53.0102566807941,21.1610867026744,16.3688616748924));
#27416=CARTESIAN_POINT('Ctrl Pts',(53.0070066496492,21.0836962840125,16.3737910104972));
#27417=CARTESIAN_POINT('Ctrl Pts',(53.0058519291347,21.0561998385727,16.3755423798508));
#27418=CARTESIAN_POINT('Ctrl Pts',(53.0052655163887,21.0286605665352,16.3772937492045));
#27419=CARTESIAN_POINT('Ctrl Pts',(53.0052503038905,21.0011010772302,16.3790451185582));
#27420=CARTESIAN_POINT('Ctrl Pts',(55.1644482585673,22.9879598418364,16.0088160704683));
#27421=CARTESIAN_POINT('Ctrl Pts',(55.1457889506031,22.989503379405,16.0099594675921));
#27422=CARTESIAN_POINT('Ctrl Pts',(55.1271029719689,22.9907846175602,16.0111105027836));
#27423=CARTESIAN_POINT('Ctrl Pts',(55.0885664790205,22.9928818093192,16.013498622497));
#27424=CARTESIAN_POINT('Ctrl Pts',(55.06872277886,22.9936647317237,16.0147361448708));
#27425=CARTESIAN_POINT('Ctrl Pts',(55.0392785788694,22.994386329206,16.0165853219081));
#27426=CARTESIAN_POINT('Ctrl Pts',(55.029684485984,22.9945521961065,16.0171898897632));
#27427=CARTESIAN_POINT('Ctrl Pts',(55.012591174321,22.9947243565124,16.0182707931545));
#27428=CARTESIAN_POINT('Ctrl Pts',(55.0050923645821,22.9947575946588,16.0187462778363));
#27429=CARTESIAN_POINT('Ctrl Pts',(54.9892722264279,22.9947385099822,16.019752208976));
#27430=CARTESIAN_POINT('Ctrl Pts',(54.9809510746703,22.9946764006515,16.0202829523085));
#27431=CARTESIAN_POINT('Ctrl Pts',(54.9588658666389,22.9943733478775,16.0216960681835));
#27432=CARTESIAN_POINT('Ctrl Pts',(54.9451036948436,22.9940419874137,16.0225812462238));
#27433=CARTESIAN_POINT('Ctrl Pts',(54.8850280974205,22.9919731292414,16.0264661235822));
#27434=CARTESIAN_POINT('Ctrl Pts',(54.8387830086853,22.9887644352494,16.0295112098734));
#27435=CARTESIAN_POINT('Ctrl Pts',(54.7591401374331,22.9804424463828,16.0348535462997));
#27436=CARTESIAN_POINT('Ctrl Pts',(54.7256816112575,22.9760857719085,16.0371279668841));
#27437=CARTESIAN_POINT('Ctrl Pts',(54.5216007139205,22.9442293553838,16.0511777547821));
#27438=CARTESIAN_POINT('Ctrl Pts',(54.3550595163861,22.895504348459,16.0634895911408));
#27439=CARTESIAN_POINT('Ctrl Pts',(54.1725059008658,22.8152109195625,16.0770257718055));
#27440=CARTESIAN_POINT('Ctrl Pts',(54.1483379122983,22.8039980593172,16.0788167511038));
#27441=CARTESIAN_POINT('Ctrl Pts',(54.1086890281423,22.784628275968,16.0817449757792));
#27442=CARTESIAN_POINT('Ctrl Pts',(54.0930783862331,22.7767460619921,16.0828952554278));
#27443=CARTESIAN_POINT('Ctrl Pts',(54.0718746616439,22.7656874635857,16.0844520305494));
#27444=CARTESIAN_POINT('Ctrl Pts',(54.0661908340431,22.7626880912674,16.0848687758715));
#27445=CARTESIAN_POINT('Ctrl Pts',(54.0566752679509,22.757607755675,16.0855654000156));
#27446=CARTESIAN_POINT('Ctrl Pts',(54.052835716761,22.755541624276,16.085846195349));
#27447=CARTESIAN_POINT('Ctrl Pts',(54.0455672927288,22.7515995676119,16.0863771494168));
#27448=CARTESIAN_POINT('Ctrl Pts',(54.0421371184375,22.7497261324949,16.0866274673211));
#27449=CARTESIAN_POINT('Ctrl Pts',(54.03316649505,22.7447924224116,16.0872814927629));
#27450=CARTESIAN_POINT('Ctrl Pts',(54.0276350120165,22.7417158081494,16.0876841692534));
#27451=CARTESIAN_POINT('Ctrl Pts',(54.0084975014811,22.7309519261793,16.0890755366784));
#27452=CARTESIAN_POINT('Ctrl Pts',(53.9949668246376,22.723130908364,16.0900561136177));
#27453=CARTESIAN_POINT('Ctrl Pts',(53.87478628257,22.6517667126262,16.0987501399567));
#27454=CARTESIAN_POINT('Ctrl Pts',(53.7741781525531,22.5785463603168,16.1059285814372));
#27455=CARTESIAN_POINT('Ctrl Pts',(53.603251589636,22.4278894387557,16.1191470705425));
#27456=CARTESIAN_POINT('Ctrl Pts',(53.5309475554904,22.3533873067313,16.1251595485079));
#27457=CARTESIAN_POINT('Ctrl Pts',(53.4306264773859,22.2324581660068,16.134603087711));
#27458=CARTESIAN_POINT('Ctrl Pts',(53.3981591576725,22.1899544245668,16.1378684833555));
#27459=CARTESIAN_POINT('Ctrl Pts',(53.3594667012605,22.1348438701116,16.1420661687461));
#27460=CARTESIAN_POINT('Ctrl Pts',(53.3516121522717,22.1234044693955,16.1429355520399));
#27461=CARTESIAN_POINT('Ctrl Pts',(53.3392258182463,22.1049553521019,16.1443350513175));
#27462=CARTESIAN_POINT('Ctrl Pts',(53.3346174785919,22.0979973892846,16.144862275591));
#27463=CARTESIAN_POINT('Ctrl Pts',(53.3259542686719,22.0847371158717,16.1458660367145));
#27464=CARTESIAN_POINT('Ctrl Pts',(53.3218909760959,22.078440458489,16.1463422478664));
#27465=CARTESIAN_POINT('Ctrl Pts',(53.312729314577,22.0640659940059,16.147428491456));
#27466=CARTESIAN_POINT('Ctrl Pts',(53.3076533244991,22.0559742090416,16.1480393381325));
#27467=CARTESIAN_POINT('Ctrl Pts',(53.2946342094077,22.034885067494,16.1496298877366));
#27468=CARTESIAN_POINT('Ctrl Pts',(53.2867816135123,22.0218328246239,16.1506128670995));
#27469=CARTESIAN_POINT('Ctrl Pts',(53.2296205148942,21.9243107983856,16.1579483172394));
#27470=CARTESIAN_POINT('Ctrl Pts',(53.1864421929583,21.8364191017131,16.164519497285));
#27471=CARTESIAN_POINT('Ctrl Pts',(53.0862567539958,21.5878639483914,16.1829444895923));
#27472=CARTESIAN_POINT('Ctrl Pts',(53.0430946428215,21.4225134798834,16.1950806723162));
#27473=CARTESIAN_POINT('Ctrl Pts',(53.019560450095,21.2389708759667,16.207429839885));
#27474=CARTESIAN_POINT('Ctrl Pts',(53.0178369812036,21.224226863223,16.2084136164476));
#27475=CARTESIAN_POINT('Ctrl Pts',(53.0151045608743,21.1983496313746,16.2101242684407));
#27476=CARTESIAN_POINT('Ctrl Pts',(53.0140243256173,21.1872247716244,16.2108545328205));
#27477=CARTESIAN_POINT('Ctrl Pts',(53.012563477568,21.1707409752606,16.2119283601322));
#27478=CARTESIAN_POINT('Ctrl Pts',(53.0121109345581,21.1653888643838,16.2122757404523));
#27479=CARTESIAN_POINT('Ctrl Pts',(53.0113439388647,21.1558594884621,16.2128918921499));
#27480=CARTESIAN_POINT('Ctrl Pts',(53.0110210213271,21.1516830021988,16.2131611271738));
#27481=CARTESIAN_POINT('Ctrl Pts',(53.0103506777345,21.1426426084044,16.2137421494669));
#27482=CARTESIAN_POINT('Ctrl Pts',(53.0100079292455,21.1377784413014,16.2140536741187));
#27483=CARTESIAN_POINT('Ctrl Pts',(53.0091136985282,21.1243877079883,16.2149083929715));
#27484=CARTESIAN_POINT('Ctrl Pts',(53.0085991502623,21.1158586603934,16.2154495736587));
#27485=CARTESIAN_POINT('Ctrl Pts',(53.0062315447716,21.0719184875,16.2182222715861));
#27486=CARTESIAN_POINT('Ctrl Pts',(53.005268012528,21.0364634276237,16.220408186291));
#27487=CARTESIAN_POINT('Ctrl Pts',(53.0052114627833,20.9235559606981,16.2272590344726));
#27488=CARTESIAN_POINT('Ctrl Pts',(53.0096826393143,20.8461699327346,16.231791070704));
#27489=CARTESIAN_POINT('Ctrl Pts',(53.0376471964672,20.6060655371141,16.2458467845655));
#27490=CARTESIAN_POINT('Ctrl Pts',(53.0767300789211,20.4458884136019,16.255272797407));
#27491=CARTESIAN_POINT('Ctrl Pts',(53.1432410906208,20.270607673638,16.2668316519313));
#27492=CARTESIAN_POINT('Ctrl Pts',(53.1518577358801,20.2490426677452,16.2682751043158));
#27493=CARTESIAN_POINT('Ctrl Pts',(53.1644092478992,20.2191551260109,16.2703077732677));
#27494=CARTESIAN_POINT('Ctrl Pts',(53.1680284209469,20.2107014155392,16.2708863488285));
#27495=CARTESIAN_POINT('Ctrl Pts',(53.1747591454076,20.1952754035754,16.2719489257832));
#27496=CARTESIAN_POINT('Ctrl Pts',(53.1778525359606,20.1882953307888,16.2724323022653));
#27497=CARTESIAN_POINT('Ctrl Pts',(53.1841974042331,20.1741975246071,16.2734138946782));
#27498=CARTESIAN_POINT('Ctrl Pts',(53.1874508439226,20.1670808267956,16.2739121712414));
#27499=CARTESIAN_POINT('Ctrl Pts',(53.1955770116634,20.1495784302649,16.2751445222893));
#27500=CARTESIAN_POINT('Ctrl Pts',(53.2004975722282,20.1392153751135,16.2758802367237));
#27501=CARTESIAN_POINT('Ctrl Pts',(53.2191328965773,20.1008262304549,16.278628594994));
#27502=CARTESIAN_POINT('Ctrl Pts',(53.2334146535228,20.0730819135206,16.280660813995));
#27503=CARTESIAN_POINT('Ctrl Pts',(53.2706802502663,20.0046803400512,16.2857900156761));
#27504=CARTESIAN_POINT('Ctrl Pts',(53.2944512999519,19.9644754515107,16.2889131877857));
#27505=CARTESIAN_POINT('Ctrl Pts',(53.4153373850623,19.7754865697994,16.3041177557704));
#27506=CARTESIAN_POINT('Ctrl Pts',(53.5306127163732,19.6393095934495,16.3167788658583));
#27507=CARTESIAN_POINT('Ctrl Pts',(53.6929151901574,19.4926012712055,16.331650335323));
#27508=CARTESIAN_POINT('Ctrl Pts',(53.7242983911151,19.4659505916624,16.3344083711954));
#27509=CARTESIAN_POINT('Ctrl Pts',(53.7628670143991,19.4352009290907,16.3376385935785));
#27510=CARTESIAN_POINT('Ctrl Pts',(53.769279073216,19.4301528220171,16.3381705209695));
#27511=CARTESIAN_POINT('Ctrl Pts',(53.779841816629,19.4219414461249,16.3390382089016));
#27512=CARTESIAN_POINT('Ctrl Pts',(53.7839741802801,19.4187549212141,16.3393755394956));
#27513=CARTESIAN_POINT('Ctrl Pts',(53.7914383943204,19.4130457247644,16.3399809625644));
#27514=CARTESIAN_POINT('Ctrl Pts',(53.7947656909792,19.4105172892665,16.3402494530888));
#27515=CARTESIAN_POINT('Ctrl Pts',(53.8020869206996,19.4049900439929,16.3408371885131));
#27516=CARTESIAN_POINT('Ctrl Pts',(53.8060841713356,19.4019957757557,16.34115611786));
#27517=CARTESIAN_POINT('Ctrl Pts',(53.8175791558619,19.3934522983513,16.3420677915827));
#27518=CARTESIAN_POINT('Ctrl Pts',(53.8251047437251,19.3879405360954,16.3426580048986));
#27519=CARTESIAN_POINT('Ctrl Pts',(53.8777816013139,19.3499246865882,16.3467454085895));
#27520=CARTESIAN_POINT('Ctrl Pts',(53.9242412615003,19.31926591777,16.3501274585887));
#27521=CARTESIAN_POINT('Ctrl Pts',(54.0549708930179,19.2406426252822,16.3592251429767));
#27522=CARTESIAN_POINT('Ctrl Pts',(54.1415488574591,19.1968133497588,16.3648035508219));
#27523=CARTESIAN_POINT('Ctrl Pts',(54.3534521741567,19.1082750677843,16.3781430333399));
#27524=CARTESIAN_POINT('Ctrl Pts',(54.4807143850366,19.0694604406214,16.3859326024104));
#27525=CARTESIAN_POINT('Ctrl Pts',(54.6260522568909,19.0405536513744,16.395130678593));
#27526=CARTESIAN_POINT('Ctrl Pts',(54.6412600799103,19.0377124175135,16.3960963192744));
#27527=CARTESIAN_POINT('Ctrl Pts',(54.6659791115634,19.0333911863508,16.3976717178932));
#27528=CARTESIAN_POINT('Ctrl Pts',(54.675470869626,19.0318025967531,16.3982780355323));
#27529=CARTESIAN_POINT('Ctrl Pts',(54.6923817387835,19.0290979598449,16.399360895248));
#27530=CARTESIAN_POINT('Ctrl Pts',(54.6997963992206,19.0279549594167,16.3998365749015));
#27531=CARTESIAN_POINT('Ctrl Pts',(54.7154333123549,19.0256346962244,16.4008417044252));
#27532=CARTESIAN_POINT('Ctrl Pts',(54.723656805477,19.0244669104591,16.4013714439846));
#27533=CARTESIAN_POINT('Ctrl Pts',(54.7454592099145,19.0215096321512,16.4027790394612));
#27534=CARTESIAN_POINT('Ctrl Pts',(54.7590494791707,19.0198086000397,16.4036596620654));
#27535=CARTESIAN_POINT('Ctrl Pts',(54.8236584247461,19.0123967445265,16.4078621950756));
#27536=CARTESIAN_POINT('Ctrl Pts',(54.8748635201592,19.0085173571559,16.4112408832987));
#27537=CARTESIAN_POINT('Ctrl Pts',(55.0990859493058,19.0002113142077,16.4262556258336));
#27538=CARTESIAN_POINT('Ctrl Pts',(55.2720999440669,19.0163373238995,16.4384970524789));
#27539=CARTESIAN_POINT('Ctrl Pts',(55.4605248569908,19.0590330781742,16.451824864577));
#27540=CARTESIAN_POINT('Ctrl Pts',(55.4801601745615,19.0637970192429,16.4532124640954));
#27541=CARTESIAN_POINT('Ctrl Pts',(55.5451225170653,19.0806072815599,16.45779257595));
#27542=CARTESIAN_POINT('Ctrl Pts',(55.5901006235765,19.0939546155396,16.460946542983));
#27543=CARTESIAN_POINT('Ctrl Pts',(55.6426049299667,19.1115725339209,16.4645757495137));
#27544=CARTESIAN_POINT('Ctrl Pts',(55.6506227064949,19.1143198864729,16.4651284776957));
#27545=CARTESIAN_POINT('Ctrl Pts',(55.6636387322246,19.1188728292564,16.4660230887076));
#27546=CARTESIAN_POINT('Ctrl Pts',(55.6686476066829,19.1206474042688,16.466366705827));
#27547=CARTESIAN_POINT('Ctrl Pts',(55.6775880103507,19.1238551334369,16.4669787924025));
#27548=CARTESIAN_POINT('Ctrl Pts',(55.6815221667754,19.1252806585091,16.4672477010287));
#27549=CARTESIAN_POINT('Ctrl Pts',(55.6900701921505,19.1284084643146,16.4678310216155));
#27550=CARTESIAN_POINT('Ctrl Pts',(55.6946822540327,19.1301154276973,16.4681451521033));
#27551=CARTESIAN_POINT('Ctrl Pts',(55.7076888940472,19.1349840603751,16.4690294770064));
#27552=CARTESIAN_POINT('Ctrl Pts',(55.7160686529637,19.1381853697941,16.4695973719998));
#27553=CARTESIAN_POINT('Ctrl Pts',(55.7687123792409,19.1587047971324,16.4731550793167));
#27554=CARTESIAN_POINT('Ctrl Pts',(55.8123710089035,19.1775453629133,16.4760611975641));
#27555=CARTESIAN_POINT('Ctrl Pts',(55.9172009039299,19.2273008779699,16.4830268194116));
#27556=CARTESIAN_POINT('Ctrl Pts',(55.9775332045311,19.2598420691,16.4870259601096));
#27557=CARTESIAN_POINT('Ctrl Pts',(56.1728184389423,19.3785403082978,16.5003053403762));
#27558=CARTESIAN_POINT('Ctrl Pts',(56.2990479960508,19.477796743011,16.5095064997491));
#27559=CARTESIAN_POINT('Ctrl Pts',(56.4283795654249,19.6074149562052,16.5207916209559));
#27560=CARTESIAN_POINT('Ctrl Pts',(56.4444114981475,19.6240506396237,16.5222270383163));
#27561=CARTESIAN_POINT('Ctrl Pts',(56.4665726693188,19.6478605748917,16.5242656996864));
#27562=CARTESIAN_POINT('Ctrl Pts',(56.4729458644109,19.6548060009975,16.5248585418334));
#27563=CARTESIAN_POINT('Ctrl Pts',(56.4839631225199,19.6669846351443,16.525895038272));
#27564=CARTESIAN_POINT('Ctrl Pts',(56.4886293608479,19.6721976291882,16.5263377499807));
#27565=CARTESIAN_POINT('Ctrl Pts',(56.4983385426044,19.6831599719289,16.5272667999152));
#27566=CARTESIAN_POINT('Ctrl Pts',(56.5033760311357,19.6889139791321,16.5277533547985));
#27567=CARTESIAN_POINT('Ctrl Pts',(56.515291062202,19.7026827317148,16.5289151292469));
#27568=CARTESIAN_POINT('Ctrl Pts',(56.5221382309122,19.7107233436249,16.5295915836029));
#27569=CARTESIAN_POINT('Ctrl Pts',(56.5451317183074,19.7381630232643,16.5318936416007));
#27570=CARTESIAN_POINT('Ctrl Pts',(56.5609730477529,19.7578133674733,16.5335314801522));
#27571=CARTESIAN_POINT('Ctrl Pts',(56.5980423517159,19.8056250313779,16.5374929556275));
#27572=CARTESIAN_POINT('Ctrl Pts',(56.6189041182807,19.8340582662579,16.5398299786787));
#27573=CARTESIAN_POINT('Ctrl Pts',(56.6979812095146,19.9480517405075,16.5491275802197));
#27574=CARTESIAN_POINT('Ctrl Pts',(56.7502502868686,20.0375267274254,16.5562819317914));
#27575=CARTESIAN_POINT('Ctrl Pts',(56.8495589492488,20.2426120419385,16.5721658004954));
#27576=CARTESIAN_POINT('Ctrl Pts',(56.8931895521639,20.3594193327613,16.580890335521));
#27577=CARTESIAN_POINT('Ctrl Pts',(56.9297335230146,20.4946284319398,16.5901651817147));
#27578=CARTESIAN_POINT('Ctrl Pts',(56.9336345488825,20.5097660156899,16.5911920441129));
#27579=CARTESIAN_POINT('Ctrl Pts',(56.9388648674058,20.5310963239378,16.5926213706501));
#27580=CARTESIAN_POINT('Ctrl Pts',(56.9403431168462,20.5372514472932,16.5930317695687));
#27581=CARTESIAN_POINT('Ctrl Pts',(56.9426866973043,20.5472183363115,16.5936928925391));
#27582=CARTESIAN_POINT('Ctrl Pts',(56.9435701542898,20.5510257302973,16.5939446369818));
#27583=CARTESIAN_POINT('Ctrl Pts',(56.9454154319158,20.559085757558,16.59447582234));
#27584=CARTESIAN_POINT('Ctrl Pts',(56.946374511523,20.5633389947533,16.5947550999943));
#27585=CARTESIAN_POINT('Ctrl Pts',(56.9487125913686,20.5738684586513,16.5954440292946));
#27586=CARTESIAN_POINT('Ctrl Pts',(56.9500752383944,20.5801483337848,16.59585275498));
#27587=CARTESIAN_POINT('Ctrl Pts',(56.9550319564925,20.6035366091234,16.5973673306903));
#27588=CARTESIAN_POINT('Ctrl Pts',(56.9584315491732,20.6206860301097,16.5984626898699));
#27589=CARTESIAN_POINT('Ctrl Pts',(56.9664395307292,20.6640651294788,16.6012001961631));
#27590=CARTESIAN_POINT('Ctrl Pts',(56.9707490718081,20.6903471285931,16.6028283394322));
#27591=CARTESIAN_POINT('Ctrl Pts',(56.9990482898444,20.887591833986,16.6148731472246));
#27592=CARTESIAN_POINT('Ctrl Pts',(57.0012812043129,21.0609456362895,16.6245431781641));
#27593=CARTESIAN_POINT('Ctrl Pts',(56.9771446920451,21.2666737381516,16.6368093550055));
#27594=CARTESIAN_POINT('Ctrl Pts',(56.9722409103681,21.3008016651394,16.6388680968441));
#27595=CARTESIAN_POINT('Ctrl Pts',(56.9587562077782,21.3800080994893,16.643720968125));
#27596=CARTESIAN_POINT('Ctrl Pts',(56.9494997089953,21.424949908316,16.6465317899244));
#27597=CARTESIAN_POINT('Ctrl Pts',(56.9354743870564,21.4828608366111,16.6502470679314));
#27598=CARTESIAN_POINT('Ctrl Pts',(56.9321085390098,21.4961575043093,16.6511065531592));
#27599=CARTESIAN_POINT('Ctrl Pts',(56.9264836019209,21.5174529507766,16.6524938843764));
#27600=CARTESIAN_POINT('Ctrl Pts',(56.9243111407577,21.5254743142202,16.6530189284386));
#27601=CARTESIAN_POINT('Ctrl Pts',(56.92008247535,21.5407098296726,16.6540210039146));
#27602=CARTESIAN_POINT('Ctrl Pts',(56.9180355717871,21.5479264320045,16.6544977260633));
#27603=CARTESIAN_POINT('Ctrl Pts',(56.9132720092965,21.564367117701,16.655588592212));
#27604=CARTESIAN_POINT('Ctrl Pts',(56.9105292757201,21.57358339094,16.6562035764157));
#27605=CARTESIAN_POINT('Ctrl Pts',(56.9018876950974,21.6018714846647,16.6581020777423));
#27606=CARTESIAN_POINT('Ctrl Pts',(56.895769243688,21.6208743958594,16.6593927302699));
#27607=CARTESIAN_POINT('Ctrl Pts',(56.8418651447053,21.7800608989802,16.6703374175295));
#27608=CARTESIAN_POINT('Ctrl Pts',(56.778897755014,21.9145866874014,16.6805124866896));
#27609=CARTESIAN_POINT('Ctrl Pts',(56.6375284497124,22.1456987581866,16.6994001612998));
#27610=CARTESIAN_POINT('Ctrl Pts',(56.5638594129683,22.2443770308778,16.7080119947219));
#27611=CARTESIAN_POINT('Ctrl Pts',(56.471073987426,22.3472990300759,16.7171888389506));
#27612=CARTESIAN_POINT('Ctrl Pts',(56.4604391214733,22.3588196944641,16.7182188162755));
#27613=CARTESIAN_POINT('Ctrl Pts',(56.4453156391032,22.3748201459238,16.7196517189097));
#27614=CARTESIAN_POINT('Ctrl Pts',(56.4409401371259,22.3794053987654,16.7200626305579));
#27615=CARTESIAN_POINT('Ctrl Pts',(56.4338300562903,22.3867855709037,16.7207243574907));
#27616=CARTESIAN_POINT('Ctrl Pts',(56.4311090268805,22.3895933951395,16.7209761966869));
#27617=CARTESIAN_POINT('Ctrl Pts',(56.4253375241308,22.3955140627817,16.7215073704384));
#27618=CARTESIAN_POINT('Ctrl Pts',(56.4222850715316,22.3986249436822,16.7217865427214));
#27619=CARTESIAN_POINT('Ctrl Pts',(56.4147126925049,22.4062918425188,16.722474847349));
#27620=CARTESIAN_POINT('Ctrl Pts',(56.4101808816058,22.4108361465969,16.722883057474));
#27621=CARTESIAN_POINT('Ctrl Pts',(56.3932638787373,22.4276368350131,16.7243935122706));
#27622=CARTESIAN_POINT('Ctrl Pts',(56.3807397681024,22.4397530726264,16.7254853400426));
#27623=CARTESIAN_POINT('Ctrl Pts',(56.2927548360319,22.5226683776526,16.7329886492401));
#27624=CARTESIAN_POINT('Ctrl Pts',(56.2120341576318,22.5876752337866,16.7390388118718));
#27625=CARTESIAN_POINT('Ctrl Pts',(55.9944577645075,22.7365861631073,16.7543595782276));
#27626=CARTESIAN_POINT('Ctrl Pts',(55.8518958447368,22.8107857545053,16.7635678864731));
#27627=CARTESIAN_POINT('Ctrl Pts',(55.6803890940358,22.8752683604837,16.7748607244433));
#27628=CARTESIAN_POINT('Ctrl Pts',(55.6586368096638,22.883018382106,16.776295422476));
#27629=CARTESIAN_POINT('Ctrl Pts',(55.6278242752848,22.8933972273267,16.7783332271837));
#27630=CARTESIAN_POINT('Ctrl Pts',(55.6188718945133,22.8963422566568,16.7789259437965));
#27631=CARTESIAN_POINT('Ctrl Pts',(55.6032382395922,22.9013627037559,16.7799622834222));
#27632=CARTESIAN_POINT('Ctrl Pts',(55.5965662407865,22.9034666330844,16.7804049645839));
#27633=CARTESIAN_POINT('Ctrl Pts',(55.582577433782,22.9077970510717,16.7813340124989));
#27634=CARTESIAN_POINT('Ctrl Pts',(55.5752586251918,22.9100166402144,16.7818205962305));
#27635=CARTESIAN_POINT('Ctrl Pts',(55.5578010711509,22.915201585621,16.7829825547831));
#27636=CARTESIAN_POINT('Ctrl Pts',(55.5476512611181,22.9181285769288,16.7836591654271));
#27637=CARTESIAN_POINT('Ctrl Pts',(55.5131590942342,22.9277793074789,16.7859623196652));
#27638=CARTESIAN_POINT('Ctrl Pts',(55.4887133005297,22.9341211252453,16.7876011139753));
#27639=CARTESIAN_POINT('Ctrl Pts',(55.429835511088,22.9482079500885,16.7915653208806));
#27640=CARTESIAN_POINT('Ctrl Pts',(55.3953064592348,22.9555064135001,16.7939041439786));
#27641=CARTESIAN_POINT('Ctrl Pts',(55.2956630533863,22.9738213409399,16.8006939504547));
#27642=CARTESIAN_POINT('Ctrl Pts',(55.230196952794,22.9825209717304,16.8052054740242));
#27643=CARTESIAN_POINT('Ctrl Pts',(55.1644482145651,22.9879598454764,16.809768216174));
#27644=CARTESIAN_POINT('Origin',(55.,21.,6.22095488139522));
#27645=CARTESIAN_POINT('',(55.1644483624361,22.9879598332441,17.7696788290115));
#27646=CARTESIAN_POINT('',(55.1644483516309,22.987959834138,17.6123430797447));
#27647=CARTESIAN_POINT('',(55.1644483516311,22.987959834138,6.22095488139522));
#27648=CARTESIAN_POINT('Ctrl Pts',(55.1644483624361,22.9879598332441,17.7696788290115));
#27649=CARTESIAN_POINT('Ctrl Pts',(55.1727211370528,22.9872754913295,17.7691119138002));
#27650=CARTESIAN_POINT('Ctrl Pts',(55.1809902822389,22.9865394563269,17.7685438340102));
#27651=CARTESIAN_POINT('Ctrl Pts',(55.3342501289964,22.9719327759608,17.7579896043575));
#27652=CARTESIAN_POINT('Ctrl Pts',(55.4772844216076,22.942276542055,17.7476720793255));
#27653=CARTESIAN_POINT('Ctrl Pts',(55.6630129392337,22.8819947351274,17.7343263805435));
#27654=CARTESIAN_POINT('Ctrl Pts',(55.7096317441393,22.8649166339012,17.7309856455773));
#27655=CARTESIAN_POINT('Ctrl Pts',(55.7639655352898,22.8426791733497,17.7271408954905));
#27656=CARTESIAN_POINT('Ctrl Pts',(55.7723387837987,22.8391853320381,17.7265498015878));
#27657=CARTESIAN_POINT('Ctrl Pts',(55.7852346520752,22.8337007699802,17.7256419507824));
#27658=CARTESIAN_POINT('Ctrl Pts',(55.7897740721651,22.8317502255672,17.7253228651882));
#27659=CARTESIAN_POINT('Ctrl Pts',(55.7981441236325,22.8281167974787,17.7247354730493));
#27660=CARTESIAN_POINT('Ctrl Pts',(55.8019766854936,22.826438738037,17.7244668911211));
#27661=CARTESIAN_POINT('Ctrl Pts',(55.8106409613816,22.8226126171648,17.7238605448605));
#27662=CARTESIAN_POINT('Ctrl Pts',(55.8154694237916,22.8204573988237,17.7235232214984));
#27663=CARTESIAN_POINT('Ctrl Pts',(55.82976969201,22.8140060611981,17.7225257536937));
#27664=CARTESIAN_POINT('Ctrl Pts',(55.8392167053402,22.8096549572621,17.7218688589099));
#27665=CARTESIAN_POINT('Ctrl Pts',(55.9420755893927,22.7613015174512,17.7147344541242));
#27666=CARTESIAN_POINT('Ctrl Pts',(56.0319838577951,22.7101768510187,17.7086558723331));
#27667=CARTESIAN_POINT('Ctrl Pts',(56.2215883363034,22.5819381445825,17.6953264893371));
#27668=CARTESIAN_POINT('Ctrl Pts',(56.3187526462928,22.5018975623111,17.6881240682622));
#27669=CARTESIAN_POINT('Ctrl Pts',(56.449843344617,22.3713178956923,17.6770487735918));
#27670=CARTESIAN_POINT('Ctrl Pts',(56.4900444139618,22.3275259363384,17.6734308050266));
#27671=CARTESIAN_POINT('Ctrl Pts',(56.5374449600636,22.2710217147678,17.6688360902894));
#27672=CARTESIAN_POINT('Ctrl Pts',(56.5465423610585,22.2599364718552,17.6679380709916));
#27673=CARTESIAN_POINT('Ctrl Pts',(56.5608087049701,22.2421655041724,17.6665032667212));
#27674=CARTESIAN_POINT('Ctrl Pts',(56.5660561595535,22.2355432225677,17.6659696391487));
#27675=CARTESIAN_POINT('Ctrl Pts',(56.5758687535112,22.2229967978546,17.6649604958994));
#27676=CARTESIAN_POINT('Ctrl Pts',(56.5804429689339,22.2170799132784,17.664485352131));
#27677=CARTESIAN_POINT('Ctrl Pts',(56.5906836826698,22.2036781610116,17.6634107947475));
#27678=CARTESIAN_POINT('Ctrl Pts',(56.5963308018917,22.1961787740802,17.6628106345124));
#27679=CARTESIAN_POINT('Ctrl Pts',(56.6106751101889,22.1768470138711,17.6612663160671));
#27680=CARTESIAN_POINT('Ctrl Pts',(56.6192948340342,22.1649581219788,17.660319190064));
#27681=CARTESIAN_POINT('Ctrl Pts',(56.6745942781716,22.0868858081109,17.6541153324867));
#27682=CARTESIAN_POINT('Ctrl Pts',(56.7173318081134,22.0180153344787,17.6487109847649));
#27683=CARTESIAN_POINT('Ctrl Pts',(56.8162142209219,21.8346356495947,17.634500610101));
#27684=CARTESIAN_POINT('Ctrl Pts',(56.865787044583,21.7169973038166,17.6255363549217));
#27685=CARTESIAN_POINT('Ctrl Pts',(56.9248551351996,21.5281419240925,17.6118278296533));
#27686=CARTESIAN_POINT('Ctrl Pts',(56.9423250724568,21.459757043164,17.6070005688506));
#27687=CARTESIAN_POINT('Ctrl Pts',(56.9589731226165,21.3763796971723,17.6013819138472));
#27688=CARTESIAN_POINT('Ctrl Pts',(56.9616546305764,21.3621443237195,17.6004319136836));
#27689=CARTESIAN_POINT('Ctrl Pts',(56.9652214123138,21.3420057867138,17.5991022549349));
#27690=CARTESIAN_POINT('Ctrl Pts',(56.9662355536595,21.3361263264149,17.5987157738654));
#27691=CARTESIAN_POINT('Ctrl Pts',(56.9679305830337,21.3260291911563,17.5980550892619));
#27692=CARTESIAN_POINT('Ctrl Pts',(56.9686243242136,21.3218137421265,17.5977801694701));
#27693=CARTESIAN_POINT('Ctrl Pts',(56.9699431343234,21.3136362502739,17.5972486542128));
#27694=CARTESIAN_POINT('Ctrl Pts',(56.9705697986139,21.3096745379212,17.5969919651593));
#27695=CARTESIAN_POINT('Ctrl Pts',(56.9722360397465,21.2989308303612,17.5962979873865));
#27696=CARTESIAN_POINT('Ctrl Pts',(56.9732525937669,21.2921452418095,17.5958619817642));
#27697=CARTESIAN_POINT('Ctrl Pts',(56.9769530600663,21.266543441906,17.594225159882));
#27698=CARTESIAN_POINT('Ctrl Pts',(56.9794031119317,21.247693744364,17.5930367277394));
#27699=CARTESIAN_POINT('Ctrl Pts',(56.9979493596186,21.0870768118537,17.5830300119546));
#27700=CARTESIAN_POINT('Ctrl Pts',(56.9990639254823,20.9439758305669,17.5748856529494));
#27701=CARTESIAN_POINT('Ctrl Pts',(56.9721269600911,20.6739874262591,17.5591149443914));
#27702=CARTESIAN_POINT('Ctrl Pts',(56.9470139027634,20.5475628890419,17.5515500306981));
#27703=CARTESIAN_POINT('Ctrl Pts',(56.9050123411785,20.408185958683,17.5425121361114));
#27704=CARTESIAN_POINT('Ctrl Pts',(56.8999057734108,20.3919918555079,17.5414514650829));
#27705=CARTESIAN_POINT('Ctrl Pts',(56.8917718970462,20.3673010524774,17.539817191712));
#27706=CARTESIAN_POINT('Ctrl Pts',(56.8888925825961,20.3587561495401,17.539248448773));
#27707=CARTESIAN_POINT('Ctrl Pts',(56.8835501137769,20.3432496218506,17.538210455999));
#27708=CARTESIAN_POINT('Ctrl Pts',(56.8811060357845,20.3362815581554,17.5377418439537));
#27709=CARTESIAN_POINT('Ctrl Pts',(56.8756982038185,20.3211336634636,17.5367183022653));
#27710=CARTESIAN_POINT('Ctrl Pts',(56.87271952222,20.3129593594056,17.5361628843627));
#27711=CARTESIAN_POINT('Ctrl Pts',(56.8644324160613,20.2906716606282,17.5346399306964));
#27712=CARTESIAN_POINT('Ctrl Pts',(56.8590173722913,20.2765987863634,17.5336688570134));
#27713=CARTESIAN_POINT('Ctrl Pts',(56.8299940618303,20.2036502384309,17.5285846948711));
#27714=CARTESIAN_POINT('Ctrl Pts',(56.8037491725794,20.1458696502639,17.524383602192));
#27715=CARTESIAN_POINT('Ctrl Pts',(56.6959452379606,19.935745355291,17.5084392774208));
#27716=CARTESIAN_POINT('Ctrl Pts',(56.5974757924373,19.7929679034666,17.4961674473908));
#27717=CARTESIAN_POINT('Ctrl Pts',(56.446552971803,19.6254840691648,17.4807284424302));
#27718=CARTESIAN_POINT('Ctrl Pts',(56.4097007471355,19.5877130492383,17.4771711809947));
#27719=CARTESIAN_POINT('Ctrl Pts',(56.3647017797651,19.5451111837247,17.4731119635997));
#27720=CARTESIAN_POINT('Ctrl Pts',(56.3579685440455,19.5388244949092,17.4725116942493));
#27721=CARTESIAN_POINT('Ctrl Pts',(56.3475354173537,19.5292177025552,17.4715927996984));
#27722=CARTESIAN_POINT('Ctrl Pts',(56.3438663695168,19.52586450769,17.4712717576575));
#27723=CARTESIAN_POINT('Ctrl Pts',(56.3370874547228,19.5197155044717,17.4706825348509));
#27724=CARTESIAN_POINT('Ctrl Pts',(56.3339813442382,19.5169157734268,17.4704140653092));
#27725=CARTESIAN_POINT('Ctrl Pts',(56.326955473649,19.5106228487159,17.4698101850031));
#27726=CARTESIAN_POINT('Ctrl Pts',(56.3230307201806,19.5071353568412,17.4694751994743));
#27727=CARTESIAN_POINT('Ctrl Pts',(56.3114213973615,19.4969011845475,17.4684910651037));
#27728=CARTESIAN_POINT('Ctrl Pts',(56.3036985283561,19.4901979308098,17.4678450384129));
#27729=CARTESIAN_POINT('Ctrl Pts',(56.2423831296835,19.4377990172389,17.4627805203232));
#27730=CARTESIAN_POINT('Ctrl Pts',(56.1864498876303,19.394906012039,17.4585457210283));
#27731=CARTESIAN_POINT('Ctrl Pts',(55.9883735449417,19.2590342867202,17.4443698665764));
#27732=CARTESIAN_POINT('Ctrl Pts',(55.8367087728335,19.1812738922679,17.4347996376259));
#27733=CARTESIAN_POINT('Ctrl Pts',(55.6459759638719,19.1124533991687,17.4225818331388));
#27734=CARTESIAN_POINT('Ctrl Pts',(55.6146550000423,19.1020231377892,17.4205726507406));
#27735=CARTESIAN_POINT('Ctrl Pts',(55.5601498832996,19.0853629241264,17.4170614155901));
#27736=CARTESIAN_POINT('Ctrl Pts',(55.5370850522489,19.0787653465232,17.4155711009342));
#27737=CARTESIAN_POINT('Ctrl Pts',(55.5039053807717,19.0699186321814,17.4134184167345));
#27738=CARTESIAN_POINT('Ctrl Pts',(55.4938827112266,19.0673296762664,17.4127670150505));
#27739=CARTESIAN_POINT('Ctrl Pts',(55.4764554173765,19.0629724456127,17.411632206341));
#27740=CARTESIAN_POINT('Ctrl Pts',(55.4690599165999,19.0611683148806,17.4111499640131));
#27741=CARTESIAN_POINT('Ctrl Pts',(55.4547996665773,19.0577758956194,17.4102187218161));
#27742=CARTESIAN_POINT('Ctrl Pts',(55.4479364619659,19.0561815588124,17.4097699243761));
#27743=CARTESIAN_POINT('Ctrl Pts',(55.4298682306864,19.0520850430731,17.4085867425501));
#27744=CARTESIAN_POINT('Ctrl Pts',(55.4186499263322,19.0496432107887,17.4078504392147));
#27745=CARTESIAN_POINT('Ctrl Pts',(55.3791285066018,19.0413974679117,17.405250224726));
#27746=CARTESIAN_POINT('Ctrl Pts',(55.350722097956,19.0361119766629,17.4033699724366));
#27747=CARTESIAN_POINT('Ctrl Pts',(55.1336625962208,19.0005837761638,17.388909471515));
#27748=CARTESIAN_POINT('Ctrl Pts',(54.9416818636509,18.9969771899368,17.3754473186876));
#27749=CARTESIAN_POINT('Ctrl Pts',(54.7010742129763,19.0271027123333,17.3586600033628));
#27750=CARTESIAN_POINT('Ctrl Pts',(54.6502315123305,19.0354789221204,17.3551270455247));
#27751=CARTESIAN_POINT('Ctrl Pts',(54.5815218559772,19.0495512179538,17.350417226066));
#27752=CARTESIAN_POINT('Ctrl Pts',(54.563329282594,19.0535434381311,17.3491764989184));
#27753=CARTESIAN_POINT('Ctrl Pts',(54.5322131563923,19.0608298707927,17.3470682356078));
#27754=CARTESIAN_POINT('Ctrl Pts',(54.519262091081,19.0639998948768,17.3461948901747));
#27755=CARTESIAN_POINT('Ctrl Pts',(54.5007525320873,19.0687276667856,17.3449536162804));
#27756=CARTESIAN_POINT('Ctrl Pts',(54.4951678304224,19.0701799716471,17.3445800042905));
#27757=CARTESIAN_POINT('Ctrl Pts',(54.4854910175825,19.0727413138723,17.3439342992412));
#27758=CARTESIAN_POINT('Ctrl Pts',(54.4813960244936,19.073839193056,17.3436615733915));
#27759=CARTESIAN_POINT('Ctrl Pts',(54.4728131920417,19.0761696304915,17.3430910838046));
#27760=CARTESIAN_POINT('Ctrl Pts',(54.468326149636,19.0774048426558,17.3427934749137));
#27761=CARTESIAN_POINT('Ctrl Pts',(54.456364918728,19.080742658224,17.342001735944));
#27762=CARTESIAN_POINT('Ctrl Pts',(54.4488985230971,19.0828732403836,17.3415091954168));
#27763=CARTESIAN_POINT('Ctrl Pts',(54.4163336554861,19.0923717952355,17.3393675308833));
#27764=CARTESIAN_POINT('Ctrl Pts',(54.3913677678926,19.1001898174323,17.3377426940248));
#27765=CARTESIAN_POINT('Ctrl Pts',(54.1650774284183,19.1759713614955,17.3231105887006));
#27766=CARTESIAN_POINT('Ctrl Pts',(53.9756480155405,19.2752087188727,17.3114183926279));
#27767=CARTESIAN_POINT('Ctrl Pts',(53.7611385650347,19.4356123219912,17.2953408045764));
#27768=CARTESIAN_POINT('Ctrl Pts',(53.7182454651794,19.4705586211622,17.2919662809799));
#27769=CARTESIAN_POINT('Ctrl Pts',(53.6663646236829,19.5165442291925,17.2876454266519));
#27770=CARTESIAN_POINT('Ctrl Pts',(53.6559656773835,19.5259592730773,17.2867666912311));
#27771=CARTESIAN_POINT('Ctrl Pts',(53.6395141801564,19.5411730290735,17.2853555949521));
#27772=CARTESIAN_POINT('Ctrl Pts',(53.6333972541059,19.5469016796722,17.2848262110897));
#27773=CARTESIAN_POINT('Ctrl Pts',(53.6218821568268,19.5578228704351,17.2838205594798));
#27774=CARTESIAN_POINT('Ctrl Pts',(53.6164767648721,19.5630076137764,17.2833446325426));
#27775=CARTESIAN_POINT('Ctrl Pts',(53.6042825750738,19.5748366181754,17.2822621013265));
#27776=CARTESIAN_POINT('Ctrl Pts',(53.597511819851,19.5814991383441,17.2816547051114));
#27777=CARTESIAN_POINT('Ctrl Pts',(53.5801362097604,19.5988430032695,17.2800793348104));
#27778=CARTESIAN_POINT('Ctrl Pts',(53.5696043582906,19.6095963176532,17.2791081880461));
#27779=CARTESIAN_POINT('Ctrl Pts',(53.4959217533156,19.6865515447671,17.2721960569072));
#27780=CARTESIAN_POINT('Ctrl Pts',(53.4372786470323,19.7569006716248,17.2660648101233));
#27781=CARTESIAN_POINT('Ctrl Pts',(53.298438532853,19.9488714009877,17.2498215277306));
#27782=CARTESIAN_POINT('Ctrl Pts',(53.2263529908419,20.0756863860817,17.2395187277375));
#27783=CARTESIAN_POINT('Ctrl Pts',(53.149033594468,20.2547409998105,17.226189050458));
#27784=CARTESIAN_POINT('Ctrl Pts',(53.1310739760065,20.3009978180914,17.2228502222859));
#27785=CARTESIAN_POINT('Ctrl Pts',(53.1118905809067,20.3564530527736,17.219007367434));
#27786=CARTESIAN_POINT('Ctrl Pts',(53.1089834404711,20.3650462765884,17.2184163581595));
#27787=CARTESIAN_POINT('Ctrl Pts',(53.1045837023256,20.3783497539317,17.2175086092736));
#27788=CARTESIAN_POINT('Ctrl Pts',(53.1030498576763,20.3830460886352,17.2171895417771));
#27789=CARTESIAN_POINT('Ctrl Pts',(53.1002492861543,20.3917300823297,17.2166021664195));
#27790=CARTESIAN_POINT('Ctrl Pts',(53.0989776641877,20.3957160048397,17.2163335832994));
#27791=CARTESIAN_POINT('Ctrl Pts',(53.0961272337681,20.4047487805527,17.2157272135416));
#27792=CARTESIAN_POINT('Ctrl Pts',(53.0945559490641,20.4097979205734,17.2153898680229));
#27793=CARTESIAN_POINT('Ctrl Pts',(53.0905445382888,20.4228711235624,17.2145204112469));
#27794=CARTESIAN_POINT('Ctrl Pts',(53.0881348760144,20.4309045301535,17.2139900173989));
#27795=CARTESIAN_POINT('Ctrl Pts',(53.073075665954,20.4822847281425,17.2106210336925));
#27796=CARTESIAN_POINT('Ctrl Pts',(53.0618493043905,20.5260389516752,17.2078576814511));
#27797=CARTESIAN_POINT('Ctrl Pts',(53.0471334016904,20.5927231404566,17.2037525131035));
#27798=CARTESIAN_POINT('Ctrl Pts',(53.0425427310998,20.6153917667218,17.2023753145903));
#27799=CARTESIAN_POINT('Ctrl Pts',(53.0164266325669,20.7569661677294,17.1938600935992));
#27800=CARTESIAN_POINT('Ctrl Pts',(53.0053482399933,20.8775452457192,17.1869681386615));
#27801=CARTESIAN_POINT('Ctrl Pts',(53.0051725872726,21.0950537116775,17.1742123628961));
#27802=CARTESIAN_POINT('Ctrl Pts',(53.0121208370533,21.1915841068912,17.1684384195527));
#27803=CARTESIAN_POINT('Ctrl Pts',(53.0282260160935,21.3022682024253,17.1614932105762));
#27804=CARTESIAN_POINT('Ctrl Pts',(53.0305870496939,21.3172874421646,17.1605439941625));
#27805=CARTESIAN_POINT('Ctrl Pts',(53.0347094477701,21.3416894991796,17.1589900572137));
#27806=CARTESIAN_POINT('Ctrl Pts',(53.0363669180387,21.351089422884,17.1583886211391));
#27807=CARTESIAN_POINT('Ctrl Pts',(53.039446211268,21.3678485820801,17.1573110830264));
#27808=CARTESIAN_POINT('Ctrl Pts',(53.0408421787836,21.3752124290471,17.1568358104766));
#27809=CARTESIAN_POINT('Ctrl Pts',(53.0438817756099,21.390766992798,17.1558279880372));
#27810=CARTESIAN_POINT('Ctrl Pts',(53.0455354211034,21.3989555824773,17.155295127194));
#27811=CARTESIAN_POINT('Ctrl Pts',(53.0500787943295,21.4207472473699,17.1538708106436));
#27812=CARTESIAN_POINT('Ctrl Pts',(53.0530593799626,21.4343307038317,17.1529764713609));
#27813=CARTESIAN_POINT('Ctrl Pts',(53.0682623591484,21.5003120457261,17.1485996333796));
#27814=CARTESIAN_POINT('Ctrl Pts',(53.0824582988953,21.5522276395413,17.1450544744596));
#27815=CARTESIAN_POINT('Ctrl Pts',(53.1575551697278,21.7888119097579,17.1284151964815));
#27816=CARTESIAN_POINT('Ctrl Pts',(53.2431358141639,21.9644865340944,17.114539294953));
#27817=CARTESIAN_POINT('Ctrl Pts',(53.3771894969855,22.1607716562556,17.0983561041384));
#27818=CARTESIAN_POINT('Ctrl Pts',(53.4027861275306,22.1957479873078,17.0954487816379));
#27819=CARTESIAN_POINT('Ctrl Pts',(53.4346130811539,22.2363899179212,17.0920673616161));
#27820=CARTESIAN_POINT('Ctrl Pts',(53.4397630794305,22.2428825335638,17.0915270815543));
#27821=CARTESIAN_POINT('Ctrl Pts',(53.4482463724457,22.2534416155369,17.0906485204068));
#27822=CARTESIAN_POINT('Ctrl Pts',(53.4515554864122,22.2575272538061,17.0903086044777));
#27823=CARTESIAN_POINT('Ctrl Pts',(53.4575257571423,22.2648392239252,17.0897003870114));
#27824=CARTESIAN_POINT('Ctrl Pts',(53.460180929635,22.2680702992331,17.0894316709026));
#27825=CARTESIAN_POINT('Ctrl Pts',(53.4660102950184,22.2751187371143,17.0888455894302));
#27826=CARTESIAN_POINT('Ctrl Pts',(53.4691885780625,22.2789326020124,17.0885285259616));
#27827=CARTESIAN_POINT('Ctrl Pts',(53.4782868494599,22.289767806072,17.0876277917881));
#27828=CARTESIAN_POINT('Ctrl Pts',(53.4842412267826,22.2967602921213,17.0870465574006));
#27829=CARTESIAN_POINT('Ctrl Pts',(53.5242952520686,22.3431446411389,17.0831893733766));
#27830=CARTESIAN_POINT('Ctrl Pts',(53.5598818965131,22.3812323923223,17.0800142384225));
#27831=CARTESIAN_POINT('Ctrl Pts',(53.7151413161528,22.534870245432,17.0669520766201));
#27832=CARTESIAN_POINT('Ctrl Pts',(53.8475294004122,22.6366145161376,17.0576060951706));
#27833=CARTESIAN_POINT('Ctrl Pts',(54.0511572360998,22.7560139947072,17.0435772240663));
#27834=CARTESIAN_POINT('Ctrl Pts',(54.113097599399,22.788096837687,17.0393578806663));
#27835=CARTESIAN_POINT('Ctrl Pts',(54.1894605549981,22.8227049086856,17.0341442132824));
#27836=CARTESIAN_POINT('Ctrl Pts',(54.2023969634172,22.8284027882109,17.0332606849461));
#27837=CARTESIAN_POINT('Ctrl Pts',(54.2238692035841,22.8375890601044,17.0317931618583));
#27838=CARTESIAN_POINT('Ctrl Pts',(54.2323707497069,22.8411566735212,17.0312118631701));
#27839=CARTESIAN_POINT('Ctrl Pts',(54.2478000530563,22.8475060298456,17.0301562682346));
#27840=CARTESIAN_POINT('Ctrl Pts',(54.2547193117933,22.8503080780797,17.0296826686529));
#27841=CARTESIAN_POINT('Ctrl Pts',(54.2696106760838,22.8562414596052,17.028662859584));
#27842=CARTESIAN_POINT('Ctrl Pts',(54.2775875237172,22.8593604091688,17.0281162449008));
#27843=CARTESIAN_POINT('Ctrl Pts',(54.2994661794092,22.8677529271903,17.0266159645061));
#27844=CARTESIAN_POINT('Ctrl Pts',(54.3134070308409,22.8729225039108,17.0256588526289));
#27845=CARTESIAN_POINT('Ctrl Pts',(54.3907645191626,22.9006286356879,17.0203404472342));
#27846=CARTESIAN_POINT('Ctrl Pts',(54.4552258628825,22.920098034461,17.0158790951855));
#27847=CARTESIAN_POINT('Ctrl Pts',(54.6821159162959,22.976280384899,17.0000704083081));
#27848=CARTESIAN_POINT('Ctrl Pts',(54.8480585653068,22.9959051086786,16.9882598562966));
#27849=CARTESIAN_POINT('Ctrl Pts',(55.0645299534269,22.9943342479137,16.973410028092));
#27850=CARTESIAN_POINT('Ctrl Pts',(55.1145566822883,22.9920869813143,16.9700231672771));
#27851=CARTESIAN_POINT('Ctrl Pts',(55.164448352281,22.9879598340842,16.9667227887628));
#27852=CARTESIAN_POINT('',(53.0052507533592,21.0011686008279,17.0195584283291));
#27853=CARTESIAN_POINT('Ctrl Pts',(55.1644482145651,22.9879598454764,16.809768216174));
#27854=CARTESIAN_POINT('Ctrl Pts',(55.1270233745594,22.9910557068607,16.8123653746829));
#27855=CARTESIAN_POINT('Ctrl Pts',(55.0895069287072,22.9930950923982,16.8149786665284));
#27856=CARTESIAN_POINT('Ctrl Pts',(54.9277669391599,22.9973082404018,16.8262571771688));
#27857=CARTESIAN_POINT('Ctrl Pts',(54.8035490652872,22.988936975352,16.8349678322256));
#27858=CARTESIAN_POINT('Ctrl Pts',(54.6654731627478,22.9665614313119,16.8442306065549));
#27859=CARTESIAN_POINT('Ctrl Pts',(54.6500672154177,22.963878598751,16.8452578452758));
#27860=CARTESIAN_POINT('Ctrl Pts',(54.6284699684782,22.9598553719831,16.8466876038589));
#27861=CARTESIAN_POINT('Ctrl Pts',(54.622251540512,22.9586663185466,16.8470980647222));
#27862=CARTESIAN_POINT('Ctrl Pts',(54.6122032007223,22.9566952963273,16.8477592606505));
#27863=CARTESIAN_POINT('Ctrl Pts',(54.6083698031279,22.9559316526256,16.8480110165315));
#27864=CARTESIAN_POINT('Ctrl Pts',(54.6002653966804,22.954292408274,16.8485422004317));
#27865=CARTESIAN_POINT('Ctrl Pts',(54.5959949664327,22.9534140635474,16.8488214653095));
#27866=CARTESIAN_POINT('Ctrl Pts',(54.5854385510223,22.9512067154736,16.8495103189212));
#27867=CARTESIAN_POINT('Ctrl Pts',(54.5791559770559,22.9498613162404,16.8499189821482));
#27868=CARTESIAN_POINT('Ctrl Pts',(54.5558104933033,22.944743841768,16.8514330581171));
#27869=CARTESIAN_POINT('Ctrl Pts',(54.5387902910449,22.9407778290165,16.8525279889959));
#27870=CARTESIAN_POINT('Ctrl Pts',(54.4959850095967,22.9302084850896,16.8552642067769));
#27871=CARTESIAN_POINT('Ctrl Pts',(54.4702752776269,22.9233116659363,16.8568915066384));
#27872=CARTESIAN_POINT('Ctrl Pts',(54.2791252386108,22.867910245082,16.8689215851795));
#27873=CARTESIAN_POINT('Ctrl Pts',(54.1204494749173,22.7986525842951,16.8785794332166));
#27874=CARTESIAN_POINT('Ctrl Pts',(53.9072096408508,22.6705282122025,16.8933090557485));
#27875=CARTESIAN_POINT('Ctrl Pts',(53.8440912404547,22.6274913894997,16.8979143554293));
#27876=CARTESIAN_POINT('Ctrl Pts',(53.7721360340915,22.5721281151553,16.9035575948327));
#27877=CARTESIAN_POINT('Ctrl Pts',(53.7607701400038,22.5631845911631,16.9044612488006));
#27878=CARTESIAN_POINT('Ctrl Pts',(53.7422425684839,22.5482766685299,16.905955190256));
#27879=CARTESIAN_POINT('Ctrl Pts',(53.7350235306683,22.5423841694385,16.9065426062463));
#27880=CARTESIAN_POINT('Ctrl Pts',(53.7220918787951,22.5316769267259,16.9076046421431));
#27881=CARTESIAN_POINT('Ctrl Pts',(53.7163644909864,22.5268802348656,16.9080785243193));
#27882=CARTESIAN_POINT('Ctrl Pts',(53.7044268244303,22.5167677912694,16.9090737030635));
#27883=CARTESIAN_POINT('Ctrl Pts',(53.6982220187961,22.5114458211461,16.9095952498259));
#27884=CARTESIAN_POINT('Ctrl Pts',(53.6816560379525,22.4970592105694,16.9109993828928));
#27885=CARTESIAN_POINT('Ctrl Pts',(53.6713558472513,22.4879253280386,16.9118848323158));
#27886=CARTESIAN_POINT('Ctrl Pts',(53.6488121421553,22.4675135456373,16.9138507936399));
#27887=CARTESIAN_POINT('Ctrl Pts',(53.6366136964173,22.4561876229523,16.9149332907983));
#27888=CARTESIAN_POINT('Ctrl Pts',(53.6002464329836,22.4215640562012,16.9182182046268));
#27889=CARTESIAN_POINT('Ctrl Pts',(53.5765235694982,22.3978086588392,16.9204397750863));
#27890=CARTESIAN_POINT('Ctrl Pts',(53.4908320714251,22.3075551326671,16.9287647626614));
#27891=CARTESIAN_POINT('Ctrl Pts',(53.4328362517925,22.237450121718,16.9350150246275));
#27892=CARTESIAN_POINT('Ctrl Pts',(53.2974014799077,22.0488804840534,16.9511623833349));
#27893=CARTESIAN_POINT('Ctrl Pts',(53.2273978641206,21.92567777455,16.961131717472));
#27894=CARTESIAN_POINT('Ctrl Pts',(53.1651243630623,21.7826082134327,16.9714511792834));
#27895=CARTESIAN_POINT('Ctrl Pts',(53.1593992663036,21.7690469351358,16.9724172569298));
#27896=CARTESIAN_POINT('Ctrl Pts',(53.1517150514553,21.7502675131983,16.9737372671607));
#27897=CARTESIAN_POINT('Ctrl Pts',(53.1496270661421,21.7451030799978,16.9740984357724));
#27898=CARTESIAN_POINT('Ctrl Pts',(53.1460864180662,21.7362389488729,16.9747151061792));
#27899=CARTESIAN_POINT('Ctrl Pts',(53.1446231426043,21.7325435665087,16.9749712322888));
#27900=CARTESIAN_POINT('Ctrl Pts',(53.1416012497567,21.72484488184,16.9755027967752));
#27901=CARTESIAN_POINT('Ctrl Pts',(53.1400445107646,21.7208408951201,16.9757781135687));
#27902=CARTESIAN_POINT('Ctrl Pts',(53.1363078168127,21.7111372905205,16.9764426437643));
#27903=CARTESIAN_POINT('Ctrl Pts',(53.1341410337677,21.7054325765969,16.9768310753747));
#27904=CARTESIAN_POINT('Ctrl Pts',(53.1266220836563,21.6853596369317,16.9781902681982));
#27905=CARTESIAN_POINT('Ctrl Pts',(53.1214092688239,21.6709393027526,16.9791531351863));
#27906=CARTESIAN_POINT('Ctrl Pts',(53.090322711761,21.5817399506995,16.9850342022889));
#27907=CARTESIAN_POINT('Ctrl Pts',(53.0687483153913,21.5055279359674,16.9897378428035));
#27908=CARTESIAN_POINT('Ctrl Pts',(53.0209256920076,21.2879566568982,17.0027834515498));
#27909=CARTESIAN_POINT('Ctrl Pts',(53.0053346483509,21.1447775937495,17.0109571210933));
#27910=CARTESIAN_POINT('Ctrl Pts',(53.0052503437261,21.0011710231689,17.0195575702349));
#27911=CARTESIAN_POINT('Ctrl Pts',(53.0052503422808,21.0011685585087,17.0195577178409));
#27912=CARTESIAN_POINT('Ctrl Pts',(53.0052282297145,20.9634220241211,17.0218183198799));
#27913=CARTESIAN_POINT('Ctrl Pts',(53.0062775294282,20.9256837997141,17.0241037505693));
#27914=CARTESIAN_POINT('Ctrl Pts',(53.0096914951773,20.8649765409554,17.0278357116731));
#27915=CARTESIAN_POINT('Ctrl Pts',(53.0113852710205,20.8419788892939,17.0292623188599));
#27916=CARTESIAN_POINT('Ctrl Pts',(53.0143580688015,20.8093486808741,17.0313069960328));
#27917=CARTESIAN_POINT('Ctrl Pts',(53.0153094101569,20.7996875896606,17.0319149414409));
#27918=CARTESIAN_POINT('Ctrl Pts',(53.0171097776151,20.7826784927092,17.0329899684286));
#27919=CARTESIAN_POINT('Ctrl Pts',(53.017929230875,20.7753274930776,17.0334561211071));
#27920=CARTESIAN_POINT('Ctrl Pts',(53.0196191109161,20.7608975871625,17.034374290602));
#27921=CARTESIAN_POINT('Ctrl Pts',(53.020486657703,20.7538184507588,17.0348262105417));
#27922=CARTESIAN_POINT('Ctrl Pts',(53.0222878775683,20.7397460872159,17.0357275702168));
#27923=CARTESIAN_POINT('Ctrl Pts',(53.0232207252282,20.7327528577128,17.0361769777382));
#27924=CARTESIAN_POINT('Ctrl Pts',(53.025776933553,20.7143358919914,17.0373644847243));
#27925=CARTESIAN_POINT('Ctrl Pts',(53.0274623303945,20.7029211697004,17.0381045310651));
#27926=CARTESIAN_POINT('Ctrl Pts',(53.0337741641412,20.6625971794646,17.0407334996856));
#27927=CARTESIAN_POINT('Ctrl Pts',(53.0389377224389,20.6337769892865,17.0426392514805));
#27928=CARTESIAN_POINT('Ctrl Pts',(53.0544905074254,20.5567740484736,17.0478058798917));
#27929=CARTESIAN_POINT('Ctrl Pts',(53.0660337898085,20.5088478201049,17.0511012989055));
#27930=CARTESIAN_POINT('Ctrl Pts',(53.1266152446108,20.2928123345647,17.0663141948278));
#27931=CARTESIAN_POINT('Ctrl Pts',(53.1958738204969,20.1312061570943,17.0787840294952));
#27932=CARTESIAN_POINT('Ctrl Pts',(53.3075152487275,19.9433976242558,17.0936528268165));
#27933=CARTESIAN_POINT('Ctrl Pts',(53.3309189772368,19.9068017566302,17.0965648605047));
#27934=CARTESIAN_POINT('Ctrl Pts',(53.3604553582758,19.8637792628891,17.0999802740345));
#27935=CARTESIAN_POINT('Ctrl Pts',(53.3654575988638,19.8565948481283,17.1005503368414));
#27936=CARTESIAN_POINT('Ctrl Pts',(53.3733166215605,19.8454643898302,17.1014327700867));
#27937=CARTESIAN_POINT('Ctrl Pts',(53.3761407612178,19.8414955922848,17.1017472728104));
#27938=CARTESIAN_POINT('Ctrl Pts',(53.381420996735,19.8341324579373,17.1023304202088));
#27939=CARTESIAN_POINT('Ctrl Pts',(53.3838732277932,19.8307355422858,17.1025993090487));
#27940=CARTESIAN_POINT('Ctrl Pts',(53.3894980944814,19.8229952831613,17.1032117089723));
#27941=CARTESIAN_POINT('Ctrl Pts',(53.3926776033082,19.8186570329224,17.1035547404343));
#27942=CARTESIAN_POINT('Ctrl Pts',(53.4010399306432,19.8073433962147,17.1044489393539));
#27943=CARTESIAN_POINT('Ctrl Pts',(53.4062509173405,19.8003888355234,17.1049982224616));
#27944=CARTESIAN_POINT('Ctrl Pts',(53.4423669258554,19.7528393008698,17.1087527985512));
#27945=CARTESIAN_POINT('Ctrl Pts',(53.4747769367784,19.7134051967517,17.1118618325421));
#27946=CARTESIAN_POINT('Ctrl Pts',(53.6215576721776,19.5481667098535,17.1250819054131));
#27947=CARTESIAN_POINT('Ctrl Pts',(53.7502330640489,19.4360264659343,17.1346223656856));
#27948=CARTESIAN_POINT('Ctrl Pts',(53.9287744385668,19.3166982308119,17.1474081622781));
#27949=CARTESIAN_POINT('Ctrl Pts',(53.9667934505477,19.2930984582603,17.1501039250887));
#27950=CARTESIAN_POINT('Ctrl Pts',(54.0232386120249,19.2606380225472,17.1540911993001));
#27951=CARTESIAN_POINT('Ctrl Pts',(54.041059514219,19.2507498758644,17.1553478977601));
#27952=CARTESIAN_POINT('Ctrl Pts',(54.0733735368401,19.2334622438081,17.1576248513136));
#27953=CARTESIAN_POINT('Ctrl Pts',(54.0878117648029,19.2259636854803,17.1586415890998));
#27954=CARTESIAN_POINT('Ctrl Pts',(54.1102094533104,19.2146770588854,17.1602186208604));
#27955=CARTESIAN_POINT('Ctrl Pts',(54.1181052242804,19.2107636205405,17.1607745244843));
#27956=CARTESIAN_POINT('Ctrl Pts',(54.126097447189,19.2068681317572,17.1613372440087));
#27957=CARTESIAN_POINT('Ctrl Pts',(54.1261683301154,19.2068335879165,17.1613422347632));
#27958=CARTESIAN_POINT('Ctrl Pts',(54.1263115822088,19.206763786447,17.16135232092));
#27959=CARTESIAN_POINT('Ctrl Pts',(54.1263839515305,19.2067285289625,17.1613574163333));
#27960=CARTESIAN_POINT('Ctrl Pts',(54.1265302143088,19.2066572824081,17.1613677144761));
#27961=CARTESIAN_POINT('Ctrl Pts',(54.1266041078101,19.2066212935464,17.1613729172089));
#27962=CARTESIAN_POINT('Ctrl Pts',(54.1267534577984,19.2065485660112,17.1613834327266));
#27963=CARTESIAN_POINT('Ctrl Pts',(54.1268289143291,19.2065118275573,17.1613887455146));
#27964=CARTESIAN_POINT('Ctrl Pts',(54.1269814301541,19.2064375821987,17.1613994839439));
#27965=CARTESIAN_POINT('Ctrl Pts',(54.1270584895868,19.2064000754788,17.161404909595));
#27966=CARTESIAN_POINT('Ctrl Pts',(54.1272142523196,19.2063242743443,17.1614158766449));
#27967=CARTESIAN_POINT('Ctrl Pts',(54.1272929557242,19.2062859801429,17.1614214180511));
#27968=CARTESIAN_POINT('Ctrl Pts',(54.1334147112952,19.2033078558133,17.1618524432571));
#27969=CARTESIAN_POINT('Ctrl Pts',(54.1394725171775,19.2003986071688,17.1622789821813));
#27970=CARTESIAN_POINT('Ctrl Pts',(54.1533654548371,19.1938127407448,17.1632573008765));
#27971=CARTESIAN_POINT('Ctrl Pts',(54.161210002858,19.1901564141182,17.1638097717616));
#27972=CARTESIAN_POINT('Ctrl Pts',(54.1826120144117,19.18035001467,17.1653173824498));
#27973=CARTESIAN_POINT('Ctrl Pts',(54.196214715213,19.1743005767348,17.1662759446621));
#27974=CARTESIAN_POINT('Ctrl Pts',(54.265604693008,19.1443670294446,17.1711685403789));
#27975=CARTESIAN_POINT('Ctrl Pts',(54.3223881671798,19.1228875648691,17.1751827828518));
#27976=CARTESIAN_POINT('Ctrl Pts',(54.5469272948283,19.049467937643,17.1911038657804));
#27977=CARTESIAN_POINT('Ctrl Pts',(54.7202659108089,19.0171775457291,17.2035801827156));
#27978=CARTESIAN_POINT('Ctrl Pts',(54.9484848791322,19.0052108601123,17.2192326395157));
#27979=CARTESIAN_POINT('Ctrl Pts',(55.0015162116316,19.0045460869513,17.2228082920327));
#27980=CARTESIAN_POINT('Ctrl Pts',(55.0637332178123,19.0062470905787,17.2268855274453));
#27981=CARTESIAN_POINT('Ctrl Pts',(55.0729489975857,19.006563008638,17.2274864112289));
#27982=CARTESIAN_POINT('Ctrl Pts',(55.0871297543628,19.0071476009795,17.2284059871015));
#27983=CARTESIAN_POINT('Ctrl Pts',(55.0920963248733,19.0073709460541,17.22872710234));
#27984=CARTESIAN_POINT('Ctrl Pts',(55.1012374127485,19.0078162676123,17.2293163079198));
#27985=CARTESIAN_POINT('Ctrl Pts',(55.1054120488351,19.0080327969816,17.2295846880311));
#27986=CARTESIAN_POINT('Ctrl Pts',(55.1148235951357,19.008550623565,17.2301881719018));
#27987=CARTESIAN_POINT('Ctrl Pts',(55.120060006064,19.0088594541408,17.2305228520609));
#27988=CARTESIAN_POINT('Ctrl Pts',(55.135482498669,19.0098300959499,17.231505522582));
#27989=CARTESIAN_POINT('Ctrl Pts',(55.1456649715014,19.010549452499,17.2321504037089));
#27990=CARTESIAN_POINT('Ctrl Pts',(55.2255554787207,19.0168101095267,17.2371824809964));
#27991=CARTESIAN_POINT('Ctrl Pts',(55.2949420943089,19.0259359612075,17.2413885968003));
#27992=CARTESIAN_POINT('Ctrl Pts',(55.5301343028818,19.069550926971,17.255509836364));
#27993=CARTESIAN_POINT('Ctrl Pts',(55.6919465233094,19.1214664013584,17.2650516446389));
#27994=CARTESIAN_POINT('Ctrl Pts',(55.8912991074485,19.2147279031276,17.2783045908966));
#27995=CARTESIAN_POINT('Ctrl Pts',(55.9364905981275,19.2380138331888,17.2814127320696));
#27996=CARTESIAN_POINT('Ctrl Pts',(55.9926286619352,19.2697103514369,17.2854328500481));
#27997=CARTESIAN_POINT('Ctrl Pts',(56.0044468267607,19.2765440284278,17.2862883594516));
#27998=CARTESIAN_POINT('Ctrl Pts',(56.0233326361246,19.2877246994094,17.2876708034926));
#27999=CARTESIAN_POINT('Ctrl Pts',(56.0304450579602,19.2919955010819,17.2881949719419));
#28000=CARTESIAN_POINT('Ctrl Pts',(56.0439400335977,19.300213811629,17.2891963846448));
#28001=CARTESIAN_POINT('Ctrl Pts',(56.0503273707911,19.3041532228507,17.2896733262955));
#28002=CARTESIAN_POINT('Ctrl Pts',(56.0648703657362,19.3132363420414,17.2907661182679));
#28003=CARTESIAN_POINT('Ctrl Pts',(56.0730112120985,19.3184032983662,17.2913828195811));
#28004=CARTESIAN_POINT('Ctrl Pts',(56.0941672214076,19.3320470927586,17.2929987012246));
#28005=CARTESIAN_POINT('Ctrl Pts',(56.1071211977915,19.3406171508883,17.2940013323799));
#28006=CARTESIAN_POINT('Ctrl Pts',(56.2288240594514,19.4231924622085,17.303549098214));
#28007=CARTESIAN_POINT('Ctrl Pts',(56.3300818856742,19.5076190556918,17.3125032713316));
#28008=CARTESIAN_POINT('Ctrl Pts',(56.4990739640982,19.6794696141971,17.329253380577));
#28009=CARTESIAN_POINT('Ctrl Pts',(56.5693067563976,19.7637553713725,17.3369560473026));
#28010=CARTESIAN_POINT('Ctrl Pts',(56.6581158761281,19.8901795060794,17.3474820975607));
#28011=CARTESIAN_POINT('Ctrl Pts',(56.6827155839725,19.9278438729621,17.350500671266));
#28012=CARTESIAN_POINT('Ctrl Pts',(56.7106030373156,19.9738699256933,17.3540233582064));
#28013=CARTESIAN_POINT('Ctrl Pts',(56.7151329768377,19.9814595936254,17.3545989923099));
#28014=CARTESIAN_POINT('Ctrl Pts',(56.7220902604696,19.9932941828284,17.3554881498165));
#28015=CARTESIAN_POINT('Ctrl Pts',(56.7245526280848,19.9975182287229,17.35580385691));
#28016=CARTESIAN_POINT('Ctrl Pts',(56.7290950245993,20.005376707975,17.3563880770171));
#28017=CARTESIAN_POINT('Ctrl Pts',(56.7311791244573,20.0090086091838,17.3566568425868));
#28018=CARTESIAN_POINT('Ctrl Pts',(56.7359012342226,20.0172980524552,17.3572674803803));
#28019=CARTESIAN_POINT('Ctrl Pts',(56.7385319412906,20.0219596616678,17.3576088838684));
#28020=CARTESIAN_POINT('Ctrl Pts',(56.7453421432941,20.0341416319052,17.3584960273213));
#28021=CARTESIAN_POINT('Ctrl Pts',(56.7494918565667,20.0416786371629,17.3590399310725));
#28022=CARTESIAN_POINT('Ctrl Pts',(56.7772000836354,20.0927841420803,17.3626960678013));
#28023=CARTESIAN_POINT('Ctrl Pts',(56.799179723665,20.1371941269563,17.3657175979258));
#28024=CARTESIAN_POINT('Ctrl Pts',(56.825032587595,20.1947256362167,17.3694950294889));
#28025=CARTESIAN_POINT('Ctrl Pts',(56.8304545148343,20.2071273568894,17.3703014121258));
#28026=CARTESIAN_POINT('Ctrl Pts',(56.888977488126,20.3447891594825,17.3791754100728));
#28027=CARTESIAN_POINT('Ctrl Pts',(56.9292577720349,20.4751145380018,17.3869001552498));
#28028=CARTESIAN_POINT('Ctrl Pts',(56.9717024110678,20.6871871098442,17.3996379146852));
#28029=CARTESIAN_POINT('Ctrl Pts',(56.9826844779074,20.7667138796778,17.4044450714505));
#28030=CARTESIAN_POINT('Ctrl Pts',(56.9904379101828,20.8672905262963,17.4106814756371));
#28031=CARTESIAN_POINT('Ctrl Pts',(56.9917062433862,20.8879238251917,17.4119688461712));
#28032=CARTESIAN_POINT('Ctrl Pts',(56.9931005896258,20.9183134770827,17.4138782126926));
#28033=CARTESIAN_POINT('Ctrl Pts',(56.9934760871349,20.9280574327564,17.4144924220295));
#28034=CARTESIAN_POINT('Ctrl Pts',(56.9940145442228,20.9453183233746,17.4155841670529));
#28035=CARTESIAN_POINT('Ctrl Pts',(56.9942064773797,20.9528342138752,17.4160607880231));
#28036=CARTESIAN_POINT('Ctrl Pts',(56.9945197054289,20.9685896442367,17.4170626046355));
#28037=CARTESIAN_POINT('Ctrl Pts',(56.9946324413719,20.9768291937568,17.4175880587941));
#28038=CARTESIAN_POINT('Ctrl Pts',(56.9947944057266,20.9984668341991,17.4189720913434));
#28039=CARTESIAN_POINT('Ctrl Pts',(56.9947597048359,21.0118649546367,17.4198332731779));
#28040=CARTESIAN_POINT('Ctrl Pts',(56.9940456106234,21.068248321421,17.4234756260347));
#28041=CARTESIAN_POINT('Ctrl Pts',(56.9921117113091,21.1112033659112,17.4262954821884));
#28042=CARTESIAN_POINT('Ctrl Pts',(56.9865147359738,21.1834559463117,17.4311177745792));
#28043=CARTESIAN_POINT('Ctrl Pts',(56.9835862190795,21.2127967441085,17.4330980854677));
#28044=CARTESIAN_POINT('Ctrl Pts',(56.9596587964209,21.4085182984303,17.4464515129929));
#28045=CARTESIAN_POINT('Ctrl Pts',(56.9184043192903,21.5717202820277,17.458360223942));
#28046=CARTESIAN_POINT('Ctrl Pts',(56.8381678069039,21.7764634803227,17.4734146017883));
#28047=CARTESIAN_POINT('Ctrl Pts',(56.8172023502372,21.8243379752131,17.4769366710391));
#28048=CARTESIAN_POINT('Ctrl Pts',(56.7903659012228,21.8796032744308,17.4809609988127));
#28049=CARTESIAN_POINT('Ctrl Pts',(56.7862953168531,21.8878406554434,17.4815597076296));
#28050=CARTESIAN_POINT('Ctrl Pts',(56.7799378063459,21.9004852103375,17.4824766670891));
#28051=CARTESIAN_POINT('Ctrl Pts',(56.7776911648896,21.9049123339151,17.4827973198358));
#28052=CARTESIAN_POINT('Ctrl Pts',(56.7735221463885,21.9130521548027,17.4833860891038));
#28053=CARTESIAN_POINT('Ctrl Pts',(56.771604634777,21.9167671785994,17.4836544922397));
#28054=CARTESIAN_POINT('Ctrl Pts',(56.7672509304274,21.9251374580231,17.4842585430835));
#28055=CARTESIAN_POINT('Ctrl Pts',(56.7648080212372,21.929789125036,17.4845937635503));
#28056=CARTESIAN_POINT('Ctrl Pts',(56.7584689293285,21.9417447173621,17.4854542599012));
#28057=CARTESIAN_POINT('Ctrl Pts',(56.7545455630325,21.9490342253862,17.4859778761507));
#28058=CARTESIAN_POINT('Ctrl Pts',(56.7298679116876,21.9942085004141,17.4892176432448));
#28059=CARTESIAN_POINT('Ctrl Pts',(56.7079312678399,22.0314382875009,17.4918650088071));
#28060=CARTESIAN_POINT('Ctrl Pts',(56.6706518018995,22.0902516273973,17.496058411627));
#28061=CARTESIAN_POINT('Ctrl Pts',(56.656059795806,22.112291373541,17.4976325065464));
#28062=CARTESIAN_POINT('Ctrl Pts',(56.5530661637046,22.2613308368027,17.5083409481435));
#28063=CARTESIAN_POINT('Ctrl Pts',(56.4505873391505,22.3779582975479,17.5170882911868));
#28064=CARTESIAN_POINT('Ctrl Pts',(56.2870519022641,22.5253875142597,17.53021665306));
#28065=CARTESIAN_POINT('Ctrl Pts',(56.23632679504,22.5667815379512,17.534188922913));
#28066=CARTESIAN_POINT('Ctrl Pts',(56.1717919965796,22.6143570207519,17.5391810022206));
#28067=CARTESIAN_POINT('Ctrl Pts',(56.1598244592822,22.622976364248,17.5401041941419));
#28068=CARTESIAN_POINT('Ctrl Pts',(56.1407803563322,22.6363742309858,17.5415698395245));
#28069=CARTESIAN_POINT('Ctrl Pts',(56.1337666460221,22.6412414916542,17.5421088927472));
#28070=CARTESIAN_POINT('Ctrl Pts',(56.1205615670358,22.6502803001597,17.5431225523562));
#28071=CARTESIAN_POINT('Ctrl Pts',(56.1143775855266,22.6544624169216,17.5435967470435));
#28072=CARTESIAN_POINT('Ctrl Pts',(56.1004775738827,22.6637494606909,17.544661566767));
#28073=CARTESIAN_POINT('Ctrl Pts',(56.0927492503656,22.668835590952,17.5452528837576));
#28074=CARTESIAN_POINT('Ctrl Pts',(56.0730328309638,22.6816155959624,17.5467597816189));
#28075=CARTESIAN_POINT('Ctrl Pts',(56.0609973484829,22.6892350570445,17.5476780928876));
#28076=CARTESIAN_POINT('Ctrl Pts',(55.9880687607172,22.7343180603892,17.5532343389441));
#28077=CARTESIAN_POINT('Ctrl Pts',(55.9252859664274,22.7686104150834,17.5579862155025));
#28078=CARTESIAN_POINT('Ctrl Pts',(55.7123592879946,22.8704679564178,17.5740010576374));
#28079=CARTESIAN_POINT('Ctrl Pts',(55.5557191482132,22.9228294359365,17.5856835241405));
#28080=CARTESIAN_POINT('Ctrl Pts',(55.343557311208,22.9656272243959,17.6004974378189));
#28081=CARTESIAN_POINT('Ctrl Pts',(55.2922877788073,22.9739024557423,17.6039965427397));
#28082=CARTESIAN_POINT('Ctrl Pts',(55.2316426747659,22.981275697247,17.607998169059));
#28083=CARTESIAN_POINT('Ctrl Pts',(55.2225284005698,22.9823200639648,17.6085959305618));
#28084=CARTESIAN_POINT('Ctrl Pts',(55.2084741055388,22.9838323329807,17.6095117502064));
#28085=CARTESIAN_POINT('Ctrl Pts',(55.2035391449796,22.9843447270625,17.6098322013106));
#28086=CARTESIAN_POINT('Ctrl Pts',(55.1944420827845,22.985254975888,17.6104207808997));
#28087=CARTESIAN_POINT('Ctrl Pts',(55.1902806623755,22.9856581561204,17.6106891946222));
#28088=CARTESIAN_POINT('Ctrl Pts',(55.1808830002383,22.9865388361046,17.6112934951304));
#28089=CARTESIAN_POINT('Ctrl Pts',(55.1756461292743,22.9870087181303,17.6116289530757));
#28090=CARTESIAN_POINT('Ctrl Pts',(55.1684213005163,22.9876281849431,17.6120900505316));
#28091=CARTESIAN_POINT('Ctrl Pts',(55.1664349523431,22.9877954982159,17.6122166442961));
#28092=CARTESIAN_POINT('Ctrl Pts',(55.1644483516309,22.987959834138,17.6123430797447));
#28093=CARTESIAN_POINT('Origin',(55.,21.,6.22095488139522));
#28094=CARTESIAN_POINT('',(55.1644483870895,22.9879598312048,18.5698477239299));
#28095=CARTESIAN_POINT('',(55.1644483276976,22.9879598361178,18.4096837786395));
#28096=CARTESIAN_POINT('',(55.1644483516311,22.987959834138,6.22095488139522));
#28097=CARTESIAN_POINT('',(53.005250018775,20.9997263157889,17.977164327174));
#28098=CARTESIAN_POINT('Ctrl Pts',(55.1644483870895,22.9879598312048,18.5698477239299));
#28099=CARTESIAN_POINT('Ctrl Pts',(55.2202125884814,22.9833468944481,18.5664985446111));
#28100=CARTESIAN_POINT('Ctrl Pts',(55.2757651209119,22.9763890857523,18.5630945022204));
#28101=CARTESIAN_POINT('Ctrl Pts',(55.345429404889,22.9646682653898,18.5587047603187));
#28102=CARTESIAN_POINT('Ctrl Pts',(55.3598716684571,22.9620742164863,18.557788148223));
#28103=CARTESIAN_POINT('Ctrl Pts',(55.3835013436058,22.9575603049037,18.5562770626812));
#28104=CARTESIAN_POINT('Ctrl Pts',(55.392706313787,22.9557344845718,18.5556855752152));
#28105=CARTESIAN_POINT('Ctrl Pts',(55.4092231058344,22.9523370458588,18.5546189895675));
#28106=CARTESIAN_POINT('Ctrl Pts',(55.4165396644161,22.9507891214737,18.5541446552504));
#28107=CARTESIAN_POINT('Ctrl Pts',(55.4321058374983,22.9474043074352,18.5531314494343));
#28108=CARTESIAN_POINT('Ctrl Pts',(55.4403528068018,22.9455560627577,18.5525922226949));
#28109=CARTESIAN_POINT('Ctrl Pts',(55.4625706111333,22.9404282850618,18.5511328271776));
#28110=CARTESIAN_POINT('Ctrl Pts',(55.4765179982505,22.9370503553693,18.5502095202972));
#28111=CARTESIAN_POINT('Ctrl Pts',(55.5481631395077,22.918877954508,18.5454287629383));
#28112=CARTESIAN_POINT('Ctrl Pts',(55.6052083342172,22.901656402103,18.5414937754309));
#28113=CARTESIAN_POINT('Ctrl Pts',(55.8080857904678,22.8303555804687,18.5270216142908));
#28114=CARTESIAN_POINT('Ctrl Pts',(55.9482365999881,22.7618286765473,18.5160567343815));
#28115=CARTESIAN_POINT('Ctrl Pts',(56.0848077522488,22.6739975041881,18.5048197954305));
#28116=CARTESIAN_POINT('Ctrl Pts',(56.0906118277199,22.6702219450827,18.5043412342372));
#28117=CARTESIAN_POINT('Ctrl Pts',(56.1156936467252,22.6537196992259,18.5022691095257));
#28118=CARTESIAN_POINT('Ctrl Pts',(56.1347696941903,22.6406885623914,18.5006826648513));
#28119=CARTESIAN_POINT('Ctrl Pts',(56.1905374747404,22.6011547035486,18.4960220325946));
#28120=CARTESIAN_POINT('Ctrl Pts',(56.2265612268519,22.5737293719741,18.4929814162581));
#28121=CARTESIAN_POINT('Ctrl Pts',(56.2681240496237,22.5397919946942,18.4894657435641));
#28122=CARTESIAN_POINT('Ctrl Pts',(56.2745911126011,22.5344430565401,18.4889184978524));
#28123=CARTESIAN_POINT('Ctrl Pts',(56.2850790040417,22.5256564145294,18.4880309224914));
#28124=CARTESIAN_POINT('Ctrl Pts',(56.2891201776302,22.5222433153131,18.4876889028458));
#28125=CARTESIAN_POINT('Ctrl Pts',(56.2963334785277,22.5161017711609,18.487078451632));
#28126=CARTESIAN_POINT('Ctrl Pts',(56.2995106313505,22.5133793933153,18.4868095917362));
#28127=CARTESIAN_POINT('Ctrl Pts',(56.306419722873,22.5074214622475,18.4862249701831));
#28128=CARTESIAN_POINT('Ctrl Pts',(56.3101482119455,22.5041820438922,18.4859094990922));
#28129=CARTESIAN_POINT('Ctrl Pts',(56.3206857875882,22.494957789727,18.4850178319057));
#28130=CARTESIAN_POINT('Ctrl Pts',(56.3274662671838,22.4889402471251,18.4844439955723));
#28131=CARTESIAN_POINT('Ctrl Pts',(56.3709811532486,22.4497880963588,18.4807589261419));
#28132=CARTESIAN_POINT('Ctrl Pts',(56.4065165324325,22.4153398879028,18.4777384577085));
#28133=CARTESIAN_POINT('Ctrl Pts',(56.5406647906645,22.2752471144406,18.466114250022));
#28134=CARTESIAN_POINT('Ctrl Pts',(56.6289641326701,22.1603382267268,18.457933684225));
#28135=CARTESIAN_POINT('Ctrl Pts',(56.7521688761919,21.9578573946524,18.4440097988615));
#28136=CARTESIAN_POINT('Ctrl Pts',(56.7946968886593,21.8755834700867,18.4384725327784));
#28137=CARTESIAN_POINT('Ctrl Pts',(56.8373387112217,21.7768149834651,18.4317913221677));
#28138=CARTESIAN_POINT('Ctrl Pts',(56.843159787831,21.7629004097895,18.4308495168397));
#28139=CARTESIAN_POINT('Ctrl Pts',(56.8523923454617,21.7401084879591,18.4293053128249));
#28140=CARTESIAN_POINT('Ctrl Pts',(56.8558991930661,21.7312702343236,18.4287061296352));
#28141=CARTESIAN_POINT('Ctrl Pts',(56.8620555756946,21.7154248465002,18.4276310888642));
#28142=CARTESIAN_POINT('Ctrl Pts',(56.8647290979311,21.7084271781865,18.4271560458992));
#28143=CARTESIAN_POINT('Ctrl Pts',(56.8703080200864,21.6935745189449,18.4261470872008));
#28144=CARTESIAN_POINT('Ctrl Pts',(56.8732034860626,21.6857159759003,18.4256128508302));
#28145=CARTESIAN_POINT('Ctrl Pts',(56.8808075065142,21.6646704084152,18.4241809628902));
#28146=CARTESIAN_POINT('Ctrl Pts',(56.8854267721292,21.6514518391507,18.4232803735629));
#28147=CARTESIAN_POINT('Ctrl Pts',(56.9074990060411,21.5860877360653,18.4188202022194));
#28148=CARTESIAN_POINT('Ctrl Pts',(56.922928281924,21.5332889833962,18.4151950318157));
#28149=CARTESIAN_POINT('Ctrl Pts',(56.986222630186,21.2779409735762,18.3975451254666));
#28150=CARTESIAN_POINT('Ctrl Pts',(57.0043675350158,21.06941396785,18.3826081914984));
#28151=CARTESIAN_POINT('Ctrl Pts',(56.9878730977885,20.8317792311816,18.3665679747899));
#28152=CARTESIAN_POINT('Ctrl Pts',(56.9851015121624,20.8017327510515,18.364561594309));
#28153=CARTESIAN_POINT('Ctrl Pts',(56.980713358151,20.7636336529914,18.3620546121964));
#28154=CARTESIAN_POINT('Ctrl Pts',(56.979727535631,20.7555141161702,18.3615224875028));
#28155=CARTESIAN_POINT('Ctrl Pts',(56.9780908080833,20.7426931011819,18.3606858942117));
#28156=CARTESIAN_POINT('Ctrl Pts',(56.9774730306547,20.7379875968981,18.3603796300042));
#28157=CARTESIAN_POINT('Ctrl Pts',(56.9763316031958,20.7295275866611,18.3598304533164));
#28158=CARTESIAN_POINT('Ctrl Pts',(56.9758140492738,20.7257724026701,18.3595872092326));
#28159=CARTESIAN_POINT('Ctrl Pts',(56.9745408872015,20.7167255415235,18.3590024230482));
#28160=CARTESIAN_POINT('Ctrl Pts',(56.9737747108645,20.7114354034022,18.3586614796522));
#28161=CARTESIAN_POINT('Ctrl Pts',(56.9713610039278,20.6952292231322,18.3576199293075));
#28162=CARTESIAN_POINT('Ctrl Pts',(56.9696440790612,20.6843235054932,18.3569230977361));
#28163=CARTESIAN_POINT('Ctrl Pts',(56.9497303468782,20.5643270280834,18.3492950633841));
#28164=CARTESIAN_POINT('Ctrl Pts',(56.9225786224382,20.4568996828676,18.3428184475189));
#28165=CARTESIAN_POINT('Ctrl Pts',(56.8339257917892,20.1986810104784,18.3269484744231));
#28166=CARTESIAN_POINT('Ctrl Pts',(56.7626484749413,20.0521286071546,18.3176222977082));
#28167=CARTESIAN_POINT('Ctrl Pts',(56.6619496819017,19.8966071660058,18.3062011074394));
#28168=CARTESIAN_POINT('Ctrl Pts',(56.6491672172954,19.877591913113,18.3047773687284));
#28169=CARTESIAN_POINT('Ctrl Pts',(56.6306855909202,19.8510960302802,18.3027525202415));
#28170=CARTESIAN_POINT('Ctrl Pts',(56.62525642031,19.8434286051115,18.3021616208862));
#28171=CARTESIAN_POINT('Ctrl Pts',(56.615693738953,19.830123867528,18.3011274610985));
#28172=CARTESIAN_POINT('Ctrl Pts',(56.6115843523806,19.8244693553302,18.3006851314795));
#28173=CARTESIAN_POINT('Ctrl Pts',(56.6029112088682,19.8126660734097,18.2997558291476));
#28174=CARTESIAN_POINT('Ctrl Pts',(56.5983416052488,19.8065217609895,18.2992686342007));
#28175=CARTESIAN_POINT('Ctrl Pts',(56.5873590699229,19.7919307901023,18.2981033663541));
#28176=CARTESIAN_POINT('Ctrl Pts',(56.5809139841092,19.7835087339296,18.2974240402795));
#28177=CARTESIAN_POINT('Ctrl Pts',(56.5587470114853,19.7550159351203,18.2951025025564));
#28178=CARTESIAN_POINT('Ctrl Pts',(56.5427081649495,19.7351960683515,18.2934477762744));
#28179=CARTESIAN_POINT('Ctrl Pts',(56.5032928554732,19.6883542950074,18.2894381428955));
#28180=CARTESIAN_POINT('Ctrl Pts',(56.4795623183198,19.6616431909438,18.28706941898));
#28181=CARTESIAN_POINT('Ctrl Pts',(56.319862845399,19.4913260526437,18.2714147125477));
#28182=CARTESIAN_POINT('Ctrl Pts',(56.1639299389151,19.3680133961798,18.2572811155302));
#28183=CARTESIAN_POINT('Ctrl Pts',(55.9577238662413,19.2497446771605,18.2411368997023));
#28184=CARTESIAN_POINT('Ctrl Pts',(55.9224194627306,19.2308839644028,18.2384575581676));
#28185=CARTESIAN_POINT('Ctrl Pts',(55.8786186609643,19.2091522745397,18.2352560130777));
#28186=CARTESIAN_POINT('Ctrl Pts',(55.8706420409106,19.2052608070149,18.2346778420237));
#28187=CARTESIAN_POINT('Ctrl Pts',(55.8581742485012,19.1992809638347,18.2337819990987));
#28188=CARTESIAN_POINT('Ctrl Pts',(55.8537009403369,19.197155915294,18.2334621466761));
#28189=CARTESIAN_POINT('Ctrl Pts',(55.8454347400095,19.1932667158331,18.2328740408688));
#28190=CARTESIAN_POINT('Ctrl Pts',(55.8416442331606,19.1914978448726,18.2326055068407));
#28191=CARTESIAN_POINT('Ctrl Pts',(55.8330630260706,19.1875261771249,18.2320001444627));
#28192=CARTESIAN_POINT('Ctrl Pts',(55.8282691473866,19.1853304474255,18.2316637508312));
#28193=CARTESIAN_POINT('Ctrl Pts',(55.8137451246246,19.1787475861821,18.2306498185943));
#28194=CARTESIAN_POINT('Ctrl Pts',(55.8039882351973,19.1744194314529,18.2299757700748));
#28195=CARTESIAN_POINT('Ctrl Pts',(55.7813582296454,19.1645973849098,18.2284276529297));
#28196=CARTESIAN_POINT('Ctrl Pts',(55.7684609545631,19.1591601841217,18.2275566643062));
#28197=CARTESIAN_POINT('Ctrl Pts',(55.7242738048925,19.141077217006,18.2246074913335));
#28198=CARTESIAN_POINT('Ctrl Pts',(55.6927193180748,19.1290893488974,18.2225606579838));
#28199=CARTESIAN_POINT('Ctrl Pts',(55.5183778678744,19.0678714553228,18.2114948815126));
#28200=CARTESIAN_POINT('Ctrl Pts',(55.3706537662896,19.0341774636865,18.2029643591093));
#28201=CARTESIAN_POINT('Ctrl Pts',(55.1355711628408,19.0080271136283,18.1890247390312));
#28202=CARTESIAN_POINT('Ctrl Pts',(55.0500986170244,19.0040483494604,18.1838906530859));
#28203=CARTESIAN_POINT('Ctrl Pts',(54.9497892416695,19.0058267161011,18.1776580658687));
#28204=CARTESIAN_POINT('Ctrl Pts',(54.9349412163163,19.0062558984568,18.1767303323942));
#28205=CARTESIAN_POINT('Ctrl Pts',(54.9106679695835,19.0072289517114,18.1752046208743));
#28206=CARTESIAN_POINT('Ctrl Pts',(54.9012391984114,19.0076739820777,18.1746097291929));
#28207=CARTESIAN_POINT('Ctrl Pts',(54.8843412544219,19.0085917985542,18.1735394184055));
#28208=CARTESIAN_POINT('Ctrl Pts',(54.8768708670858,19.0090397331067,18.1730647856077));
#28209=CARTESIAN_POINT('Ctrl Pts',(54.8610045068052,19.0100807408148,18.1720535309262));
#28210=CARTESIAN_POINT('Ctrl Pts',(54.852609434091,19.0106849362897,18.1715165694118));
#28211=CARTESIAN_POINT('Ctrl Pts',(54.8300695381513,19.012450598502,18.1700696687479));
#28212=CARTESIAN_POINT('Ctrl Pts',(54.8159330798686,19.0137099061572,18.1691566831818));
#28213=CARTESIAN_POINT('Ctrl Pts',(54.7446656905325,19.0208258890891,18.1645251761169));
#28214=CARTESIAN_POINT('Ctrl Pts',(54.6877982594137,19.0289965153539,18.1607348160656));
#28215=CARTESIAN_POINT('Ctrl Pts',(54.5214216863452,19.0602820491896,18.1493578524263));
#28216=CARTESIAN_POINT('Ctrl Pts',(54.4134219282403,19.0901665261438,18.1415873595785));
#28217=CARTESIAN_POINT('Ctrl Pts',(54.204424388932,19.1674061561086,18.1260456705321));
#28218=CARTESIAN_POINT('Ctrl Pts',(54.1037211095135,19.2144945524295,18.1183043979673));
#28219=CARTESIAN_POINT('Ctrl Pts',(53.9936629048854,19.2776278481176,18.1098988340941));
#28220=CARTESIAN_POINT('Ctrl Pts',(53.9799707464633,19.2857011524708,18.1088543676414));
#28221=CARTESIAN_POINT('Ctrl Pts',(53.9610134601336,19.2971864913064,18.107411577396));
#28222=CARTESIAN_POINT('Ctrl Pts',(53.9556661370826,19.3004607504565,18.1070049789038));
#28223=CARTESIAN_POINT('Ctrl Pts',(53.9467445197301,19.3059816185808,18.1063273403788));
#28224=CARTESIAN_POINT('Ctrl Pts',(53.9431618040958,19.3082144309057,18.106055417801));
#28225=CARTESIAN_POINT('Ctrl Pts',(53.9359489083239,19.3127414904947,18.105508420365));
#28226=CARTESIAN_POINT('Ctrl Pts',(53.9323189970091,19.3150361190162,18.1052333744081));
#28227=CARTESIAN_POINT('Ctrl Pts',(53.9249611539264,19.3197206629811,18.1046762671901));
#28228=CARTESIAN_POINT('Ctrl Pts',(53.9212337082464,19.3221113089179,18.1043942555766));
#28229=CARTESIAN_POINT('Ctrl Pts',(53.9122873276334,19.3278913226216,18.1037178310794));
#28230=CARTESIAN_POINT('Ctrl Pts',(53.9070761941631,19.3312927627624,18.1033241875757));
#28231=CARTESIAN_POINT('Ctrl Pts',(53.8680422959972,19.3570324758745,18.1003776665499));
#28232=CARTESIAN_POINT('Ctrl Pts',(53.8348888402359,19.3803744132371,18.0978866511344));
#28233=CARTESIAN_POINT('Ctrl Pts',(53.7264717610765,19.4617597363295,18.0896971088378));
#28234=CARTESIAN_POINT('Ctrl Pts',(53.6546436625375,19.5241692333759,18.0841941283589));
#28235=CARTESIAN_POINT('Ctrl Pts',(53.4888799811698,19.6903956552318,18.0705749288932));
#28236=CARTESIAN_POINT('Ctrl Pts',(53.40090425155,19.7994026292388,18.0624607386536));
#28237=CARTESIAN_POINT('Ctrl Pts',(53.311973076662,19.9369046592596,18.0523783459512));
#28238=CARTESIAN_POINT('Ctrl Pts',(53.2992721075174,19.9573441816079,18.05088428344));
#28239=CARTESIAN_POINT('Ctrl Pts',(53.2820303870684,19.9862446230175,18.0487757877934));
#28240=CARTESIAN_POINT('Ctrl Pts',(53.2771759181116,19.9945166669516,18.0481727405671));
#28241=CARTESIAN_POINT('Ctrl Pts',(53.2688625729294,20.0089196206766,18.0471233726622));
#28242=CARTESIAN_POINT('Ctrl Pts',(53.2653761151732,20.0150344748127,18.0466780540171));
#28243=CARTESIAN_POINT('Ctrl Pts',(53.2581841963012,20.0278049091693,18.045748379084));
#28244=CARTESIAN_POINT('Ctrl Pts',(53.2544843548618,20.0344635073783,18.0452638309936));
#28245=CARTESIAN_POINT('Ctrl Pts',(53.2458326394616,20.050246240761,18.0441156820576));
#28246=CARTESIAN_POINT('Ctrl Pts',(53.2409137129459,20.0593880928241,18.0434509238052));
#28247=CARTESIAN_POINT('Ctrl Pts',(53.224784615579,20.0899331561639,18.0412304976867));
#28248=CARTESIAN_POINT('Ctrl Pts',(53.2138923275532,20.1115009180208,18.0396637443223));
#28249=CARTESIAN_POINT('Ctrl Pts',(53.1889188276402,20.163266777723,18.0359042936883));
#28250=CARTESIAN_POINT('Ctrl Pts',(53.1751975650715,20.193629516267,18.0336999461982));
#28251=CARTESIAN_POINT('Ctrl Pts',(53.0963511761303,20.3804339800807,18.0201404974891));
#28252=CARTESIAN_POINT('Ctrl Pts',(53.0506263109386,20.5442951756006,18.0081741166929));
#28253=CARTESIAN_POINT('Ctrl Pts',(53.0183460487092,20.765471068342,17.9927254304657));
#28254=CARTESIAN_POINT('Ctrl Pts',(53.0127123528883,20.8193209261681,17.9890251584671));
#28255=CARTESIAN_POINT('Ctrl Pts',(53.0079015399726,20.8949310862832,17.9839693754571));
#28256=CARTESIAN_POINT('Ctrl Pts',(53.0068789659841,20.9165470964787,17.9825399757031));
#28257=CARTESIAN_POINT('Ctrl Pts',(53.0059889285599,20.9452505700444,17.9806667847098));
#28258=CARTESIAN_POINT('Ctrl Pts',(53.0058072219952,20.9523258885091,17.9802070541033));
#28259=CARTESIAN_POINT('Ctrl Pts',(53.0055702728741,20.9639658246103,17.9794541920673));
#28260=CARTESIAN_POINT('Ctrl Pts',(53.0054930359905,20.9685298589266,17.9791598692181));
#28261=CARTESIAN_POINT('Ctrl Pts',(53.0053776218438,20.9770856796647,17.9786098177043));
#28262=CARTESIAN_POINT('Ctrl Pts',(53.0053357599012,20.9810773405698,17.9783538897146));
#28263=CARTESIAN_POINT('Ctrl Pts',(53.0052817465577,20.9882932692173,17.9778924539535));
#28264=CARTESIAN_POINT('Ctrl Pts',(53.0052654298016,20.9915174903657,17.9776867142566));
#28265=CARTESIAN_POINT('Ctrl Pts',(53.0052525506544,20.9964032715986,17.9773755954274));
#28266=CARTESIAN_POINT('Ctrl Pts',(53.0052502467401,20.9980647900871,17.9772699057812));
#28267=CARTESIAN_POINT('Ctrl Pts',(53.005250018775,20.9997263157889,17.977164327174));
#28268=CARTESIAN_POINT('Ctrl Pts',(53.0052500188593,20.9997257026673,17.9771643661337));
#28269=CARTESIAN_POINT('Ctrl Pts',(53.0052494450772,21.0038983710389,17.9768992214964));
#28270=CARTESIAN_POINT('Ctrl Pts',(53.0052619640291,21.0080710814626,17.9766347773869));
#28271=CARTESIAN_POINT('Ctrl Pts',(53.0053538573503,21.0230420189037,17.9756884241139));
#28272=CARTESIAN_POINT('Ctrl Pts',(53.005507822225,21.0338398229537,17.9750103918437));
#28273=CARTESIAN_POINT('Ctrl Pts',(53.0071547221884,21.1074199519088,17.9704176544664));
#28274=CARTESIAN_POINT('Ctrl Pts',(53.0115242338651,21.1701089876393,17.9666413452699));
#28275=CARTESIAN_POINT('Ctrl Pts',(53.0387504349818,21.4021129147237,17.9528371188982));
#28276=CARTESIAN_POINT('Ctrl Pts',(53.0803544361884,21.5684703042354,17.9432174536033));
#28277=CARTESIAN_POINT('Ctrl Pts',(53.1612566031942,21.7750193040438,17.9298618881239));
#28278=CARTESIAN_POINT('Ctrl Pts',(53.1816851286079,21.8218044507097,17.926741108731));
#28279=CARTESIAN_POINT('Ctrl Pts',(53.2098315604115,21.8800633292514,17.9227065457421));
#28280=CARTESIAN_POINT('Ctrl Pts',(53.2159057361774,21.8923128087379,17.9218497314756));
#28281=CARTESIAN_POINT('Ctrl Pts',(53.2258698832391,21.911898470956,17.9204655842242));
#28282=CARTESIAN_POINT('Ctrl Pts',(53.2296806400684,21.9192746341561,17.9199410285296));
#28283=CARTESIAN_POINT('Ctrl Pts',(53.2370240187829,21.9332735882501,17.9189391422026));
#28284=CARTESIAN_POINT('Ctrl Pts',(53.2405481991838,21.9399006644069,17.9184621161182));
#28285=CARTESIAN_POINT('Ctrl Pts',(53.2486829115608,21.9549915760907,17.9173695054215));
#28286=CARTESIAN_POINT('Ctrl Pts',(53.2533175241753,21.96344215079,17.916753072165));
#28287=CARTESIAN_POINT('Ctrl Pts',(53.2655714428253,21.9854064195783,17.9151386657299));
#28288=CARTESIAN_POINT('Ctrl Pts',(53.2732873599082,21.9988651899356,17.9141372533314));
#28289=CARTESIAN_POINT('Ctrl Pts',(53.3472771587176,22.1245050057304,17.904671824096));
#28290=CARTESIAN_POINT('Ctrl Pts',(53.4242234170566,22.2300084939949,17.8958069767272));
#28291=CARTESIAN_POINT('Ctrl Pts',(53.5722309234845,22.3960669040283,17.8803521929355));
#28292=CARTESIAN_POINT('Ctrl Pts',(53.6382716916887,22.4605559430281,17.8738812392954));
#28293=CARTESIAN_POINT('Ctrl Pts',(53.7406474613458,22.5475251183407,17.8646335643374));
#28294=CARTESIAN_POINT('Ctrl Pts',(53.7736169143373,22.5737813678214,17.8617621345993));
#28295=CARTESIAN_POINT('Ctrl Pts',(53.8204541377859,22.6087151778961,17.8578529871092));
#28296=CARTESIAN_POINT('Ctrl Pts',(53.8336323024185,22.6182952129195,17.8567710266859));
#28297=CARTESIAN_POINT('Ctrl Pts',(53.8567349434588,22.634661141775,17.8549071425359));
#28298=CARTESIAN_POINT('Ctrl Pts',(53.8666059702485,22.6415206451121,17.8541209796374));
#28299=CARTESIAN_POINT('Ctrl Pts',(53.8810525446767,22.6513673107975,17.8529858737762));
#28300=CARTESIAN_POINT('Ctrl Pts',(53.8855790877041,22.6544254092883,17.8526323942762));
#28301=CARTESIAN_POINT('Ctrl Pts',(53.8934926366194,22.65972452833,17.8520182980648));
#28302=CARTESIAN_POINT('Ctrl Pts',(53.896873999554,22.6619738516238,17.8517571298189));
#28303=CARTESIAN_POINT('Ctrl Pts',(53.9040795682481,22.6667354032401,17.8512032186045));
#28304=CARTESIAN_POINT('Ctrl Pts',(53.9079055554001,22.6692448059649,17.8509106628627));
#28305=CARTESIAN_POINT('Ctrl Pts',(53.9180341847305,22.6758382794084,17.8501401838109));
#28306=CARTESIAN_POINT('Ctrl Pts',(53.9243513879879,22.6799000065192,17.8496637194643));
#28307=CARTESIAN_POINT('Ctrl Pts',(53.9520022329641,22.6974585470658,17.8475952425497));
#28308=CARTESIAN_POINT('Ctrl Pts',(53.9735691118003,22.710586042899,17.8460258710962));
#28309=CARTESIAN_POINT('Ctrl Pts',(54.1798420557591,22.8308353659649,17.8313698557903));
#28310=CARTESIAN_POINT('Ctrl Pts',(54.3803894157015,22.9080688046697,17.8196276533187));
#28311=CARTESIAN_POINT('Ctrl Pts',(54.6435865608881,22.963431601144,17.8034844103809));
#28312=CARTESIAN_POINT('Ctrl Pts',(54.6982247080355,22.9725681278073,17.8001057467596));
#28313=CARTESIAN_POINT('Ctrl Pts',(54.7670941439632,22.9811560661568,17.7957802291301));
#28314=CARTESIAN_POINT('Ctrl Pts',(54.7810372469934,22.982745519,17.794901152001));
#28315=CARTESIAN_POINT('Ctrl Pts',(54.8033331284136,22.9850491074886,17.7934896356091));
#28316=CARTESIAN_POINT('Ctrl Pts',(54.8116758145035,22.9858579544376,17.7929601765003));
#28317=CARTESIAN_POINT('Ctrl Pts',(54.8274824888452,22.9872899556359,17.791954464385));
#28318=CARTESIAN_POINT('Ctrl Pts',(54.834945391041,22.9879236989832,17.7914785527464));
#28319=CARTESIAN_POINT('Ctrl Pts',(54.8518789490896,22.9892656711317,17.7903961697416));
#28320=CARTESIAN_POINT('Ctrl Pts',(54.8613513944569,22.9899483197032,17.7897889072776));
#28321=CARTESIAN_POINT('Ctrl Pts',(54.8858414105554,22.9915375276376,17.7882141125563));
#28322=CARTESIAN_POINT('Ctrl Pts',(54.9008647894016,22.9923418624736,17.7872434114754));
#28323=CARTESIAN_POINT('Ctrl Pts',(54.9987883104993,22.9964742798257,17.7808848360862));
#28324=CARTESIAN_POINT('Ctrl Pts',(55.0817996358081,22.9947967157224,17.7753425660883));
#28325=CARTESIAN_POINT('Ctrl Pts',(55.1644483624361,22.9879598332441,17.7696788290115));
#28326=CARTESIAN_POINT('Ctrl Pts',(55.1644483516309,22.987959834138,17.6123430797447));
#28327=CARTESIAN_POINT('Ctrl Pts',(55.1562045015407,22.9886417833077,17.6128677523061));
#28328=CARTESIAN_POINT('Ctrl Pts',(55.1479563026721,22.9892724618085,17.6133896986423));
#28329=CARTESIAN_POINT('Ctrl Pts',(55.0677606366728,22.9949028679997,17.6184373849476));
#28330=CARTESIAN_POINT('Ctrl Pts',(54.9955872414676,22.9960490787526,17.6227690321975));
#28331=CARTESIAN_POINT('Ctrl Pts',(54.8040372429016,22.988697859225,17.6340712088978));
#28332=CARTESIAN_POINT('Ctrl Pts',(54.6852244011128,22.9733824803268,17.6408932882945));
#28333=CARTESIAN_POINT('Ctrl Pts',(54.4852692573094,22.9290791790024,17.6529245798835));
#28334=CARTESIAN_POINT('Ctrl Pts',(54.4033195040415,22.9053251999907,17.6580186770147));
#28335=CARTESIAN_POINT('Ctrl Pts',(54.3030787995379,22.8691665230097,17.6646019813089));
#28336=CARTESIAN_POINT('Ctrl Pts',(54.2831296890994,22.8616067127958,17.6659298580941));
#28337=CARTESIAN_POINT('Ctrl Pts',(54.2541292348581,22.8500815880836,17.6678880000106));
#28338=CARTESIAN_POINT('Ctrl Pts',(54.2449795764475,22.8463664953737,17.668509886183));
#28339=CARTESIAN_POINT('Ctrl Pts',(54.2288974532969,22.8396970421661,17.6696103633674));
#28340=CARTESIAN_POINT('Ctrl Pts',(54.2219533876263,22.8367710284402,17.6700879885599));
#28341=CARTESIAN_POINT('Ctrl Pts',(54.2075044672345,22.830586063314,17.6710870168727));
#28342=CARTESIAN_POINT('Ctrl Pts',(54.2000027644792,22.8273201483388,17.6716086499419));
#28343=CARTESIAN_POINT('Ctrl Pts',(54.1805134167674,22.8186923198195,17.6729716623769));
#28344=CARTESIAN_POINT('Ctrl Pts',(54.1685584088082,22.8132580845056,17.6738155028113));
#28345=CARTESIAN_POINT('Ctrl Pts',(54.1197620705901,22.7904933282162,17.6772922870721));
#28346=CARTESIAN_POINT('Ctrl Pts',(54.0834040458055,22.7721559259544,17.6799596723616));
#28347=CARTESIAN_POINT('Ctrl Pts',(53.9238312740723,22.6854497877812,17.6920224988731));
#28348=CARTESIAN_POINT('Ctrl Pts',(53.8075206808867,22.6052606332593,17.701825405699));
#28349=CARTESIAN_POINT('Ctrl Pts',(53.6250892957,22.4486422179421,17.7185907525939));
#28350=CARTESIAN_POINT('Ctrl Pts',(53.5544889031656,22.3782036715191,17.7255086726988));
#28351=CARTESIAN_POINT('Ctrl Pts',(53.4782604843642,22.2898175871467,17.7332500684554));
#28352=CARTESIAN_POINT('Ctrl Pts',(53.4672480082366,22.2767113772083,17.7343756775415));
#28353=CARTESIAN_POINT('Ctrl Pts',(53.4523683839545,22.2585327019815,17.7359047365575));
#28354=CARTESIAN_POINT('Ctrl Pts',(53.448355185388,22.253581490339,17.7363179793279));
#28355=CARTESIAN_POINT('Ctrl Pts',(53.4416433816397,22.2452193090097,17.7370103967235));
#28356=CARTESIAN_POINT('Ctrl Pts',(53.4389321025213,22.2418186252974,17.7372904643731));
#28357=CARTESIAN_POINT('Ctrl Pts',(53.4337996127573,22.2353377104096,17.7378212816247));
#28358=CARTESIAN_POINT('Ctrl Pts',(53.4313763284458,22.2322591811168,17.738072183426));
#28359=CARTESIAN_POINT('Ctrl Pts',(53.4250302557155,22.2241481042436,17.7387300372019));
#28360=CARTESIAN_POINT('Ctrl Pts',(53.4211224777992,22.219103789306,17.7391359345444));
#28361=CARTESIAN_POINT('Ctrl Pts',(53.4075409594136,22.2013973826035,17.7405498094826));
#28362=CARTESIAN_POINT('Ctrl Pts',(53.3979944938757,22.188637818215,17.7415493208835));
#28363=CARTESIAN_POINT('Ctrl Pts',(53.3233700787058,22.0863642451851,17.749420566706));
#28364=CARTESIAN_POINT('Ctrl Pts',(53.2656825385003,21.9916776715775,17.7558701204304));
#28365=CARTESIAN_POINT('Ctrl Pts',(53.1659830209991,21.792447182916,17.7688056194371));
#28366=CARTESIAN_POINT('Ctrl Pts',(53.1243633307069,21.688168563644,17.7752727116892));
#28367=CARTESIAN_POINT('Ctrl Pts',(53.0749785239509,21.5259515459231,17.7854357337141));
#28368=CARTESIAN_POINT('Ctrl Pts',(53.0606218528491,21.4702596896598,17.78893955973));
#28369=CARTESIAN_POINT('Ctrl Pts',(53.0457447154624,21.4001441262871,17.7934057894077));
#28370=CARTESIAN_POINT('Ctrl Pts',(53.0429469182247,21.3862282454544,17.794294799184));
#28371=CARTESIAN_POINT('Ctrl Pts',(53.0387272992062,21.3640161793848,17.795718427982));
#28372=CARTESIAN_POINT('Ctrl Pts',(53.0372090268368,21.3557386370439,17.7962499738281));
#28373=CARTESIAN_POINT('Ctrl Pts',(53.0344400697943,21.3400848337445,17.7972572138348));
#28374=CARTESIAN_POINT('Ctrl Pts',(53.0331784118291,21.3327106418171,17.7977325503167));
#28375=CARTESIAN_POINT('Ctrl Pts',(53.0304196251321,21.3160216987476,17.7988103008251));
#28376=CARTESIAN_POINT('Ctrl Pts',(53.028947044128,21.3067031255748,17.7994134810618));
#28377=CARTESIAN_POINT('Ctrl Pts',(53.0253279823429,21.2826982085954,17.8009710425391));
#28378=CARTESIAN_POINT('Ctrl Pts',(53.0232792450156,21.2679979319093,17.8019284794512));
#28379=CARTESIAN_POINT('Ctrl Pts',(53.0105718795586,21.168727525581,17.8084195391141));
#28380=CARTESIAN_POINT('Ctrl Pts',(53.0051808167741,21.0835833700158,17.814117348025));
#28381=CARTESIAN_POINT('Ctrl Pts',(53.0053221874591,20.9111163160786,17.8259064425452));
#28382=CARTESIAN_POINT('Ctrl Pts',(53.011117899514,20.8239711767105,17.8319914019213));
#28383=CARTESIAN_POINT('Ctrl Pts',(53.0362352718391,20.6347694196324,17.8453021719777));
#28384=CARTESIAN_POINT('Ctrl Pts',(53.0578570235185,20.5332556518522,17.8525094658393));
#28385=CARTESIAN_POINT('Ctrl Pts',(53.0917985374451,20.4185800854817,17.8604324808444));
#28386=CARTESIAN_POINT('Ctrl Pts',(53.096508475266,20.4033409746875,17.861480581088));
#28387=CARTESIAN_POINT('Ctrl Pts',(53.1033587664401,20.382083873452,17.862934291384));
#28388=CARTESIAN_POINT('Ctrl Pts',(53.105345853607,20.376017647246,17.8633481905447));
#28389=CARTESIAN_POINT('Ctrl Pts',(53.1085996399528,20.366243269563,17.8640134398983));
#28390=CARTESIAN_POINT('Ctrl Pts',(53.1098481853777,20.3625291899305,17.8642658345858));
#28391=CARTESIAN_POINT('Ctrl Pts',(53.1125054868191,20.3547008941483,17.8647969611761));
#28392=CARTESIAN_POINT('Ctrl Pts',(53.1139167669824,20.3505875639856,17.8650755365102));
#28393=CARTESIAN_POINT('Ctrl Pts',(53.1174286831053,20.3404597164924,17.8657602819341));
#28394=CARTESIAN_POINT('Ctrl Pts',(53.1195447246738,20.3344505210533,17.8661655510608));
#28395=CARTESIAN_POINT('Ctrl Pts',(53.1274463675306,20.3123497530297,17.8676526786476));
#28396=CARTESIAN_POINT('Ctrl Pts',(53.1334102185185,20.2963220888684,17.868724533539));
#28397=CARTESIAN_POINT('Ctrl Pts',(53.1754252388377,20.187702567236,17.8759560006637));
#28398=CARTESIAN_POINT('Ctrl Pts',(53.2181494670196,20.0978283067108,17.8817815184293));
#28399=CARTESIAN_POINT('Ctrl Pts',(53.3493547384341,19.8678564877928,17.8971798982329));
#28400=CARTESIAN_POINT('Ctrl Pts',(53.4488439872008,19.7349752051024,17.9066644753506));
#28401=CARTESIAN_POINT('Ctrl Pts',(53.5780304856674,19.6009061297597,17.9181448238755));
#28402=CARTESIAN_POINT('Ctrl Pts',(53.5927089817492,19.5861425471189,17.9194379305167));
#28403=CARTESIAN_POINT('Ctrl Pts',(53.6155882352154,19.5638399828379,17.9214381078498));
#28404=CARTESIAN_POINT('Ctrl Pts',(53.6236258274172,19.5561351661683,17.9221379533497));
#28405=CARTESIAN_POINT('Ctrl Pts',(53.6368073602356,19.543709463285,17.9232813597396));
#28406=CARTESIAN_POINT('Ctrl Pts',(53.6419123990199,19.5389475141249,17.9237231479039));
#28407=CARTESIAN_POINT('Ctrl Pts',(53.6526718425486,19.5290162844542,17.9246521637944));
#28408=CARTESIAN_POINT('Ctrl Pts',(53.658331230077,19.5238525939511,17.9251396180283));
#28409=CARTESIAN_POINT('Ctrl Pts',(53.6719178870085,19.5115986510805,17.9263070973087));
#28410=CARTESIAN_POINT('Ctrl Pts',(53.6798723257742,19.5045390039179,17.9269883891786));
#28411=CARTESIAN_POINT('Ctrl Pts',(53.7072329406929,19.4806445791536,17.9293245609996));
#28412=CARTESIAN_POINT('Ctrl Pts',(53.7269070304031,19.4641218300135,17.9309921727932));
#28413=CARTESIAN_POINT('Ctrl Pts',(53.7749703286756,19.4253152597557,17.9350389534557));
#28414=CARTESIAN_POINT('Ctrl Pts',(53.8036550615148,19.4034135649357,17.9374322816553));
#28415=CARTESIAN_POINT('Ctrl Pts',(53.9984469996218,19.2628814157508,17.9535434791861));
#28416=CARTESIAN_POINT('Ctrl Pts',(54.1812864394909,19.1695972228511,17.9681701016849));
#28417=CARTESIAN_POINT('Ctrl Pts',(54.4072482774499,19.0950535110198,17.9842474096289));
#28418=CARTESIAN_POINT('Ctrl Pts',(54.4396947113639,19.0852587539316,17.9865069636685));
#28419=CARTESIAN_POINT('Ctrl Pts',(54.480492657853,19.0740689264257,17.9892743459269));
#28420=CARTESIAN_POINT('Ctrl Pts',(54.4886223565755,19.0718943777495,17.9898221735318));
#28421=CARTESIAN_POINT('Ctrl Pts',(54.5014555291512,19.0685486125408,17.9906809883666));
#28422=CARTESIAN_POINT('Ctrl Pts',(54.5061498145874,19.0673430084171,17.990993884413));
#28423=CARTESIAN_POINT('Ctrl Pts',(54.5148747243736,19.065136108919,17.9915730569207));
#28424=CARTESIAN_POINT('Ctrl Pts',(54.5189040459838,19.0641303004787,17.9918395807374));
#28425=CARTESIAN_POINT('Ctrl Pts',(54.528172512234,19.0618474099565,17.9924505047803));
#28426=CARTESIAN_POINT('Ctrl Pts',(54.5334137106305,19.0605789841502,17.9927944062752));
#28427=CARTESIAN_POINT('Ctrl Pts',(54.549640293066,19.0567215650556,17.9938544513704));
#28428=CARTESIAN_POINT('Ctrl Pts',(54.5606427811524,19.0542044841279,17.9945666211606));
#28429=CARTESIAN_POINT('Ctrl Pts',(54.6663645224537,19.030960599864,18.0013518295103));
#28430=CARTESIAN_POINT('Ctrl Pts',(54.7624683906608,19.017069679181,18.007077724491));
#28431=CARTESIAN_POINT('Ctrl Pts',(55.0302602034514,18.9981220000316,18.0227330081393));
#28432=CARTESIAN_POINT('Ctrl Pts',(55.202135997427,19.0081245413483,18.032509369554));
#28433=CARTESIAN_POINT('Ctrl Pts',(55.3959612922766,19.0447742476639,18.0446333951751));
#28434=CARTESIAN_POINT('Ctrl Pts',(55.4212135645324,19.0500584301943,18.0462332173317));
#28435=CARTESIAN_POINT('Ctrl Pts',(55.4570432278468,19.0582844437768,18.0485352313109));
#28436=CARTESIAN_POINT('Ctrl Pts',(55.4677104729348,19.060826279257,18.0492246675227));
#28437=CARTESIAN_POINT('Ctrl Pts',(55.4857795428145,19.0652896162356,18.0503996564562));
#28438=CARTESIAN_POINT('Ctrl Pts',(55.4931923447348,19.0671659818529,18.05088374976));
#28439=CARTESIAN_POINT('Ctrl Pts',(55.5081550219907,19.0710450896589,18.0518651320567));
#28440=CARTESIAN_POINT('Ctrl Pts',(55.5157042836134,19.0730496473672,18.0523624722264));
#28441=CARTESIAN_POINT('Ctrl Pts',(55.5342447022756,19.0780894460937,18.0535894009449));
#28442=CARTESIAN_POINT('Ctrl Pts',(55.5452218722551,19.0811746613631,18.0543205975186));
#28443=CARTESIAN_POINT('Ctrl Pts',(55.5856651498453,19.0929166052565,18.0570325855697));
#28444=CARTESIAN_POINT('Ctrl Pts',(55.6149553597626,19.102158996729,18.0590322851738));
#28445=CARTESIAN_POINT('Ctrl Pts',(55.8126117461888,19.1695845628228,18.0727779922741));
#28446=CARTESIAN_POINT('Ctrl Pts',(55.9727162279006,19.2494122324784,18.0852707420328));
#28447=CARTESIAN_POINT('Ctrl Pts',(56.1908819300966,19.3974541575924,18.1035854257354));
#28448=CARTESIAN_POINT('Ctrl Pts',(56.2585466056439,19.4500268158847,18.1094643958355));
#28449=CARTESIAN_POINT('Ctrl Pts',(56.3304248252236,19.5136939228655,18.1157699205793));
#28450=CARTESIAN_POINT('Ctrl Pts',(56.3381649037691,19.5206587033246,18.1164497107711));
#28451=CARTESIAN_POINT('Ctrl Pts',(56.3497541224738,19.5312524568443,18.1174682865368));
#28452=CARTESIAN_POINT('Ctrl Pts',(56.3536438009291,19.5348365284269,18.1178102751639));
#28453=CARTESIAN_POINT('Ctrl Pts',(56.3605839747286,19.5412826504657,18.1184206194939));
#28454=CARTESIAN_POINT('Ctrl Pts',(56.363639755466,19.5441388539873,18.1186894037461));
#28455=CARTESIAN_POINT('Ctrl Pts',(56.3702825341245,19.5503870482726,18.1192737953573));
#28456=CARTESIAN_POINT('Ctrl Pts',(56.373865926059,19.553782743973,18.1195891127425));
#28457=CARTESIAN_POINT('Ctrl Pts',(56.3839884990392,19.563446678012,18.1204801734757));
#28458=CARTESIAN_POINT('Ctrl Pts',(56.3904977429562,19.5697462999101,18.1210535613128));
#28459=CARTESIAN_POINT('Ctrl Pts',(56.4321962417984,19.6106557036476,18.1247310997206));
#28460=CARTESIAN_POINT('Ctrl Pts',(56.4661367907011,19.6465202396826,18.1277449032578));
#28461=CARTESIAN_POINT('Ctrl Pts',(56.5935327507123,19.7915610197578,18.1393152319278));
#28462=CARTESIAN_POINT('Ctrl Pts',(56.676415330692,19.9094456753282,18.1474527152592));
#28463=CARTESIAN_POINT('Ctrl Pts',(56.7910905743534,20.1169679609911,18.1613760968619));
#28464=CARTESIAN_POINT('Ctrl Pts',(56.8304615896814,20.2017781649908,18.1669639254012));
#28465=CARTESIAN_POINT('Ctrl Pts',(56.8691292678486,20.3031416551187,18.1737013152484));
#28466=CARTESIAN_POINT('Ctrl Pts',(56.8743529720651,20.3173165526956,18.1746445756106));
#28467=CARTESIAN_POINT('Ctrl Pts',(56.8826033392081,20.340513267139,18.176190599125));
#28468=CARTESIAN_POINT('Ctrl Pts',(56.885727395688,20.3494999863818,18.1767901326521));
#28469=CARTESIAN_POINT('Ctrl Pts',(56.8911956139495,20.3656004350518,18.1778654377349));
#28470=CARTESIAN_POINT('Ctrl Pts',(56.8935642401564,20.3727057117032,18.1783403916789));
#28471=CARTESIAN_POINT('Ctrl Pts',(56.898494255385,20.3877768873769,18.1793487760228));
#28472=CARTESIAN_POINT('Ctrl Pts',(56.9010456424856,20.3957458820755,18.1798825245754));
#28473=CARTESIAN_POINT('Ctrl Pts',(56.9077242778553,20.4170669405824,18.1813121762884));
#28474=CARTESIAN_POINT('Ctrl Pts',(56.9117614128221,20.43044652926,18.1822110025009));
#28475=CARTESIAN_POINT('Ctrl Pts',(56.9309034563253,20.4963832933026,18.1866496052671));
#28476=CARTESIAN_POINT('Ctrl Pts',(56.9439820569651,20.5494994476613,18.1902542139655));
#28477=CARTESIAN_POINT('Ctrl Pts',(56.995502981766,20.8032450654264,18.2076218195061));
#28478=CARTESIAN_POINT('Ctrl Pts',(57.0051560067028,21.0084170783801,18.2222589669907));
#28479=CARTESIAN_POINT('Ctrl Pts',(56.9799318898453,21.2450240881615,18.2383349641945));
#28480=CARTESIAN_POINT('Ctrl Pts',(56.9755016666597,21.2784970004414,18.2405858010395));
#28481=CARTESIAN_POINT('Ctrl Pts',(56.9689097393642,21.3201447108673,18.2433440609429));
#28482=CARTESIAN_POINT('Ctrl Pts',(56.9675433722257,21.3284376380569,18.2438911783563));
#28483=CARTESIAN_POINT('Ctrl Pts',(56.9653069034859,21.3414964167728,18.2447491264122));
#28484=CARTESIAN_POINT('Ctrl Pts',(56.9644718043535,21.3462680445421,18.2450618596848));
#28485=CARTESIAN_POINT('Ctrl Pts',(56.9628884082495,21.3551252030003,18.245640891276));
#28486=CARTESIAN_POINT('Ctrl Pts',(56.9621447403126,21.3592114022993,18.2459074358058));
#28487=CARTESIAN_POINT('Ctrl Pts',(56.960405526547,21.3686012096881,18.2465186135264));
#28488=CARTESIAN_POINT('Ctrl Pts',(56.9594012198622,21.3739031178642,18.2468627464483));
#28489=CARTESIAN_POINT('Ctrl Pts',(56.9562262718579,21.3903000701685,18.2479242220518));
#28490=CARTESIAN_POINT('Ctrl Pts',(56.9539827702364,21.4013810149472,18.2486375754434));
#28491=CARTESIAN_POINT('Ctrl Pts',(56.9314523282586,21.507993252029,18.2554676872703));
#28492=CARTESIAN_POINT('Ctrl Pts',(56.9042667132261,21.6019458019501,18.2612322963091));
#28493=CARTESIAN_POINT('Ctrl Pts',(56.808634556282,21.8598419475643,18.2772686881828));
#28494=CARTESIAN_POINT('Ctrl Pts',(56.7250710365429,22.0171587037543,18.2873818537632));
#28495=CARTESIAN_POINT('Ctrl Pts',(56.6093125594821,22.1788137130835,18.29965958357));
#28496=CARTESIAN_POINT('Ctrl Pts',(56.5965297125613,22.1960691892853,18.3009956821411));
#28497=CARTESIAN_POINT('Ctrl Pts',(56.577421007896,22.2210116694871,18.3029665504077));
#28498=CARTESIAN_POINT('Ctrl Pts',(56.5713119480881,22.2288634135698,18.3035928390739));
#28499=CARTESIAN_POINT('Ctrl Pts',(56.5604496049368,22.2426109372477,18.3046999735444));
#28500=CARTESIAN_POINT('Ctrl Pts',(56.5557209666886,22.2485260037902,18.3051798329161));
#28501=CARTESIAN_POINT('Ctrl Pts',(56.5458787301679,22.260694956201,18.3061743820476));
#28502=CARTESIAN_POINT('Ctrl Pts',(56.5407606011256,22.2669449821651,18.3066892489413));
#28503=CARTESIAN_POINT('Ctrl Pts',(56.5275247612064,22.2829091653812,18.3080149371423));
#28504=CARTESIAN_POINT('Ctrl Pts',(56.5193523815999,22.2925773288248,18.3088279740569));
#28505=CARTESIAN_POINT('Ctrl Pts',(56.4844998806572,22.3330216229214,18.3122729252365));
#28506=CARTESIAN_POINT('Ctrl Pts',(56.456974049518,22.3630527353309,18.314939626909));
#28507=CARTESIAN_POINT('Ctrl Pts',(56.3812563343511,22.4407463800846,18.3221411966938));
#28508=CARTESIAN_POINT('Ctrl Pts',(56.3315252068369,22.4868282534473,18.3267378413131));
#28509=CARTESIAN_POINT('Ctrl Pts',(56.2001581392498,22.5966708849461,18.3385245556724));
#28510=CARTESIAN_POINT('Ctrl Pts',(56.1157217532898,22.656774264336,18.3457926163767));
#28511=CARTESIAN_POINT('Ctrl Pts',(55.9587613575349,22.7510402709429,18.3584895285864));
#28512=CARTESIAN_POINT('Ctrl Pts',(55.8881122679599,22.7879107729435,18.3639416023737));
#28513=CARTESIAN_POINT('Ctrl Pts',(55.8059883029279,22.8246966031938,18.369850279464));
#28514=CARTESIAN_POINT('Ctrl Pts',(55.796502784846,22.8288570646599,18.3705264605794));
#28515=CARTESIAN_POINT('Ctrl Pts',(55.7821356742016,22.8350256677382,18.3715407043809));
#28516=CARTESIAN_POINT('Ctrl Pts',(55.7772779868933,22.8370885516932,18.3718819308855));
#28517=CARTESIAN_POINT('Ctrl Pts',(55.7685563061934,22.8407515465929,18.3724914635764));
#28518=CARTESIAN_POINT('Ctrl Pts',(55.7646954300366,22.842358801205,18.3727601933346));
#28519=CARTESIAN_POINT('Ctrl Pts',(55.7562575598405,22.8458403305667,18.373345102971));
#28520=CARTESIAN_POINT('Ctrl Pts',(55.7516786483577,22.8477097265659,18.3736609888215));
#28521=CARTESIAN_POINT('Ctrl Pts',(55.738654751645,22.8529704632052,18.3745552820806));
#28522=CARTESIAN_POINT('Ctrl Pts',(55.7301933149097,22.8563211225432,18.3751313068388));
#28523=CARTESIAN_POINT('Ctrl Pts',(55.6748456596824,22.8778013369524,18.3788686023687));
#28524=CARTESIAN_POINT('Ctrl Pts',(55.6273070024344,22.8942126062599,18.3819361079782));
#28525=CARTESIAN_POINT('Ctrl Pts',(55.4441175609856,22.9497981757071,18.3934013495461));
#28526=CARTESIAN_POINT('Ctrl Pts',(55.3050908075108,22.9763255866786,18.4014016019433));
#28527=CARTESIAN_POINT('Ctrl Pts',(55.1644483276976,22.9879598361178,18.4096837786395));
#28528=CARTESIAN_POINT('Origin',(55.,21.,6.22095488139522));
#28529=CARTESIAN_POINT('',(55.1644484414293,22.9879598267097,19.3668580791575));
#28530=CARTESIAN_POINT('',(55.1644482551197,22.9879598421216,19.2088565303878));
#28531=CARTESIAN_POINT('',(55.1644483516311,22.987959834138,6.22095488139522));
#28532=CARTESIAN_POINT('Ctrl Pts',(55.1644484414294,22.9879598267096,19.3668580791575));
#28533=CARTESIAN_POINT('Ctrl Pts',(55.2859411225326,22.9779096829471,19.3594542727769));
#28534=CARTESIAN_POINT('Ctrl Pts',(55.4063260452155,22.9567375761454,19.3524631524528));
#28535=CARTESIAN_POINT('Ctrl Pts',(55.6455879656927,22.8915870241497,19.3380541657924));
#28536=CARTESIAN_POINT('Ctrl Pts',(55.763668940839,22.8470758363702,19.3306581368666));
#28537=CARTESIAN_POINT('Ctrl Pts',(55.8945022252663,22.7830545490934,19.3216439778995));
#28538=CARTESIAN_POINT('Ctrl Pts',(55.9121147099626,22.7741094860059,19.320412915732));
#28539=CARTESIAN_POINT('Ctrl Pts',(55.9380642882356,22.7604416118804,19.3185714466332));
#28540=CARTESIAN_POINT('Ctrl Pts',(55.9465052330122,22.7559177419324,19.3179680374095));
#28541=CARTESIAN_POINT('Ctrl Pts',(55.9614967478699,22.7477436299196,19.3168883043627));
#28542=CARTESIAN_POINT('Ctrl Pts',(55.9680599695535,22.7441168782306,19.3164128230613));
#28543=CARTESIAN_POINT('Ctrl Pts',(55.9818757293327,22.7363804600097,19.3154059585645));
#28544=CARTESIAN_POINT('Ctrl Pts',(55.9891232510803,22.7322621742828,19.3148742727427));
#28545=CARTESIAN_POINT('Ctrl Pts',(56.0083213540756,22.7211934036829,19.313456421284));
#28546=CARTESIAN_POINT('Ctrl Pts',(56.0202256836369,22.7141640016197,19.3125674180118));
#28547=CARTESIAN_POINT('Ctrl Pts',(56.0721720160992,22.6827573541728,19.3086440047641));
#28548=CARTESIAN_POINT('Ctrl Pts',(56.1114177796997,22.6570983842651,19.305563096701));
#28549=CARTESIAN_POINT('Ctrl Pts',(56.1733121277617,22.6134434068244,19.3005079660549));
#28550=CARTESIAN_POINT('Ctrl Pts',(56.1965384618161,22.5962946341269,19.2985639143542));
#28551=CARTESIAN_POINT('Ctrl Pts',(56.3592069202022,22.4706458575167,19.2846133016888));
#28552=CARTESIAN_POINT('Ctrl Pts',(56.4840430907995,22.3445625351326,19.2720196080004));
#28553=CARTESIAN_POINT('Ctrl Pts',(56.6068527546109,22.1822748165837,19.2582023413602));
#28554=CARTESIAN_POINT('Ctrl Pts',(56.6226328388219,22.1605224399621,19.256395412602));
#28555=CARTESIAN_POINT('Ctrl Pts',(56.6480140422458,22.1240049075826,19.2534438913056));
#28556=CARTESIAN_POINT('Ctrl Pts',(56.6578674368494,22.1094200867443,19.2522860172605));
#28557=CARTESIAN_POINT('Ctrl Pts',(56.6710632659378,22.0893193505371,19.250720648619));
#28558=CARTESIAN_POINT('Ctrl Pts',(56.6745735682473,22.0839153350375,19.2503027622713));
#28559=CARTESIAN_POINT('Ctrl Pts',(56.6804174688579,22.0748226563168,19.2496047080065));
#28560=CARTESIAN_POINT('Ctrl Pts',(56.6827652343025,22.0711432114743,19.2493236162086));
#28561=CARTESIAN_POINT('Ctrl Pts',(56.6871916767807,22.0641555678516,19.24879245394));
#28562=CARTESIAN_POINT('Ctrl Pts',(56.6892727365996,22.0608489283642,19.2485422222219));
#28563=CARTESIAN_POINT('Ctrl Pts',(56.6946931116549,22.0521799866763,19.2478890643441));
#28564=CARTESIAN_POINT('Ctrl Pts',(56.6980167260998,22.0468078465211,19.2474871633156));
#28565=CARTESIAN_POINT('Ctrl Pts',(56.7094314437805,22.0281602021427,19.2461016374019));
#28566=CARTESIAN_POINT('Ctrl Pts',(56.717393071944,22.0148055645266,19.2451260345438));
#28567=CARTESIAN_POINT('Ctrl Pts',(56.7885443434707,21.8922220883278,19.2363087268229));
#28568=CARTESIAN_POINT('Ctrl Pts',(56.8414010223003,21.7773045663453,19.2290205339028));
#28569=CARTESIAN_POINT('Ctrl Pts',(56.9322448850836,21.5173886680701,19.2130470023684));
#28570=CARTESIAN_POINT('Ctrl Pts',(56.9654983874495,21.3715773312364,19.2043735255265));
#28571=CARTESIAN_POINT('Ctrl Pts',(56.9841432547822,21.2061672739225,19.1940435979984));
#28572=CARTESIAN_POINT('Ctrl Pts',(56.9858635750629,21.1888788810052,19.1929587154274));
#28573=CARTESIAN_POINT('Ctrl Pts',(56.9881404233005,21.1625054168029,19.1912948756796));
#28574=CARTESIAN_POINT('Ctrl Pts',(56.9888609877338,21.1534350686597,19.1907210593371));
#28575=CARTESIAN_POINT('Ctrl Pts',(56.9900591919319,21.1369218599516,19.1896733626656));
#28576=CARTESIAN_POINT('Ctrl Pts',(56.9905571965844,21.1294806077392,19.1892001295129));
#28577=CARTESIAN_POINT('Ctrl Pts',(56.9915431674171,21.1133946330175,19.1881746404512));
#28578=CARTESIAN_POINT('Ctrl Pts',(56.9920165990437,21.1047492038947,19.1876219390821));
#28579=CARTESIAN_POINT('Ctrl Pts',(56.9931513650979,21.0812224525582,19.1861135261575));
#28580=CARTESIAN_POINT('Ctrl Pts',(56.9937023063196,21.0663366021663,19.1851543875142));
#28581=CARTESIAN_POINT('Ctrl Pts',(56.9956548405061,20.9906553271943,19.1802529698554));
#28582=CARTESIAN_POINT('Ctrl Pts',(56.9944424018773,20.9298304569224,19.1762301306353));
#28583=CARTESIAN_POINT('Ctrl Pts',(56.9789477710719,20.6941106977564,19.1603083652287));
#28584=CARTESIAN_POINT('Ctrl Pts',(56.9443974063182,20.5213485816138,19.147841826439));
#28585=CARTESIAN_POINT('Ctrl Pts',(56.8705912524161,20.3052159700822,19.1321993940028));
#28586=CARTESIAN_POINT('Ctrl Pts',(56.8514700241245,20.2557578829777,19.128624413463));
#28587=CARTESIAN_POINT('Ctrl Pts',(56.8267337208243,20.1986533035171,19.1245477093294));
#28588=CARTESIAN_POINT('Ctrl Pts',(56.8230092300837,20.1902160969155,19.1239467257505));
#28589=CARTESIAN_POINT('Ctrl Pts',(56.8171865895121,20.1772696739806,19.1230269720805));
#28590=CARTESIAN_POINT('Ctrl Pts',(56.815129928672,20.1727420995832,19.1227057782285));
#28591=CARTESIAN_POINT('Ctrl Pts',(56.8113126842604,20.1644215130259,19.122116412038));
#28592=CARTESIAN_POINT('Ctrl Pts',(56.8095571130897,20.1606263626173,19.1218479498882));
#28593=CARTESIAN_POINT('Ctrl Pts',(56.805571516607,20.1520810199969,19.1212442549411));
#28594=CARTESIAN_POINT('Ctrl Pts',(56.803334678042,20.1473340990033,19.1209094461875));
#28595=CARTESIAN_POINT('Ctrl Pts',(56.7966893743056,20.1333748480332,19.1199263165851));
#28596=CARTESIAN_POINT('Ctrl Pts',(56.7922287849532,20.1241873176264,19.1192811083811));
#28597=CARTESIAN_POINT('Ctrl Pts',(56.7566305321969,20.0522761580961,19.1142425209722));
#28598=CARTESIAN_POINT('Ctrl Pts',(56.7222764159288,19.9911900500591,19.1100307326643));
#28599=CARTESIAN_POINT('Ctrl Pts',(56.5942065319402,19.7891531139887,19.0959099571347));
#28600=CARTESIAN_POINT('Ctrl Pts',(56.4858333894587,19.6583792528013,19.086372882142));
#28601=CARTESIAN_POINT('Ctrl Pts',(56.3251399575892,19.508151174059,19.0731264165011));
#28602=CARTESIAN_POINT('Ctrl Pts',(56.286717084246,19.4748877726493,19.0700192992901));
#28603=CARTESIAN_POINT('Ctrl Pts',(56.2364131051047,19.434593793396,19.0660001799576));
#28604=CARTESIAN_POINT('Ctrl Pts',(56.2256702745376,19.4261682677051,19.0651446028397));
#28605=CARTESIAN_POINT('Ctrl Pts',(56.2082604099772,19.412800201317,19.063761976281));
#28606=CARTESIAN_POINT('Ctrl Pts',(56.2016474232291,19.4077877383555,19.063237693029));
#28607=CARTESIAN_POINT('Ctrl Pts',(56.1889927101028,19.3983195539257,19.0622360118921));
#28608=CARTESIAN_POINT('Ctrl Pts',(56.1829567160759,19.393856382082,19.0617589164768));
#28609=CARTESIAN_POINT('Ctrl Pts',(56.1691072327962,19.3837361315295,19.0606657015447));
#28610=CARTESIAN_POINT('Ctrl Pts',(56.1612776604253,19.3781014815065,19.0600487299997));
#28611=CARTESIAN_POINT('Ctrl Pts',(56.1407279121673,19.3635376811794,19.0584319890772));
#28612=CARTESIAN_POINT('Ctrl Pts',(56.127943908675,19.3547001468704,19.0574287642209));
#28613=CARTESIAN_POINT('Ctrl Pts',(56.0185596456632,19.2809572269973,19.0488645519399));
#28614=CARTESIAN_POINT('Ctrl Pts',(55.9165700116096,19.2244823821459,19.0409883898205));
#28615=CARTESIAN_POINT('Ctrl Pts',(55.7339085957034,19.1432860802634,19.0271511329896));
#28616=CARTESIAN_POINT('Ctrl Pts',(55.6555040412386,19.1141785838989,19.0212947313369));
#28617=CARTESIAN_POINT('Ctrl Pts',(55.5022637327687,19.0680034849264,19.0101841413865));
#28618=CARTESIAN_POINT('Ctrl Pts',(55.4278024087881,19.0501623323476,19.0049307881534));
#28619=CARTESIAN_POINT('Ctrl Pts',(55.3376492762529,19.0339766083183,18.9988726566501));
#28620=CARTESIAN_POINT('Ctrl Pts',(55.3227749481266,19.0314799020175,18.9978829148723));
#28621=CARTESIAN_POINT('Ctrl Pts',(55.3018825969923,19.0282162331309,18.9965077607259));
#28622=CARTESIAN_POINT('Ctrl Pts',(55.2958876562402,19.0273077222059,18.9961148975625));
#28623=CARTESIAN_POINT('Ctrl Pts',(55.2856445244367,19.0258031585704,18.9954466984697));
#28624=CARTESIAN_POINT('Ctrl Pts',(55.2813984089412,19.0251934525496,18.9951706046192));
#28625=CARTESIAN_POINT('Ctrl Pts',(55.2732032762931,19.0240436700801,18.994639502561));
#28626=CARTESIAN_POINT('Ctrl Pts',(55.2692545880594,19.0235017289619,18.9943843859319));
#28627=CARTESIAN_POINT('Ctrl Pts',(55.259744688178,19.0222255626833,18.9937718050246));
#28628=CARTESIAN_POINT('Ctrl Pts',(55.2541819139722,19.0215029481025,18.9934149869697));
#28629=CARTESIAN_POINT('Ctrl Pts',(55.2337303375651,19.0189339300017,18.9921084385052));
#28630=CARTESIAN_POINT('Ctrl Pts',(55.218823443012,19.0172319911626,18.991166414364));
#28631=CARTESIAN_POINT('Ctrl Pts',(55.0669568627943,19.0016268389757,18.9816611373217));
#28632=CARTESIAN_POINT('Ctrl Pts',(54.9289057299566,19.0017669528759,18.9737617623569));
#28633=CARTESIAN_POINT('Ctrl Pts',(54.6538696557266,19.0306096821275,18.9577096318486));
#28634=CARTESIAN_POINT('Ctrl Pts',(54.5176951447003,19.0594641864507,18.9495869235747));
#28635=CARTESIAN_POINT('Ctrl Pts',(54.3693612343454,19.1074845707804,18.9399081266529));
#28636=CARTESIAN_POINT('Ctrl Pts',(54.3531632342526,19.112959440672,18.9388401922774));
#28637=CARTESIAN_POINT('Ctrl Pts',(54.3285103167869,19.1216467532982,18.9371970450356));
#28638=CARTESIAN_POINT('Ctrl Pts',(54.3200032794803,19.124709683864,18.9366267752276));
#28639=CARTESIAN_POINT('Ctrl Pts',(54.3051994858916,19.1301537166707,18.935628567122));
#28640=CARTESIAN_POINT('Ctrl Pts',(54.2988933664387,19.1325090725132,18.9352014919745));
#28641=CARTESIAN_POINT('Ctrl Pts',(54.2847045013276,19.1378906565276,18.9342363096098));
#28642=CARTESIAN_POINT('Ctrl Pts',(54.2768288441288,19.1409350917279,18.9336975996116));
#28643=CARTESIAN_POINT('Ctrl Pts',(54.2556543266914,19.1492752815392,18.9322410558365));
#28644=CARTESIAN_POINT('Ctrl Pts',(54.2423929518496,19.1546642560872,18.9313201049836));
#28645=CARTESIAN_POINT('Ctrl Pts',(54.1814180226552,19.1802104598729,18.927044303893));
#28646=CARTESIAN_POINT('Ctrl Pts',(54.1344467672732,19.2020769736481,18.9236320436585));
#28647=CARTESIAN_POINT('Ctrl Pts',(53.9238397523617,19.3102874238033,18.9077713883804));
#28648=CARTESIAN_POINT('Ctrl Pts',(53.7718659321933,19.4173070585869,18.8946186371054));
#28649=CARTESIAN_POINT('Ctrl Pts',(53.5975470639746,19.5804750873222,18.8782569343677));
#28650=CARTESIAN_POINT('Ctrl Pts',(53.5597485021142,19.6188403492554,18.8746241484992));
#28651=CARTESIAN_POINT('Ctrl Pts',(53.5173204782722,19.6655432969737,18.8704904622032));
#28652=CARTESIAN_POINT('Ctrl Pts',(53.5111434503766,19.6724385366253,18.8698871852652));
#28653=CARTESIAN_POINT('Ctrl Pts',(53.5017174151732,19.6831090932932,18.8689646735319));
#28654=CARTESIAN_POINT('Ctrl Pts',(53.4984342698925,19.6868538833614,18.8686429926959));
#28655=CARTESIAN_POINT('Ctrl Pts',(53.4924205767139,19.6937652099313,18.8680531653004));
#28656=CARTESIAN_POINT('Ctrl Pts',(53.4896859709943,19.6969280224366,18.8677847256112));
#28657=CARTESIAN_POINT('Ctrl Pts',(53.483547535146,19.704072947265,18.8671816196277));
#28658=CARTESIAN_POINT('Ctrl Pts',(53.4801494412468,19.7080598757135,18.8668473735814));
#28659=CARTESIAN_POINT('Ctrl Pts',(53.4702000527617,19.7198269135833,18.8658674391641));
#28660=CARTESIAN_POINT('Ctrl Pts',(53.4636923930911,19.7276439346457,18.8652248333013));
#28661=CARTESIAN_POINT('Ctrl Pts',(53.4137008338015,19.7886367311673,18.8602723444036));
#28662=CARTESIAN_POINT('Ctrl Pts',(53.3729251067131,19.8439829344545,18.8561371453906));
#28663=CARTESIAN_POINT('Ctrl Pts',(53.2412452134526,20.0435295706021,18.8420128218157));
#28664=CARTESIAN_POINT('Ctrl Pts',(53.1660131308663,20.1971618808354,18.83241418035));
#28665=CARTESIAN_POINT('Ctrl Pts',(53.0948243031391,20.4067614341369,18.8190863012976));
#28666=CARTESIAN_POINT('Ctrl Pts',(53.0802871436911,20.4556395411664,18.8159688878775));
#28667=CARTESIAN_POINT('Ctrl Pts',(53.0642471398112,20.5182581239285,18.8119381294669));
#28668=CARTESIAN_POINT('Ctrl Pts',(53.0609918215238,20.5315326692724,18.8110816194378));
#28669=CARTESIAN_POINT('Ctrl Pts',(53.055979048103,20.5529216924376,18.8096978461553));
#28670=CARTESIAN_POINT('Ctrl Pts',(53.054135352594,20.5610156664466,18.8091733574607));
#28671=CARTESIAN_POINT('Ctrl Pts',(53.0507208803157,20.5764497454351,18.8081715216709));
#28672=CARTESIAN_POINT('Ctrl Pts',(53.0491409042501,20.5837876856904,18.8076944786128));
#28673=CARTESIAN_POINT('Ctrl Pts',(53.0456264614121,20.6005696988359,18.8066017196924));
#28674=CARTESIAN_POINT('Ctrl Pts',(53.0437189770464,20.6100191701411,18.8059851543555));
#28675=CARTESIAN_POINT('Ctrl Pts',(53.0389194403859,20.6347172589119,18.8043701752034));
#28676=CARTESIAN_POINT('Ctrl Pts',(53.0361367730995,20.6499862207568,18.803368318183));
#28677=CARTESIAN_POINT('Ctrl Pts',(53.0146074315655,20.7764724624523,18.7950390063809));
#28678=CARTESIAN_POINT('Ctrl Pts',(53.0051492669158,20.8890447531017,18.7874166042857));
#28679=CARTESIAN_POINT('Ctrl Pts',(53.0053603005261,21.1233753678906,18.7712141163126));
#28680=CARTESIAN_POINT('Ctrl Pts',(53.0165845065903,21.244687115159,18.7626384351935));
#28681=CARTESIAN_POINT('Ctrl Pts',(53.0479813616346,21.4137492010836,18.750874704986));
#28682=CARTESIAN_POINT('Ctrl Pts',(53.0590530088554,21.4629156453414,18.7474797070929));
#28683=CARTESIAN_POINT('Ctrl Pts',(53.07419398738,21.5199745951858,18.7436097376684));
#28684=CARTESIAN_POINT('Ctrl Pts',(53.07646683976,21.5283205142837,18.7430454720404));
#28685=CARTESIAN_POINT('Ctrl Pts',(53.0802379140464,21.5418209141714,18.7421359098346));
#28686=CARTESIAN_POINT('Ctrl Pts',(53.0817027498944,21.5469844893309,18.7417887852761));
#28687=CARTESIAN_POINT('Ctrl Pts',(53.0843481357721,21.556168186226,18.7411728398162));
#28688=CARTESIAN_POINT('Ctrl Pts',(53.0855205256801,21.5601905567017,18.7409035573398));
#28689=CARTESIAN_POINT('Ctrl Pts',(53.0880863509747,21.5688915457478,18.7403221450275));
#28690=CARTESIAN_POINT('Ctrl Pts',(53.0894842876925,21.5735687460209,18.7400102797632));
#28691=CARTESIAN_POINT('Ctrl Pts',(53.0934499994578,21.5866618075168,18.7391390256548));
#28692=CARTESIAN_POINT('Ctrl Pts',(53.0960563457867,21.5950660041951,18.7385818283651));
#28693=CARTESIAN_POINT('Ctrl Pts',(53.1120900707537,21.6455830041664,18.7352433522298));
#28694=CARTESIAN_POINT('Ctrl Pts',(53.1268596743861,21.6872607255614,18.7325342811241));
#28695=CARTESIAN_POINT('Ctrl Pts',(53.1816596222082,21.8269655643011,18.7234994424352));
#28696=CARTESIAN_POINT('Ctrl Pts',(53.2281023500646,21.9222883818736,18.7174066970902));
#28697=CARTESIAN_POINT('Ctrl Pts',(53.3511608409721,22.1309036358589,18.7033441619654));
#28698=CARTESIAN_POINT('Ctrl Pts',(53.432271159131,22.2409000095519,18.6953577156356));
#28699=CARTESIAN_POINT('Ctrl Pts',(53.5342969807604,22.3531365666591,18.685941551004));
#28700=CARTESIAN_POINT('Ctrl Pts',(53.5447688712159,22.3643922638929,18.6849818853084));
#28701=CARTESIAN_POINT('Ctrl Pts',(53.5619867986147,22.3824752005507,18.6834142329667));
#28702=CARTESIAN_POINT('Ctrl Pts',(53.568653971561,22.3893769068135,18.682809629137));
#28703=CARTESIAN_POINT('Ctrl Pts',(53.5806208511983,22.4015871923155,18.6817285638286));
#28704=CARTESIAN_POINT('Ctrl Pts',(53.5859012261112,22.4069145250838,18.6812529527673));
#28705=CARTESIAN_POINT('Ctrl Pts',(53.5971054056754,22.4180915445048,18.680246651841));
#28706=CARTESIAN_POINT('Ctrl Pts',(53.6030360230924,22.42393416812,18.6797156643237));
#28707=CARTESIAN_POINT('Ctrl Pts',(53.6188770319087,22.4393459248997,18.6783016540643));
#28708=CARTESIAN_POINT('Ctrl Pts',(53.6288501356403,22.4488496741154,18.677415820841));
#28709=CARTESIAN_POINT('Ctrl Pts',(53.6771102268659,22.4938939737484,18.6731493125576));
#28710=CARTESIAN_POINT('Ctrl Pts',(53.7166819983548,22.5280218010313,18.6697097423274));
#28711=CARTESIAN_POINT('Ctrl Pts',(53.835507587072,22.622626286645,18.6595392475672));
#28712=CARTESIAN_POINT('Ctrl Pts',(53.9180039774493,22.6787611985284,18.6526617795959));
#28713=CARTESIAN_POINT('Ctrl Pts',(54.1169543912512,22.7933622779506,18.6366662995435));
#28714=CARTESIAN_POINT('Ctrl Pts',(54.2356484977355,22.8470761231287,18.6275336185841));
#28715=CARTESIAN_POINT('Ctrl Pts',(54.3732785186139,22.8938013930089,18.6179124591341));
#28716=CARTESIAN_POINT('Ctrl Pts',(54.38788147624,22.8985716944163,18.6169035935973));
#28717=CARTESIAN_POINT('Ctrl Pts',(54.4085360592497,22.9050557691459,18.6154948596926));
#28718=CARTESIAN_POINT('Ctrl Pts',(54.4145424755502,22.9069102145659,18.615087352264));
#28719=CARTESIAN_POINT('Ctrl Pts',(54.424662054852,22.9099822538324,18.6144045269025));
#28720=CARTESIAN_POINT('Ctrl Pts',(54.4287705250835,22.9112150190991,18.6141283391773));
#28721=CARTESIAN_POINT('Ctrl Pts',(54.4371590525104,22.9137025690496,18.6135665807633));
#28722=CARTESIAN_POINT('Ctrl Pts',(54.4414393901271,22.9149562660828,18.6132810736569));
#28723=CARTESIAN_POINT('Ctrl Pts',(54.4523418269694,22.9181098896567,18.6125566627342));
#28724=CARTESIAN_POINT('Ctrl Pts',(54.4589696951312,22.9199899051409,18.612118900844));
#28725=CARTESIAN_POINT('Ctrl Pts',(54.4858090013379,22.9274529419544,18.6103563046855));
#28726=CARTESIAN_POINT('Ctrl Pts',(54.5060989900034,22.9327516917152,18.6090469285729));
#28727=CARTESIAN_POINT('Ctrl Pts',(54.5596293300779,22.9458331019816,18.605643821469));
#28728=CARTESIAN_POINT('Ctrl Pts',(54.5929934487368,22.95308441272,18.603574315374));
#28729=CARTESIAN_POINT('Ctrl Pts',(54.7793468777514,22.988602877633,18.5922184537084));
#28730=CARTESIAN_POINT('Ctrl Pts',(54.9350536377415,22.9997543790344,18.5834452992847));
#28731=CARTESIAN_POINT('Ctrl Pts',(55.1151708305678,22.9915757571036,18.5727943099788));
#28732=CARTESIAN_POINT('Ctrl Pts',(55.1398302308105,22.9899962989591,18.5713262821773));
#28733=CARTESIAN_POINT('Ctrl Pts',(55.1644483870895,22.9879598312048,18.5698477239299));
#28734=CARTESIAN_POINT('',(53.0052494851995,20.9997435532217,18.6227928887582));
#28735=CARTESIAN_POINT('Ctrl Pts',(55.1644483276976,22.9879598361178,18.4096837786395));
#28736=CARTESIAN_POINT('Ctrl Pts',(55.1550885057686,22.9887341007864,18.4102349613203));
#28737=CARTESIAN_POINT('Ctrl Pts',(55.1457215198892,22.989442403148,18.4107872590292));
#28738=CARTESIAN_POINT('Ctrl Pts',(55.1025841399482,22.9923979045278,18.4133348257717));
#28739=CARTESIAN_POINT('Ctrl Pts',(55.0687679341149,22.9938514852108,18.4153435664557));
#28740=CARTESIAN_POINT('Ctrl Pts',(54.9795085102815,22.9954148400144,18.4206979885749));
#28741=CARTESIAN_POINT('Ctrl Pts',(54.9240728494658,22.9940748504138,18.4240771874888));
#28742=CARTESIAN_POINT('Ctrl Pts',(54.8543195138251,22.9894759199281,18.4284303062247));
#28743=CARTESIAN_POINT('Ctrl Pts',(54.8398817502561,22.9883660047059,18.4293367516838));
#28744=CARTESIAN_POINT('Ctrl Pts',(54.8169289460162,22.9863498814668,18.4307869649421));
#28745=CARTESIAN_POINT('Ctrl Pts',(54.8084052687768,22.9855458487978,18.4313275264826));
#28746=CARTESIAN_POINT('Ctrl Pts',(54.7924618242377,22.9839382963969,18.4323425262472));
#28747=CARTESIAN_POINT('Ctrl Pts',(54.7850408547072,22.9831479575876,18.4328165421133));
#28748=CARTESIAN_POINT('Ctrl Pts',(54.7684638842948,22.9812883596184,18.4338790073341));
#28749=CARTESIAN_POINT('Ctrl Pts',(54.7593105551118,22.9801972435193,18.4344681349272));
#28750=CARTESIAN_POINT('Ctrl Pts',(54.7323455245529,22.9767931725836,18.4362111026556));
#28751=CARTESIAN_POINT('Ctrl Pts',(54.7145575059956,22.9743030955237,18.4373704850324));
#28752=CARTESIAN_POINT('Ctrl Pts',(54.6742428158626,22.9681033907971,18.4400206626057));
#28753=CARTESIAN_POINT('Ctrl Pts',(54.6517416569175,22.9642466126832,18.4415159195772));
#28754=CARTESIAN_POINT('Ctrl Pts',(54.5775504343614,22.9502151320402,18.4465005513552));
#28755=CARTESIAN_POINT('Ctrl Pts',(54.5262006422796,22.9383797554411,18.4500391954169));
#28756=CARTESIAN_POINT('Ctrl Pts',(54.347440951541,22.889650692891,18.4626600303391));
#28757=CARTESIAN_POINT('Ctrl Pts',(54.223301076904,22.8421039058492,18.4720010607957));
#28758=CARTESIAN_POINT('Ctrl Pts',(54.0386104597179,22.7493557372527,18.4863063329261));
#28759=CARTESIAN_POINT('Ctrl Pts',(53.97430490171,22.7124448646036,18.4913652834678));
#28760=CARTESIAN_POINT('Ctrl Pts',(53.9035830886952,22.6664342458163,18.4969044543053));
#28761=CARTESIAN_POINT('Ctrl Pts',(53.8950135514606,22.6607643115071,18.4975751844623));
#28762=CARTESIAN_POINT('Ctrl Pts',(53.8821239031164,22.6520920861037,18.4985828813699));
#28763=CARTESIAN_POINT('Ctrl Pts',(53.8777713830982,22.6491386120931,18.4989229530907));
#28764=CARTESIAN_POINT('Ctrl Pts',(53.8700764270214,22.6438725013522,18.4995237428057));
#28765=CARTESIAN_POINT('Ctrl Pts',(53.8667293412371,22.6415668418983,18.4997849183142));
#28766=CARTESIAN_POINT('Ctrl Pts',(53.8633680990657,22.6392362504958,18.5000470433025));
#28767=CARTESIAN_POINT('Ctrl Pts',(53.8633469696672,22.6392215993564,18.5000486910634));
#28768=CARTESIAN_POINT('Ctrl Pts',(53.8633048768407,22.6391924109563,18.5000519736303));
#28769=CARTESIAN_POINT('Ctrl Pts',(53.8632839137361,22.6391778739294,18.5000536084111));
#28770=CARTESIAN_POINT('Ctrl Pts',(53.863242150943,22.6391489120114,18.5000568652175));
#28771=CARTESIAN_POINT('Ctrl Pts',(53.8632213509964,22.6391344869504,18.5000584872632));
#28772=CARTESIAN_POINT('Ctrl Pts',(53.8631799101496,22.6391057459613,18.5000617189402));
#28773=CARTESIAN_POINT('Ctrl Pts',(53.8631592696543,22.6390914303229,18.5000633285401));
#28774=CARTESIAN_POINT('Ctrl Pts',(53.863118144229,22.6390629057911,18.5000665355972));
#28775=CARTESIAN_POINT('Ctrl Pts',(53.8630976596403,22.639048697143,18.5000681330279));
#28776=CARTESIAN_POINT('Ctrl Pts',(53.8630568434283,22.6390203848144,18.5000713159497));
#28777=CARTESIAN_POINT('Ctrl Pts',(53.8630365115884,22.639006280992,18.5000729014578));
#28778=CARTESIAN_POINT('Ctrl Pts',(53.8629959978564,22.6389781762467,18.5000760607699));
#28779=CARTESIAN_POINT('Ctrl Pts',(53.862975815614,22.6389641750888,18.5000776346013));
#28780=CARTESIAN_POINT('Ctrl Pts',(53.8629355981506,22.638936273667,18.5000807707886));
#28781=CARTESIAN_POINT('Ctrl Pts',(53.862915562651,22.6389223732176,18.5000823331663));
#28782=CARTESIAN_POINT('Ctrl Pts',(53.8628756340883,22.6388946700555,18.5000854468038));
#28783=CARTESIAN_POINT('Ctrl Pts',(53.8628557416861,22.6388808678088,18.5000869980122));
#28784=CARTESIAN_POINT('Ctrl Pts',(53.8628160973718,22.6388533597248,18.5000900894632));
#28785=CARTESIAN_POINT('Ctrl Pts',(53.8627963453358,22.6388396538088,18.5000916297155));
#28786=CARTESIAN_POINT('Ctrl Pts',(53.862756978903,22.6388123364303,18.5000946994769));
#28787=CARTESIAN_POINT('Ctrl Pts',(53.8627373644,22.6387987249013,18.5000962289944));
#28788=CARTESIAN_POINT('Ctrl Pts',(53.8586701621368,22.6359761724477,18.5004133839195));
#28789=CARTESIAN_POINT('Ctrl Pts',(53.854632942132,22.6331522095715,18.5007279856178));
#28790=CARTESIAN_POINT('Ctrl Pts',(53.8462369048929,22.6272328850598,18.5013818936148));
#28791=CARTESIAN_POINT('Ctrl Pts',(53.8418799778788,22.6241348951849,18.501721022344));
#28792=CARTESIAN_POINT('Ctrl Pts',(53.8306498442973,22.6160815481713,18.5025947651682));
#28793=CARTESIAN_POINT('Ctrl Pts',(53.8237955823877,22.611099789195,18.5031276862468));
#28794=CARTESIAN_POINT('Ctrl Pts',(53.8036536372127,22.5962633269787,18.5046933262786));
#28795=CARTESIAN_POINT('Ctrl Pts',(53.7904562363721,22.5862865916265,18.5057186431587));
#28796=CARTESIAN_POINT('Ctrl Pts',(53.7433236293698,22.5497258539722,18.5093846405643));
#28797=CARTESIAN_POINT('Ctrl Pts',(53.7101263146181,22.5222063212168,18.511974882489));
#28798=CARTESIAN_POINT('Ctrl Pts',(53.575545856806,22.4030763258956,18.5226325200484));
#28799=CARTESIAN_POINT('Ctrl Pts',(53.4828182024347,22.3022500541807,18.5303886168244));
#28800=CARTESIAN_POINT('Ctrl Pts',(53.3499079523017,22.1240817051133,18.5434873898295));
#28801=CARTESIAN_POINT('Ctrl Pts',(53.3031753228346,22.0522104306539,18.5486308867433));
#28802=CARTESIAN_POINT('Ctrl Pts',(53.2539276187076,21.9646136738307,18.5548737786316));
#28803=CARTESIAN_POINT('Ctrl Pts',(53.2467916214334,21.9515821893404,18.5558017067762));
#28804=CARTESIAN_POINT('Ctrl Pts',(53.2353613305279,21.930143547732,18.557327582821));
#28805=CARTESIAN_POINT('Ctrl Pts',(53.230979888414,21.9217833221826,18.5579224419543));
#28806=CARTESIAN_POINT('Ctrl Pts',(53.2232320915487,21.9067410543683,18.5589925919422));
#28807=CARTESIAN_POINT('Ctrl Pts',(53.21984366561,21.9000705321351,18.5594670960113));
#28808=CARTESIAN_POINT('Ctrl Pts',(53.2127250609459,21.885859261093,18.5604779661414));
#28809=CARTESIAN_POINT('Ctrl Pts',(53.2090049093078,21.8783136796017,18.5610146709743));
#28810=CARTESIAN_POINT('Ctrl Pts',(53.1991422028856,21.8579859377695,18.5624606071198));
#28811=CARTESIAN_POINT('Ctrl Pts',(53.1930881335572,21.8451616203493,18.5633728791751));
#28812=CARTESIAN_POINT('Ctrl Pts',(53.1632549635988,21.7801801176472,18.5679966090179));
#28813=CARTESIAN_POINT('Ctrl Pts',(53.1415972910451,21.7270843242576,18.5717796241899));
#28814=CARTESIAN_POINT('Ctrl Pts',(53.0861655787287,21.5724546300179,18.582817890383));
#28815=CARTESIAN_POINT('Ctrl Pts',(53.0582333669201,21.469046053463,18.5902349100963));
#28816=CARTESIAN_POINT('Ctrl Pts',(53.0164415917545,21.2438109623391,18.6062119264787));
#28817=CARTESIAN_POINT('Ctrl Pts',(53.005234400944,21.1219108081174,18.6147522648045));
#28818=CARTESIAN_POINT('Ctrl Pts',(53.0052500162953,20.9997450290738,18.6227937120875));
#28819=CARTESIAN_POINT('Ctrl Pts',(53.0052500164767,20.9997436136241,18.6227938052581));
#28820=CARTESIAN_POINT('Ctrl Pts',(53.0052508228815,20.9934695837175,18.6232067871531));
#28821=CARTESIAN_POINT('Ctrl Pts',(53.0052812295882,20.9871954844429,18.6236183689611));
#28822=CARTESIAN_POINT('Ctrl Pts',(53.0054036384665,20.9743976083966,18.6244549063218));
#28823=CARTESIAN_POINT('Ctrl Pts',(53.0054980455807,20.9678739275997,18.6248797358704));
#28824=CARTESIAN_POINT('Ctrl Pts',(53.0057060265368,20.9571417189301,18.625575880343));
#28825=CARTESIAN_POINT('Ctrl Pts',(53.0058009183083,20.9529329391716,18.6258481869857));
#28826=CARTESIAN_POINT('Ctrl Pts',(53.0060117717511,20.9447329124107,18.6263773290831));
#28827=CARTESIAN_POINT('Ctrl Pts',(53.0061263948672,20.9407416397901,18.6266342372098));
#28828=CARTESIAN_POINT('Ctrl Pts',(53.0063978370226,20.9321852354407,18.6271835742972));
#28829=CARTESIAN_POINT('Ctrl Pts',(53.0065583523545,20.9276202723663,18.6274757948803));
#28830=CARTESIAN_POINT('Ctrl Pts',(53.0070192428518,20.9156807415714,18.6282379373242));
#28831=CARTESIAN_POINT('Ctrl Pts',(53.0073448721434,20.9083071365057,18.6287064723275));
#28832=CARTESIAN_POINT('Ctrl Pts',(53.0088491839476,20.8780539245543,18.6306206308297));
#28833=CARTESIAN_POINT('Ctrl Pts',(53.0103811057744,20.8551926124682,18.6320478496479));
#28834=CARTESIAN_POINT('Ctrl Pts',(53.0163547483494,20.7843629450692,18.636423954629));
#28835=CARTESIAN_POINT('Ctrl Pts',(53.0221404518353,20.7365230494234,18.639314563721));
#28836=CARTESIAN_POINT('Ctrl Pts',(53.0565943291302,20.5182844616601,18.652388534347));
#28837=CARTESIAN_POINT('Ctrl Pts',(53.1055892988108,20.3518587322202,18.6621091859325));
#28838=CARTESIAN_POINT('Ctrl Pts',(53.1961502569472,20.1468965143007,18.6755976310348));
#28839=CARTESIAN_POINT('Ctrl Pts',(53.2186849502699,20.1007917580869,18.678734267687));
#28840=CARTESIAN_POINT('Ctrl Pts',(53.2494529895803,20.0435481028146,18.6827865920195));
#28841=CARTESIAN_POINT('Ctrl Pts',(53.2560597815123,20.0315540454702,18.6836446733391));
#28842=CARTESIAN_POINT('Ctrl Pts',(53.266871289259,20.0123961252027,18.6850302788032));
#28843=CARTESIAN_POINT('Ctrl Pts',(53.2709982532485,20.0051887124398,18.6855550136619));
#28844=CARTESIAN_POINT('Ctrl Pts',(53.2789386319406,19.9915201459098,18.6865568541372));
#28845=CARTESIAN_POINT('Ctrl Pts',(53.2827437322724,19.9850543082703,18.687033652837));
#28846=CARTESIAN_POINT('Ctrl Pts',(53.2915135587098,19.9703426378938,18.6881251943778));
#28847=CARTESIAN_POINT('Ctrl Pts',(53.2965016427007,19.9621110152232,18.6887407812074));
#28848=CARTESIAN_POINT('Ctrl Pts',(53.3096643504369,19.9407396796292,18.6903518310582));
#28849=CARTESIAN_POINT('Ctrl Pts',(53.3179325240055,19.9276586279107,18.6913507113138));
#28850=CARTESIAN_POINT('Ctrl Pts',(53.3984520140796,19.8034918173579,18.700957262903));
#28851=CARTESIAN_POINT('Ctrl Pts',(53.4814378430074,19.6997905442718,18.7099805762316));
#28852=CARTESIAN_POINT('Ctrl Pts',(53.6410368518047,19.536641868137,18.7258447849989));
#28853=CARTESIAN_POINT('Ctrl Pts',(53.7128447848687,19.4730979473654,18.7325680028708));
#28854=CARTESIAN_POINT('Ctrl Pts',(53.8194027678941,19.3916817949866,18.7417737253925));
#28855=CARTESIAN_POINT('Ctrl Pts',(53.8505320890769,19.3692881435037,18.7443786988831));
#28856=CARTESIAN_POINT('Ctrl Pts',(53.8949430311443,19.3392441323328,18.7479597324971));
#28857=CARTESIAN_POINT('Ctrl Pts',(53.9076950912779,19.3308292555581,18.7489728983643));
#28858=CARTESIAN_POINT('Ctrl Pts',(53.9272789220579,19.3182267650912,18.7505045605717));
#28859=CARTESIAN_POINT('Ctrl Pts',(53.9340410368713,19.3139326174054,18.751029080199));
#28860=CARTESIAN_POINT('Ctrl Pts',(53.9451974662106,19.3069418928873,18.7518870993712));
#28861=CARTESIAN_POINT('Ctrl Pts',(53.9495766200719,19.3042214579562,18.7522220448244));
#28862=CARTESIAN_POINT('Ctrl Pts',(53.9580400840686,19.2990091164134,18.752865757851));
#28863=CARTESIAN_POINT('Ctrl Pts',(53.9621229043583,19.2965148700495,18.7531746724887));
#28864=CARTESIAN_POINT('Ctrl Pts',(53.9696612779904,19.2919467451694,18.753742013591));
#28865=CARTESIAN_POINT('Ctrl Pts',(53.9731141180961,19.2898686631034,18.7540007060626));
#28866=CARTESIAN_POINT('Ctrl Pts',(53.9810914230275,19.2851004167674,18.7545957079765));
#28867=CARTESIAN_POINT('Ctrl Pts',(53.9856202486522,19.2824176903602,18.7549315336374));
#28868=CARTESIAN_POINT('Ctrl Pts',(53.9990360537877,19.2745421819368,18.755920723018));
#28869=CARTESIAN_POINT('Ctrl Pts',(54.0079528263097,19.2694001272963,18.7565709156031));
#28870=CARTESIAN_POINT('Ctrl Pts',(54.1107066663573,19.2112000149813,18.7639852005353));
#28871=CARTESIAN_POINT('Ctrl Pts',(54.2086709083405,19.165755446381,18.7703134755018));
#28872=CARTESIAN_POINT('Ctrl Pts',(54.4245021411702,19.0861648989031,18.7836954551731));
#28873=CARTESIAN_POINT('Ctrl Pts',(54.5427996290358,19.0545106843378,18.7907147107882));
#28874=CARTESIAN_POINT('Ctrl Pts',(54.7209853631643,19.023991434884,18.801541812735));
#28875=CARTESIAN_POINT('Ctrl Pts',(54.7791259874304,19.0166511402908,18.8051099869406));
#28876=CARTESIAN_POINT('Ctrl Pts',(54.8517297169933,19.0107168929062,18.8096485719435));
#28877=CARTESIAN_POINT('Ctrl Pts',(54.8659697024608,19.0097067503554,18.8105426065393));
#28878=CARTESIAN_POINT('Ctrl Pts',(54.8886373473691,19.0083431402858,18.8119724128908));
#28879=CARTESIAN_POINT('Ctrl Pts',(54.8970586980233,19.0078901204862,18.8125050642727));
#28880=CARTESIAN_POINT('Ctrl Pts',(54.9129527438069,19.0071361645025,18.8135132213141));
#28881=CARTESIAN_POINT('Ctrl Pts',(54.9204247717523,19.0068238230911,18.8139883612269));
#28882=CARTESIAN_POINT('Ctrl Pts',(54.9372978334304,19.0062135350853,18.815064070495));
#28883=CARTESIAN_POINT('Ctrl Pts',(54.9466995209903,19.0059400502247,18.8156653944411));
#28884=CARTESIAN_POINT('Ctrl Pts',(54.9708473502626,19.0054085138189,18.8172149985182));
#28885=CARTESIAN_POINT('Ctrl Pts',(54.9855948468531,19.0052474975823,18.8181662821324));
#28886=CARTESIAN_POINT('Ctrl Pts',(55.0830677673982,19.0052642313653,18.8244874088679));
#28887=CARTESIAN_POINT('Ctrl Pts',(55.1657010683349,19.0104244140644,18.8300115289142));
#28888=CARTESIAN_POINT('Ctrl Pts',(55.4002460553659,19.0397844651118,18.8461485552684));
#28889=CARTESIAN_POINT('Ctrl Pts',(55.5499937451085,19.0764243864063,18.8570456105036));
#28890=CARTESIAN_POINT('Ctrl Pts',(55.7258940761164,19.1417052287217,18.86987739487));
#28891=CARTESIAN_POINT('Ctrl Pts',(55.7574383189822,19.1543377533466,18.8721773553897));
#28892=CARTESIAN_POINT('Ctrl Pts',(55.8078384912854,19.1760314912753,18.8758340144915));
#28893=CARTESIAN_POINT('Ctrl Pts',(55.8269007222035,19.1845938668317,18.8772127140775));
#28894=CARTESIAN_POINT('Ctrl Pts',(55.8520556419838,19.1963714172464,18.8790229733888));
#28895=CARTESIAN_POINT('Ctrl Pts',(55.8582704862637,19.1993205012178,18.879469472828));
#28896=CARTESIAN_POINT('Ctrl Pts',(55.8684867444005,19.2042332551658,18.8802020628601));
#28897=CARTESIAN_POINT('Ctrl Pts',(55.8724969923835,19.2061782623995,18.8804892765138));
#28898=CARTESIAN_POINT('Ctrl Pts',(55.8803538291335,19.210021481499,18.881051236974));
#28899=CARTESIAN_POINT('Ctrl Pts',(55.8842008600772,19.2119186817273,18.8813260406449));
#28900=CARTESIAN_POINT('Ctrl Pts',(55.8936745482161,19.2166287724571,18.8820019655575));
#28901=CARTESIAN_POINT('Ctrl Pts',(55.8992941366587,19.2194559281791,18.88240220631));
#28902=CARTESIAN_POINT('Ctrl Pts',(55.9186199264016,19.2292933636027,18.8837765290042));
#28903=CARTESIAN_POINT('Ctrl Pts',(55.9322586938332,19.2364359032744,18.8847427592111));
#28904=CARTESIAN_POINT('Ctrl Pts',(56.0595658203018,19.304995550461,18.8937399942552));
#28905=CARTESIAN_POINT('Ctrl Pts',(56.1671140392041,19.3771709353203,18.9011894054926));
#28906=CARTESIAN_POINT('Ctrl Pts',(56.3797709982094,19.5520358888799,18.9171628638262));
#28907=CARTESIAN_POINT('Ctrl Pts',(56.4820569208504,19.656918540189,18.9256729962863));
#28908=CARTESIAN_POINT('Ctrl Pts',(56.5827496905881,19.7858181602609,18.9358218910243));
#28909=CARTESIAN_POINT('Ctrl Pts',(56.5933458396525,19.7997570547188,18.9369151002039));
#28910=CARTESIAN_POINT('Ctrl Pts',(56.6091831877372,19.821169943452,18.9385889967104));
#28911=CARTESIAN_POINT('Ctrl Pts',(56.6145590233695,19.8285436459229,18.9391644440272));
#28912=CARTESIAN_POINT('Ctrl Pts',(56.6238162816745,19.8414260260623,18.9401682375366));
#28913=CARTESIAN_POINT('Ctrl Pts',(56.6277207655822,19.8469180093384,18.9405956870642));
#28914=CARTESIAN_POINT('Ctrl Pts',(56.6364186979856,19.8592845912053,18.9415571721671));
#28915=CARTESIAN_POINT('Ctrl Pts',(56.641196777209,19.8661697949329,18.9420917835269));
#28916=CARTESIAN_POINT('Ctrl Pts',(56.6538604544527,19.8846659006487,18.9435261857914));
#28917=CARTESIAN_POINT('Ctrl Pts',(56.6616670175088,19.8963300936447,18.9444289338833));
#28918=CARTESIAN_POINT('Ctrl Pts',(56.6961341467995,19.9490239280437,18.9484997829654));
#28919=CARTESIAN_POINT('Ctrl Pts',(56.7214007537069,19.990940783661,18.9517187949409));
#28920=CARTESIAN_POINT('Ctrl Pts',(56.8275093696642,20.1825768818737,18.9663612683641));
#28921=CARTESIAN_POINT('Ctrl Pts',(56.8905319436068,20.3413320469431,18.9783755644266));
#28922=CARTESIAN_POINT('Ctrl Pts',(56.9487071097244,20.5689800820716,18.9946153425056));
#28923=CARTESIAN_POINT('Ctrl Pts',(56.9616968761499,20.6325974655493,18.999042275886));
#28924=CARTESIAN_POINT('Ctrl Pts',(56.9736747446051,20.7104685202268,19.0042442285143));
#28925=CARTESIAN_POINT('Ctrl Pts',(56.9756429530676,20.7242185227259,19.0051545938565));
#28926=CARTESIAN_POINT('Ctrl Pts',(56.9782378569705,20.7438029162838,19.0064385917439));
#28927=CARTESIAN_POINT('Ctrl Pts',(56.9789826328377,20.7496208764765,19.0068184463785));
#28928=CARTESIAN_POINT('Ctrl Pts',(56.980223270161,20.7596638648082,19.0074713231178));
#28929=CARTESIAN_POINT('Ctrl Pts',(56.980731294894,20.7638873227034,19.0077450187738));
#28930=CARTESIAN_POINT('Ctrl Pts',(56.9817618282143,20.7726921051408,19.0083137663207));
#28931=CARTESIAN_POINT('Ctrl Pts',(56.9822819656755,20.7772736377574,19.0086086852659));
#28932=CARTESIAN_POINT('Ctrl Pts',(56.9836145891381,20.789386367956,19.0093857825045));
#28933=CARTESIAN_POINT('Ctrl Pts',(56.9844000809099,20.7969205487186,19.0098664725015));
#28934=CARTESIAN_POINT('Ctrl Pts',(56.9875450505553,20.8288484750968,19.0118929118764));
#28935=CARTESIAN_POINT('Ctrl Pts',(56.9894979076109,20.853281301279,19.0134174621401));
#28936=CARTESIAN_POINT('Ctrl Pts',(56.9994446793162,21.0152710298696,19.0233887507599));
#28937=CARTESIAN_POINT('Ctrl Pts',(56.9936185569763,21.1533185713378,19.0312550500828));
#28938=CARTESIAN_POINT('Ctrl Pts',(56.9633649545991,21.3594405805898,19.0433684390515));
#28939=CARTESIAN_POINT('Ctrl Pts',(56.9494338727199,21.4286095605217,19.0474941419294));
#28940=CARTESIAN_POINT('Ctrl Pts',(56.9168038199123,21.5554721118379,19.0553294145845));
#28941=CARTESIAN_POINT('Ctrl Pts',(56.8990813714044,21.6133310825879,19.059010236262));
#28942=CARTESIAN_POINT('Ctrl Pts',(56.8739157975448,21.6838676103112,19.0636753812177));
#28943=CARTESIAN_POINT('Ctrl Pts',(56.868925403165,21.6973902385962,19.064577949759));
#28944=CARTESIAN_POINT('Ctrl Pts',(56.8607727625021,21.718765557537,19.0660182472214));
#28945=CARTESIAN_POINT('Ctrl Pts',(56.8577062624627,21.7266544152496,19.066552774916));
#28946=CARTESIAN_POINT('Ctrl Pts',(56.851837472589,21.741472454897,19.0675625117386));
#28947=CARTESIAN_POINT('Ctrl Pts',(56.8490462549128,21.7484058865056,19.0680373415218));
#28948=CARTESIAN_POINT('Ctrl Pts',(56.8426724697429,21.7639851541,19.0691096997419));
#28949=CARTESIAN_POINT('Ctrl Pts',(56.8390679101149,21.7726217467077,19.0697079636187));
#28950=CARTESIAN_POINT('Ctrl Pts',(56.8296872124572,21.7946604581037,19.0712444747469));
#28951=CARTESIAN_POINT('Ctrl Pts',(56.8238246087663,21.8080249481113,19.0721856405075));
#28952=CARTESIAN_POINT('Ctrl Pts',(56.7854309130868,21.8930008009626,19.0782314167247));
#28953=CARTESIAN_POINT('Ctrl Pts',(56.7488389785588,21.9626907338934,19.0834749306784));
#28954=CARTESIAN_POINT('Ctrl Pts',(56.6433048237484,22.1377114784355,19.09739769515));
#28955=CARTESIAN_POINT('Ctrl Pts',(56.5683430000971,22.239005197639,19.1062382761555));
#28956=CARTESIAN_POINT('Ctrl Pts',(56.4333577097724,22.389367217848,19.1202550848713));
#28957=CARTESIAN_POINT('Ctrl Pts',(56.3791340580155,22.4432073183055,19.1254893040685));
#28958=CARTESIAN_POINT('Ctrl Pts',(56.3119880604447,22.502628334578,19.1314041193109));
#28959=CARTESIAN_POINT('Ctrl Pts',(56.3019361160822,22.5113460739271,19.1322756212419));
#28960=CARTESIAN_POINT('Ctrl Pts',(56.2874049583898,22.5236959226534,19.133514692726));
#28961=CARTESIAN_POINT('Ctrl Pts',(56.2829963113869,22.5274099837878,19.133887920117));
#28962=CARTESIAN_POINT('Ctrl Pts',(56.2753188896451,22.5338211270435,19.1345331175107));
#28963=CARTESIAN_POINT('Ctrl Pts',(56.2720575298319,22.5365269806357,19.1348057181737));
#28964=CARTESIAN_POINT('Ctrl Pts',(56.265196074598,22.5421829066819,19.1353761067526));
#28965=CARTESIAN_POINT('Ctrl Pts',(56.2615942647183,22.545130783185,19.1356737389799));
#28966=CARTESIAN_POINT('Ctrl Pts',(56.2519521153634,22.5529661410109,19.1364658617054));
#28967=CARTESIAN_POINT('Ctrl Pts',(56.2458934082106,22.5578310416755,19.1369587592221));
#28968=CARTESIAN_POINT('Ctrl Pts',(56.2192646124145,22.5789581827537,19.1391048146271));
#28969=CARTESIAN_POINT('Ctrl Pts',(56.1984023821149,22.5948501572263,19.1407335595669));
#28970=CARTESIAN_POINT('Ctrl Pts',(56.0057508557561,22.7356883109164,19.155364529448));
#28971=CARTESIAN_POINT('Ctrl Pts',(55.8153320901779,22.8328687894064,19.1670536088278));
#28972=CARTESIAN_POINT('Ctrl Pts',(55.5605167343166,22.9151780027317,19.1831270554104));
#28973=CARTESIAN_POINT('Ctrl Pts',(55.5072127802324,22.9299793118287,19.1865012302363));
#28974=CARTESIAN_POINT('Ctrl Pts',(55.4397086254523,22.9457339430014,19.1908215268714));
#28975=CARTESIAN_POINT('Ctrl Pts',(55.4260180932031,22.9487772629551,19.191700066807));
#28976=CARTESIAN_POINT('Ctrl Pts',(55.4040994593774,22.9534076343674,19.1931108235232));
#28977=CARTESIAN_POINT('Ctrl Pts',(55.3958913136936,22.9550876766389,19.1936400645022));
#28978=CARTESIAN_POINT('Ctrl Pts',(55.3803279771533,22.9581711514163,19.1946454273428));
#28979=CARTESIAN_POINT('Ctrl Pts',(55.3729749745889,22.9595849801089,19.1951212084902));
#28980=CARTESIAN_POINT('Ctrl Pts',(55.3562793278265,22.9626978303845,19.1962033830579));
#28981=CARTESIAN_POINT('Ctrl Pts',(55.3469322156051,22.9643715955625,19.1968105677649));
#28982=CARTESIAN_POINT('Ctrl Pts',(55.3227450990553,22.9685247095706,19.198385334843));
#28983=CARTESIAN_POINT('Ctrl Pts',(55.3078885737934,22.9709029749561,19.1993560871394));
#28984=CARTESIAN_POINT('Ctrl Pts',(55.2503105410471,22.9794533020705,19.2031325060876));
#28985=CARTESIAN_POINT('Ctrl Pts',(55.2074350719438,22.9844038814477,19.2059750470036));
#28986=CARTESIAN_POINT('Ctrl Pts',(55.1644482551197,22.9879598421216,19.2088565303878));
#28987=CARTESIAN_POINT('Origin',(55.,21.,6.22095488139522));
#28988=CARTESIAN_POINT('',(55.1644485224877,22.9879598200043,20.1685383772559));
#28989=CARTESIAN_POINT('',(55.1644483497948,22.9879598342899,20.0118645378774));
#28990=CARTESIAN_POINT('',(55.1644483516311,22.987959834138,6.22095488139522));
#28991=CARTESIAN_POINT('',(53.0052501477468,20.9992322527395,19.5807109120749));
#28992=CARTESIAN_POINT('Ctrl Pts',(55.1644485224877,22.9879598200043,20.1685383772559));
#28993=CARTESIAN_POINT('Ctrl Pts',(55.2068925657508,22.9844487529632,20.1655689947827));
#28994=CARTESIAN_POINT('Ctrl Pts',(55.2492396823092,22.9795771043672,20.1625933152215));
#28995=CARTESIAN_POINT('Ctrl Pts',(55.3776735384323,22.9606099556836,20.1535712346217));
#28996=CARTESIAN_POINT('Ctrl Pts',(55.4630056307296,22.9422301896129,20.147577910066));
#28997=CARTESIAN_POINT('Ctrl Pts',(55.5568977412209,22.9154637043003,20.141166337482));
#28998=CARTESIAN_POINT('Ctrl Pts',(55.5669034753316,22.9125262763177,20.1404855109366));
#28999=CARTESIAN_POINT('Ctrl Pts',(55.5819530740513,22.9079796123358,20.1394656324163));
#29000=CARTESIAN_POINT('Ctrl Pts',(55.5870141353317,22.9064285950373,20.1391233664781));
#29001=CARTESIAN_POINT('Ctrl Pts',(55.5960646797729,22.9036154988886,20.1385126525331));
#29002=CARTESIAN_POINT('Ctrl Pts',(55.600056408017,22.9023610010509,20.13824377459));
#29003=CARTESIAN_POINT('Ctrl Pts',(55.6087487066744,22.8995991526048,20.1376593184724));
#29004=CARTESIAN_POINT('Ctrl Pts',(55.6134476314019,22.8980869140415,20.1373440295626));
#29005=CARTESIAN_POINT('Ctrl Pts',(55.626747170255,22.8937522229867,20.1364533975958));
#29006=CARTESIAN_POINT('Ctrl Pts',(55.6353343864784,22.8908886065108,20.1358804056323));
#29007=CARTESIAN_POINT('Ctrl Pts',(55.6904512913292,22.872090664813,20.1322142100668));
#29008=CARTESIAN_POINT('Ctrl Pts',(55.7364019065688,22.8544971200174,20.1292107028611));
#29009=CARTESIAN_POINT('Ctrl Pts',(55.9126743407584,22.7794190039197,20.1177256518476));
#29010=CARTESIAN_POINT('Ctrl Pts',(56.0373446780462,22.7097450354183,20.1096565212819));
#29011=CARTESIAN_POINT('Ctrl Pts',(56.2308614065062,22.5725745027399,20.0957351796463));
#29012=CARTESIAN_POINT('Ctrl Pts',(56.3041702827222,22.5123315865029,20.0900687275271));
#29013=CARTESIAN_POINT('Ctrl Pts',(56.3839052386286,22.4366848540956,20.0832434936051));
#29014=CARTESIAN_POINT('Ctrl Pts',(56.3947764399891,22.426133143199,20.0822975786373));
#29015=CARTESIAN_POINT('Ctrl Pts',(56.4122876962951,22.4087447684215,20.0807479769109));
#29016=CARTESIAN_POINT('Ctrl Pts',(56.419000932948,22.4019824203177,20.08014754381));
#29017=CARTESIAN_POINT('Ctrl Pts',(56.4309062958685,22.389816852452,20.0790711186767));
#29018=CARTESIAN_POINT('Ctrl Pts',(56.4361169455721,22.3844319510374,20.0785959495107));
#29019=CARTESIAN_POINT('Ctrl Pts',(56.4470787788155,22.3729750595595,20.0775876269041));
#29020=CARTESIAN_POINT('Ctrl Pts',(56.4528223499427,22.3668960173567,20.0770541582223));
#29021=CARTESIAN_POINT('Ctrl Pts',(56.4680431136402,22.3505819301759,20.075626496364));
#29022=CARTESIAN_POINT('Ctrl Pts',(56.4774513255192,22.340283439406,20.0747293957232));
#29023=CARTESIAN_POINT('Ctrl Pts',(56.5229678364551,22.2893981528988,20.0703159827555));
#29024=CARTESIAN_POINT('Ctrl Pts',(56.5575128165892,22.2474500041035,20.0667357340029));
#29025=CARTESIAN_POINT('Ctrl Pts',(56.7110285342887,22.0447040053157,20.0496818824254));
#29026=CARTESIAN_POINT('Ctrl Pts',(56.8070677364786,21.8680489617466,20.0353749807913));
#29027=CARTESIAN_POINT('Ctrl Pts',(56.888131111058,21.6445302884007,20.0192556003222));
#29028=CARTESIAN_POINT('Ctrl Pts',(56.9000145208163,21.6086079578724,20.0167264169441));
#29029=CARTESIAN_POINT('Ctrl Pts',(56.9133725609547,21.5640115935997,20.0136791359467));
#29030=CARTESIAN_POINT('Ctrl Pts',(56.9158204343277,21.5556399057395,20.0131110669112));
#29031=CARTESIAN_POINT('Ctrl Pts',(56.9195624907968,21.5425233534145,20.012227518829));
#29032=CARTESIAN_POINT('Ctrl Pts',(56.9208941362448,21.5377894231772,20.0119099514943));
#29033=CARTESIAN_POINT('Ctrl Pts',(56.9233268667823,21.529016869178,20.0113239570294));
#29034=CARTESIAN_POINT('Ctrl Pts',(56.9244327389331,21.5249797312436,20.0110552649709));
#29035=CARTESIAN_POINT('Ctrl Pts',(56.9269146787255,21.515805837139,20.0104469017423));
#29036=CARTESIAN_POINT('Ctrl Pts',(56.9282829170921,21.5106670480304,20.0101076842579));
#29037=CARTESIAN_POINT('Ctrl Pts',(56.932392922781,21.4949787484439,20.00907665891));
#29038=CARTESIAN_POINT('Ctrl Pts',(56.9350688413667,21.4844119747152,20.0083885163746));
#29039=CARTESIAN_POINT('Ctrl Pts',(56.94107266634,21.4598598798263,20.006803049675));
#29040=CARTESIAN_POINT('Ctrl Pts',(56.9443363169651,21.4458593022139,20.0059090169516));
#29041=CARTESIAN_POINT('Ctrl Pts',(56.9824281581862,21.2740720558003,19.9950484346713));
#29042=CARTESIAN_POINT('Ctrl Pts',(56.9981154240316,21.1126331009586,19.9859281415125));
#29043=CARTESIAN_POINT('Ctrl Pts',(56.9915269694546,20.8442136350118,19.9702403132308));
#29044=CARTESIAN_POINT('Ctrl Pts',(56.9803234833983,20.7377720854204,19.9638886483225));
#29045=CARTESIAN_POINT('Ctrl Pts',(56.9578064547157,20.617560178734,19.9562969303724));
#29046=CARTESIAN_POINT('Ctrl Pts',(56.9547852568531,20.6024060996335,19.9553324358982));
#29047=CARTESIAN_POINT('Ctrl Pts',(56.9495980750784,20.5778774511832,19.953758448497));
#29048=CARTESIAN_POINT('Ctrl Pts',(56.9475397526504,20.5684805830598,19.9531523842822));
#29049=CARTESIAN_POINT('Ctrl Pts',(56.9437550286249,20.5517810174614,19.9520696869347));
#29050=CARTESIAN_POINT('Ctrl Pts',(56.9420552260762,20.5444724333594,19.9515939138762));
#29051=CARTESIAN_POINT('Ctrl Pts',(56.9383856057007,20.5290882241893,19.9505882855224));
#29052=CARTESIAN_POINT('Ctrl Pts',(56.936406469353,20.5210149908562,19.9500581385882));
#29053=CARTESIAN_POINT('Ctrl Pts',(56.9310276047434,20.4996519950869,19.9486487514117));
#29054=CARTESIAN_POINT('Ctrl Pts',(56.9275411953813,20.4863847151677,19.9477667332299));
#29055=CARTESIAN_POINT('Ctrl Pts',(56.9103017794413,20.4234303167523,19.943548601787));
#29056=CARTESIAN_POINT('Ctrl Pts',(56.8947638294469,20.3742566725778,19.9401552042871));
#29057=CARTESIAN_POINT('Ctrl Pts',(56.8182924566594,20.161336567381,19.9250135828607));
#29058=CARTESIAN_POINT('Ctrl Pts',(56.7379064757038,20.0054107632745,19.9126472932553));
#29059=CARTESIAN_POINT('Ctrl Pts',(56.6290782609817,19.8487435828613,19.8994990849802));
#29060=CARTESIAN_POINT('Ctrl Pts',(56.6197231540655,19.8356185147986,19.8983922274142));
#29061=CARTESIAN_POINT('Ctrl Pts',(56.5813444803813,19.7831315618491,19.8939481734097));
#29062=CARTESIAN_POINT('Ctrl Pts',(56.5510343901165,19.7447261804967,19.89065524359));
#29063=CARTESIAN_POINT('Ctrl Pts',(56.5137840228758,19.7009391742751,19.8868871761587));
#29064=CARTESIAN_POINT('Ctrl Pts',(56.5081853980093,19.6944434487974,19.8863278299679));
#29065=CARTESIAN_POINT('Ctrl Pts',(56.4990294406559,19.6839578783113,19.885424617158));
#29066=CARTESIAN_POINT('Ctrl Pts',(56.4954977253194,19.6799459536861,19.8850789629116));
#29067=CARTESIAN_POINT('Ctrl Pts',(56.4891700794169,19.6728159224833,19.8844646100367));
#29068=CARTESIAN_POINT('Ctrl Pts',(56.4863804195372,19.6696923849885,19.8841954593919));
#29069=CARTESIAN_POINT('Ctrl Pts',(56.4803070036286,19.6629350338627,19.8836131686394));
#29070=CARTESIAN_POINT('Ctrl Pts',(56.4770197005771,19.6593045259956,19.8833003003856));
#29071=CARTESIAN_POINT('Ctrl Pts',(56.4677394973076,19.6491310001588,19.8824233839512));
#29072=CARTESIAN_POINT('Ctrl Pts',(56.461716175867,19.6426157084796,19.8818615734112));
#29073=CARTESIAN_POINT('Ctrl Pts',(56.4244841058512,19.6028778546974,19.8784320280204));
#29074=CARTESIAN_POINT('Ctrl Pts',(56.3921850067446,19.5706900649949,19.8756411600798));
#29075=CARTESIAN_POINT('Ctrl Pts',(56.2711269226517,19.4580506009503,19.8656981913342));
#29076=CARTESIAN_POINT('Ctrl Pts',(56.1762697154891,19.3845231516665,19.8588476372468));
#29077=CARTESIAN_POINT('Ctrl Pts',(55.9738486166519,19.2549557580819,19.8448576589149));
#29078=CARTESIAN_POINT('Ctrl Pts',(55.8666466787993,19.199311704218,19.8377406684143));
#29079=CARTESIAN_POINT('Ctrl Pts',(55.7406842837202,19.1477968583911,19.829294390675));
#29080=CARTESIAN_POINT('Ctrl Pts',(55.7262137737636,19.1420755614667,19.8283232495568));
#29081=CARTESIAN_POINT('Ctrl Pts',(55.7026612586077,19.1330806443398,19.8267405453512));
#29082=CARTESIAN_POINT('Ctrl Pts',(55.6936196485723,19.1297025630317,19.8261324746091));
#29083=CARTESIAN_POINT('Ctrl Pts',(55.6775023375678,19.1238138394213,19.8250475289918));
#29084=CARTESIAN_POINT('Ctrl Pts',(55.670436261774,19.121277257566,19.8245715274688));
#29085=CARTESIAN_POINT('Ctrl Pts',(55.6555332613929,19.1160221572389,19.8235667945475));
#29086=CARTESIAN_POINT('Ctrl Pts',(55.6476933788636,19.1133125186303,19.8230377796548));
#29087=CARTESIAN_POINT('Ctrl Pts',(55.6269187105331,19.1062770762251,19.8216346175487));
#29088=CARTESIAN_POINT('Ctrl Pts',(55.6139562465485,19.1020349598471,19.8207577359749));
#29089=CARTESIAN_POINT('Ctrl Pts',(55.5526555776869,19.0826672925725,19.8166036979754));
#29090=CARTESIAN_POINT('Ctrl Pts',(55.5037999514034,19.0692546150528,19.813271354255));
#29091=CARTESIAN_POINT('Ctrl Pts',(55.2896497763713,19.0191439196562,19.7985610711798));
#29092=CARTESIAN_POINT('Ctrl Pts',(55.1205826956811,19.0017178666944,19.7866052978476));
#29093=CARTESIAN_POINT('Ctrl Pts',(54.8813061483446,19.0075508506724,19.7700633461535));
#29094=CARTESIAN_POINT('Ctrl Pts',(54.8113555479435,19.012952615346,19.7652859010389));
#29095=CARTESIAN_POINT('Ctrl Pts',(54.7316989150764,19.0233496943716,19.7600124900731));
#29096=CARTESIAN_POINT('Ctrl Pts',(54.7215801589999,19.0247495587463,19.7593457524462));
#29097=CARTESIAN_POINT('Ctrl Pts',(54.7062796539748,19.0269861984518,19.7583427951155));
#29098=CARTESIAN_POINT('Ctrl Pts',(54.7010899026329,19.0277657699983,19.7580035136203));
#29099=CARTESIAN_POINT('Ctrl Pts',(54.6917705275639,19.0292032980762,19.7573959660451));
#29100=CARTESIAN_POINT('Ctrl Pts',(54.6876398614154,19.0298537635999,19.7571272895497));
#29101=CARTESIAN_POINT('Ctrl Pts',(54.6786017645963,19.0313061535103,19.7565407508599));
#29102=CARTESIAN_POINT('Ctrl Pts',(54.6736952850307,19.0321134379197,19.7562231940534));
#29103=CARTESIAN_POINT('Ctrl Pts',(54.659699085798,19.0344700785973,19.7553196439212));
#29104=CARTESIAN_POINT('Ctrl Pts',(54.6506168770577,19.0360641493851,19.7547361109213));
#29105=CARTESIAN_POINT('Ctrl Pts',(54.5894479640549,19.0472380207953,19.7508228152732));
#29106=CARTESIAN_POINT('Ctrl Pts',(54.5377445535237,19.0588268201204,19.7475972640817));
#29107=CARTESIAN_POINT('Ctrl Pts',(54.3174720489465,19.1175010831857,19.7339747062371));
#29108=CARTESIAN_POINT('Ctrl Pts',(54.1550424812256,19.1845934450898,19.7241677248914));
#29109=CARTESIAN_POINT('Ctrl Pts',(53.9504336949272,19.3025953076205,19.7100558375068));
#29110=CARTESIAN_POINT('Ctrl Pts',(53.898864081405,19.3355869801227,19.7063364495535));
#29111=CARTESIAN_POINT('Ctrl Pts',(53.8366943943565,19.379515250865,19.7015990230936));
#29112=CARTESIAN_POINT('Ctrl Pts',(53.8245907743834,19.3882730108671,19.700664253588));
#29113=CARTESIAN_POINT('Ctrl Pts',(53.8056216393073,19.402325741884,19.6991788331372));
#29114=CARTESIAN_POINT('Ctrl Pts',(53.7986901565374,19.4075310490625,19.6986316615048));
#29115=CARTESIAN_POINT('Ctrl Pts',(53.7860799382922,19.417130076053,19.6976280383304));
#29116=CARTESIAN_POINT('Ctrl Pts',(53.7803905503967,19.4215096134015,19.6971721492099));
#29117=CARTESIAN_POINT('Ctrl Pts',(53.7746202439719,19.4260012599635,19.6967065927026));
#29118=CARTESIAN_POINT('Ctrl Pts',(53.7745155054043,19.426082805982,19.6966981411737));
#29119=CARTESIAN_POINT('Ctrl Pts',(53.774310284996,19.4262426167749,19.6966815794954));
#29120=CARTESIAN_POINT('Ctrl Pts',(53.7742098024999,19.4263208807273,19.6966734693784));
#29121=CARTESIAN_POINT('Ctrl Pts',(53.7740128039319,19.4264743495741,19.6966575673437));
#29122=CARTESIAN_POINT('Ctrl Pts',(53.7739162873851,19.426549553646,19.6966497754639));
#29123=CARTESIAN_POINT('Ctrl Pts',(53.7737269564555,19.4266971051241,19.6966344887941));
#29124=CARTESIAN_POINT('Ctrl Pts',(53.7736341415466,19.4267694518703,19.6966269940299));
#29125=CARTESIAN_POINT('Ctrl Pts',(53.7734519725674,19.4269114736481,19.696612282306));
#29126=CARTESIAN_POINT('Ctrl Pts',(53.7733626179518,19.426981148142,19.6966050653637));
#29127=CARTESIAN_POINT('Ctrl Pts',(53.7731871484474,19.4271179949871,19.696590891606));
#29128=CARTESIAN_POINT('Ctrl Pts',(53.7731010331595,19.427185166781,19.6965839348141));
#29129=CARTESIAN_POINT('Ctrl Pts',(53.7658317660991,19.4328563131827,19.6959966283242));
#29130=CARTESIAN_POINT('Ctrl Pts',(53.758687185818,19.438509347611,19.6954143322578));
#29131=CARTESIAN_POINT('Ctrl Pts',(53.743874080362,19.450395890613,19.6941963105001));
#29132=CARTESIAN_POINT('Ctrl Pts',(53.7362126675136,19.4566378279134,19.6935602554901));
#29133=CARTESIAN_POINT('Ctrl Pts',(53.7163741286914,19.4730475299799,19.6918971411821));
#29134=CARTESIAN_POINT('Ctrl Pts',(53.7042715482737,19.4833039267833,19.6908665168312));
#29135=CARTESIAN_POINT('Ctrl Pts',(53.6686113282836,19.5142627181813,19.6877810675712));
#29136=CARTESIAN_POINT('Ctrl Pts',(53.6454190792924,19.535376698602,19.6857096885247));
#29137=CARTESIAN_POINT('Ctrl Pts',(53.5106817081229,19.6639786375248,19.6732814911991));
#29138=CARTESIAN_POINT('Ctrl Pts',(53.4114802739554,19.7836063389707,19.6624158048673));
#29139=CARTESIAN_POINT('Ctrl Pts',(53.2792396776596,19.9872108322123,19.6455412103445));
#29140=CARTESIAN_POINT('Ctrl Pts',(53.2362702536912,20.0640411028892,19.6394949453696));
#29141=CARTESIAN_POINT('Ctrl Pts',(53.1940278570395,20.1528866520976,19.6330344712594));
#29142=CARTESIAN_POINT('Ctrl Pts',(53.1896219453678,20.1623439154723,19.6323532998204));
#29143=CARTESIAN_POINT('Ctrl Pts',(53.1830922351114,20.1766520983904,19.6313330074889));
#29144=CARTESIAN_POINT('Ctrl Pts',(53.1809133008997,20.181477443241,19.6309906688664));
#29145=CARTESIAN_POINT('Ctrl Pts',(53.1770467441223,20.1901318023486,19.630379877338));
#29146=CARTESIAN_POINT('Ctrl Pts',(53.175351939108,20.1939574914394,19.6301109940216));
#29147=CARTESIAN_POINT('Ctrl Pts',(53.1716843337103,20.2023072368301,19.6295265865118));
#29148=CARTESIAN_POINT('Ctrl Pts',(53.1697162839979,20.2068332834615,19.6292113511998));
#29149=CARTESIAN_POINT('Ctrl Pts',(53.164187932384,20.2196773245214,19.6283210237136));
#29150=CARTESIAN_POINT('Ctrl Pts',(53.1606673421879,20.2280124309603,19.6277482800863));
#29151=CARTESIAN_POINT('Ctrl Pts',(53.1384078926944,20.2817291656545,19.6240876069672));
#29152=CARTESIAN_POINT('Ctrl Pts',(53.1212915379535,20.3277697052877,19.6210890625608));
#29153=CARTESIAN_POINT('Ctrl Pts',(53.0393055075407,20.5759958794105,19.6054175802769));
#29154=CARTESIAN_POINT('Ctrl Pts',(53.0053318643117,20.7869174531364,19.5936625725931));
#29155=CARTESIAN_POINT('Ctrl Pts',(53.0052501477468,20.9992322527395,19.5807109120749));
#29156=CARTESIAN_POINT('Ctrl Pts',(53.0052501469746,20.9992342617848,19.5807107895187));
#29157=CARTESIAN_POINT('Ctrl Pts',(53.0052371631856,21.0330570625816,19.5786475248104));
#29158=CARTESIAN_POINT('Ctrl Pts',(53.0060844221468,21.0668734766943,19.5765607928456));
#29159=CARTESIAN_POINT('Ctrl Pts',(53.0082529989016,21.1097966440269,19.5738751223118));
#29160=CARTESIAN_POINT('Ctrl Pts',(53.0087780256483,21.1189389080265,19.5733009712841));
#29161=CARTESIAN_POINT('Ctrl Pts',(53.0098294143081,21.135280079236,19.5722707643735));
#29162=CARTESIAN_POINT('Ctrl Pts',(53.0103319388128,21.1424803989021,19.5718154567695));
#29163=CARTESIAN_POINT('Ctrl Pts',(53.0114234462309,21.156985869494,19.5708953708877));
#29164=CARTESIAN_POINT('Ctrl Pts',(53.0120136320268,21.1642908148114,19.5704305618937));
#29165=CARTESIAN_POINT('Ctrl Pts',(53.0133666780071,21.1799615911391,19.5694302443483));
#29166=CARTESIAN_POINT('Ctrl Pts',(53.0141421543837,21.1883261632965,19.5688943483502));
#29167=CARTESIAN_POINT('Ctrl Pts',(53.0163624924566,21.2107347144899,19.5674533198062));
#29168=CARTESIAN_POINT('Ctrl Pts',(53.0179036343077,21.2247684615977,19.5665451835389));
#29169=CARTESIAN_POINT('Ctrl Pts',(53.025169795944,21.2850318402525,19.5626203544289));
#29170=CARTESIAN_POINT('Ctrl Pts',(53.0323638547637,21.3310662888805,19.5595580230171));
#29171=CARTESIAN_POINT('Ctrl Pts',(53.0778666466899,21.5676153984877,19.5434780508149));
#29172=CARTESIAN_POINT('Ctrl Pts',(53.1422567129725,21.7520306695359,19.5296374991767));
#29173=CARTESIAN_POINT('Ctrl Pts',(53.2556018130522,21.9688355601604,19.5129086321886));
#29174=CARTESIAN_POINT('Ctrl Pts',(53.2806371710585,22.0126005140549,19.5095144760629));
#29175=CARTESIAN_POINT('Ctrl Pts',(53.3121247011643,22.0631027681698,19.5056166761565));
#29176=CARTESIAN_POINT('Ctrl Pts',(53.3169965703753,22.0707987596201,19.5050232392136));
#29177=CARTESIAN_POINT('Ctrl Pts',(53.3245963776032,22.0826240113679,19.5041125670641));
#29178=CARTESIAN_POINT('Ctrl Pts',(53.32728717751,22.0867768228566,19.5037929807899));
#29179=CARTESIAN_POINT('Ctrl Pts',(53.332281251709,22.0944218742721,19.5032051232543));
#29180=CARTESIAN_POINT('Ctrl Pts',(53.3345800453534,22.0979168627573,19.5029365731739));
#29181=CARTESIAN_POINT('Ctrl Pts',(53.3398040465678,22.105805052509,19.5023308718945));
#29182=CARTESIAN_POINT('Ctrl Pts',(53.3427357003899,22.1101938842967,19.5019941575711));
#29183=CARTESIAN_POINT('Ctrl Pts',(53.3514705647922,22.123158709302,19.5010001715235));
#29184=CARTESIAN_POINT('Ctrl Pts',(53.3573232774822,22.1317013657367,19.5003461159191));
#29185=CARTESIAN_POINT('Ctrl Pts',(53.4092020266819,22.206173445886,19.4946484646242));
#29186=CARTESIAN_POINT('Ctrl Pts',(53.4591147094195,22.2693180566445,19.4898451893965));
#29187=CARTESIAN_POINT('Ctrl Pts',(53.5957691520135,22.4222161164272,19.477805380152));
#29188=CARTESIAN_POINT('Ctrl Pts',(53.687355306074,22.5071587836494,19.4706957785555));
#29189=CARTESIAN_POINT('Ctrl Pts',(53.8288123647533,22.615617778181,19.4601615225846));
#29190=CARTESIAN_POINT('Ctrl Pts',(53.8726488913392,22.6465054272489,19.456953440164));
#29191=CARTESIAN_POINT('Ctrl Pts',(53.9370828462569,22.6881257579331,19.4522742454483));
#29192=CARTESIAN_POINT('Ctrl Pts',(53.9567076222584,22.7003242042576,19.450853806563));
#29193=CARTESIAN_POINT('Ctrl Pts',(53.987515511676,22.7187397268907,19.4486284417327));
#29194=CARTESIAN_POINT('Ctrl Pts',(53.9985543751627,22.7251949850885,19.4478319507107));
#29195=CARTESIAN_POINT('Ctrl Pts',(54.0193504056747,22.7370891465052,19.4463326301377));
#29196=CARTESIAN_POINT('Ctrl Pts',(54.0290927122807,22.7425531154884,19.4456307237154));
#29197=CARTESIAN_POINT('Ctrl Pts',(54.0456129294963,22.7516369248106,19.4444410495563));
#29198=CARTESIAN_POINT('Ctrl Pts',(54.0523668748041,22.7552999897592,19.4439548334359));
#29199=CARTESIAN_POINT('Ctrl Pts',(54.0658674139152,22.7625215038587,19.4429831605944));
#29200=CARTESIAN_POINT('Ctrl Pts',(54.0726135905341,22.7660804581988,19.4424977322375));
#29201=CARTESIAN_POINT('Ctrl Pts',(54.0875067382461,22.7738284950377,19.441426249969));
#29202=CARTESIAN_POINT('Ctrl Pts',(54.0956624534876,22.7780003036803,19.4408396008201));
#29203=CARTESIAN_POINT('Ctrl Pts',(54.1243865609606,22.7924444886978,19.4387736458949));
#29204=CARTESIAN_POINT('Ctrl Pts',(54.145102900839,22.8024169928704,19.4372839739443));
#29205=CARTESIAN_POINT('Ctrl Pts',(54.3173800160284,22.8817101429592,19.4248937712895));
#29206=CARTESIAN_POINT('Ctrl Pts',(54.4768823188497,22.932130734221,19.4133262550094));
#29207=CARTESIAN_POINT('Ctrl Pts',(54.7154101072182,22.9758028013711,19.3964193239194));
#29208=CARTESIAN_POINT('Ctrl Pts',(54.7907916730864,22.9852006129768,19.3911449524743));
#29209=CARTESIAN_POINT('Ctrl Pts',(54.8902459032051,22.9918701242246,19.3844030382907));
#29210=CARTESIAN_POINT('Ctrl Pts',(54.9139898417861,22.9930366057191,19.3828098068299));
#29211=CARTESIAN_POINT('Ctrl Pts',(54.95379973578,22.9942795547432,19.3801718621156));
#29212=CARTESIAN_POINT('Ctrl Pts',(54.9698555359257,22.9945868638877,19.3791170211022));
#29213=CARTESIAN_POINT('Ctrl Pts',(54.9921299514766,22.9947441605632,19.3776677986508));
#29214=CARTESIAN_POINT('Ctrl Pts',(54.9983462787192,22.9947590008506,19.3772648817731));
#29215=CARTESIAN_POINT('Ctrl Pts',(55.0088813151271,22.9947349035656,19.3765847534222));
#29216=CARTESIAN_POINT('Ctrl Pts',(55.0131999822727,22.9947110003732,19.3763067179034));
#29217=CARTESIAN_POINT('Ctrl Pts',(55.0214688473508,22.9946383774056,19.3757758886985));
#29218=CARTESIAN_POINT('Ctrl Pts',(55.0254190081611,22.9945919489241,19.3755229643999));
#29219=CARTESIAN_POINT('Ctrl Pts',(55.0348448988605,22.9944531548722,19.3749209568026));
#29220=CARTESIAN_POINT('Ctrl Pts',(55.0403204729803,22.9943499730766,19.3745724711733));
#29221=CARTESIAN_POINT('Ctrl Pts',(55.059856266311,22.9939013505279,19.3733332932094));
#29222=CARTESIAN_POINT('Ctrl Pts',(55.0739135629932,22.9934297529035,19.3724492966085));
#29223=CARTESIAN_POINT('Ctrl Pts',(55.1134988303262,22.9916824086026,19.3699786420784));
#29224=CARTESIAN_POINT('Ctrl Pts',(55.138997925654,22.9900651497633,19.3684090424697));
#29225=CARTESIAN_POINT('Ctrl Pts',(55.1644484414294,22.9879598267096,19.3668580791575));
#29226=CARTESIAN_POINT('Ctrl Pts',(55.1644482551197,22.9879598421216,19.2088565303878));
#29227=CARTESIAN_POINT('Ctrl Pts',(55.1164235541647,22.9919325472575,19.2120757121755));
#29228=CARTESIAN_POINT('Ctrl Pts',(55.0682598856658,22.9941646009509,19.2153436145953));
#29229=CARTESIAN_POINT('Ctrl Pts',(54.8745044393767,22.9961123335879,19.2286277370617));
#29230=CARTESIAN_POINT('Ctrl Pts',(54.7292455990042,22.9816412960441,19.2389382050322));
#29231=CARTESIAN_POINT('Ctrl Pts',(54.5383242544354,22.941222362976,19.2522759805422));
#29232=CARTESIAN_POINT('Ctrl Pts',(54.490185009616,22.9291392781345,19.2556155999308));
#29233=CARTESIAN_POINT('Ctrl Pts',(54.433833685962,22.9127377060894,19.259459113372));
#29234=CARTESIAN_POINT('Ctrl Pts',(54.4251422512942,22.9101435557911,19.2600500342616));
#29235=CARTESIAN_POINT('Ctrl Pts',(54.4117454702894,22.9060452687648,19.2609576191734));
#29236=CARTESIAN_POINT('Ctrl Pts',(54.4070276443249,22.9045828270238,19.2612766105901));
#29237=CARTESIAN_POINT('Ctrl Pts',(54.3983247978874,22.9018496280869,19.2618638273113));
#29238=CARTESIAN_POINT('Ctrl Pts',(54.394338365156,22.9005838685347,19.2621323278565));
#29239=CARTESIAN_POINT('Ctrl Pts',(54.3853229523286,22.8976900771953,19.2627384815896));
#29240=CARTESIAN_POINT('Ctrl Pts',(54.3802964521158,22.896054592123,19.2630756941362));
#29241=CARTESIAN_POINT('Ctrl Pts',(54.3673156402131,22.8917738579905,19.2639447506841));
#29242=CARTESIAN_POINT('Ctrl Pts',(54.3593712999462,22.8890983837241,19.2644748792226));
#29243=CARTESIAN_POINT('Ctrl Pts',(54.3087899700228,22.8717079563113,19.267840481561));
#29244=CARTESIAN_POINT('Ctrl Pts',(54.2666419600412,22.855599273756,19.2706008833762));
#29245=CARTESIAN_POINT('Ctrl Pts',(54.2036781179509,22.8290538877672,19.2747087804833));
#29246=CARTESIAN_POINT('Ctrl Pts',(54.1824417261714,22.8196607363434,19.2760914732854));
#29247=CARTESIAN_POINT('Ctrl Pts',(54.0052082832568,22.7375386556203,19.287645036104));
#29248=CARTESIAN_POINT('Ctrl Pts',(53.8590674237203,22.6452742426492,19.2973325736992));
#29249=CARTESIAN_POINT('Ctrl Pts',(53.7005386125679,22.5137940129388,19.3097310430515));
#29250=CARTESIAN_POINT('Ctrl Pts',(53.675051928234,22.4915376723493,19.3117888414203));
#29251=CARTESIAN_POINT('Ctrl Pts',(53.6321441004869,22.4521003878389,19.3153775061418));
#29252=CARTESIAN_POINT('Ctrl Pts',(53.6144500044582,22.4352269599802,19.3168959022713));
#29253=CARTESIAN_POINT('Ctrl Pts',(53.5896577241284,22.4106987554048,19.3190819021862));
#29254=CARTESIAN_POINT('Ctrl Pts',(53.5823021147227,22.4033064572881,19.3197380544933));
#29255=CARTESIAN_POINT('Ctrl Pts',(53.5696699360315,22.3904105851689,19.3208783377645));
#29256=CARTESIAN_POINT('Ctrl Pts',(53.5643662833939,22.3849337588327,19.321361270751));
#29257=CARTESIAN_POINT('Ctrl Pts',(53.5542360562668,22.3743520421015,19.3222918543878));
#29258=CARTESIAN_POINT('Ctrl Pts',(53.5494047897019,22.3692517848848,19.3227392916359));
#29259=CARTESIAN_POINT('Ctrl Pts',(53.5380750332793,22.3571639583152,19.3237972382723));
#29260=CARTESIAN_POINT('Ctrl Pts',(53.531599587864,22.3501551179287,19.3244087188796));
#29261=CARTESIAN_POINT('Ctrl Pts',(53.5091619929107,22.3255169476345,19.3265517176119));
#29262=CARTESIAN_POINT('Ctrl Pts',(53.4934655467442,22.3076494185639,19.3280942903949));
#29263=CARTESIAN_POINT('Ctrl Pts',(53.3821769886106,22.1763039006498,19.339356246757));
#29264=CARTESIAN_POINT('Ctrl Pts',(53.2992079854051,22.0527739587075,19.3495891113861));
#29265=CARTESIAN_POINT('Ctrl Pts',(53.1750738120978,21.8143620607659,19.3683360480522));
#29266=CARTESIAN_POINT('Ctrl Pts',(53.1292260147525,21.7026747310107,19.3767583772891));
#29267=CARTESIAN_POINT('Ctrl Pts',(53.0899288958268,21.5751721234695,19.3855546121299));
#29268=CARTESIAN_POINT('Ctrl Pts',(53.0862423046888,21.5627842386849,19.3864008089817));
#29269=CARTESIAN_POINT('Ctrl Pts',(53.0811043915696,21.5448850006598,19.3876105057389));
#29270=CARTESIAN_POINT('Ctrl Pts',(53.0795559647117,21.5394021962001,19.3879793094464));
#29271=CARTESIAN_POINT('Ctrl Pts',(53.0768994922329,21.5298394770684,19.3886194243245));
#29272=CARTESIAN_POINT('Ctrl Pts',(53.0757808965114,21.5257625676637,19.3888913375845));
#29273=CARTESIAN_POINT('Ctrl Pts',(53.0734497681459,21.5171592826609,19.3894630285431));
#29274=CARTESIAN_POINT('Ctrl Pts',(53.0722402196731,21.5126321780285,19.3897626344889));
#29275=CARTESIAN_POINT('Ctrl Pts',(53.0690312899238,21.5004498001904,19.3905656931775));
#29276=CARTESIAN_POINT('Ctrl Pts',(53.0670614579455,21.4927867281508,19.3910674749642));
#29277=CARTESIAN_POINT('Ctrl Pts',(53.0584401785665,21.4584008689281,19.3933048578202));
#29278=CARTESIAN_POINT('Ctrl Pts',(53.0522965714095,21.431552348586,19.3950134281741));
#29279=CARTESIAN_POINT('Ctrl Pts',(53.0192661032615,21.2720845587933,19.4049820283951));
#29280=CARTESIAN_POINT('Ctrl Pts',(53.0053715179969,21.1371217686103,19.4127076039949));
#29281=CARTESIAN_POINT('Ctrl Pts',(53.0052400231811,20.9897047796908,19.4212811242379));
#29282=CARTESIAN_POINT('Ctrl Pts',(53.0053388864299,20.9776304700278,19.4219841569368));
#29283=CARTESIAN_POINT('Ctrl Pts',(53.0074951688973,20.8527658903822,19.429267747121));
#29284=CARTESIAN_POINT('Ctrl Pts',(53.0190067377703,20.740357836622,19.4359529339334));
#29285=CARTESIAN_POINT('Ctrl Pts',(53.0428354453693,20.6142860386737,19.4439164798049));
#29286=CARTESIAN_POINT('Ctrl Pts',(53.0458951129595,20.5990730452447,19.4448849878315));
#29287=CARTESIAN_POINT('Ctrl Pts',(53.0511423179492,20.5744718761667,19.4464641469683));
#29288=CARTESIAN_POINT('Ctrl Pts',(53.053221000515,20.5650609571702,19.4470713303533));
#29289=CARTESIAN_POINT('Ctrl Pts',(53.0570392923982,20.5483501792133,19.4481551599258));
#29290=CARTESIAN_POINT('Ctrl Pts',(53.0587520607387,20.5410443292631,19.4486309379635));
#29291=CARTESIAN_POINT('Ctrl Pts',(53.062445683413,20.5256797513961,19.4496356802081));
#29292=CARTESIAN_POINT('Ctrl Pts',(53.0644356816222,20.5176233899194,19.4501649305873));
#29293=CARTESIAN_POINT('Ctrl Pts',(53.0698347957964,20.4963369153628,19.4515698360714));
#29294=CARTESIAN_POINT('Ctrl Pts',(53.073329615684,20.4831291910576,19.4524482390299));
#29295=CARTESIAN_POINT('Ctrl Pts',(53.0904968011746,20.4208450125265,19.4566230466793));
#29296=CARTESIAN_POINT('Ctrl Pts',(53.1059092393993,20.3722720515927,19.4599753212668));
#29297=CARTESIAN_POINT('Ctrl Pts',(53.180796879,20.1642486584671,19.4747661500816));
#29298=CARTESIAN_POINT('Ctrl Pts',(53.2586757381836,20.0121974587063,19.4867880933559));
#29299=CARTESIAN_POINT('Ctrl Pts',(53.3938778456414,19.8150294730267,19.5033030612794));
#29300=CARTESIAN_POINT('Ctrl Pts',(53.4358067592171,19.7602076220886,19.5080000140803));
#29301=CARTESIAN_POINT('Ctrl Pts',(53.4870892855641,19.6999106561882,19.5131958264936));
#29302=CARTESIAN_POINT('Ctrl Pts',(53.4937419824709,19.6922087602041,19.513860061296));
#29303=CARTESIAN_POINT('Ctrl Pts',(53.5039082788993,19.6806196263997,19.5148599504606));
#29304=CARTESIAN_POINT('Ctrl Pts',(53.5073786077768,19.6766948994329,19.5151986403122));
#29305=CARTESIAN_POINT('Ctrl Pts',(53.513645543789,19.6696634016772,19.515805489465));
#29306=CARTESIAN_POINT('Ctrl Pts',(53.5164364759301,19.6665517237775,19.5160740557362));
#29307=CARTESIAN_POINT('Ctrl Pts',(53.5225719554495,19.6597542369672,19.5166607704125));
#29308=CARTESIAN_POINT('Ctrl Pts',(53.5259205168586,19.6560721705251,19.5169786109325));
#29309=CARTESIAN_POINT('Ctrl Pts',(53.535529347177,19.6455854542032,19.5178840520559));
#29310=CARTESIAN_POINT('Ctrl Pts',(53.5418232935969,19.6388116384558,19.5184691753026));
#29311=CARTESIAN_POINT('Ctrl Pts',(53.5849303019189,19.5930601528613,19.5224250037372));
#29312=CARTESIAN_POINT('Ctrl Pts',(53.6232583050245,19.5555328261958,19.5256888725022));
#29313=CARTESIAN_POINT('Ctrl Pts',(53.798407688852,19.3973568163892,19.5397852195365));
#29314=CARTESIAN_POINT('Ctrl Pts',(53.9498845304327,19.2942582737765,19.5499850027547));
#29315=CARTESIAN_POINT('Ctrl Pts',(54.1617773051667,19.1891045072329,19.5641852042072));
#29316=CARTESIAN_POINT('Ctrl Pts',(54.2112390945761,19.1670201268651,19.5674883514007));
#29317=CARTESIAN_POINT('Ctrl Pts',(54.2749009167004,19.1416496814903,19.5717564531704));
#29318=CARTESIAN_POINT('Ctrl Pts',(54.288323927706,19.1364679402001,19.572657230165));
#29319=CARTESIAN_POINT('Ctrl Pts',(54.3098017083296,19.128442675443,19.5741004146536));
#29320=CARTESIAN_POINT('Ctrl Pts',(54.3178208802088,19.125504829087,19.5746396694983));
#29321=CARTESIAN_POINT('Ctrl Pts',(54.3328843918502,19.1200957325136,19.5756535073451));
#29322=CARTESIAN_POINT('Ctrl Pts',(54.3399242398537,19.1176123465302,19.5761276772201));
#29323=CARTESIAN_POINT('Ctrl Pts',(54.3557154848138,19.1121412823444,19.5771921778424));
#29324=CARTESIAN_POINT('Ctrl Pts',(54.3644740064394,19.1091748412168,19.5777831986893));
#29325=CARTESIAN_POINT('Ctrl Pts',(54.390439946614,19.1005811780775,19.579537314554));
#29326=CARTESIAN_POINT('Ctrl Pts',(54.4077033284704,19.0951273174334,19.5807060593448));
#29327=CARTESIAN_POINT('Ctrl Pts',(54.5437218857599,19.0541839786941,19.5899369008179));
#29328=CARTESIAN_POINT('Ctrl Pts',(54.6654553813722,19.0296041974743,19.5983565985381));
#29329=CARTESIAN_POINT('Ctrl Pts',(54.9241372785108,19.0020424536455,19.6164096001258));
#29330=CARTESIAN_POINT('Ctrl Pts',(55.0607383076031,19.0015247788187,19.6260344543267));
#29331=CARTESIAN_POINT('Ctrl Pts',(55.2225932696649,19.0175327654814,19.6369451841208));
#29332=CARTESIAN_POINT('Ctrl Pts',(55.2488045419604,19.020651480542,19.6386954191261));
#29333=CARTESIAN_POINT('Ctrl Pts',(55.2826620000217,19.025363218265,19.6409280968758));
#29334=CARTESIAN_POINT('Ctrl Pts',(55.2903701386604,19.0264819703274,19.6414345004279));
#29335=CARTESIAN_POINT('Ctrl Pts',(55.3026778258275,19.0283419674287,19.642239834126));
#29336=CARTESIAN_POINT('Ctrl Pts',(55.307281577987,19.0290542126776,19.6425403456731));
#29337=CARTESIAN_POINT('Ctrl Pts',(55.316067037083,19.0304449394086,19.6431123749036));
#29338=CARTESIAN_POINT('Ctrl Pts',(55.3202490940301,19.0311206165215,19.6433840395558));
#29339=CARTESIAN_POINT('Ctrl Pts',(55.3301076813416,19.0327456685199,19.6440230075638));
#29340=CARTESIAN_POINT('Ctrl Pts',(55.3357823608304,19.0337063052159,19.6443896775027));
#29341=CARTESIAN_POINT('Ctrl Pts',(55.354509903229,19.0369600302397,19.6455962784053));
#29342=CARTESIAN_POINT('Ctrl Pts',(55.3675444013262,19.0393586942867,19.6464304885923));
#29343=CARTESIAN_POINT('Ctrl Pts',(55.4386234464613,19.0531727326352,19.6509537413615));
#29344=CARTESIAN_POINT('Ctrl Pts',(55.4961675879103,19.0670369808496,19.6545216768063));
#29345=CARTESIAN_POINT('Ctrl Pts',(55.6907079419305,19.1231708011607,19.6665196744245));
#29346=CARTESIAN_POINT('Ctrl Pts',(55.8237199279675,19.1776241095011,19.6746406379077));
#29347=CARTESIAN_POINT('Ctrl Pts',(56.0186852213769,19.2831853301941,19.6877531701362));
#29348=CARTESIAN_POINT('Ctrl Pts',(56.0853503538962,19.324534492639,19.6924771274866));
#29349=CARTESIAN_POINT('Ctrl Pts',(56.1613242034307,19.3780979286924,19.6982541700892));
#29350=CARTESIAN_POINT('Ctrl Pts',(56.1731503187056,19.3866313048789,19.6991652478416));
#29351=CARTESIAN_POINT('Ctrl Pts',(56.1924076933736,19.4008505449274,19.7006689605137));
#29352=CARTESIAN_POINT('Ctrl Pts',(56.1998945291834,19.4064604802815,19.701258658233));
#29353=CARTESIAN_POINT('Ctrl Pts',(56.2132909750004,19.4166464602075,19.7023231684609));
#29354=CARTESIAN_POINT('Ctrl Pts',(56.2192148883148,19.4212034723824,19.7027972282011));
#29355=CARTESIAN_POINT('Ctrl Pts',(56.2317941480738,19.4309931763722,19.7038110962697));
#29356=CARTESIAN_POINT('Ctrl Pts',(56.2384420535122,19.4362351480266,19.7043512671971));
#29357=CARTESIAN_POINT('Ctrl Pts',(56.256325265804,19.4505218857369,19.7058163277697));
#29358=CARTESIAN_POINT('Ctrl Pts',(56.267495997736,19.4596463140994,19.7067443988404));
#29359=CARTESIAN_POINT('Ctrl Pts',(56.3250977554175,19.5077471845461,19.7115987559919));
#29360=CARTESIAN_POINT('Ctrl Pts',(56.3698288833484,19.5487005617066,19.7156054870268));
#29361=CARTESIAN_POINT('Ctrl Pts',(56.4625974085047,19.641748762918,19.7244542463367));
#29362=CARTESIAN_POINT('Ctrl Pts',(56.5098648005875,19.6944945810795,19.7293180844682));
#29363=CARTESIAN_POINT('Ctrl Pts',(56.6411803330977,19.8577223324104,19.7438601814206));
#29364=CARTESIAN_POINT('Ctrl Pts',(56.7166253647752,19.9745869600304,19.7536621172669));
#29365=CARTESIAN_POINT('Ctrl Pts',(56.7899214054424,20.1192290840442,19.764504966925));
#29366=CARTESIAN_POINT('Ctrl Pts',(56.8001393510069,20.1403055911879,19.7660544001512));
#29367=CARTESIAN_POINT('Ctrl Pts',(56.8131133997085,20.1683132894064,19.7680688623158));
#29368=CARTESIAN_POINT('Ctrl Pts',(56.8162047712208,20.1750859329538,19.7685526011871));
#29369=CARTESIAN_POINT('Ctrl Pts',(56.8211374434818,20.1860546894093,19.769330406236));
#29370=CARTESIAN_POINT('Ctrl Pts',(56.8230022942124,20.19024003988,19.7696258736925));
#29371=CARTESIAN_POINT('Ctrl Pts',(56.8265756783595,20.1983348232381,19.7701947325401));
#29372=CARTESIAN_POINT('Ctrl Pts',(56.8282861015554,20.2022433356164,19.7704682319084));
#29373=CARTESIAN_POINT('Ctrl Pts',(56.8323473828459,20.2116054927032,19.7711206168165));
#29374=CARTESIAN_POINT('Ctrl Pts',(56.8346864747123,20.2170642604663,19.7714987912119));
#29375=CARTESIAN_POINT('Ctrl Pts',(56.8425846236466,20.2357260401746,19.7727843913507));
#29376=CARTESIAN_POINT('Ctrl Pts',(56.8480259710898,20.2489788158847,19.7736850170145));
#29377=CARTESIAN_POINT('Ctrl Pts',(56.8788412980894,20.3263950835175,19.7788809541708));
#29378=CARTESIAN_POINT('Ctrl Pts',(56.9010179035226,20.3917885517414,19.7830122320168));
#29379=CARTESIAN_POINT('Ctrl Pts',(56.9741705522803,20.6509936759879,19.7988689494135));
#29380=CARTESIAN_POINT('Ctrl Pts',(56.9992281490352,20.8508609233056,19.810123257884));
#29381=CARTESIAN_POINT('Ctrl Pts',(56.9935140332236,21.073779096414,19.8238797470968));
#29382=CARTESIAN_POINT('Ctrl Pts',(56.9925467620333,21.096430760457,19.8252895498713));
#29383=CARTESIAN_POINT('Ctrl Pts',(56.9906500318475,21.1281521353835,19.8272825816398));
#29384=CARTESIAN_POINT('Ctrl Pts',(56.9900441448628,21.1372399948239,19.8278557222121));
#29385=CARTESIAN_POINT('Ctrl Pts',(56.988817645199,21.1539151901534,19.8289114713054));
#29386=CARTESIAN_POINT('Ctrl Pts',(56.9882157936343,21.1615037675762,19.8293934846216));
#29387=CARTESIAN_POINT('Ctrl Pts',(56.9869047567751,21.1769144917045,19.8303756008559));
#29388=CARTESIAN_POINT('Ctrl Pts',(56.9861927804803,21.1847362599377,19.8308757831142));
#29389=CARTESIAN_POINT('Ctrl Pts',(56.9843137250247,21.2041113491262,19.8321190959192));
#29390=CARTESIAN_POINT('Ctrl Pts',(56.9830919314014,21.2156589537308,19.8328639314231));
#29391=CARTESIAN_POINT('Ctrl Pts',(56.9781005907492,21.2591972566589,19.835687021727));
#29392=CARTESIAN_POINT('Ctrl Pts',(56.9736573347616,21.2911042584922,19.8377862612634));
#29393=CARTESIAN_POINT('Ctrl Pts',(56.9605518089326,21.3710002985612,19.8431223992178));
#29394=CARTESIAN_POINT('Ctrl Pts',(56.9508992139678,21.4188033403561,19.8463882742498));
#29395=CARTESIAN_POINT('Ctrl Pts',(56.9156101561332,21.5656138861686,19.8566399746164));
#29396=CARTESIAN_POINT('Ctrl Pts',(56.8841081750391,21.6630343102633,19.8637692015355));
#29397=CARTESIAN_POINT('Ctrl Pts',(56.8064411892692,21.8522068062502,19.8780297204591));
#29398=CARTESIAN_POINT('Ctrl Pts',(56.7603782294296,21.9436943121763,19.8851386057246));
#29399=CARTESIAN_POINT('Ctrl Pts',(56.6992634622289,22.0448851041563,19.8929700113413));
#29400=CARTESIAN_POINT('Ctrl Pts',(56.690866785817,22.0584189841168,19.8940165535413));
#29401=CARTESIAN_POINT('Ctrl Pts',(56.6788807662267,22.0772314658685,19.8954684742823));
#29402=CARTESIAN_POINT('Ctrl Pts',(56.6754270788242,22.0825951988191,19.8958821157221));
#29403=CARTESIAN_POINT('Ctrl Pts',(56.6698110200541,22.0912259468111,19.8965470609926));
#29404=CARTESIAN_POINT('Ctrl Pts',(56.6676646866509,22.0945032678046,19.8967994075373));
#29405=CARTESIAN_POINT('Ctrl Pts',(56.6631150393526,22.1014058499247,19.8973305368456));
#29406=CARTESIAN_POINT('Ctrl Pts',(56.6607094990114,22.1050296108641,19.8976091625521));
#29407=CARTESIAN_POINT('Ctrl Pts',(56.6547491547136,22.1139449871829,19.8982942096986));
#29408=CARTESIAN_POINT('Ctrl Pts',(56.6511807632165,22.1192275413642,19.8986997283771));
#29409=CARTESIAN_POINT('Ctrl Pts',(56.6379319843243,22.1386394157245,19.9001888235182));
#29410=CARTESIAN_POINT('Ctrl Pts',(56.6280947391582,22.152661472925,19.9012623618939));
#29411=CARTESIAN_POINT('Ctrl Pts',(56.559770566702,22.2474309105063,19.9085164198208));
#29412=CARTESIAN_POINT('Ctrl Pts',(56.4954742589598,22.3238314791382,19.9143606224698));
#29413=CARTESIAN_POINT('Ctrl Pts',(56.3103674702416,22.5130004445966,19.9297520586874));
#29414=CARTESIAN_POINT('Ctrl Pts',(56.1808476884012,22.6161144661068,19.939213404145));
#29415=CARTESIAN_POINT('Ctrl Pts',(56.0203583561287,22.7141857284793,19.9508104067281));
#29416=CARTESIAN_POINT('Ctrl Pts',(56.0003890583831,22.7259158580431,19.9522500019627));
#29417=CARTESIAN_POINT('Ctrl Pts',(55.9722204093258,22.7418092370725,19.9542781309132));
#29418=CARTESIAN_POINT('Ctrl Pts',(55.9641891513502,22.7462677969175,19.9548560877129));
#29419=CARTESIAN_POINT('Ctrl Pts',(55.9494291120574,22.7543289814693,19.9559178857759));
#29420=CARTESIAN_POINT('Ctrl Pts',(55.9427098694798,22.7579487800826,19.956401105518));
#29421=CARTESIAN_POINT('Ctrl Pts',(55.9290570262866,22.7652030725092,19.957382749616));
#29422=CARTESIAN_POINT('Ctrl Pts',(55.9221224782036,22.7688354863034,19.9578812367055));
#29423=CARTESIAN_POINT('Ctrl Pts',(55.904959673297,22.7776972503598,19.9591148034006));
#29424=CARTESIAN_POINT('Ctrl Pts',(55.8947073837488,22.7828791917985,19.9598515301343));
#29425=CARTESIAN_POINT('Ctrl Pts',(55.8563444936526,22.8018551943899,19.9626080957199));
#29426=CARTESIAN_POINT('Ctrl Pts',(55.8279563185152,22.8150747046868,19.9646476619746));
#29427=CARTESIAN_POINT('Ctrl Pts',(55.7562817474945,22.8464200269799,19.969799423453));
#29428=CARTESIAN_POINT('Ctrl Pts',(55.7126465679376,22.8636961382306,19.9729381041316));
#29429=CARTESIAN_POINT('Ctrl Pts',(55.5058007313037,22.9372642745294,19.9878199946336));
#29430=CARTESIAN_POINT('Ctrl Pts',(55.336389978457,22.9737364497894,20.000100773204));
#29431=CARTESIAN_POINT('Ctrl Pts',(55.1644483497948,22.9879598342899,20.0118645378774));
#29432=CARTESIAN_POINT('Origin',(55.,21.,6.22095488139522));
#29433=CARTESIAN_POINT('',(55.164448351653,22.9879598341362,20.9703924394033));
#29434=CARTESIAN_POINT('',(55.1644479523467,22.9879598671676,20.810886410834));
#29435=CARTESIAN_POINT('',(55.1644483516311,22.987959834138,6.22095488139522));
#29436=CARTESIAN_POINT('Ctrl Pts',(55.164448351653,22.9879598341362,20.9703924394033));
#29437=CARTESIAN_POINT('Ctrl Pts',(55.1674230284317,22.9877137624175,20.9702048747357));
#29438=CARTESIAN_POINT('Ctrl Pts',(55.1703971503059,22.9874610141927,20.9700171029999));
#29439=CARTESIAN_POINT('Ctrl Pts',(55.1816941270429,22.986475424851,20.9693029362251));
#29440=CARTESIAN_POINT('Ctrl Pts',(55.1900128099936,22.9856969803913,20.9687751308099));
#29441=CARTESIAN_POINT('Ctrl Pts',(55.2057839210713,22.9841211435724,20.9677707359783));
#29442=CARTESIAN_POINT('Ctrl Pts',(55.2132372426693,22.9833339633978,20.9672944756293));
#29443=CARTESIAN_POINT('Ctrl Pts',(55.2301702614005,22.9814490358388,20.9662087748862));
#29444=CARTESIAN_POINT('Ctrl Pts',(55.2396468165603,22.980325233122,20.9655985246649));
#29445=CARTESIAN_POINT('Ctrl Pts',(55.2641928228773,22.9772356114773,20.9640108576897));
#29446=CARTESIAN_POINT('Ctrl Pts',(55.2792482977141,22.9751655317869,20.9630301853784));
#29447=CARTESIAN_POINT('Ctrl Pts',(55.3896647822656,22.9586959759476,20.9557860260432));
#29448=CARTESIAN_POINT('Ctrl Pts',(55.4838793385295,22.9375717834717,20.9493101660023));
#29449=CARTESIAN_POINT('Ctrl Pts',(55.7110793384366,22.8690228625102,20.9330034180314));
#29450=CARTESIAN_POINT('Ctrl Pts',(55.8412732870271,22.8141491572639,20.9230297150245));
#29451=CARTESIAN_POINT('Ctrl Pts',(56.0074579539029,22.7223396428782,20.910059195898));
#29452=CARTESIAN_POINT('Ctrl Pts',(56.0494372138678,22.6970880352632,20.9067641324717));
#29453=CARTESIAN_POINT('Ctrl Pts',(56.098019053344,22.6653718720301,20.9029648095425));
#29454=CARTESIAN_POINT('Ctrl Pts',(56.1055565950768,22.660377648669,20.9023757618624));
#29455=CARTESIAN_POINT('Ctrl Pts',(56.1171545444495,22.6525790845585,20.9014703756665));
#29456=CARTESIAN_POINT('Ctrl Pts',(56.1212388260881,22.6498107173418,20.9011517279255));
#29457=CARTESIAN_POINT('Ctrl Pts',(56.1287678509004,22.6446665956117,20.9005647409862));
#29458=CARTESIAN_POINT('Ctrl Pts',(56.1322153697563,22.6422951710914,20.9002961294141));
#29459=CARTESIAN_POINT('Ctrl Pts',(56.1400095241046,22.6368976438306,20.8996892110244));
#29460=CARTESIAN_POINT('Ctrl Pts',(56.144351579208,22.633865072811,20.8993513487972));
#29461=CARTESIAN_POINT('Ctrl Pts',(56.1572175527002,22.6248027912319,20.8983507955241));
#29462=CARTESIAN_POINT('Ctrl Pts',(56.1657064220464,22.6187233004501,20.8976913840031));
#29463=CARTESIAN_POINT('Ctrl Pts',(56.2464132023215,22.559959199221,20.8914251855198));
#29464=CARTESIAN_POINT('Ctrl Pts',(56.3150703335734,22.5025354666116,20.8861161382822));
#29465=CARTESIAN_POINT('Ctrl Pts',(56.4665497277803,22.3574741599096,20.8738493725367));
#29466=CARTESIAN_POINT('Ctrl Pts',(56.5457399134418,22.2665671157769,20.8669703483775));
#29467=CARTESIAN_POINT('Ctrl Pts',(56.6459214280707,22.1280657288151,20.85684456982));
#29468=CARTESIAN_POINT('Ctrl Pts',(56.6740132769748,22.0859413573564,20.8538086046394));
#29469=CARTESIAN_POINT('Ctrl Pts',(56.7120818784239,22.0238634975641,20.8493609680054));
#29470=CARTESIAN_POINT('Ctrl Pts',(56.7233749312408,22.004738577009,20.8479942972763));
#29471=CARTESIAN_POINT('Ctrl Pts',(56.7430277870541,21.9701497536569,20.8455261127801));
#29472=CARTESIAN_POINT('Ctrl Pts',(56.7515070562206,21.954756205564,20.8444288937728));
#29473=CARTESIAN_POINT('Ctrl Pts',(56.7640854927739,21.9311892845362,20.8427500044087));
#29474=CARTESIAN_POINT('Ctrl Pts',(56.768333830923,21.9230961853327,20.8421736211191));
#29475=CARTESIAN_POINT('Ctrl Pts',(56.7756187688728,21.9089834996872,20.8411686811578));
#29476=CARTESIAN_POINT('Ctrl Pts',(56.7786807745463,21.9029771400828,20.8407410265619));
#29477=CARTESIAN_POINT('Ctrl Pts',(56.7854781175839,21.8894748980991,20.8397797104226));
#29478=CARTESIAN_POINT('Ctrl Pts',(56.7891967967909,21.8819708167198,20.839245476425));
#29479=CARTESIAN_POINT('Ctrl Pts',(56.7990062384634,21.8618585601611,20.8378136015503));
#29480=CARTESIAN_POINT('Ctrl Pts',(56.80501159718,21.8492094801694,20.836913023009));
#29481=CARTESIAN_POINT('Ctrl Pts',(56.8312572660477,21.7923918759971,20.8328668456321));
#29482=CARTESIAN_POINT('Ctrl Pts',(56.8500115510239,21.747559124156,20.8296710939062));
#29483=CARTESIAN_POINT('Ctrl Pts',(56.876626825179,21.6767795062985,20.8246176764712));
#29484=CARTESIAN_POINT('Ctrl Pts',(56.8856281868899,21.6512794933545,20.8227956035008));
#29485=CARTESIAN_POINT('Ctrl Pts',(56.9494568421169,21.4580292435766,20.8089809449915));
#29486=CARTESIAN_POINT('Ctrl Pts',(56.9823164063856,21.2838734544756,20.7964017044736));
#29487=CARTESIAN_POINT('Ctrl Pts',(56.9932913339742,21.0808613355804,20.7825988310038));
#29488=CARTESIAN_POINT('Ctrl Pts',(56.9941994478126,21.0540148703273,20.7807926985989));
#29489=CARTESIAN_POINT('Ctrl Pts',(56.9948046623135,21.009564387303,20.7778423363127));
#29490=CARTESIAN_POINT('Ctrl Pts',(56.9948114365766,20.9919686815038,20.7766848374015));
#29491=CARTESIAN_POINT('Ctrl Pts',(56.9945026232366,20.9679319188483,20.7751198893588));
#29492=CARTESIAN_POINT('Ctrl Pts',(56.9943886368266,20.9614896896558,20.7747020555433));
#29493=CARTESIAN_POINT('Ctrl Pts',(56.9941450829581,20.9506846997236,20.7740040644679));
#29494=CARTESIAN_POINT('Ctrl Pts',(56.9940324086913,20.9463216532779,20.7737229836803));
#29495=CARTESIAN_POINT('Ctrl Pts',(56.9937917295154,20.9380535137136,20.7731918239267));
#29496=CARTESIAN_POINT('Ctrl Pts',(56.9936665700738,20.9341483799728,20.7729415838163));
#29497=CARTESIAN_POINT('Ctrl Pts',(56.9933090045446,20.9239297108976,20.7722883704098));
#29498=CARTESIAN_POINT('Ctrl Pts',(56.9930580745282,20.9176168060753,20.771886422586));
#29499=CARTESIAN_POINT('Ctrl Pts',(56.9920856822456,20.8957693146422,20.7705005692399));
#29500=CARTESIAN_POINT('Ctrl Pts',(56.9912125346022,20.8802415833859,20.7695246907944));
#29501=CARTESIAN_POINT('Ctrl Pts',(56.9816277673975,20.7392309537141,20.7607323535998));
#29502=CARTESIAN_POINT('Ctrl Pts',(56.9612455081957,20.6148064370411,20.7534658079392));
#29503=CARTESIAN_POINT('Ctrl Pts',(56.8912471377406,20.3483818893744,20.7374846252002));
#29504=CARTESIAN_POINT('Ctrl Pts',(56.8370611430115,20.2084063475262,20.728781679857));
#29505=CARTESIAN_POINT('Ctrl Pts',(56.7597290742827,20.0604894283604,20.7184225061462));
#29506=CARTESIAN_POINT('Ctrl Pts',(56.7515194567132,20.0452717180328,20.7173427181159));
#29507=CARTESIAN_POINT('Ctrl Pts',(56.738697742356,20.0222269171076,20.7156850963962));
#29508=CARTESIAN_POINT('Ctrl Pts',(56.7342281513733,20.0143211702162,20.7151123437113));
#29509=CARTESIAN_POINT('Ctrl Pts',(56.7259905209259,19.9999800538894,20.7140657564104));
#29510=CARTESIAN_POINT('Ctrl Pts',(56.7222400641669,19.9935347348997,20.7135925619177));
#29511=CARTESIAN_POINT('Ctrl Pts',(56.7140499061264,19.9796394295651,20.7125662011117));
#29512=CARTESIAN_POINT('Ctrl Pts',(56.709597597621,19.9721970886018,20.7120125833335));
#29513=CARTESIAN_POINT('Ctrl Pts',(56.6973344622424,19.9519985627831,20.7104992690216));
#29514=CARTESIAN_POINT('Ctrl Pts',(56.689428587873,19.9393010250909,20.7095361082156));
#29515=CARTESIAN_POINT('Ctrl Pts',(56.6481878988791,19.8746956875284,20.7045734428999));
#29516=CARTESIAN_POINT('Ctrl Pts',(56.6126040650623,19.8242704762318,20.7004909205695));
#29517=CARTESIAN_POINT('Ctrl Pts',(56.4676178674006,19.6378017786085,20.6845618592019));
#29518=CARTESIAN_POINT('Ctrl Pts',(56.3428742196192,19.5146847552323,20.6721602944548));
#29519=CARTESIAN_POINT('Ctrl Pts',(56.1615462750977,19.3774594662395,20.6565862895012));
#29520=CARTESIAN_POINT('Ctrl Pts',(56.1180939983872,19.3472161556225,20.6530171864849));
#29521=CARTESIAN_POINT('Ctrl Pts',(56.0657163263958,19.3137730697115,20.648946281753));
#29522=CARTESIAN_POINT('Ctrl Pts',(56.0579118228645,19.3088657262903,20.6483455344967));
#29523=CARTESIAN_POINT('Ctrl Pts',(56.0458461140064,19.3013952229324,20.647426065082));
#29524=CARTESIAN_POINT('Ctrl Pts',(56.0416090018581,19.2987936717097,20.6471049214531));
#29525=CARTESIAN_POINT('Ctrl Pts',(56.0337904688587,19.2940333195063,20.6465156027183));
#29526=CARTESIAN_POINT('Ctrl Pts',(56.0302120031055,19.2918699470695,20.6462471381438));
#29527=CARTESIAN_POINT('Ctrl Pts',(56.022126734077,19.2870166236971,20.645643381968));
#29528=CARTESIAN_POINT('Ctrl Pts',(56.0176161102669,19.284333202032,20.6453085148042));
#29529=CARTESIAN_POINT('Ctrl Pts',(56.0042936433659,19.2764785384598,20.6443250532595));
#29530=CARTESIAN_POINT('Ctrl Pts',(55.9954524427132,19.2713570654234,20.6436795746621));
#29531=CARTESIAN_POINT('Ctrl Pts',(55.9255935344047,19.2316033645784,20.6386323612639));
#29532=CARTESIAN_POINT('Ctrl Pts',(55.8628193852695,19.2001402744882,20.6344129152759));
#29533=CARTESIAN_POINT('Ctrl Pts',(55.6433143105828,19.1042530800487,20.620274017616));
#29534=CARTESIAN_POINT('Ctrl Pts',(55.4801207465749,19.0564989924778,20.6107261049396));
#29535=CARTESIAN_POINT('Ctrl Pts',(55.2629546702188,19.0220124120218,20.5974824352307));
#29536=CARTESIAN_POINT('Ctrl Pts',(55.2127782967319,19.0159877021967,20.5943922231503));
#29537=CARTESIAN_POINT('Ctrl Pts',(55.1488478241707,19.0107645681261,20.5903922177872));
#29538=CARTESIAN_POINT('Ctrl Pts',(55.1352545862278,19.0097941160572,20.5895381798738));
#29539=CARTESIAN_POINT('Ctrl Pts',(55.1133756637403,19.0084573097662,20.5881574452446));
#29540=CARTESIAN_POINT('Ctrl Pts',(55.1050956238109,19.0080032041589,20.5876335009309));
#29541=CARTESIAN_POINT('Ctrl Pts',(55.0893137710545,19.0072363448163,20.5866320739116));
#29542=CARTESIAN_POINT('Ctrl Pts',(55.0818125368117,19.0069142915034,20.5861548910852));
#29543=CARTESIAN_POINT('Ctrl Pts',(55.0646597454618,19.0062748605324,20.5850609188074));
#29544=CARTESIAN_POINT('Ctrl Pts',(55.0550074029834,19.0059852070202,20.5844432730887));
#29545=CARTESIAN_POINT('Ctrl Pts',(55.0297816716614,19.0054115158649,20.5828236068537));
#29546=CARTESIAN_POINT('Ctrl Pts',(55.0142066330443,19.005239784399,20.5818181104334));
#29547=CARTESIAN_POINT('Ctrl Pts',(54.8755670251517,19.0053348955324,20.5728172585312));
#29548=CARTESIAN_POINT('Ctrl Pts',(54.7527968477784,19.0168073208097,20.5644671001361));
#29549=CARTESIAN_POINT('Ctrl Pts',(54.5174745044657,19.0609930284037,20.5478608836285));
#29550=CARTESIAN_POINT('Ctrl Pts',(54.4051636237486,19.0924493833604,20.5396599905331));
#29551=CARTESIAN_POINT('Ctrl Pts',(54.2528736897793,19.1498709640958,20.528560729112));
#29552=CARTESIAN_POINT('Ctrl Pts',(54.2100902752486,19.1677285765733,20.5254473195951));
#29553=CARTESIAN_POINT('Ctrl Pts',(54.1598644909494,19.19077936269,20.5218293675881));
#29554=CARTESIAN_POINT('Ctrl Pts',(54.1517895058775,19.1945510384253,20.521248871853));
#29555=CARTESIAN_POINT('Ctrl Pts',(54.139308794379,19.2004827645161,20.5203537929136));
#29556=CARTESIAN_POINT('Ctrl Pts',(54.1348854247366,19.2026051059486,20.5200369810864));
#29557=CARTESIAN_POINT('Ctrl Pts',(54.1267015664905,19.2065689475409,20.5194516742339));
#29558=CARTESIAN_POINT('Ctrl Pts',(54.1229390723983,19.2084059545516,20.5191829195049));
#29559=CARTESIAN_POINT('Ctrl Pts',(54.1143971941174,19.2126098143923,20.5185735171007));
#29560=CARTESIAN_POINT('Ctrl Pts',(54.1096215063393,19.2149839930656,20.5182333296135));
#29561=CARTESIAN_POINT('Ctrl Pts',(54.0972266198962,19.2212080901248,20.5173516188828));
#29562=CARTESIAN_POINT('Ctrl Pts',(54.0896224169046,19.2250878622303,20.5168118944855));
#29563=CARTESIAN_POINT('Ctrl Pts',(54.039336206552,19.2511527954617,20.513249162095));
#29564=CARTESIAN_POINT('Ctrl Pts',(53.9974399770341,19.2748287901999,20.5103116558492));
#29565=CARTESIAN_POINT('Ctrl Pts',(53.941344621708,19.3092634803323,20.5063649352237));
#29566=CARTESIAN_POINT('Ctrl Pts',(53.926375630425,19.3187290731782,20.5053103886359));
#29567=CARTESIAN_POINT('Ctrl Pts',(53.7656887926224,19.4233601835461,20.4939536770142));
#29568=CARTESIAN_POINT('Ctrl Pts',(53.6329003794888,19.5370031223853,20.4841682600082));
#29569=CARTESIAN_POINT('Ctrl Pts',(53.4821303526843,19.704720603262,20.4705945041983));
#29570=CARTESIAN_POINT('Ctrl Pts',(53.4492162693372,19.7443144851912,20.4674477287167));
#29571=CARTESIAN_POINT('Ctrl Pts',(53.4095218062548,19.79600886326,20.4633837887107));
#29572=CARTESIAN_POINT('Ctrl Pts',(53.4012841473777,19.806968923359,20.4625246370339));
#29573=CARTESIAN_POINT('Ctrl Pts',(53.3882357586937,19.8247074145035,20.4611376165708));
#29574=CARTESIAN_POINT('Ctrl Pts',(53.3833531787427,19.8314326365131,20.4606125460986));
#29575=CARTESIAN_POINT('Ctrl Pts',(53.374142225133,19.8442879386755,20.4596102698405));
#29576=CARTESIAN_POINT('Ctrl Pts',(53.3698061285429,19.850412329691,20.4591333725194));
#29577=CARTESIAN_POINT('Ctrl Pts',(53.3599888609184,19.8644456773597,20.4580418926502));
#29578=CARTESIAN_POINT('Ctrl Pts',(53.3545301886841,19.8723700737114,20.4574264677949));
#29579=CARTESIAN_POINT('Ctrl Pts',(53.340450359488,19.8931298093583,20.4558164317961));
#29580=CARTESIAN_POINT('Ctrl Pts',(53.3319208587762,19.9060262413924,20.4548184117751));
#29581=CARTESIAN_POINT('Ctrl Pts',(53.2525376226562,20.029139215747,20.4453095200631));
#29582=CARTESIAN_POINT('Ctrl Pts',(53.1925686254404,20.1459651661725,20.4363929075652));
#29583=CARTESIAN_POINT('Ctrl Pts',(53.1040966006011,20.3701682368526,20.4196446705431));
#29584=CARTESIAN_POINT('Ctrl Pts',(53.0722422031285,20.4757015867278,20.4119042718392));
#29585=CARTESIAN_POINT('Ctrl Pts',(53.0398376707431,20.6274100019294,20.4013343876645));
#29586=CARTESIAN_POINT('Ctrl Pts',(53.0319175842728,20.6718049617459,20.3983082367895));
#29587=CARTESIAN_POINT('Ctrl Pts',(53.0242506916948,20.725190089852,20.3947778141092));
#29588=CARTESIAN_POINT('Ctrl Pts',(53.0230513959082,20.7339548163091,20.3942016750867));
#29589=CARTESIAN_POINT('Ctrl Pts',(53.0212794990037,20.7475783857891,20.3933118511797));
#29590=CARTESIAN_POINT('Ctrl Pts',(53.0206664157599,20.75243171461,20.3929959782657));
#29591=CARTESIAN_POINT('Ctrl Pts',(53.0195615352845,20.7614447773959,20.3924115183356));
#29592=CARTESIAN_POINT('Ctrl Pts',(53.0190649894414,20.7656037730739,20.3921426781295));
#29593=CARTESIAN_POINT('Ctrl Pts',(53.0179637055182,20.7750814756494,20.3915319499965));
#29594=CARTESIAN_POINT('Ctrl Pts',(53.0173672742555,20.7804010663618,20.391190530508));
#29595=CARTESIAN_POINT('Ctrl Pts',(53.0158682594814,20.7942749709469,20.3903034921914));
#29596=CARTESIAN_POINT('Ctrl Pts',(53.014999569509,20.8028329425468,20.3897597081598));
#29597=CARTESIAN_POINT('Ctrl Pts',(53.0095102181503,20.8606305249053,20.3861083325675));
#29598=CARTESIAN_POINT('Ctrl Pts',(53.0066663550327,20.9100261099869,20.3830911672217));
#29599=CARTESIAN_POINT('Ctrl Pts',(53.0053965898443,20.9725231609778,20.3793472544449));
#29600=CARTESIAN_POINT('Ctrl Pts',(53.0052595471134,20.9855681999382,20.3785698364135));
#29601=CARTESIAN_POINT('Ctrl Pts',(53.0051605434955,21.1280385974422,20.370114841767));
#29602=CARTESIAN_POINT('Ctrl Pts',(53.0176666334288,21.2571685736435,20.3627516861738));
#29603=CARTESIAN_POINT('Ctrl Pts',(53.0606284182064,21.4760589360895,20.3496536461333));
#29604=CARTESIAN_POINT('Ctrl Pts',(53.0851053900687,21.5665417532498,20.3440526453093));
#29605=CARTESIAN_POINT('Ctrl Pts',(53.1208059723588,21.6692427601496,20.3373003989082));
#29606=CARTESIAN_POINT('Ctrl Pts',(53.1259313573745,21.6834638019527,20.3363565432676));
#29607=CARTESIAN_POINT('Ctrl Pts',(53.1345467272863,21.7065424647017,20.3348096461472));
#29608=CARTESIAN_POINT('Ctrl Pts',(53.1379394274192,21.7154359412877,20.3342098391779));
#29609=CARTESIAN_POINT('Ctrl Pts',(53.1441160321685,21.7312854383,20.3331341078978));
#29610=CARTESIAN_POINT('Ctrl Pts',(53.1468757374519,21.7382507428896,20.3326590023201));
#29611=CARTESIAN_POINT('Ctrl Pts',(53.1528011265525,21.752963429734,20.331650362858));
#29612=CARTESIAN_POINT('Ctrl Pts',(53.1559764523568,21.7607067482283,20.3311165110364));
#29613=CARTESIAN_POINT('Ctrl Pts',(53.1645841243105,21.7813267191913,20.3296867401662));
#29614=CARTESIAN_POINT('Ctrl Pts',(53.1701031472025,21.7941664627037,20.3287878985512));
#29615=CARTESIAN_POINT('Ctrl Pts',(53.1978660935373,21.8569294210491,20.3243512290707));
#29616=CARTESIAN_POINT('Ctrl Pts',(53.2220185390199,21.9059777127488,20.320748646002));
#29617=CARTESIAN_POINT('Ctrl Pts',(53.3456460786204,22.1330046286085,20.3034093914893));
#29618=CARTESIAN_POINT('Ctrl Pts',(53.4699834378642,22.2959986858709,20.2888023758561));
#29619=CARTESIAN_POINT('Ctrl Pts',(53.6414155634742,22.4609721945682,20.2727232123482));
#29620=CARTESIAN_POINT('Ctrl Pts',(53.6666020427726,22.4839951629618,20.270447895774));
#29621=CARTESIAN_POINT('Ctrl Pts',(53.6987390984976,22.5118924555845,20.2676639237699));
#29622=CARTESIAN_POINT('Ctrl Pts',(53.7051449215525,22.5173823061244,20.2671147168241));
#29623=CARTESIAN_POINT('Ctrl Pts',(53.7152897943443,22.5259655284435,20.2662541627227));
#29624=CARTESIAN_POINT('Ctrl Pts',(53.7190055438801,22.5290861032402,20.2659408950456));
#29625=CARTESIAN_POINT('Ctrl Pts',(53.7259231839884,22.5348527885235,20.265361306799));
#29626=CARTESIAN_POINT('Ctrl Pts',(53.7291219247398,22.537502433754,20.2650947367863));
#29627=CARTESIAN_POINT('Ctrl Pts',(53.7364890013257,22.5435661787747,20.2644840499161));
#29628=CARTESIAN_POINT('Ctrl Pts',(53.7406629059793,22.5469733925608,20.264140429536));
#29629=CARTESIAN_POINT('Ctrl Pts',(53.7536007086018,22.5574476283076,20.2630824341896));
#29630=CARTESIAN_POINT('Ctrl Pts',(53.7624108484027,22.5644575463269,20.2623720098396));
#29631=CARTESIAN_POINT('Ctrl Pts',(53.8467941030825,22.6304393881571,20.2556572531532));
#29632=CARTESIAN_POINT('Ctrl Pts',(53.9264770258553,22.6839744214656,20.2499922583744));
#29633=CARTESIAN_POINT('Ctrl Pts',(54.1552643952985,22.814817960271,20.2346174489977));
#29634=CARTESIAN_POINT('Ctrl Pts',(54.3107173179637,22.8793690659443,20.2250608349423));
#29635=CARTESIAN_POINT('Ctrl Pts',(54.5007371812649,22.9314830994437,20.2129921582343));
#29636=CARTESIAN_POINT('Ctrl Pts',(54.5292309243637,22.9386249416802,20.2111749281898));
#29637=CARTESIAN_POINT('Ctrl Pts',(54.5691380299008,22.9476958266206,20.2086147682938));
#29638=CARTESIAN_POINT('Ctrl Pts',(54.5804270376897,22.9501588629238,20.2078888948675));
#29639=CARTESIAN_POINT('Ctrl Pts',(54.5986468384981,22.9539685363602,20.2067144664454));
#29640=CARTESIAN_POINT('Ctrl Pts',(54.6055646051,22.9553767203535,20.2062678818821));
#29641=CARTESIAN_POINT('Ctrl Pts',(54.619947656748,22.9582251102734,20.2053379041096));
#29642=CARTESIAN_POINT('Ctrl Pts',(54.6274139807704,22.9596594147358,20.2048543311882));
#29643=CARTESIAN_POINT('Ctrl Pts',(54.6450098508634,22.9629354433468,20.2037126920569));
#29644=CARTESIAN_POINT('Ctrl Pts',(54.6551457406575,22.9647414827317,20.2030535046837));
#29645=CARTESIAN_POINT('Ctrl Pts',(54.688623608902,22.9704396199011,20.2008708831504));
#29646=CARTESIAN_POINT('Ctrl Pts',(54.7120201477154,22.9739947004307,20.1993368744682));
#29647=CARTESIAN_POINT('Ctrl Pts',(54.7676193837334,22.9814334865604,20.1956695590525));
#29648=CARTESIAN_POINT('Ctrl Pts',(54.7998636694171,22.9849495366825,20.1935253475222));
#29649=CARTESIAN_POINT('Ctrl Pts',(54.9428175769606,22.9970193138447,20.1839410375635));
#29650=CARTESIAN_POINT('Ctrl Pts',(55.053961948805,22.9970995187115,20.176268010679));
#29651=CARTESIAN_POINT('Ctrl Pts',(55.1644485224877,22.9879598200043,20.1685383772559));
#29652=CARTESIAN_POINT('',(53.0052506746727,20.9991991220829,20.2192088779402));
#29653=CARTESIAN_POINT('Ctrl Pts',(55.1644483497948,22.9879598342899,20.0118645378774));
#29654=CARTESIAN_POINT('Ctrl Pts',(55.1566329193673,22.9886063436481,20.0123992477384));
#29655=CARTESIAN_POINT('Ctrl Pts',(55.1488122479989,22.9892068830392,20.0129327173509));
#29656=CARTESIAN_POINT('Ctrl Pts',(55.1027605991908,22.9924699232624,20.0160639036847));
#29657=CARTESIAN_POINT('Ctrl Pts',(55.0644612791749,22.9940765621712,20.018627077361));
#29658=CARTESIAN_POINT('Ctrl Pts',(55.0173804434754,22.9946935019973,20.0217093294711));
#29659=CARTESIAN_POINT('Ctrl Pts',(55.0086233865615,22.994750583586,20.0222797101055));
#29660=CARTESIAN_POINT('Ctrl Pts',(54.9949413723923,22.9947496647945,20.0231660164658));
#29661=CARTESIAN_POINT('Ctrl Pts',(54.9900166520139,22.9947310969016,20.0234840517854));
#29662=CARTESIAN_POINT('Ctrl Pts',(54.9809082541158,22.9946630222509,20.0240703858775));
#29663=CARTESIAN_POINT('Ctrl Pts',(54.9767246902512,22.9946185920111,20.0243389533152));
#29664=CARTESIAN_POINT('Ctrl Pts',(54.9672370138689,22.9944879765663,20.0249463661045));
#29665=CARTESIAN_POINT('Ctrl Pts',(54.961933094064,22.9943937961616,20.0252847628645));
#29666=CARTESIAN_POINT('Ctrl Pts',(54.9457935346285,22.9940428019841,20.0263111073102));
#29667=CARTESIAN_POINT('Ctrl Pts',(54.9349593432274,22.9937188273287,20.0269954370683));
#29668=CARTESIAN_POINT('Ctrl Pts',(54.8070971436177,22.9888519617868,20.0350226279865));
#29669=CARTESIAN_POINT('Ctrl Pts',(54.6906672441414,22.9740985651303,20.0418539099103));
#29670=CARTESIAN_POINT('Ctrl Pts',(54.4243140087695,22.9161863867218,20.0576831805409));
#29671=CARTESIAN_POINT('Ctrl Pts',(54.2768356094417,22.8655325390301,20.0666402517219));
#29672=CARTESIAN_POINT('Ctrl Pts',(54.1156290181243,22.7881453356953,20.0776576226879));
#29673=CARTESIAN_POINT('Ctrl Pts',(54.0947019890323,22.777642037903,20.0791120607571));
#29674=CARTESIAN_POINT('Ctrl Pts',(54.0655689754216,22.7623722902422,20.0811733624578));
#29675=CARTESIAN_POINT('Ctrl Pts',(54.0572042040394,22.7579116904035,20.0817695097477));
#29676=CARTESIAN_POINT('Ctrl Pts',(54.0427101802509,22.7500493988139,20.0828101388912));
#29677=CARTESIAN_POINT('Ctrl Pts',(54.0365664261213,22.7466746817789,20.0832536588524));
#29678=CARTESIAN_POINT('Ctrl Pts',(54.0239002526467,22.7396300913181,20.0841731096089));
#29679=CARTESIAN_POINT('Ctrl Pts',(54.0173804528119,22.7359557581859,20.0846491947927));
#29680=CARTESIAN_POINT('Ctrl Pts',(54.0020409894496,22.7271968659256,20.0857760290131));
#29681=CARTESIAN_POINT('Ctrl Pts',(53.9932393348237,22.7220813445061,20.0864278864217));
#29682=CARTESIAN_POINT('Ctrl Pts',(53.9746754343755,22.711101045727,20.0878141544641));
#29683=CARTESIAN_POINT('Ctrl Pts',(53.9649235148682,22.705219608894,20.0885491548534));
#29684=CARTESIAN_POINT('Ctrl Pts',(53.9385593557217,22.6890097553492,20.0905549330596));
#29685=CARTESIAN_POINT('Ctrl Pts',(53.9220481689928,22.6785201816267,20.0918315373929));
#29686=CARTESIAN_POINT('Ctrl Pts',(53.799734437143,22.5982651012062,20.1014446963132));
#29687=CARTESIAN_POINT('Ctrl Pts',(53.7006584225284,22.5188121813552,20.1101443146449));
#29688=CARTESIAN_POINT('Ctrl Pts',(53.515187165902,22.3385680694808,20.1281578835595));
#29689=CARTESIAN_POINT('Ctrl Pts',(53.4299214652856,22.2374541144539,20.1374355271461));
#29690=CARTESIAN_POINT('Ctrl Pts',(53.3466356361515,22.1160852140934,20.1471776157299));
#29691=CARTESIAN_POINT('Ctrl Pts',(53.3381547518389,22.1034175681686,20.1481786198885));
#29692=CARTESIAN_POINT('Ctrl Pts',(53.3263940015529,22.0854076552707,20.1495782548254));
#29693=CARTESIAN_POINT('Ctrl Pts',(53.3229930655321,22.0801456200284,20.1499843979058));
#29694=CARTESIAN_POINT('Ctrl Pts',(53.3173082956327,22.0712583938614,20.1506655385312));
#29695=CARTESIAN_POINT('Ctrl Pts',(53.3150112661832,22.0676417406842,20.1509413970973));
#29696=CARTESIAN_POINT('Ctrl Pts',(53.3103447846438,22.0602418319038,20.1515030645192));
#29697=CARTESIAN_POINT('Ctrl Pts',(53.3079763529492,22.0564579819734,20.1517888066249));
#29698=CARTESIAN_POINT('Ctrl Pts',(53.3019737727127,22.0467961836572,20.1525148035911));
#29699=CARTESIAN_POINT('Ctrl Pts',(53.2983573946826,22.0409071840548,20.1529539059083));
#29700=CARTESIAN_POINT('Ctrl Pts',(53.2837958406155,22.0169160832294,20.1547294876088));
#29701=CARTESIAN_POINT('Ctrl Pts',(53.2731078714952,21.9986584494134,20.1560502176154));
#29702=CARTESIAN_POINT('Ctrl Pts',(53.2457293605358,21.9501349421749,20.1594900885044));
#29703=CARTESIAN_POINT('Ctrl Pts',(53.2295308993368,21.9195984587963,20.1615843445483));
#29704=CARTESIAN_POINT('Ctrl Pts',(53.1236474573046,21.7068119815938,20.1758044579148));
#29705=CARTESIAN_POINT('Ctrl Pts',(53.0614625627725,21.5122166207992,20.1870894103567));
#29706=CARTESIAN_POINT('Ctrl Pts',(53.0236449015922,21.2730703255374,20.2017943876848));
#29707=CARTESIAN_POINT('Ctrl Pts',(53.0186867722596,21.2344023426098,20.2041919383045));
#29708=CARTESIAN_POINT('Ctrl Pts',(53.0135996032508,21.1827770779012,20.2074303062342));
#29709=CARTESIAN_POINT('Ctrl Pts',(53.0124590742998,21.169926609611,20.2082394417033));
#29710=CARTESIAN_POINT('Ctrl Pts',(53.0108030558203,21.1489603783053,20.2095649259071));
#29711=CARTESIAN_POINT('Ctrl Pts',(53.0102123916873,21.1408507993118,20.2100789117005));
#29712=CARTESIAN_POINT('Ctrl Pts',(53.0091929700689,21.1255651606017,20.2110502562633));
#29713=CARTESIAN_POINT('Ctrl Pts',(53.0087533901421,21.118389934071,20.2115072678539));
#29714=CARTESIAN_POINT('Ctrl Pts',(53.0079440432529,21.1038957658281,20.212432632476));
#29715=CARTESIAN_POINT('Ctrl Pts',(53.0075758047057,21.0965768533619,20.2129010261413));
#29716=CARTESIAN_POINT('Ctrl Pts',(53.0066503942713,21.0759159418415,20.2142265338185));
#29717=CARTESIAN_POINT('Ctrl Pts',(53.0061868645549,21.0625703397498,20.2150865585809));
#29718=CARTESIAN_POINT('Ctrl Pts',(53.0054458586132,21.032549395174,20.2170301178252));
#29719=CARTESIAN_POINT('Ctrl Pts',(53.0052434517756,21.0158734438085,20.2181159179354));
#29720=CARTESIAN_POINT('Ctrl Pts',(53.0052501614646,20.9991974023945,20.2192080988249));
#29721=CARTESIAN_POINT('Ctrl Pts',(53.0052501607968,20.9991990637311,20.2192079900173));
#29722=CARTESIAN_POINT('Ctrl Pts',(53.0053403195642,20.7746566204111,20.2339141702458));
#29723=CARTESIAN_POINT('Ctrl Pts',(53.0433501436141,20.5517424599308,20.2499366245077));
#29724=CARTESIAN_POINT('Ctrl Pts',(53.1338646609569,20.2936191810681,20.2686246850473));
#29725=CARTESIAN_POINT('Ctrl Pts',(53.1518051562617,20.2479284074731,20.2719265187195));
#29726=CARTESIAN_POINT('Ctrl Pts',(53.1750281533055,20.1946509312683,20.2757324527616));
#29727=CARTESIAN_POINT('Ctrl Pts',(53.1786985269636,20.1863844178494,20.2763216833574));
#29728=CARTESIAN_POINT('Ctrl Pts',(53.1844578210452,20.1736474720491,20.2772272324041));
#29729=CARTESIAN_POINT('Ctrl Pts',(53.1865072581479,20.1691594734588,20.2775458621683));
#29730=CARTESIAN_POINT('Ctrl Pts',(53.1903250497029,20.1608804407195,20.27813274407));
#29731=CARTESIAN_POINT('Ctrl Pts',(53.1920886666457,20.1570873878118,20.2784012689636));
#29732=CARTESIAN_POINT('Ctrl Pts',(53.1961108902961,20.1485073946983,20.2790078946423));
#29733=CARTESIAN_POINT('Ctrl Pts',(53.1983766220866,20.1437238864098,20.2793455517999));
#29734=CARTESIAN_POINT('Ctrl Pts',(53.2051635369318,20.1295412615098,20.280345206341));
#29735=CARTESIAN_POINT('Ctrl Pts',(53.2097395093082,20.1201683506742,20.2810039319593));
#29736=CARTESIAN_POINT('Ctrl Pts',(53.253516195955,20.0322568472779,20.2871682187445));
#29737=CARTESIAN_POINT('Ctrl Pts',(53.297792716928,19.9563396634317,20.2923868143711));
#29738=CARTESIAN_POINT('Ctrl Pts',(53.4334088231285,19.7555351393658,20.3065677298066));
#29739=CARTESIAN_POINT('Ctrl Pts',(53.5344627596391,19.6379793421624,20.3153520336596));
#29740=CARTESIAN_POINT('Ctrl Pts',(53.67134187088,19.5118142698688,20.326586243232));
#29741=CARTESIAN_POINT('Ctrl Pts',(53.6951191596315,19.4909224586767,20.3285151054779));
#29742=CARTESIAN_POINT('Ctrl Pts',(53.7316234030019,19.4603561226493,20.3314506204188));
#29743=CARTESIAN_POINT('Ctrl Pts',(53.7439866679006,19.4502539085609,20.3324405264744));
#29744=CARTESIAN_POINT('Ctrl Pts',(53.7642286633495,19.4341151899381,20.334055215494));
#29745=CARTESIAN_POINT('Ctrl Pts',(53.7720336692597,19.4279870484575,20.3346763848127));
#29746=CARTESIAN_POINT('Ctrl Pts',(53.7871142530653,19.4163272892635,20.3358740645364));
#29747=CARTESIAN_POINT('Ctrl Pts',(53.7943827751812,19.4107869266249,20.3364502126285));
#29748=CARTESIAN_POINT('Ctrl Pts',(53.8017798890779,19.4052284987491,20.3370355133223));
#29749=CARTESIAN_POINT('Ctrl Pts',(53.8018707661501,19.4051602229645,20.3370427038622));
#29750=CARTESIAN_POINT('Ctrl Pts',(53.8020555593073,19.4050214128996,20.3370573250788));
#29751=CARTESIAN_POINT('Ctrl Pts',(53.8021494757282,19.4049508791899,20.3370647557713));
#29752=CARTESIAN_POINT('Ctrl Pts',(53.8023405620233,19.4048073947359,20.3370798742274));
#29753=CARTESIAN_POINT('Ctrl Pts',(53.8024377324258,19.4047344445057,20.3370875620209));
#29754=CARTESIAN_POINT('Ctrl Pts',(53.8026355618305,19.4045859532567,20.337103213247));
#29755=CARTESIAN_POINT('Ctrl Pts',(53.802736221174,19.4045104129923,20.3371111766935));
#29756=CARTESIAN_POINT('Ctrl Pts',(53.8029412855932,19.4043565517957,20.3371273995285));
#29757=CARTESIAN_POINT('Ctrl Pts',(53.8030456912114,19.4042782315808,20.3371356589452));
#29758=CARTESIAN_POINT('Ctrl Pts',(53.8032585307919,19.4041186019172,20.3371524960335));
#29759=CARTESIAN_POINT('Ctrl Pts',(53.8033669654118,19.4040372932298,20.3371610737409));
#29760=CARTESIAN_POINT('Ctrl Pts',(53.8035881742186,19.4038714570896,20.3371785719805));
#29761=CARTESIAN_POINT('Ctrl Pts',(53.8037009491561,19.403786930478,20.3371874925538));
#29762=CARTESIAN_POINT('Ctrl Pts',(53.8039311826814,19.4036144048888,20.3372057036876));
#29763=CARTESIAN_POINT('Ctrl Pts',(53.8040486419052,19.403526407011,20.3372149942778));
#29764=CARTESIAN_POINT('Ctrl Pts',(53.8042886244024,19.4033466587275,20.3372339754716));
#29765=CARTESIAN_POINT('Ctrl Pts',(53.8044111485808,19.4032549094197,20.3372436661238));
#29766=CARTESIAN_POINT('Ctrl Pts',(53.8046616835939,19.4030673472566,20.3372634807965));
#29767=CARTESIAN_POINT('Ctrl Pts',(53.8047896954448,19.4029715356475,20.3372736048716));
#29768=CARTESIAN_POINT('Ctrl Pts',(53.805051676911,19.4027755024296,20.3372943235698));
#29769=CARTESIAN_POINT('Ctrl Pts',(53.8051856474742,19.4026752823892,20.3373049182387));
#29770=CARTESIAN_POINT('Ctrl Pts',(53.8053956221648,19.4025182467516,20.3373215229405));
#29771=CARTESIAN_POINT('Ctrl Pts',(53.8054716177938,19.4024614196807,20.337327532531));
#29772=CARTESIAN_POINT('Ctrl Pts',(53.8056425644816,19.4023336103003,20.3373410504267));
#29773=CARTESIAN_POINT('Ctrl Pts',(53.8057375178363,19.4022626310153,20.3373485588524));
#29774=CARTESIAN_POINT('Ctrl Pts',(53.805951791935,19.4021024871712,20.3373655021698));
#29775=CARTESIAN_POINT('Ctrl Pts',(53.806071116382,19.4020133274804,20.3373749372561));
#29776=CARTESIAN_POINT('Ctrl Pts',(53.8063414911553,19.4018113495877,20.337396315415));
#29777=CARTESIAN_POINT('Ctrl Pts',(53.8064925474982,19.4016985394279,20.3374082588024));
#29778=CARTESIAN_POINT('Ctrl Pts',(53.8068366455046,19.4014416400969,20.3374354642049));
#29779=CARTESIAN_POINT('Ctrl Pts',(53.8070296971665,19.4012975645593,20.3374507267399));
#29780=CARTESIAN_POINT('Ctrl Pts',(53.8074725503158,19.4009671856527,20.3374857368146));
#29781=CARTESIAN_POINT('Ctrl Pts',(53.807722369393,19.4007809058282,20.3375054852754));
#29782=CARTESIAN_POINT('Ctrl Pts',(53.813836058201,19.3962244080137,20.3379887503409));
#29783=CARTESIAN_POINT('Ctrl Pts',(53.8197238087314,19.3918864603942,20.3384535154984));
#29784=CARTESIAN_POINT('Ctrl Pts',(53.8333588035398,19.3819557549988,20.3395284342928));
#29785=CARTESIAN_POINT('Ctrl Pts',(53.8411225948208,19.3763861251602,20.3401394666954));
#29786=CARTESIAN_POINT('Ctrl Pts',(53.8613739974453,19.3620773223339,20.3417308180093));
#29787=CARTESIAN_POINT('Ctrl Pts',(53.8739221032475,19.3534252459284,20.3427144188101));
#29788=CARTESIAN_POINT('Ctrl Pts',(53.9673687209747,19.2905604031253,20.3500230239132));
#29789=CARTESIAN_POINT('Ctrl Pts',(54.0520291948315,19.2422009869957,20.3565647329655));
#29790=CARTESIAN_POINT('Ctrl Pts',(54.2662014451588,19.139846297466,20.3728822910458));
#29791=CARTESIAN_POINT('Ctrl Pts',(54.3985303097303,19.0929435951701,20.3827920588229));
#29792=CARTESIAN_POINT('Ctrl Pts',(54.5821668682738,19.048890518195,20.3956923159089));
#29793=CARTESIAN_POINT('Ctrl Pts',(54.6300646841011,19.039244665239,20.3989784177812));
#29794=CARTESIAN_POINT('Ctrl Pts',(54.6871877961556,19.0299092168263,20.4027686921682));
#29795=CARTESIAN_POINT('Ctrl Pts',(54.6961131446509,19.0285127554538,20.4033572108659));
#29796=CARTESIAN_POINT('Ctrl Pts',(54.7099250600226,19.0264477685282,20.4042619023432));
#29797=CARTESIAN_POINT('Ctrl Pts',(54.7148049983627,19.0257366706874,20.4045803796771));
#29798=CARTESIAN_POINT('Ctrl Pts',(54.7238293357576,19.0244558151327,20.405167120805));
#29799=CARTESIAN_POINT('Ctrl Pts',(54.7279728646564,19.0238810004604,20.405435656307));
#29800=CARTESIAN_POINT('Ctrl Pts',(54.7373662011215,19.02260800636,20.4060424824625));
#29801=CARTESIAN_POINT('Ctrl Pts',(54.7426169915334,19.0219176970264,20.4063803282222));
#29802=CARTESIAN_POINT('Ctrl Pts',(54.7582308092374,19.0199282087064,20.4073810634377));
#29803=CARTESIAN_POINT('Ctrl Pts',(54.7686015496836,19.0186894719334,20.408040670648));
#29804=CARTESIAN_POINT('Ctrl Pts',(54.8699296938782,19.0073927619749,20.4144400243648));
#29805=CARTESIAN_POINT('Ctrl Pts',(54.9614804101356,19.0035224452643,20.4198675447271));
#29806=CARTESIAN_POINT('Ctrl Pts',(55.1742802323822,19.0091767730949,20.4323082048308));
#29807=CARTESIAN_POINT('Ctrl Pts',(55.2950260752195,19.0234600784067,20.4392474172708));
#29808=CARTESIAN_POINT('Ctrl Pts',(55.4613563915135,19.0587250241781,20.449335555546));
#29809=CARTESIAN_POINT('Ctrl Pts',(55.5085987887294,19.0705635478535,20.452260273667));
#29810=CARTESIAN_POINT('Ctrl Pts',(55.5761220434655,19.0901365745287,20.4565576935917));
#29811=CARTESIAN_POINT('Ctrl Pts',(55.59678574912,19.0964922830254,20.4578888736637));
#29812=CARTESIAN_POINT('Ctrl Pts',(55.6336970749415,19.1085055061932,20.4602982659284));
#29813=CARTESIAN_POINT('Ctrl Pts',(55.6499827001584,19.1140398033436,20.4613724789185));
#29814=CARTESIAN_POINT('Ctrl Pts',(55.6747353528252,19.1228101126171,20.4630231922844));
#29815=CARTESIAN_POINT('Ctrl Pts',(55.6832555378721,19.1258944706238,20.4635946760777));
#29816=CARTESIAN_POINT('Ctrl Pts',(55.698745816016,19.1316217164249,20.4646398090001));
#29817=CARTESIAN_POINT('Ctrl Pts',(55.7057227081686,19.134245840781,20.4651128256796));
#29818=CARTESIAN_POINT('Ctrl Pts',(55.7207960586341,19.140011820763,20.4661397952983));
#29819=CARTESIAN_POINT('Ctrl Pts',(55.7288870076235,19.1431675597338,20.4666942057045));
#29820=CARTESIAN_POINT('Ctrl Pts',(55.7509119887205,19.151924170374,20.468212193807));
#29821=CARTESIAN_POINT('Ctrl Pts',(55.7648035637279,19.1576296313476,20.4691792728014));
#29822=CARTESIAN_POINT('Ctrl Pts',(55.8362542196819,19.187922740249,20.4742045540793));
#29823=CARTESIAN_POINT('Ctrl Pts',(55.8926916595462,19.2150503381232,20.4783483361877));
#29824=CARTESIAN_POINT('Ctrl Pts',(55.9674512363783,19.2554179112062,20.4840813191748));
#29825=CARTESIAN_POINT('Ctrl Pts',(55.9869654597915,19.2663830624136,20.4856011458115));
#29826=CARTESIAN_POINT('Ctrl Pts',(56.1264336521346,19.3478690979151,20.4966294480829));
#29827=CARTESIAN_POINT('Ctrl Pts',(56.238899543939,19.4304419632926,20.5064579534391));
#29828=CARTESIAN_POINT('Ctrl Pts',(56.3851888059707,19.5634377843653,20.5200806281248));
#29829=CARTESIAN_POINT('Ctrl Pts',(56.4267802694536,19.6047371532754,20.5240622904371));
#29830=CARTESIAN_POINT('Ctrl Pts',(56.4754356628923,19.6575056608068,20.5287963236997));
#29831=CARTESIAN_POINT('Ctrl Pts',(56.484278382368,19.6672887964536,20.529659956273));
#29832=CARTESIAN_POINT('Ctrl Pts',(56.4968326966673,19.6814582181467,20.5308899032649));
#29833=CARTESIAN_POINT('Ctrl Pts',(56.5006231512401,19.6857737210601,20.5312617642927));
#29834=CARTESIAN_POINT('Ctrl Pts',(56.5071756085384,19.6932991244838,20.5319053878705));
#29835=CARTESIAN_POINT('Ctrl Pts',(56.5099461070008,19.6965015349573,20.5321777722523));
#29836=CARTESIAN_POINT('Ctrl Pts',(56.5153641628133,19.7028047025723,20.5327109148783));
#29837=CARTESIAN_POINT('Ctrl Pts',(56.5180124119615,19.705904754872,20.5329717303642));
#29838=CARTESIAN_POINT('Ctrl Pts',(56.5253103928492,19.7145010324666,20.533691174219));
#29839=CARTESIAN_POINT('Ctrl Pts',(56.5299399603325,19.7200144095966,20.5341483487297));
#29840=CARTESIAN_POINT('Ctrl Pts',(56.5482646518245,19.7420788517825,20.5359616435059));
#29841=CARTESIAN_POINT('Ctrl Pts',(56.5617224449554,19.7588263052324,20.5373016945309));
#29842=CARTESIAN_POINT('Ctrl Pts',(56.708638651417,19.9478291851451,20.5520672808868));
#29843=CARTESIAN_POINT('Ctrl Pts',(56.8132943612363,20.1406377052644,20.5640205393494));
#29844=CARTESIAN_POINT('Ctrl Pts',(56.8967253479837,20.3812841817354,20.5793051169766));
#29845=CARTESIAN_POINT('Ctrl Pts',(56.9077942179297,20.4163071924218,20.5815330574227));
#29846=CARTESIAN_POINT('Ctrl Pts',(56.9250479874808,20.4766494398764,20.5853915908788));
#29847=CARTESIAN_POINT('Ctrl Pts',(56.9317151793355,20.5018213864632,20.587006962931));
#29848=CARTESIAN_POINT('Ctrl Pts',(56.9404222412177,20.5375030707621,20.5893080180752));
#29849=CARTESIAN_POINT('Ctrl Pts',(56.9428733631361,20.5479104386847,20.5899805024602));
#29850=CARTESIAN_POINT('Ctrl Pts',(56.9469392486697,20.5658180360187,20.5911401162445));
#29851=CARTESIAN_POINT('Ctrl Pts',(56.9485946461366,20.5733088725716,20.5916259340584));
#29852=CARTESIAN_POINT('Ctrl Pts',(56.9516715395003,20.5876235360544,20.5925558092941));
#29853=CARTESIAN_POINT('Ctrl Pts',(56.9531005625663,20.594445642871,20.5929996181203));
#29854=CARTESIAN_POINT('Ctrl Pts',(56.9567069356368,20.6121235769475,20.5941513911293));
#29855=CARTESIAN_POINT('Ctrl Pts',(56.9588296856044,20.6229901776666,20.594861083312));
#29856=CARTESIAN_POINT('Ctrl Pts',(56.9646401154627,20.654109084914,20.5968985559233));
#29857=CARTESIAN_POINT('Ctrl Pts',(56.9681048236525,20.6744010766302,20.5982333352745));
#29858=CARTESIAN_POINT('Ctrl Pts',(56.9969610546452,20.8607453010119,20.6105510200239));
#29859=CARTESIAN_POINT('Ctrl Pts',(57.0015904874806,21.0293004509427,20.6222154024361));
#29860=CARTESIAN_POINT('Ctrl Pts',(56.9745337637511,21.3027693295947,20.6413733031866));
#29861=CARTESIAN_POINT('Ctrl Pts',(56.9554755471391,21.4081343772677,20.6487886074502));
#29862=CARTESIAN_POINT('Ctrl Pts',(56.9254036700948,21.52149373697,20.6564878113769));
#29863=CARTESIAN_POINT('Ctrl Pts',(56.9226676680258,21.5314922952844,20.657164379718));
#29864=CARTESIAN_POINT('Ctrl Pts',(56.918439575517,21.5464835773153,20.6581745273555));
#29865=CARTESIAN_POINT('Ctrl Pts',(56.917005714003,21.551492338263,20.6585113114148));
#29866=CARTESIAN_POINT('Ctrl Pts',(56.9144992754106,21.5601199266028,20.6590901133012));
#29867=CARTESIAN_POINT('Ctrl Pts',(56.9134360393161,21.5637413697549,20.6593326643263));
#29868=CARTESIAN_POINT('Ctrl Pts',(56.9109874208129,21.5719947666808,20.6598845213071));
#29869=CARTESIAN_POINT('Ctrl Pts',(56.9095954761666,21.5766247082971,20.6601934410468));
#29870=CARTESIAN_POINT('Ctrl Pts',(56.905749752708,21.5892498495434,20.6610341366492));
#29871=CARTESIAN_POINT('Ctrl Pts',(56.9032624711348,21.5972348591337,20.6615640056688));
#29872=CARTESIAN_POINT('Ctrl Pts',(56.8906303508372,21.6369077306927,20.6641885124695));
#29873=CARTESIAN_POINT('Ctrl Pts',(56.8797433796901,21.6683559757757,20.666243131886));
#29874=CARTESIAN_POINT('Ctrl Pts',(56.7962869280656,21.8912273795385,20.6807166516061));
#29875=CARTESIAN_POINT('Ctrl Pts',(56.6954149776349,22.0707571048413,20.6920310262491));
#29876=CARTESIAN_POINT('Ctrl Pts',(56.5351783112772,22.2748529366196,20.707612679437));
#29877=CARTESIAN_POINT('Ctrl Pts',(56.499629453004,22.3164851469472,20.7109527195792));
#29878=CARTESIAN_POINT('Ctrl Pts',(56.4529097316357,22.3668490324397,20.7152345588774));
#29879=CARTESIAN_POINT('Ctrl Pts',(56.4432957732682,22.3769968267517,20.7161102629293));
#29880=CARTESIAN_POINT('Ctrl Pts',(56.4277573257056,22.3930565705028,20.7175175330834));
#29881=CARTESIAN_POINT('Ctrl Pts',(56.4219007941711,22.3990338515577,20.7180461495342));
#29882=CARTESIAN_POINT('Ctrl Pts',(56.4107317234163,22.4102906298756,20.7190510121644));
#29883=CARTESIAN_POINT('Ctrl Pts',(56.4054267089373,22.4155774155677,20.7195269222617));
#29884=CARTESIAN_POINT('Ctrl Pts',(56.393316125218,22.4275112030276,20.7206103365117));
#29885=CARTESIAN_POINT('Ctrl Pts',(56.3864925660458,22.4341396092007,20.7212186389543));
#29886=CARTESIAN_POINT('Ctrl Pts',(56.368714126246,22.4511641144675,20.7227982183236));
#29887=CARTESIAN_POINT('Ctrl Pts',(56.3576882871739,22.4614849094497,20.7237726974782));
#29888=CARTESIAN_POINT('Ctrl Pts',(56.277738870225,22.5346364542036,20.7308035971634));
#29889=CARTESIAN_POINT('Ctrl Pts',(56.2046109017385,22.592681309524,20.7370580497102));
#29890=CARTESIAN_POINT('Ctrl Pts',(56.0090667701674,22.7267011837668,20.7533245050715));
#29891=CARTESIAN_POINT('Ctrl Pts',(55.8819954002998,22.7949356057058,20.7635097693315));
#29892=CARTESIAN_POINT('Ctrl Pts',(55.7029321584625,22.8674452504992,20.77671117087));
#29893=CARTESIAN_POINT('Ctrl Pts',(55.6564908908065,22.8842733358081,20.7800344203223));
#29894=CARTESIAN_POINT('Ctrl Pts',(55.6008431127187,22.9021296436412,20.783861658913));
#29895=CARTESIAN_POINT('Ctrl Pts',(55.5921983921175,22.9048387593697,20.7844518508895));
#29896=CARTESIAN_POINT('Ctrl Pts',(55.5788144436279,22.9089331509356,20.7853585579187));
#29897=CARTESIAN_POINT('Ctrl Pts',(55.5740881596831,22.9103598407331,20.785677393425));
#29898=CARTESIAN_POINT('Ctrl Pts',(55.5653477694354,22.9129628741586,20.7862644656622));
#29899=CARTESIAN_POINT('Ctrl Pts',(55.561335283529,22.9141441320708,20.7865329765632));
#29900=CARTESIAN_POINT('Ctrl Pts',(55.5522407772353,22.9167904575629,20.787139333119));
#29901=CARTESIAN_POINT('Ctrl Pts',(55.547156635804,22.918247938014,20.7874767368483));
#29902=CARTESIAN_POINT('Ctrl Pts',(55.5339899558722,22.9219658489357,20.7883466161601));
#29903=CARTESIAN_POINT('Ctrl Pts',(55.5258987441039,22.9241955498973,20.7888773708691));
#29904=CARTESIAN_POINT('Ctrl Pts',(55.4740513917151,22.938131691854,20.7922554989259));
#29905=CARTESIAN_POINT('Ctrl Pts',(55.4299176142441,22.94839696424,20.7950271583184));
#29906=CARTESIAN_POINT('Ctrl Pts',(55.3630092057832,22.9615748485849,20.7991261236621));
#29907=CARTESIAN_POINT('Ctrl Pts',(55.3404743331046,22.9656115735928,20.8004893063809));
#29908=CARTESIAN_POINT('Ctrl Pts',(55.2669545374997,22.9774790071089,20.8048944116465));
#29909=CARTESIAN_POINT('Ctrl Pts',(55.2157737787945,22.983714093799,20.8078956609588));
#29910=CARTESIAN_POINT('Ctrl Pts',(55.1644479523467,22.9879598671676,20.810886410834));
#29911=CARTESIAN_POINT('Origin',(55.,21.,6.22095488139522));
#29912=CARTESIAN_POINT('',(55.1644483608155,22.9879598333782,21.7678366528264));
#29913=CARTESIAN_POINT('',(55.1644483516286,22.9879598341382,21.6085614209934));
#29914=CARTESIAN_POINT('',(55.1644483516311,22.987959834138,6.22095488139522));
#29915=CARTESIAN_POINT('',(53.005250485173,21.0016376188735,21.1784010577392));
#29916=CARTESIAN_POINT('Ctrl Pts',(55.1644483608155,22.9879598333782,21.7678366528264));
#29917=CARTESIAN_POINT('Ctrl Pts',(55.1754894884733,22.9870464872862,21.7671913811389));
#29918=CARTESIAN_POINT('Ctrl Pts',(55.186524561825,22.9860410289883,21.7665469511083));
#29919=CARTESIAN_POINT('Ctrl Pts',(55.3566374547529,22.9691104636088,21.7566134017014));
#29920=CARTESIAN_POINT('Ctrl Pts',(55.5132226965071,22.9342136858194,21.7474202726949));
#29921=CARTESIAN_POINT('Ctrl Pts',(55.6857571425906,22.8733123194524,21.7361438131223));
#29922=CARTESIAN_POINT('Ctrl Pts',(55.7074187567911,22.865240075279,21.7347075812375));
#29923=CARTESIAN_POINT('Ctrl Pts',(55.7377126217523,22.8533473987926,21.7326678499848));
#29924=CARTESIAN_POINT('Ctrl Pts',(55.746466045348,22.8498391635904,21.7320747651588));
#29925=CARTESIAN_POINT('Ctrl Pts',(55.7616719325975,22.8436193782962,21.7310378769034));
#29926=CARTESIAN_POINT('Ctrl Pts',(55.7681356622597,22.8409356716817,21.7305950170133));
#29927=CARTESIAN_POINT('Ctrl Pts',(55.7816344208231,22.8352475886342,21.7296656876547));
#29928=CARTESIAN_POINT('Ctrl Pts',(55.7886665457517,22.8322366540207,21.7291790015679));
#29929=CARTESIAN_POINT('Ctrl Pts',(55.8053673427886,22.824971940078,21.7280169708546));
#29930=CARTESIAN_POINT('Ctrl Pts',(55.8150198087588,22.820681697367,21.727340391222));
#29931=CARTESIAN_POINT('Ctrl Pts',(55.8476196067839,22.8058808406385,21.7250381717774));
#29932=CARTESIAN_POINT('Ctrl Pts',(55.8704005881403,22.7950117903822,21.7234002974448));
#29933=CARTESIAN_POINT('Ctrl Pts',(55.9244977183062,22.7679295165084,21.7194388900537));
#29934=CARTESIAN_POINT('Ctrl Pts',(55.9556012842391,22.7513128616017,21.7171019741812));
#29935=CARTESIAN_POINT('Ctrl Pts',(56.0761757063756,22.6827290970373,21.70780576173));
#29936=CARTESIAN_POINT('Ctrl Pts',(56.1619791273868,22.6246634769503,21.7006527744721));
#29937=CARTESIAN_POINT('Ctrl Pts',(56.3402035016434,22.4826879312896,21.6847691182636));
#29938=CARTESIAN_POINT('Ctrl Pts',(56.430064454559,22.3962199072172,21.6760433662476));
#29939=CARTESIAN_POINT('Ctrl Pts',(56.5214903327015,22.2900926597736,21.6667673882018));
#29940=CARTESIAN_POINT('Ctrl Pts',(56.5315534803265,22.2781298355654,21.6657404996085));
#29941=CARTESIAN_POINT('Ctrl Pts',(56.5454936556161,22.2611570110496,21.6643110716069));
#29942=CARTESIAN_POINT('Ctrl Pts',(56.5494887350424,22.2562453218568,21.6639005976305));
#29943=CARTESIAN_POINT('Ctrl Pts',(56.5559128907119,22.2482699721786,21.6632393334997));
#29944=CARTESIAN_POINT('Ctrl Pts',(56.5583564243787,22.2452180942187,21.6629875226884));
#29945=CARTESIAN_POINT('Ctrl Pts',(56.5635069596301,22.2387463712643,21.6624561743527));
#29946=CARTESIAN_POINT('Ctrl Pts',(56.566211747806,22.2353247940739,21.6621768002988));
#29947=CARTESIAN_POINT('Ctrl Pts',(56.5728755534315,22.2268379622701,21.6614875878043));
#29948=CARTESIAN_POINT('Ctrl Pts',(56.5768213882813,22.2217623354988,21.6610786763415));
#29949=CARTESIAN_POINT('Ctrl Pts',(56.5914130371749,22.2028042885497,21.659563126334));
#29950=CARTESIAN_POINT('Ctrl Pts',(56.6019009888056,22.1888006068924,21.6584669942006));
#29951=CARTESIAN_POINT('Ctrl Pts',(56.6278988651188,22.1531189057719,21.6557272927243));
#29952=CARTESIAN_POINT('Ctrl Pts',(56.6431614383659,22.1312641394717,21.6540977535843));
#29953=CARTESIAN_POINT('Ctrl Pts',(56.7541733029399,21.9653149961845,21.6420296782565));
#29954=CARTESIAN_POINT('Ctrl Pts',(56.8312565757016,21.8096095261305,21.6323404206636));
#29955=CARTESIAN_POINT('Ctrl Pts',(56.8980562515523,21.614423849292,21.6201214441714));
#29956=CARTESIAN_POINT('Ctrl Pts',(56.9080383943767,21.5826864830215,21.6181349409194));
#29957=CARTESIAN_POINT('Ctrl Pts',(56.9300694382814,21.5059891492683,21.6133175783544));
#29958=CARTESIAN_POINT('Ctrl Pts',(56.9413470110015,21.4608300347892,21.6104673293146));
#29959=CARTESIAN_POINT('Ctrl Pts',(56.9539056028261,21.4018340241064,21.6067067435587));
#29960=CARTESIAN_POINT('Ctrl Pts',(56.9566365082675,21.3883184866554,21.6058427742874));
#29961=CARTESIAN_POINT('Ctrl Pts',(56.9607916846872,21.3665963534099,21.6044498315883));
#29962=CARTESIAN_POINT('Ctrl Pts',(56.9623050887383,21.358407104246,21.6039237000099));
#29963=CARTESIAN_POINT('Ctrl Pts',(56.9650839410229,21.3428249141041,21.6029206109956));
#29964=CARTESIAN_POINT('Ctrl Pts',(56.9663590624453,21.3354338265832,21.6024439700584));
#29965=CARTESIAN_POINT('Ctrl Pts',(56.9691697124369,21.3185752592298,21.6013547772683));
#29966=CARTESIAN_POINT('Ctrl Pts',(56.9706786930536,21.3091036001149,21.6007413959425));
#29967=CARTESIAN_POINT('Ctrl Pts',(56.9750974198979,21.280019390093,21.598853308166));
#29968=CARTESIAN_POINT('Ctrl Pts',(56.9777830365202,21.2603745192495,21.5975715812533));
#29969=CARTESIAN_POINT('Ctrl Pts',(56.9965179649881,21.1062430202525,21.5874619331828));
#29970=CARTESIAN_POINT('Ctrl Pts',(56.999122018261,20.9705028515897,21.5782046123475));
#29971=CARTESIAN_POINT('Ctrl Pts',(56.9767024712422,20.6994497282687,21.5592737915135));
#29972=CARTESIAN_POINT('Ctrl Pts',(56.9514920369751,20.5648360703416,21.5496525999555));
#29973=CARTESIAN_POINT('Ctrl Pts',(56.90844468956,20.4194025784161,21.5396169532412));
#29974=CARTESIAN_POINT('Ctrl Pts',(56.9040054368081,20.4050060266285,21.5386278836632));
#29975=CARTESIAN_POINT('Ctrl Pts',(56.8976871924466,20.3853110990607,21.5372821197988));
#29976=CARTESIAN_POINT('Ctrl Pts',(56.8959484116859,20.3799687528978,21.5369178184527));
#29977=CARTESIAN_POINT('Ctrl Pts',(56.8929368025121,20.3708468166067,21.5362971409745));
#29978=CARTESIAN_POINT('Ctrl Pts',(56.8916751796471,20.3670636036148,21.5360401234846));
#29979=CARTESIAN_POINT('Ctrl Pts',(56.8890335177551,20.3592205390198,21.5355081650716));
#29980=CARTESIAN_POINT('Ctrl Pts',(56.8876517272158,20.3551613334286,21.5352333387765));
#29981=CARTESIAN_POINT('Ctrl Pts',(56.8842875030629,20.3453819294345,21.5345723489344));
#29982=CARTESIAN_POINT('Ctrl Pts',(56.8822920758952,20.3396661784901,21.5341869458362));
#29983=CARTESIAN_POINT('Ctrl Pts',(56.8752544124114,20.3197984494964,21.5328502320829));
#29984=CARTESIAN_POINT('Ctrl Pts',(56.8700782014229,20.305694006168,21.531906470716));
#29985=CARTESIAN_POINT('Ctrl Pts',(56.8377901240749,20.2206952473293,21.5262428437303));
#29986=CARTESIAN_POINT('Ctrl Pts',(56.8068063973553,20.1513294801846,21.5217207456113));
#29987=CARTESIAN_POINT('Ctrl Pts',(56.7365571746062,20.0154530975152,21.5127490369553));
#29988=CARTESIAN_POINT('Ctrl Pts',(56.6972378428167,19.949120564546,21.5083083001996));
#29989=CARTESIAN_POINT('Ctrl Pts',(56.5851592601602,19.7828102857856,21.4966416191271));
#29990=CARTESIAN_POINT('Ctrl Pts',(56.5067868852725,19.6870384723547,21.4893611461833));
#29991=CARTESIAN_POINT('Ctrl Pts',(56.4091330501258,19.5880459794073,21.4807310768693));
#29992=CARTESIAN_POINT('Ctrl Pts',(56.3980666344491,19.5770875735389,21.4797591004909));
#29993=CARTESIAN_POINT('Ctrl Pts',(56.3799328673812,19.5595465696808,21.4781753011375));
#29994=CARTESIAN_POINT('Ctrl Pts',(56.3729439014042,19.5528836115514,21.4775669785422));
#29995=CARTESIAN_POINT('Ctrl Pts',(56.3604351997828,19.5411305742946,21.476481750257));
#29996=CARTESIAN_POINT('Ctrl Pts',(56.3549345471546,19.5360203879577,21.4760057195867));
#29997=CARTESIAN_POINT('Ctrl Pts',(56.3432978951763,19.5253315294743,21.4750010967602));
#29998=CARTESIAN_POINT('Ctrl Pts',(56.3371557074732,19.519759835805,21.4744722221224));
#29999=CARTESIAN_POINT('Ctrl Pts',(56.3208274874634,19.5051327604296,21.473069831216));
#30000=CARTESIAN_POINT('Ctrl Pts',(56.3105832246439,19.4961433208029,21.472193585967));
#30001=CARTESIAN_POINT('Ctrl Pts',(56.2619216879253,19.4543171986168,21.4680474063985));
#30002=CARTESIAN_POINT('Ctrl Pts',(56.2223606117604,19.4228457771348,21.4647225389661));
#30003=CARTESIAN_POINT('Ctrl Pts',(56.0451968588485,19.2925818247809,21.4500158228365));
#30004=CARTESIAN_POINT('Ctrl Pts',(55.8965315001714,19.2100479370119,21.4380549550473));
#30005=CARTESIAN_POINT('Ctrl Pts',(55.6741095994358,19.1212968819479,21.4215038495744));
#30006=CARTESIAN_POINT('Ctrl Pts',(55.6076172798366,19.0987497276618,21.4167227152394));
#30007=CARTESIAN_POINT('Ctrl Pts',(55.5302334514801,19.0769855891393,21.4114457524316));
#30008=CARTESIAN_POINT('Ctrl Pts',(55.5203772594771,19.0742950755907,21.4107789029419));
#30009=CARTESIAN_POINT('Ctrl Pts',(55.5054271191087,19.070337196855,21.4097758111305));
#30010=CARTESIAN_POINT('Ctrl Pts',(55.5003483028555,19.0690140642844,21.4094365058221));
#30011=CARTESIAN_POINT('Ctrl Pts',(55.4912136058819,19.0666727536332,21.4088289331351));
#30012=CARTESIAN_POINT('Ctrl Pts',(55.4871597116672,19.0656472750652,21.408560255185));
#30013=CARTESIAN_POINT('Ctrl Pts',(55.4782784517001,19.0634303506945,21.4079737338022));
#30014=CARTESIAN_POINT('Ctrl Pts',(55.4734498542741,19.0622442050764,21.4076561956255));
#30015=CARTESIAN_POINT('Ctrl Pts',(55.4596555001715,19.05891025977,21.4067527518928));
#30016=CARTESIAN_POINT('Ctrl Pts',(55.4506790785466,19.0568065113292,21.4061693057533));
#30017=CARTESIAN_POINT('Ctrl Pts',(55.3900748667853,19.0430456213015,21.4022581545981));
#30018=CARTESIAN_POINT('Ctrl Pts',(55.3380104075157,19.0333838973928,21.3990345301306));
#30019=CARTESIAN_POINT('Ctrl Pts',(55.1127857324754,19.0007993257279,21.3854345428394));
#30020=CARTESIAN_POINT('Ctrl Pts',(54.9374141623584,18.9985968571262,21.3756462024406));
#30021=CARTESIAN_POINT('Ctrl Pts',(54.7028584519862,19.0265451035192,21.3615363721819));
#30022=CARTESIAN_POINT('Ctrl Pts',(54.6421050202241,19.0366540328981,21.3577952093318));
#30023=CARTESIAN_POINT('Ctrl Pts',(54.5673036422746,19.0526877794598,21.3530343675713));
#30024=CARTESIAN_POINT('Ctrl Pts',(54.5527230945712,19.0559849864387,21.3520990454241));
#30025=CARTESIAN_POINT('Ctrl Pts',(54.5297464152499,19.0614530428467,21.3506129401895));
#30026=CARTESIAN_POINT('Ctrl Pts',(54.5213248296027,19.0635153456678,21.3500656418491));
#30027=CARTESIAN_POINT('Ctrl Pts',(54.5056855770255,19.067453383774,21.3490443259059));
#30028=CARTESIAN_POINT('Ctrl Pts',(54.4984644408627,19.0693148228947,21.3485707767908));
#30029=CARTESIAN_POINT('Ctrl Pts',(54.4824701749443,19.0735335544117,21.3475174359662));
#30030=CARTESIAN_POINT('Ctrl Pts',(54.4737024101165,19.0759103637894,21.3469370214494));
#30031=CARTESIAN_POINT('Ctrl Pts',(54.4482827831913,19.0829879880305,21.3452454080577));
#30032=CARTESIAN_POINT('Ctrl Pts',(54.4316758056237,19.0878455815143,21.3441291508789));
#30033=CARTESIAN_POINT('Ctrl Pts',(54.3943128178246,19.0993040957775,21.3415919297114));
#30034=CARTESIAN_POINT('Ctrl Pts',(54.373597776892,19.1060300751715,21.3401670290836));
#30035=CARTESIAN_POINT('Ctrl Pts',(54.3064508589294,19.1290541181105,21.3354876701956));
#30036=CARTESIAN_POINT('Ctrl Pts',(54.2605140003076,19.1467302658298,21.3321904197213));
#30037=CARTESIAN_POINT('Ctrl Pts',(54.0576257492687,19.2335447568475,21.317201284429));
#30038=CARTESIAN_POINT('Ctrl Pts',(53.9093485913713,19.3210409730612,21.3049954994048));
#30039=CARTESIAN_POINT('Ctrl Pts',(53.7401932157377,19.4528215092422,21.2904000484629));
#30040=CARTESIAN_POINT('Ctrl Pts',(53.7071510813313,19.4803234842571,21.2875169677071));
#30041=CARTESIAN_POINT('Ctrl Pts',(53.6688408555479,19.5143650381535,21.2841600287597));
#30042=CARTESIAN_POINT('Ctrl Pts',(53.6626950440673,19.5198948117678,21.2836210549439));
#30043=CARTESIAN_POINT('Ctrl Pts',(53.6527016922874,19.528999520398,21.2827441852063));
#30044=CARTESIAN_POINT('Ctrl Pts',(53.6488336494572,19.5325516582693,21.2824046646985));
#30045=CARTESIAN_POINT('Ctrl Pts',(53.6419107752789,19.5389597174383,21.2817968649623));
#30046=CARTESIAN_POINT('Ctrl Pts',(53.6388508698496,19.5418099931583,21.2815281737523));
#30047=CARTESIAN_POINT('Ctrl Pts',(53.6328993700287,19.5473888217791,21.281005487869));
#30048=CARTESIAN_POINT('Ctrl Pts',(53.6300069857988,19.550116380785,21.2807514218127));
#30049=CARTESIAN_POINT('Ctrl Pts',(53.6217101913731,19.5579873691435,21.2800224372482));
#30050=CARTESIAN_POINT('Ctrl Pts',(53.6163263857495,19.5631525628869,21.2795491560039));
#30051=CARTESIAN_POINT('Ctrl Pts',(53.590967083496,19.5877568591018,21.2773179696235));
#30052=CARTESIAN_POINT('Ctrl Pts',(53.5713703758551,19.6075841025924,21.2755881774862));
#30053=CARTESIAN_POINT('Ctrl Pts',(53.5166298381279,19.6653414379712,21.2707166801807));
#30054=CARTESIAN_POINT('Ctrl Pts',(53.4825348362847,19.7042373872366,21.2676335129944));
#30055=CARTESIAN_POINT('Ctrl Pts',(53.4046658687933,19.8003663151258,21.2603500855115));
#30056=CARTESIAN_POINT('Ctrl Pts',(53.3624054867302,19.8587301986654,21.2561907234951));
#30057=CARTESIAN_POINT('Ctrl Pts',(53.2492689929766,20.0342434705624,21.2440673642995));
#30058=CARTESIAN_POINT('Ctrl Pts',(53.1871822114731,20.15653730859,21.2360548292074));
#30059=CARTESIAN_POINT('Ctrl Pts',(53.1325808302092,20.2985659809651,21.2266086550836));
#30060=CARTESIAN_POINT('Ctrl Pts',(53.1272290215093,20.312982620174,21.225648729359));
#30061=CARTESIAN_POINT('Ctrl Pts',(53.1188087439455,20.3364948153727,21.224080735826));
#30062=CARTESIAN_POINT('Ctrl Pts',(53.1156382386956,20.3455533488254,21.2234760532983));
#30063=CARTESIAN_POINT('Ctrl Pts',(53.1101064464288,20.3617318869616,21.2223949001358));
#30064=CARTESIAN_POINT('Ctrl Pts',(53.1077197036348,20.3688430421607,21.2219192804384));
#30065=CARTESIAN_POINT('Ctrl Pts',(53.102768938251,20.3838740728872,21.2209130162123));
#30066=CARTESIAN_POINT('Ctrl Pts',(53.1002142767571,20.391796857929,21.2203820743571));
#30067=CARTESIAN_POINT('Ctrl Pts',(53.0935647224293,20.4128698701276,21.2189683152526));
#30068=CARTESIAN_POINT('Ctrl Pts',(53.0895563650892,20.4260467275007,21.2180826892937));
#30069=CARTESIAN_POINT('Ctrl Pts',(53.0810829516582,20.4549743812938,21.2161345767535));
#30070=CARTESIAN_POINT('Ctrl Pts',(53.0766747347695,20.4707406484973,21.2150703190758));
#30071=CARTESIAN_POINT('Ctrl Pts',(53.027692490045,20.6546277544868,21.2026265739537));
#30072=CARTESIAN_POINT('Ctrl Pts',(53.0051081067482,20.8277933531142,21.1905097787254));
#30073=CARTESIAN_POINT('Ctrl Pts',(53.0052506707585,21.0016358455293,21.1784008569847));
#30074=CARTESIAN_POINT('Ctrl Pts',(53.005250672195,21.0016375962395,21.1784007350398));
#30075=CARTESIAN_POINT('Ctrl Pts',(53.0053322847788,21.1010495530643,21.1714762398423));
#30076=CARTESIAN_POINT('Ctrl Pts',(53.0128454026382,21.2003316121899,21.1646030799111));
#30077=CARTESIAN_POINT('Ctrl Pts',(53.0288374103171,21.305941096795,21.157590323553));
#30078=CARTESIAN_POINT('Ctrl Pts',(53.0299815660941,21.3132240151852,21.1571082961377));
#30079=CARTESIAN_POINT('Ctrl Pts',(53.0319522638281,21.3253300052478,21.1563098624624));
#30080=CARTESIAN_POINT('Ctrl Pts',(53.0327562126103,21.3301566088289,21.1559922762268));
#30081=CARTESIAN_POINT('Ctrl Pts',(53.0342446887376,21.3388943543456,21.1554187516605));
#30082=CARTESIAN_POINT('Ctrl Pts',(53.0349231460854,21.34280648483,21.1551624821585));
#30083=CARTESIAN_POINT('Ctrl Pts',(53.0363404120851,21.3508362660986,21.1546375714133));
#30084=CARTESIAN_POINT('Ctrl Pts',(53.0370804846131,21.354953573736,21.154369017967));
#30085=CARTESIAN_POINT('Ctrl Pts',(53.0387837606977,21.3642612959843,21.1537632468667));
#30086=CARTESIAN_POINT('Ctrl Pts',(53.0397546169511,21.3694502251133,21.1534264665324));
#30087=CARTESIAN_POINT('Ctrl Pts',(53.0426917494388,21.3848107322295,21.1524321033939));
#30088=CARTESIAN_POINT('Ctrl Pts',(53.0447167141181,21.394971100467,21.1517777403337));
#30089=CARTESIAN_POINT('Ctrl Pts',(53.0632279488014,21.4842191290419,21.1460558551156));
#30090=CARTESIAN_POINT('Ctrl Pts',(53.084427682745,21.5622633851735,21.1412309674618));
#30091=CARTESIAN_POINT('Ctrl Pts',(53.1266578367985,21.6871853962932,21.1334902187382));
#30092=CARTESIAN_POINT('Ctrl Pts',(53.1448610539504,21.7349111127156,21.1305286757426));
#30093=CARTESIAN_POINT('Ctrl Pts',(53.2199468207642,21.9111408890913,21.1194153198988));
#30094=CARTESIAN_POINT('Ctrl Pts',(53.2885113574716,22.0341990223419,21.111257545834));
#30095=CARTESIAN_POINT('Ctrl Pts',(53.3834686793468,22.1689517127133,21.101105735441));
#30096=CARTESIAN_POINT('Ctrl Pts',(53.3978717768692,22.1886154522353,21.0995919441415));
#30097=CARTESIAN_POINT('Ctrl Pts',(53.4189398004808,22.2162996055119,21.0974113080032));
#30098=CARTESIAN_POINT('Ctrl Pts',(53.4253132701114,22.2245398241708,21.0967558338938));
#30099=CARTESIAN_POINT('Ctrl Pts',(53.4364622905516,22.2387233410145,21.0956162387663));
#30100=CARTESIAN_POINT('Ctrl Pts',(53.4412079527354,22.2446899353636,21.0951333104319));
#30101=CARTESIAN_POINT('Ctrl Pts',(53.4503955428175,22.2561062924043,21.0942023865234));
#30102=CARTESIAN_POINT('Ctrl Pts',(53.4548323155932,22.2615600724975,21.0937546025345));
#30103=CARTESIAN_POINT('Ctrl Pts',(53.4653686668489,22.2743726257586,21.0926952935831));
#30104=CARTESIAN_POINT('Ctrl Pts',(53.471492444971,22.281711187017,21.092082792144));
#30105=CARTESIAN_POINT('Ctrl Pts',(53.4930903730536,22.3072186088595,21.089933357403));
#30106=CARTESIAN_POINT('Ctrl Pts',(53.508837134781,22.3251529506211,21.0883852841783));
#30107=CARTESIAN_POINT('Ctrl Pts',(53.6234263253456,22.4510319975778,21.0772485765513));
#30108=CARTESIAN_POINT('Ctrl Pts',(53.7335461640153,22.5480725214266,21.0671618433791));
#30109=CARTESIAN_POINT('Ctrl Pts',(53.947353604871,22.6982892958558,21.0489388683708));
#30110=CARTESIAN_POINT('Ctrl Pts',(54.0469939028785,22.7561420860029,21.0408955937351));
#30111=CARTESIAN_POINT('Ctrl Pts',(54.1622700084183,22.8103560858603,21.0324335956188));
#30112=CARTESIAN_POINT('Ctrl Pts',(54.1735172351009,22.8155183703401,21.0316165697683));
#30113=CARTESIAN_POINT('Ctrl Pts',(54.193537021413,22.8244825056827,21.0301783693731));
#30114=CARTESIAN_POINT('Ctrl Pts',(54.2022901381784,22.8283265393486,21.0295549474005));
#30115=CARTESIAN_POINT('Ctrl Pts',(54.2157007015176,22.8341013014988,21.0286083928622));
#30116=CARTESIAN_POINT('Ctrl Pts',(54.2203382469923,22.8360774836633,21.028282619978));
#30117=CARTESIAN_POINT('Ctrl Pts',(54.2249951480002,22.8380410882356,21.0279570831576));
#30118=CARTESIAN_POINT('Ctrl Pts',(54.2250070003433,22.8380460856977,21.0279562546397));
#30119=CARTESIAN_POINT('Ctrl Pts',(54.2250307442186,22.8380560968752,21.0279545948851));
#30120=CARTESIAN_POINT('Ctrl Pts',(54.2250426358363,22.8380611106258,21.0279537636426));
#30121=CARTESIAN_POINT('Ctrl Pts',(54.2250664589854,22.8380711546831,21.0279520983883));
#30122=CARTESIAN_POINT('Ctrl Pts',(54.225078389809,22.8380761846906,21.0279512644262));
#30123=CARTESIAN_POINT('Ctrl Pts',(54.2251022913704,22.8380862612591,21.0279495937329));
#30124=CARTESIAN_POINT('Ctrl Pts',(54.2251142621585,22.8380913078405,21.0279487569983));
#30125=CARTESIAN_POINT('Ctrl Pts',(54.2251382431699,22.8381014173521,21.0279470807938));
#30126=CARTESIAN_POINT('Ctrl Pts',(54.225150254146,22.8381064805989,21.0279462412714));
#30127=CARTESIAN_POINT('Ctrl Pts',(54.2251743160498,22.8381166236564,21.0279445594553));
#30128=CARTESIAN_POINT('Ctrl Pts',(54.22518636697,22.8381217034631,21.0279437171623));
#30129=CARTESIAN_POINT('Ctrl Pts',(54.2252105096485,22.8381318800111,21.0279420297433));
#30130=CARTESIAN_POINT('Ctrl Pts',(54.2252226008182,22.8381369765034,21.0279411846586));
#30131=CARTESIAN_POINT('Ctrl Pts',(54.2252468237802,22.8381471863294,21.0279394916714));
#30132=CARTESIAN_POINT('Ctrl Pts',(54.2252589559682,22.8381522998288,21.0279386437415));
#30133=CARTESIAN_POINT('Ctrl Pts',(54.2252832614519,22.8381625438704,21.0279369450302));
#30134=CARTESIAN_POINT('Ctrl Pts',(54.2252954342968,22.8381676742216,21.0279360942805));
#30135=CARTESIAN_POINT('Ctrl Pts',(54.2253198208907,22.8381779518781,21.0279343899441));
#30136=CARTESIAN_POINT('Ctrl Pts',(54.2253320352925,22.8381830994576,21.027933536312));
#30137=CARTESIAN_POINT('Ctrl Pts',(54.2253565055625,22.8381934118048,21.0279318261717));
#30138=CARTESIAN_POINT('Ctrl Pts',(54.2253687610663,22.8381985764179,21.0279309696892));
#30139=CARTESIAN_POINT('Ctrl Pts',(54.225393313842,22.8382089229567,21.0279292538272));
#30140=CARTESIAN_POINT('Ctrl Pts',(54.2254056111861,22.8382141049116,21.0279283944428));
#30141=CARTESIAN_POINT('Ctrl Pts',(54.2254302477906,22.8382244861936,21.0279266727672));
#30142=CARTESIAN_POINT('Ctrl Pts',(54.2254425870652,22.8382296855255,21.027925810475));
#30143=CARTESIAN_POINT('Ctrl Pts',(54.2254673075629,22.8382401015718,21.0279240829816));
#30144=CARTESIAN_POINT('Ctrl Pts',(54.2254796891657,22.8382453184452,21.0279232177539));
#30145=CARTESIAN_POINT('Ctrl Pts',(54.2255044947943,22.8382557697714,21.0279214843568));
#30146=CARTESIAN_POINT('Ctrl Pts',(54.2255169186937,22.83826100417,21.0279206161962));
#30147=CARTESIAN_POINT('Ctrl Pts',(54.2255418089976,22.8382714905781,21.0279188769275));
#30148=CARTESIAN_POINT('Ctrl Pts',(54.2255542757953,22.8382767427523,21.0279180057921));
#30149=CARTESIAN_POINT('Ctrl Pts',(54.2255792523612,22.8382872649047,21.0279162605416));
#30150=CARTESIAN_POINT('Ctrl Pts',(54.2255917619571,22.8382925348093,21.0279153864386));
#30151=CARTESIAN_POINT('Ctrl Pts',(54.2256168241989,22.8383030924528,21.0279136352477));
#30152=CARTESIAN_POINT('Ctrl Pts',(54.225629377232,22.8383083803539,21.0279127581327));
#30153=CARTESIAN_POINT('Ctrl Pts',(54.2256545279549,22.8383189746641,21.0279110008058));
#30154=CARTESIAN_POINT('Ctrl Pts',(54.2256671237389,22.8383242802694,21.0279101207271));
#30155=CARTESIAN_POINT('Ctrl Pts',(54.2256923587314,22.8383349094659,21.027908357559));
#30156=CARTESIAN_POINT('Ctrl Pts',(54.2257049994303,22.8383402336839,21.0279074743655));
#30157=CARTESIAN_POINT('Ctrl Pts',(54.2257303246679,22.8383509002773,21.0279057049391));
#30158=CARTESIAN_POINT('Ctrl Pts',(54.2257430087781,22.8383562424714,21.0279048187363));
#30159=CARTESIAN_POINT('Ctrl Pts',(54.2257684214111,22.8383669452551,21.0279030432513));
#30160=CARTESIAN_POINT('Ctrl Pts',(54.2257811500112,22.8383723058763,21.0279021539638));
#30161=CARTESIAN_POINT('Ctrl Pts',(54.2258066517887,22.8383830455804,21.0279003722985));
#30162=CARTESIAN_POINT('Ctrl Pts',(54.2258194249518,22.8383884246562,21.0278994799217));
#30163=CARTESIAN_POINT('Ctrl Pts',(54.2258450164915,22.8383992015344,21.0278976920333));
#30164=CARTESIAN_POINT('Ctrl Pts',(54.2258578343551,22.8384045991196,21.0278967965577));
#30165=CARTESIAN_POINT('Ctrl Pts',(54.2258835147597,22.8384154127873,21.0278950025096));
#30166=CARTESIAN_POINT('Ctrl Pts',(54.2258963782554,22.8384208292708,21.0278941038705));
#30167=CARTESIAN_POINT('Ctrl Pts',(54.2259223469412,22.838431763688,21.0278922897321));
#30168=CARTESIAN_POINT('Ctrl Pts',(54.2259354515801,22.8384372813837,21.0278913742718));
#30169=CARTESIAN_POINT('Ctrl Pts',(54.2259618723448,22.8384484054889,21.0278895286029));
#30170=CARTESIAN_POINT('Ctrl Pts',(54.2259751888655,22.8384540120593,21.027888598367));
#30171=CARTESIAN_POINT('Ctrl Pts',(54.2260020374324,22.838465315598,21.0278867228658));
#30172=CARTESIAN_POINT('Ctrl Pts',(54.2260155689803,22.8384710123509,21.0278857776358));
#30173=CARTESIAN_POINT('Ctrl Pts',(54.22988310725,22.840099187491,21.0276156192607));
#30174=CARTESIAN_POINT('Ctrl Pts',(54.2337421568283,22.8417095228866,21.0273471556168));
#30175=CARTESIAN_POINT('Ctrl Pts',(54.2424559505845,22.8453135553225,21.0267434228915));
#30176=CARTESIAN_POINT('Ctrl Pts',(54.2473135065905,22.8473002323446,21.0264085780969));
#30177=CARTESIAN_POINT('Ctrl Pts',(54.259832454678,22.8523627406793,21.0255498640903));
#30178=CARTESIAN_POINT('Ctrl Pts',(54.2675052925616,22.8554102585024,21.0250276423215));
#30179=CARTESIAN_POINT('Ctrl Pts',(54.3149519512032,22.8739150443583,21.021822183402));
#30180=CARTESIAN_POINT('Ctrl Pts',(54.3551975520365,22.8881416333466,21.019206035753));
#30181=CARTESIAN_POINT('Ctrl Pts',(54.5817331220043,22.9601309526944,21.0048847124341));
#30182=CARTESIAN_POINT('Ctrl Pts',(54.7752579932607,22.9916237211284,20.994046820029));
#30183=CARTESIAN_POINT('Ctrl Pts',(55.0241517734538,22.9953310106371,20.9790903481579));
#30184=CARTESIAN_POINT('Ctrl Pts',(55.0780184315487,22.993951225774,20.9758013057958));
#30185=CARTESIAN_POINT('Ctrl Pts',(55.1426627704664,22.9896719049851,20.9717628580345));
#30186=CARTESIAN_POINT('Ctrl Pts',(55.1535592789421,22.9888606018617,20.9710790367903));
#30187=CARTESIAN_POINT('Ctrl Pts',(55.164448351653,22.9879598341362,20.9703924394033));
#30188=CARTESIAN_POINT('Ctrl Pts',(55.1644479523467,22.9879598671676,20.810886410834));
#30189=CARTESIAN_POINT('Ctrl Pts',(55.0607747998254,22.996535914364,20.8169274332477));
#30190=CARTESIAN_POINT('Ctrl Pts',(54.9565102499621,22.9969957235706,20.8229336150651));
#30191=CARTESIAN_POINT('Ctrl Pts',(54.7871697271686,22.9844485452913,20.8330572124156));
#30192=CARTESIAN_POINT('Ctrl Pts',(54.7220202242319,22.9763751295009,20.8370398260191));
#30193=CARTESIAN_POINT('Ctrl Pts',(54.6428512111315,22.9625723296193,20.8420434974395));
#30194=CARTESIAN_POINT('Ctrl Pts',(54.6283399102779,22.9598760587348,20.8429673847499));
#30195=CARTESIAN_POINT('Ctrl Pts',(54.6054820931037,22.9553659781349,20.8444338846554));
#30196=CARTESIAN_POINT('Ctrl Pts',(54.5971148275945,22.9536591364652,20.8449730902119));
#30197=CARTESIAN_POINT('Ctrl Pts',(54.5814541126815,22.9503596158121,20.8459868844609));
#30198=CARTESIAN_POINT('Ctrl Pts',(54.5741581212833,22.9487796136636,20.8464610603752));
#30199=CARTESIAN_POINT('Ctrl Pts',(54.5578435286914,22.9451505725202,20.8475256388784));
#30200=CARTESIAN_POINT('Ctrl Pts',(54.54883000943,22.9430797023654,20.8481167320197));
#30201=CARTESIAN_POINT('Ctrl Pts',(54.5259819443459,22.9376627757252,20.8496226781042));
#30202=CARTESIAN_POINT('Ctrl Pts',(54.512168395776,22.934231231783,20.8505402554928));
#30203=CARTESIAN_POINT('Ctrl Pts',(54.4295138122808,22.9127565646085,20.8560744079859));
#30204=CARTESIAN_POINT('Ctrl Pts',(54.3616495662766,22.8911897913354,20.8608038358385));
#30205=CARTESIAN_POINT('Ctrl Pts',(54.1408558293645,22.8077835037583,20.8768148038097));
#30206=CARTESIAN_POINT('Ctrl Pts',(53.9944622246104,22.7306340577721,20.8885199670784));
#30207=CARTESIAN_POINT('Ctrl Pts',(53.8166267864544,22.606659065544,20.9033580391712));
#30208=CARTESIAN_POINT('Ctrl Pts',(53.7751892755048,22.5752984623301,20.9068594888647));
#30209=CARTESIAN_POINT('Ctrl Pts',(53.7279255786372,22.5365345459115,20.9108634338554));
#30210=CARTESIAN_POINT('Ctrl Pts',(53.720871427009,22.5306671244297,20.9114612925065));
#30211=CARTESIAN_POINT('Ctrl Pts',(53.7100651988452,22.5215519675486,20.9123772290469));
#30212=CARTESIAN_POINT('Ctrl Pts',(53.7062844471068,22.5183386482216,20.9126977008354));
#30213=CARTESIAN_POINT('Ctrl Pts',(53.6993400526779,22.5123917297111,20.9132862998663));
#30214=CARTESIAN_POINT('Ctrl Pts',(53.696173029607,22.5096623048016,20.9135547124873));
#30215=CARTESIAN_POINT('Ctrl Pts',(53.6890428222301,22.5034781279048,20.9141589873155));
#30216=CARTESIAN_POINT('Ctrl Pts',(53.6850847075932,22.5000176593484,20.9144944208466));
#30217=CARTESIAN_POINT('Ctrl Pts',(53.6734401596926,22.4897556485784,20.9154813764055));
#30218=CARTESIAN_POINT('Ctrl Pts',(53.6657923467358,22.4829102639633,20.9161297485774));
#30219=CARTESIAN_POINT('Ctrl Pts',(53.6048867112353,22.4275423767511,20.9212978745806));
#30220=CARTESIAN_POINT('Ctrl Pts',(53.5542341825184,22.3762201717164,20.9256253066365));
#30221=CARTESIAN_POINT('Ctrl Pts',(53.4271726144829,22.2327004626461,20.9369275071537));
#30222=CARTESIAN_POINT('Ctrl Pts',(53.3560959872718,22.1361855191913,20.9437532269365));
#30223=CARTESIAN_POINT('Ctrl Pts',(53.2499066655382,21.9609729685995,20.9557888787442));
#30224=CARTESIAN_POINT('Ctrl Pts',(53.2104437629289,21.8853144724378,20.9608834796954));
#30225=CARTESIAN_POINT('Ctrl Pts',(53.1673086845007,21.7878611814792,20.9674673932946));
#30226=CARTESIAN_POINT('Ctrl Pts',(53.1589876256663,21.76821616887,20.9687953401201));
#30227=CARTESIAN_POINT('Ctrl Pts',(53.14727819746,21.7392881761845,20.9707535662719));
#30228=CARTESIAN_POINT('Ctrl Pts',(53.1436409897681,21.730107050058,20.9713754655968));
#30229=CARTESIAN_POINT('Ctrl Pts',(53.137348871242,21.7138733203298,20.9724759578109));
#30230=CARTESIAN_POINT('Ctrl Pts',(53.1346654511749,21.7068319201607,20.9729535847927));
#30231=CARTESIAN_POINT('Ctrl Pts',(53.1291518034536,21.6921138118543,20.9739526086676));
#30232=CARTESIAN_POINT('Ctrl Pts',(53.1263287859798,21.6844345706829,20.9744742354621));
#30233=CARTESIAN_POINT('Ctrl Pts',(53.1190980852496,21.6643854226842,20.9758372133588));
#30234=CARTESIAN_POINT('Ctrl Pts',(53.114765224729,21.6519891342783,20.9766810252979));
#30235=CARTESIAN_POINT('Ctrl Pts',(53.0975028005418,21.6009902497448,20.9801575439806));
#30236=CARTESIAN_POINT('Ctrl Pts',(53.0856348185771,21.5620413017555,20.9828246855955));
#30237=CARTESIAN_POINT('Ctrl Pts',(53.028566217451,21.3518890833527,20.9972889867062));
#30238=CARTESIAN_POINT('Ctrl Pts',(53.0051280468784,21.1756195821554,21.0097777439398));
#30239=CARTESIAN_POINT('Ctrl Pts',(53.0052524267199,20.9958016574577,21.0222204356035));
#30240=CARTESIAN_POINT('Ctrl Pts',(53.0052603502379,20.9929831433015,21.0224153664104));
#30241=CARTESIAN_POINT('Ctrl Pts',(53.0056217097114,20.9196951694295,21.0274813119119));
#30242=CARTESIAN_POINT('Ctrl Pts',(53.0097033071661,20.8492852761408,21.0322848098706));
#30243=CARTESIAN_POINT('Ctrl Pts',(53.0186359288415,20.7690703041183,21.0375831626515));
#30244=CARTESIAN_POINT('Ctrl Pts',(53.019845685345,20.7589170107111,21.0382505606658));
#30245=CARTESIAN_POINT('Ctrl Pts',(53.0217945846738,20.7435658944533,21.0392542530492));
#30246=CARTESIAN_POINT('Ctrl Pts',(53.0224762402142,20.7383611329974,21.039593616657));
#30247=CARTESIAN_POINT('Ctrl Pts',(53.0237376682904,20.7290161721705,21.040201175821));
#30248=CARTESIAN_POINT('Ctrl Pts',(53.0243099149544,20.7248750692493,21.040469782762));
#30249=CARTESIAN_POINT('Ctrl Pts',(53.0255907784974,20.7158161258814,21.0410560055694));
#30250=CARTESIAN_POINT('Ctrl Pts',(53.0263047505476,20.7108991320484,21.0413733172875));
#30251=CARTESIAN_POINT('Ctrl Pts',(53.0283941097554,20.6968786728761,21.042275737437));
#30252=CARTESIAN_POINT('Ctrl Pts',(53.0298141815836,20.687781848586,21.0428583943469));
#30253=CARTESIAN_POINT('Ctrl Pts',(53.0397818503727,20.6267078666301,21.046752979971));
#30254=CARTESIAN_POINT('Ctrl Pts',(53.0503232228468,20.5750720645046,21.0499618260359));
#30255=CARTESIAN_POINT('Ctrl Pts',(53.1039549720638,20.3568568521578,21.06339359009));
#30256=CARTESIAN_POINT('Ctrl Pts',(53.1664488662943,20.1958125201965,21.0730432686712));
#30257=CARTESIAN_POINT('Ctrl Pts',(53.2795393011145,19.9884895491317,21.0871270167766));
#30258=CARTESIAN_POINT('Ctrl Pts',(53.3129355221435,19.9337211433496,21.0910184663241));
#30259=CARTESIAN_POINT('Ctrl Pts',(53.3573943226106,19.8681418585539,21.095947964784));
#30260=CARTESIAN_POINT('Ctrl Pts',(53.3660223049345,19.8557215653789,21.0968940302188));
#30261=CARTESIAN_POINT('Ctrl Pts',(53.3798399594767,19.8363055184964,21.0983933471359));
#30262=CARTESIAN_POINT('Ctrl Pts',(53.3849357712523,19.8292434342186,21.0989430068283));
#30263=CARTESIAN_POINT('Ctrl Pts',(53.3944359884939,19.8162575216839,21.0999618720456));
#30264=CARTESIAN_POINT('Ctrl Pts',(53.3988273641279,19.8103243140464,21.1004305672717));
#30265=CARTESIAN_POINT('Ctrl Pts',(53.4086466367444,19.7972103007902,21.1014736744091));
#30266=CARTESIAN_POINT('Ctrl Pts',(53.4140903863336,19.7900416204828,21.1020487005374));
#30267=CARTESIAN_POINT('Ctrl Pts',(53.4299018347962,19.7695101116523,21.1037097077394));
#30268=CARTESIAN_POINT('Ctrl Pts',(53.4403910053048,19.7562422389693,21.1048004714814));
#30269=CARTESIAN_POINT('Ctrl Pts',(53.5294789626568,19.646453003812,21.1139754182195));
#30270=CARTESIAN_POINT('Ctrl Pts',(53.616770879032,19.5573674759639,21.1224223843391));
#30271=CARTESIAN_POINT('Ctrl Pts',(53.8135955734517,19.3908833003054,21.1403054012116));
#30272=CARTESIAN_POINT('Ctrl Pts',(53.9237962988855,19.3151855115299,21.1497241419293));
#30273=CARTESIAN_POINT('Ctrl Pts',(54.0670432726131,19.236616875302,21.1607240020551));
#30274=CARTESIAN_POINT('Ctrl Pts',(54.0936814613359,19.2227787874426,21.1627197828048));
#30275=CARTESIAN_POINT('Ctrl Pts',(54.1279498230423,19.2059479731373,21.165215402546));
#30276=CARTESIAN_POINT('Ctrl Pts',(54.1352983669861,19.2023945712077,21.1657464343511));
#30277=CARTESIAN_POINT('Ctrl Pts',(54.1469496903084,19.1968485334546,21.166581646576));
#30278=CARTESIAN_POINT('Ctrl Pts',(54.1512380200002,19.1948260071072,21.1668876135982));
#30279=CARTESIAN_POINT('Ctrl Pts',(54.1593501879724,19.1910353228318,21.1674636400885));
#30280=CARTESIAN_POINT('Ctrl Pts',(54.1631723725153,19.1892640082249,21.1677338828896));
#30281=CARTESIAN_POINT('Ctrl Pts',(54.1720788830915,19.1851706892469,21.168360949825));
#30282=CARTESIAN_POINT('Ctrl Pts',(54.1771673837641,19.1828579333268,21.1687172061123));
#30283=CARTESIAN_POINT('Ctrl Pts',(54.1935110091238,19.175512380475,21.1698552619206));
#30284=CARTESIAN_POINT('Ctrl Pts',(54.2048033565135,19.1705624136211,21.1706321985194));
#30285=CARTESIAN_POINT('Ctrl Pts',(54.3130659566382,19.1242976845961,21.1779983881825));
#30286=CARTESIAN_POINT('Ctrl Pts',(54.4131355355802,19.0906195111814,21.1841829062938));
#30287=CARTESIAN_POINT('Ctrl Pts',(54.6765656156305,19.0246474760511,21.1999787370729));
#30288=CARTESIAN_POINT('Ctrl Pts',(54.8421114337565,19.0045820930814,21.2095028665368));
#30289=CARTESIAN_POINT('Ctrl Pts',(55.0312670312721,19.0053619564736,21.2211675716505));
#30290=CARTESIAN_POINT('Ctrl Pts',(55.0543058831779,19.0058562352423,21.2226001082778));
#30291=CARTESIAN_POINT('Ctrl Pts',(55.0864909194811,19.0071048881377,21.2246199266721));
#30292=CARTESIAN_POINT('Ctrl Pts',(55.0956488701582,19.007523426694,21.2251967483059));
#30293=CARTESIAN_POINT('Ctrl Pts',(55.1124205152232,19.0084058219758,21.2262571184485));
#30294=CARTESIAN_POINT('Ctrl Pts',(55.1200350921361,19.0088502526915,21.2267400516506));
#30295=CARTESIAN_POINT('Ctrl Pts',(55.1354650635701,19.0098396660368,21.2277217957827));
#30296=CARTESIAN_POINT('Ctrl Pts',(55.1432801648812,19.0103870402011,21.2282206733199));
#30297=CARTESIAN_POINT('Ctrl Pts',(55.1625749229147,19.0118527264968,21.2294564913953));
#30298=CARTESIAN_POINT('Ctrl Pts',(55.1740501233725,19.0128244335148,21.2301950923758));
#30299=CARTESIAN_POINT('Ctrl Pts',(55.2168979160124,19.0168267173064,21.232966910265));
#30300=CARTESIAN_POINT('Ctrl Pts',(55.2482042892155,19.0205012205246,21.2350201391712));
#30301=CARTESIAN_POINT('Ctrl Pts',(55.3262796039344,19.0315462930793,21.2402139339355));
#30302=CARTESIAN_POINT('Ctrl Pts',(55.3728959275262,19.0398427568471,21.2433815418917));
#30303=CARTESIAN_POINT('Ctrl Pts',(55.6011945313129,19.0889122944167,21.2592164764453));
#30304=CARTESIAN_POINT('Ctrl Pts',(55.7768184069374,19.1533185692433,21.2725258087657));
#30305=CARTESIAN_POINT('Ctrl Pts',(55.9698275937065,19.2565740163141,21.2873009953332));
#30306=CARTESIAN_POINT('Ctrl Pts',(55.9983168572191,19.2727294738059,21.2894827237641));
#30307=CARTESIAN_POINT('Ctrl Pts',(56.0335291870929,19.2938598645046,21.2921685141227));
#30308=CARTESIAN_POINT('Ctrl Pts',(56.040634390702,19.2981842599001,21.292709890484));
#30309=CARTESIAN_POINT('Ctrl Pts',(56.0518175443412,19.3050868201141,21.2935608294094));
#30310=CARTESIAN_POINT('Ctrl Pts',(56.0559134506624,19.3076354943915,21.2938722448973));
#30311=CARTESIAN_POINT('Ctrl Pts',(56.0631986742712,19.3122054633305,21.2944256496041));
#30312=CARTESIAN_POINT('Ctrl Pts',(56.0663914773328,19.3142209408065,21.2946680067641));
#30313=CARTESIAN_POINT('Ctrl Pts',(56.0739884292041,19.319046785339,21.2952442704191));
#30314=CARTESIAN_POINT('Ctrl Pts',(56.0783872735819,19.3218653970495,21.2955776266578));
#30315=CARTESIAN_POINT('Ctrl Pts',(56.0915406858704,19.3303666790431,21.296573638163));
#30316=CARTESIAN_POINT('Ctrl Pts',(56.1002619431771,19.3361009156461,21.2972329814958));
#30317=CARTESIAN_POINT('Ctrl Pts',(56.1202460294453,19.3494663094813,21.298742363761));
#30318=CARTESIAN_POINT('Ctrl Pts',(56.1314767223204,19.3571448393298,21.2995895330275));
#30319=CARTESIAN_POINT('Ctrl Pts',(56.2619017494144,19.448289590134,21.3094263295463));
#30320=CARTESIAN_POINT('Ctrl Pts',(56.3717131834456,19.5444534397024,21.3177161122047));
#30321=CARTESIAN_POINT('Ctrl Pts',(56.5540551939484,19.743269896032,21.3334073631076));
#30322=CARTESIAN_POINT('Ctrl Pts',(56.6292704697401,19.8424466390739,21.3407275117804));
#30323=CARTESIAN_POINT('Ctrl Pts',(56.7029816580882,19.9611913644653,21.3494017022039));
#30324=CARTESIAN_POINT('Ctrl Pts',(56.7110366769455,19.9745131021159,21.3503732839847));
#30325=CARTESIAN_POINT('Ctrl Pts',(56.7238322627505,19.996245514217,21.3519564735784));
#30326=CARTESIAN_POINT('Ctrl Pts',(56.7286692408183,20.0045988806489,21.3525645841544));
#30327=CARTESIAN_POINT('Ctrl Pts',(56.7371592383367,20.0195094696699,21.3536494538004));
#30328=CARTESIAN_POINT('Ctrl Pts',(56.7408362584413,20.0260528668419,21.3541253385847));
#30329=CARTESIAN_POINT('Ctrl Pts',(56.7484968557265,20.0398671750079,21.3551296727905));
#30330=CARTESIAN_POINT('Ctrl Pts',(56.7524721997206,20.0471424650565,21.3556584046452));
#30331=CARTESIAN_POINT('Ctrl Pts',(56.7628611281296,20.0664402124841,21.3570604589492));
#30332=CARTESIAN_POINT('Ctrl Pts',(56.7691969863179,20.0785038023653,21.3579365093459));
#30333=CARTESIAN_POINT('Ctrl Pts',(56.7984458378421,20.1356078710089,21.3620821703625));
#30334=CARTESIAN_POINT('Ctrl Pts',(56.8197637408343,20.1814400748867,21.365406704984));
#30335=CARTESIAN_POINT('Ctrl Pts',(56.9048436615531,20.3841535851292,21.3801096309927));
#30336=CARTESIAN_POINT('Ctrl Pts',(56.9502184612566,20.5479734915179,21.3920666625641));
#30337=CARTESIAN_POINT('Ctrl Pts',(56.9843732330964,20.7850104029219,21.4086188480275));
#30338=CARTESIAN_POINT('Ctrl Pts',(56.9907118387547,20.8549957456817,21.4134042527843));
#30339=CARTESIAN_POINT('Ctrl Pts',(56.9937294037265,20.9353857572704,21.4186851829452));
#30340=CARTESIAN_POINT('Ctrl Pts',(56.994034192838,20.9455979405845,21.4193520264535));
#30341=CARTESIAN_POINT('Ctrl Pts',(56.9943767550672,20.9610583036605,21.4203550522592));
#30342=CARTESIAN_POINT('Ctrl Pts',(56.994472294889,20.9663048472962,21.4206942978672));
#30343=CARTESIAN_POINT('Ctrl Pts',(56.9946067502484,20.9757317128183,21.4213017325349));
#30344=CARTESIAN_POINT('Ctrl Pts',(56.9946532289398,20.9799118152751,21.4215703322063));
#30345=CARTESIAN_POINT('Ctrl Pts',(56.99472620223,20.9890619470939,21.4221566404961));
#30346=CARTESIAN_POINT('Ctrl Pts',(56.99474726377,20.9940319312183,21.4224740443147));
#30347=CARTESIAN_POINT('Ctrl Pts',(56.994754359979,21.0082155637527,21.4233769903446));
#30348=CARTESIAN_POINT('Ctrl Pts',(56.9946951348694,21.0174292525742,21.4239600765463));
#30349=CARTESIAN_POINT('Ctrl Pts',(56.9938663718061,21.0794742271517,21.4278652099643));
#30350=CARTESIAN_POINT('Ctrl Pts',(56.9910617767251,21.1322624146185,21.4310835330584));
#30351=CARTESIAN_POINT('Ctrl Pts',(56.9700641526076,21.3578375476791,21.4446236098807));
#30352=CARTESIAN_POINT('Ctrl Pts',(56.9314432155635,21.5279536848423,21.4543625777956));
#30353=CARTESIAN_POINT('Ctrl Pts',(56.8496301055514,21.7495326483003,21.4684633052654));
#30354=CARTESIAN_POINT('Ctrl Pts',(56.8252509618901,21.8070864101332,21.4722582973101));
#30355=CARTESIAN_POINT('Ctrl Pts',(56.7917169003763,21.8769283875758,21.4770794163882));
#30356=CARTESIAN_POINT('Ctrl Pts',(56.7850678907986,21.8903850031676,21.4780184950567));
#30357=CARTESIAN_POINT('Ctrl Pts',(56.7743338627806,21.9115055111915,21.4795091565845));
#30358=CARTESIAN_POINT('Ctrl Pts',(56.7703494838012,21.9192201340762,21.4800572170207));
#30359=CARTESIAN_POINT('Ctrl Pts',(56.7628511511322,21.9335089427907,21.4810790941734));
#30360=CARTESIAN_POINT('Ctrl Pts',(56.7593504551725,21.9400899428951,21.4815524363039));
#30361=CARTESIAN_POINT('Ctrl Pts',(56.7515117324157,21.9546289122639,21.4826042289621));
#30362=CARTESIAN_POINT('Ctrl Pts',(56.74715620859,21.9625772110469,21.4831832945347));
#30363=CARTESIAN_POINT('Ctrl Pts',(56.734373421082,21.9855316321404,21.4848675933793));
#30364=CARTESIAN_POINT('Ctrl Pts',(56.7258060968734,22.0004584183694,21.4859778196608));
#30365=CARTESIAN_POINT('Ctrl Pts',(56.6405111098911,22.1447108748809,21.4968565678298));
#30366=CARTESIAN_POINT('Ctrl Pts',(56.5495998539401,22.2650544288523,21.5071694225535));
#30367=CARTESIAN_POINT('Ctrl Pts',(56.3598350097278,22.4647680912651,21.5263720659762));
#30368=CARTESIAN_POINT('Ctrl Pts',(56.2652530472732,22.5472029663485,21.5351529765438));
#30369=CARTESIAN_POINT('Ctrl Pts',(56.1509071064076,22.6293198204467,21.544474575585));
#30370=CARTESIAN_POINT('Ctrl Pts',(56.138147191481,22.6382586033366,21.5454979167646));
#30371=CARTESIAN_POINT('Ctrl Pts',(56.1200640508208,22.6506132321084,21.546923200572));
#30372=CARTESIAN_POINT('Ctrl Pts',(56.1148276929897,22.6541543874514,21.5473330198673));
#30373=CARTESIAN_POINT('Ctrl Pts',(56.1063278124381,22.659843847393,21.5479934602868));
#30374=CARTESIAN_POINT('Ctrl Pts',(56.1030747080913,22.6620075256498,21.5482450978259));
#30375=CARTESIAN_POINT('Ctrl Pts',(56.0961762140934,22.6665666192721,21.5487762975754));
#30376=CARTESIAN_POINT('Ctrl Pts',(56.0925292833072,22.6689596623734,21.5490556954033));
#30377=CARTESIAN_POINT('Ctrl Pts',(56.0834826152054,22.6748535450024,21.5497453358728));
#30378=CARTESIAN_POINT('Ctrl Pts',(56.0780736755366,22.6783402895473,21.5501546482921));
#30379=CARTESIAN_POINT('Ctrl Pts',(56.057853627364,22.6912365795538,21.5516739254081));
#30380=CARTESIAN_POINT('Ctrl Pts',(56.0429349256264,22.7004770670982,21.5527733145567));
#30381=CARTESIAN_POINT('Ctrl Pts',(56.0049592949829,22.7233109551089,21.5555229530364));
#30382=CARTESIAN_POINT('Ctrl Pts',(55.9817465824911,22.736639750144,21.5571590397498));
#30383=CARTESIAN_POINT('Ctrl Pts',(55.8049074105282,22.8335017918676,21.5693444579776));
#30384=CARTESIAN_POINT('Ctrl Pts',(55.6411540643684,22.896981199066,21.5791308292728));
#30385=CARTESIAN_POINT('Ctrl Pts',(55.4447679317786,22.9447234839942,21.5911137334633));
#30386=CARTESIAN_POINT('Ctrl Pts',(55.4182001129528,22.9506092706598,21.5927380726587));
#30387=CARTESIAN_POINT('Ctrl Pts',(55.3425947421727,22.9657431390859,21.5973810647784));
#30388=CARTESIAN_POINT('Ctrl Pts',(55.293321824915,22.9736967658627,21.6004316912233));
#30389=CARTESIAN_POINT('Ctrl Pts',(55.2297754113078,22.9815223062263,21.6044215584806));
#30390=CARTESIAN_POINT('Ctrl Pts',(55.2157276950928,22.9831008383366,21.6053069753338));
#30391=CARTESIAN_POINT('Ctrl Pts',(55.193304867483,22.985379409242,21.6067261868673));
#30392=CARTESIAN_POINT('Ctrl Pts',(55.1849398880045,22.9861760759709,21.6072569419339));
#30393=CARTESIAN_POINT('Ctrl Pts',(55.1725306376143,22.9872788402075,21.6080463271743));
#30394=CARTESIAN_POINT('Ctrl Pts',(55.1684899938156,22.9876255007255,21.6083036807173));
#30395=CARTESIAN_POINT('Ctrl Pts',(55.1644483516286,22.9879598341382,21.6085614209934));
#30396=CARTESIAN_POINT('Origin',(55.,21.,6.22095488139522));
#30397=CARTESIAN_POINT('',(55.1644483539992,22.9879598339421,22.5673314474745));
#30398=CARTESIAN_POINT('',(55.1644481205599,22.9879598532527,22.4107149109706));
#30399=CARTESIAN_POINT('',(55.1644483516311,22.987959834138,6.22095488139522));
#30400=CARTESIAN_POINT('Ctrl Pts',(55.1644483539992,22.9879598339421,22.5673314474745));
#30401=CARTESIAN_POINT('Ctrl Pts',(55.186432793039,22.986141233409,22.5658143404452));
#30402=CARTESIAN_POINT('Ctrl Pts',(55.2083957798684,22.9839572318376,22.5643048457936));
#30403=CARTESIAN_POINT('Ctrl Pts',(55.256762560822,22.9783348456478,22.5609999925179));
#30404=CARTESIAN_POINT('Ctrl Pts',(55.2831340326463,22.9747331557386,22.5592108152993));
#30405=CARTESIAN_POINT('Ctrl Pts',(55.3266898114089,22.9678939729726,22.5562851459592));
#30406=CARTESIAN_POINT('Ctrl Pts',(55.3439171797484,22.9649564741999,22.5551356491862));
#30407=CARTESIAN_POINT('Ctrl Pts',(55.3674242420906,22.9606295627408,22.5535796769631));
#30408=CARTESIAN_POINT('Ctrl Pts',(55.3737385194787,22.9594357294347,22.5531629670468));
#30409=CARTESIAN_POINT('Ctrl Pts',(55.3843280287401,22.9573805317714,22.552466327442));
#30410=CARTESIAN_POINT('Ctrl Pts',(55.3886063608675,22.9565356314759,22.5521854817854));
#30411=CARTESIAN_POINT('Ctrl Pts',(55.3967153781305,22.9549065858725,22.5516543737523));
#30412=CARTESIAN_POINT('Ctrl Pts',(55.4005465732233,22.9541251991764,22.5514039524426));
#30413=CARTESIAN_POINT('Ctrl Pts',(55.4105778031784,22.952048551499,22.5507495425099));
#30414=CARTESIAN_POINT('Ctrl Pts',(55.4167740706285,22.9507350041827,22.5503465867116));
#30415=CARTESIAN_POINT('Ctrl Pts',(55.4382556611008,22.9460740938313,22.5489536808659));
#30416=CARTESIAN_POINT('Ctrl Pts',(55.4535082362513,22.9425763095891,22.5479718670198));
#30417=CARTESIAN_POINT('Ctrl Pts',(55.5895301826335,22.9096937250625,22.5392676660209));
#30418=CARTESIAN_POINT('Ctrl Pts',(55.7073653737135,22.8692562263404,22.5320814118752));
#30419=CARTESIAN_POINT('Ctrl Pts',(55.9150440257904,22.7755113217992,22.5188622893732));
#30420=CARTESIAN_POINT('Ctrl Pts',(56.0059423165852,22.7256372722638,22.5128573205838));
#30421=CARTESIAN_POINT('Ctrl Pts',(56.1220667603981,22.6496175422141,22.5045152693617));
#30422=CARTESIAN_POINT('Ctrl Pts',(56.1510606292004,22.6295186605663,22.5023725840844));
#30423=CARTESIAN_POINT('Ctrl Pts',(56.1998664097338,22.5937332342405,22.4986489231873));
#30424=CARTESIAN_POINT('Ctrl Pts',(56.2199415630545,22.5784193094521,22.497081750701));
#30425=CARTESIAN_POINT('Ctrl Pts',(56.2479963034211,22.5561633572653,22.4948376907151));
#30426=CARTESIAN_POINT('Ctrl Pts',(56.2562202119917,22.5495321680906,22.4941731170456));
#30427=CARTESIAN_POINT('Ctrl Pts',(56.2703077222298,22.537987117644,22.4930227805335));
#30428=CARTESIAN_POINT('Ctrl Pts',(56.276196499834,22.533104228143,22.4925382733645));
#30429=CARTESIAN_POINT('Ctrl Pts',(56.287418532211,22.5236896218897,22.4916078660918));
#30430=CARTESIAN_POINT('Ctrl Pts',(56.2927563201373,22.5191634657357,22.4911621975115));
#30431=CARTESIAN_POINT('Ctrl Pts',(56.3052296449744,22.5084734153937,22.4901133453566));
#30432=CARTESIAN_POINT('Ctrl Pts',(56.3123454654043,22.5022868718878,22.489509232005));
#30433=CARTESIAN_POINT('Ctrl Pts',(56.3367487826879,22.4807647644597,22.4874172586597));
#30434=CARTESIAN_POINT('Ctrl Pts',(56.3538129422668,22.4651798656036,22.4859190267315));
#30435=CARTESIAN_POINT('Ctrl Pts',(56.4868386154005,22.3393778084727,22.4739499211205));
#30436=CARTESIAN_POINT('Ctrl Pts',(56.5894079160468,22.2158885896307,22.4628709241762));
#30437=CARTESIAN_POINT('Ctrl Pts',(56.7322939258679,21.9944456003329,22.4444902770158));
#30438=CARTESIAN_POINT('Ctrl Pts',(56.781609773601,21.9031251905772,22.4372784732087));
#30439=CARTESIAN_POINT('Ctrl Pts',(56.8306760746122,21.7924372089665,22.4292445757396));
#30440=CARTESIAN_POINT('Ctrl Pts',(56.8375335377547,21.7764033538807,22.4280975714684));
#30441=CARTESIAN_POINT('Ctrl Pts',(56.8466273112094,21.7543449879316,22.4265443965355));
#30442=CARTESIAN_POINT('Ctrl Pts',(56.8490458531047,21.7483971026065,22.4261280379886));
#30443=CARTESIAN_POINT('Ctrl Pts',(56.8530583666099,21.7383909940816,22.4254318207307));
#30444=CARTESIAN_POINT('Ctrl Pts',(56.8546678119975,21.7343390759437,22.4251510484128));
#30445=CARTESIAN_POINT('Ctrl Pts',(56.8576957873248,21.7266424290724,22.4246199557235));
#30446=CARTESIAN_POINT('Ctrl Pts',(56.8591168997318,21.7229987633105,22.424369477113));
#30447=CARTESIAN_POINT('Ctrl Pts',(56.8628132478653,21.7134385381294,22.4237146897338));
#30448=CARTESIAN_POINT('Ctrl Pts',(56.8650710359686,21.707515213637,22.4233114161112));
#30449=CARTESIAN_POINT('Ctrl Pts',(56.8728146583173,21.6869050946895,22.4219162867283));
#30450=CARTESIAN_POINT('Ctrl Pts',(56.8781557215798,21.6721640238599,22.4209326017128));
#30451=CARTESIAN_POINT('Ctrl Pts',(56.9238985156207,21.5411120730095,22.4122993674739));
#30452=CARTESIAN_POINT('Ctrl Pts',(56.9536298756021,21.4213389799999,22.4051756549556));
#30453=CARTESIAN_POINT('Ctrl Pts',(56.9949659144926,21.1492202161439,22.3892073187235));
#30454=CARTESIAN_POINT('Ctrl Pts',(57.0005342842458,20.9967693489157,22.3803749343104));
#30455=CARTESIAN_POINT('Ctrl Pts',(56.9873879101523,20.8279043227772,22.3698632487092));
#30456=CARTESIAN_POINT('Ctrl Pts',(56.9858185384235,20.8106528839217,22.3687815087444));
#30457=CARTESIAN_POINT('Ctrl Pts',(56.9830835419132,20.7843850042937,22.3671215044268));
#30458=CARTESIAN_POINT('Ctrl Pts',(56.9820806023704,20.7753521825726,22.366548343963));
#30459=CARTESIAN_POINT('Ctrl Pts',(56.9801423910683,20.7589205802785,22.3655013317745));
#30460=CARTESIAN_POINT('Ctrl Pts',(56.9792272836039,20.7515195523053,22.3650281228777));
#30461=CARTESIAN_POINT('Ctrl Pts',(56.9771589418926,20.7355284535045,22.3640020982716));
#30462=CARTESIAN_POINT('Ctrl Pts',(56.975991183469,20.7269404472431,22.3634488334084));
#30463=CARTESIAN_POINT('Ctrl Pts',(56.972659003923,20.703576258734,22.3619374071075));
#30464=CARTESIAN_POINT('Ctrl Pts',(56.970384590497,20.6888165725106,22.360975795742));
#30465=CARTESIAN_POINT('Ctrl Pts',(56.9579208864861,20.6135582510611,22.3560367769279));
#30466=CARTESIAN_POINT('Ctrl Pts',(56.9451111442671,20.5535330703515,22.3519773049891));
#30467=CARTESIAN_POINT('Ctrl Pts',(56.8852156597996,20.3250407551035,22.3360510705103));
#30468=CARTESIAN_POINT('Ctrl Pts',(56.8188212607718,20.1624539020487,22.323624433701));
#30469=CARTESIAN_POINT('Ctrl Pts',(56.7058461536601,19.9646643552094,22.3080240171846));
#30470=CARTESIAN_POINT('Ctrl Pts',(56.6777623502385,19.9197474425884,22.3044526377261));
#30471=CARTESIAN_POINT('Ctrl Pts',(56.6427262691075,19.8683803734763,22.3003794866864));
#30472=CARTESIAN_POINT('Ctrl Pts',(56.6374780034222,19.8607992404511,22.2997786478299));
#30473=CARTESIAN_POINT('Ctrl Pts',(56.6293187819763,19.849186117349,22.2988590682349));
#30474=CARTESIAN_POINT('Ctrl Pts',(56.6264450841888,19.8451282862459,22.2985379051383));
#30475=CARTESIAN_POINT('Ctrl Pts',(56.6211267593407,19.8376777217778,22.2979485680108));
#30476=CARTESIAN_POINT('Ctrl Pts',(56.618686648255,19.8342819450345,22.2976801043787));
#30477=CARTESIAN_POINT('Ctrl Pts',(56.613159982681,19.8266415831078,22.2970763719475));
#30478=CARTESIAN_POINT('Ctrl Pts',(56.6100673510037,19.8224014984017,22.2967415274334));
#30479=CARTESIAN_POINT('Ctrl Pts',(56.6009057007454,19.809944180552,22.2957581946121));
#30480=CARTESIAN_POINT('Ctrl Pts',(56.5947901440049,19.8017611577271,22.295112820871));
#30481=CARTESIAN_POINT('Ctrl Pts',(56.5462118519476,19.7377909432844,22.2900689454476));
#30482=CARTESIAN_POINT('Ctrl Pts',(56.5008926521083,19.6842240660056,22.285852462382));
#30483=CARTESIAN_POINT('Ctrl Pts',(56.3368445128139,19.5098553343201,22.2717206005191));
#30484=CARTESIAN_POINT('Ctrl Pts',(56.2056289350415,19.4018305251734,22.2621769037627));
#30485=CARTESIAN_POINT('Ctrl Pts',(56.0194893756974,19.2847062601307,22.2489321614414));
#30486=CARTESIAN_POINT('Ctrl Pts',(55.9756268141322,19.2593843441645,22.2458353891472));
#30487=CARTESIAN_POINT('Ctrl Pts',(55.9187896486327,19.2293958308093,22.2418279658114));
#30488=CARTESIAN_POINT('Ctrl Pts',(55.9066634231176,19.2231558974031,22.2409733294865));
#30489=CARTESIAN_POINT('Ctrl Pts',(55.8870604384689,19.2133214776944,22.2395918593199));
#30490=CARTESIAN_POINT('Ctrl Pts',(55.8796234395096,19.2096483683755,22.239067783237));
#30491=CARTESIAN_POINT('Ctrl Pts',(55.8654118127666,19.2027392170357,22.2380662575772));
#30492=CARTESIAN_POINT('Ctrl Pts',(55.8586413864248,19.1994948223767,22.2375891088872));
#30493=CARTESIAN_POINT('Ctrl Pts',(55.843124660319,19.1921666161996,22.2364954317892));
#30494=CARTESIAN_POINT('Ctrl Pts',(55.8343667633765,19.1881079405279,22.235878048766));
#30495=CARTESIAN_POINT('Ctrl Pts',(55.8114129816927,19.1776721695777,22.2342595225954));
#30496=CARTESIAN_POINT('Ctrl Pts',(55.7971715403123,19.1713974568206,22.2332549115109));
#30497=CARTESIAN_POINT('Ctrl Pts',(55.6730060746916,19.1184168796701,22.2244907514905));
#30498=CARTESIAN_POINT('Ctrl Pts',(55.5591856972935,19.081512438334,22.2163982511514));
#30499=CARTESIAN_POINT('Ctrl Pts',(55.3263066041796,19.0284986624644,22.1998502090009));
#30500=CARTESIAN_POINT('Ctrl Pts',(55.2077007994765,19.0125004598778,22.1914300298946));
#30501=CARTESIAN_POINT('Ctrl Pts',(55.0415072454109,19.0051301587212,22.1800807204054));
#30502=CARTESIAN_POINT('Ctrl Pts',(54.9945756370025,19.0047055589642,22.1769277564013));
#30503=CARTESIAN_POINT('Ctrl Pts',(54.9387306776766,19.0061711263204,22.173270215637));
#30504=CARTESIAN_POINT('Ctrl Pts',(54.9297940400536,19.0064657921702,22.1726877995586));
#30505=CARTESIAN_POINT('Ctrl Pts',(54.9159509820275,19.0070154399804,22.1717904051859));
#30506=CARTESIAN_POINT('Ctrl Pts',(54.9110431499649,19.0072284691933,22.1714731802757));
#30507=CARTESIAN_POINT('Ctrl Pts',(54.9019543107122,19.0076566231179,22.1708874981278));
#30508=CARTESIAN_POINT('Ctrl Pts',(54.8977732226408,19.0078667777706,22.170618778328));
#30509=CARTESIAN_POINT('Ctrl Pts',(54.8882755867065,19.008374138957,22.1700099471002));
#30510=CARTESIAN_POINT('Ctrl Pts',(54.8829595550001,19.0086794706226,22.1696702922901));
#30511=CARTESIAN_POINT('Ctrl Pts',(54.869152377627,19.0095279819264,22.1687908821062));
#30512=CARTESIAN_POINT('Ctrl Pts',(54.8606632672851,19.0101042147853,22.1682529101566));
#30513=CARTESIAN_POINT('Ctrl Pts',(54.8047780828098,19.0142570364843,22.1647277380575));
#30514=CARTESIAN_POINT('Ctrl Pts',(54.757514940367,19.0194726668748,22.1618239958289));
#30515=CARTESIAN_POINT('Ctrl Pts',(54.5389940172617,19.0515285284883,22.1485745228542));
#30516=CARTESIAN_POINT('Ctrl Pts',(54.3715119980335,19.0989268251903,22.1388622988844));
#30517=CARTESIAN_POINT('Ctrl Pts',(54.1495507206926,19.1943361415193,22.1244817679848));
#30518=CARTESIAN_POINT('Ctrl Pts',(54.0882765217809,19.2244874683744,22.1203444552746));
#30519=CARTESIAN_POINT('Ctrl Pts',(54.0156348040346,19.2649854395657,22.1151673053542));
#30520=CARTESIAN_POINT('Ctrl Pts',(54.0026797402316,19.2723997440683,22.1142331184199));
#30521=CARTESIAN_POINT('Ctrl Pts',(53.9824130131017,19.2843025142795,22.1127538640252));
#30522=CARTESIAN_POINT('Ctrl Pts',(53.9750448407289,19.2886940495118,22.1122123043797));
#30523=CARTESIAN_POINT('Ctrl Pts',(53.9613185619704,19.2969955539218,22.1111962508325));
#30524=CARTESIAN_POINT('Ctrl Pts',(53.9549536127928,19.3008939647057,22.1107221854369));
#30525=CARTESIAN_POINT('Ctrl Pts',(53.9407901968371,19.3096784790632,22.1096606739608));
#30526=CARTESIAN_POINT('Ctrl Pts',(53.9330034012854,19.3145829878334,22.1090725566859));
#30527=CARTESIAN_POINT('Ctrl Pts',(53.9133895010384,19.3271271931885,22.107579546365));
#30528=CARTESIAN_POINT('Ctrl Pts',(53.9016089855882,19.3348384562449,22.1066720103993));
#30529=CARTESIAN_POINT('Ctrl Pts',(53.8326951372653,19.3809974282371,22.1012980722475));
#30530=CARTESIAN_POINT('Ctrl Pts',(53.7775082899416,19.4222541037242,22.096726233571));
#30531=CARTESIAN_POINT('Ctrl Pts',(53.5960062618436,19.5731895882687,22.0807350084138));
#30532=CARTESIAN_POINT('Ctrl Pts',(53.481413737206,19.6958252626058,22.0688614487301));
#30533=CARTESIAN_POINT('Ctrl Pts',(53.3629398511127,19.8596977920986,22.0550185152881));
#30534=CARTESIAN_POINT('Ctrl Pts',(53.3431633339902,19.8886280507945,22.0526443634274));
#30535=CARTESIAN_POINT('Ctrl Pts',(53.3163679968268,19.9301321941513,22.049350299199));
#30536=CARTESIAN_POINT('Ctrl Pts',(53.3087081990368,19.9422826868989,22.0483990748917));
#30537=CARTESIAN_POINT('Ctrl Pts',(53.295471169318,19.9637916850545,22.0467395440868));
#30538=CARTESIAN_POINT('Ctrl Pts',(53.2898381929057,19.9731149952555,22.0460281107478));
#30539=CARTESIAN_POINT('Ctrl Pts',(53.281569917422,19.9870568247403,22.0449764997441));
#30540=CARTESIAN_POINT('Ctrl Pts',(53.278876367199,19.9916403086119,22.0446327254326));
#30541=CARTESIAN_POINT('Ctrl Pts',(53.274094843857,19.9998517734236,22.044020397084));
#30542=CARTESIAN_POINT('Ctrl Pts',(53.2719999411686,20.0034755994611,22.0437514032716));
#30543=CARTESIAN_POINT('Ctrl Pts',(53.2674681049062,20.0113721688824,22.0431679361548));
#30544=CARTESIAN_POINT('Ctrl Pts',(53.2650355666977,20.0156473333128,22.0428537442523));
#30545=CARTESIAN_POINT('Ctrl Pts',(53.2583311442625,20.0275323570095,22.0419848522127));
#30546=CARTESIAN_POINT('Ctrl Pts',(53.2540932855144,20.0351614276703,22.0414322752435));
#30547=CARTESIAN_POINT('Ctrl Pts',(53.231723197053,20.0760625074127,22.0384959727651));
#30548=CARTESIAN_POINT('Ctrl Pts',(53.2144903982374,20.1098206706753,22.0361644874006));
#30549=CARTESIAN_POINT('Ctrl Pts',(53.1206209176822,20.3074159671148,22.0229236652895));
#30550=CARTESIAN_POINT('Ctrl Pts',(53.0655852170667,20.4805861575663,22.0128265340167));
#30551=CARTESIAN_POINT('Ctrl Pts',(53.0266136607683,20.7050787864988,21.9992874647207));
#30552=CARTESIAN_POINT('Ctrl Pts',(53.0202191052899,20.7516065246491,21.9964632277785));
#30553=CARTESIAN_POINT('Ctrl Pts',(53.0123044070312,20.8294848118171,21.9916745650311));
#30554=CARTESIAN_POINT('Ctrl Pts',(53.0098715395249,20.8607242195519,21.9897374552123));
#30555=CARTESIAN_POINT('Ctrl Pts',(53.0075532874913,20.9034819731368,21.9870584401019));
#30556=CARTESIAN_POINT('Ctrl Pts',(53.007030306562,20.9149622207173,21.9863364295341));
#30557=CARTESIAN_POINT('Ctrl Pts',(53.0063178076254,20.934271758601,21.9851172066318));
#30558=CARTESIAN_POINT('Ctrl Pts',(53.0060751404237,20.9420988995984,21.9846216642222));
#30559=CARTESIAN_POINT('Ctrl Pts',(53.0056869306216,20.9575591320441,21.9836401542223));
#30560=CARTESIAN_POINT('Ctrl Pts',(53.005539108197,20.9651920358087,21.983154266534));
#30561=CARTESIAN_POINT('Ctrl Pts',(53.005309941177,20.9820125375752,21.9820805713036));
#30562=CARTESIAN_POINT('Ctrl Pts',(53.0052482514913,20.9912001865167,21.9814921593815));
#30563=CARTESIAN_POINT('Ctrl Pts',(53.0052545405657,21.0235489877355,21.9794133965494));
#30564=CARTESIAN_POINT('Ctrl Pts',(53.0056624310092,21.0467074799556,21.9779125082573));
#30565=CARTESIAN_POINT('Ctrl Pts',(53.0099793257329,21.169907119395,21.9698572499644));
#30566=CARTESIAN_POINT('Ctrl Pts',(53.0210120454064,21.2695405343755,21.9630836386395));
#30567=CARTESIAN_POINT('Ctrl Pts',(53.0595322021014,21.4748061766944,21.9486597695539));
#30568=CARTESIAN_POINT('Ctrl Pts',(53.088299572222,21.5798765704903,21.9410071814636));
#30569=CARTESIAN_POINT('Ctrl Pts',(53.1322777321936,21.7007392469975,21.9321353382661));
#30570=CARTESIAN_POINT('Ctrl Pts',(53.13934689952,21.7192996871774,21.9307713489112));
#30571=CARTESIAN_POINT('Ctrl Pts',(53.1641047985049,21.7814940467824,21.9262016597919));
#30572=CARTESIAN_POINT('Ctrl Pts',(53.1830621659017,21.8246101130648,21.9230350417638));
#30573=CARTESIAN_POINT('Ctrl Pts',(53.2072178089171,21.8746608424881,21.9193930671669));
#30574=CARTESIAN_POINT('Ctrl Pts',(53.2109550429793,21.8822798433186,21.9188396239907));
#30575=CARTESIAN_POINT('Ctrl Pts',(53.2171132348228,21.8946343528937,21.9179440361739));
#30576=CARTESIAN_POINT('Ctrl Pts',(53.2195046628134,21.8993843442424,21.9176001518224));
#30577=CARTESIAN_POINT('Ctrl Pts',(53.2238123524297,21.9078560044096,21.9169877053446));
#30578=CARTESIAN_POINT('Ctrl Pts',(53.2257213543959,21.9115812486799,21.9167187027262));
#30579=CARTESIAN_POINT('Ctrl Pts',(53.229898511729,21.9196697585728,21.916135306161));
#30580=CARTESIAN_POINT('Ctrl Pts',(53.2321710756985,21.9240306484503,21.9158211930497));
#30581=CARTESIAN_POINT('Ctrl Pts',(53.2386320346689,21.9363176907273,21.9149372322428));
#30582=CARTESIAN_POINT('Ctrl Pts',(53.2428578310199,21.9442241960658,21.9143696801352));
#30583=CARTESIAN_POINT('Ctrl Pts',(53.2697529346133,21.9937392997632,21.9108215933723));
#30584=CARTESIAN_POINT('Ctrl Pts',(53.293847455087,22.0345612616061,21.9079242214424));
#30585=CARTESIAN_POINT('Ctrl Pts',(53.3560556881346,22.131862051641,21.9009908199185));
#30586=CARTESIAN_POINT('Ctrl Pts',(53.3956521505147,22.1873220642859,21.8970142636764));
#30587=CARTESIAN_POINT('Ctrl Pts',(53.5379302761178,22.3664514415244,21.8837203187678));
#30588=CARTESIAN_POINT('Ctrl Pts',(53.6526685959417,22.4797058327579,21.8744856673388));
#30589=CARTESIAN_POINT('Ctrl Pts',(53.797978593388,22.5920752502866,21.8631639699588));
#30590=CARTESIAN_POINT('Ctrl Pts',(53.8164585148788,22.6058606879556,21.8617314956129));
#30591=CARTESIAN_POINT('Ctrl Pts',(53.8428194620852,22.6248229121148,21.8596962395714));
#30592=CARTESIAN_POINT('Ctrl Pts',(53.8505050515846,22.6302691960999,21.859103810811));
#30593=CARTESIAN_POINT('Ctrl Pts',(53.8639655317667,22.6396652693003,21.858067741994));
#30594=CARTESIAN_POINT('Ctrl Pts',(53.869723207206,22.6436395219167,21.8576250416526));
#30595=CARTESIAN_POINT('Ctrl Pts',(53.8818217826867,22.6518969666933,21.8566957223432));
#30596=CARTESIAN_POINT('Ctrl Pts',(53.8881666485841,22.6561741183351,21.8562088850777));
#30597=CARTESIAN_POINT('Ctrl Pts',(53.9033389067207,22.6662754428282,21.8550458902131));
#30598=CARTESIAN_POINT('Ctrl Pts',(53.9121882440023,22.6720660816087,21.8543684921998));
#30599=CARTESIAN_POINT('Ctrl Pts',(53.9423761163796,22.6914786925323,21.8520605289971));
#30600=CARTESIAN_POINT('Ctrl Pts',(53.9639270377739,22.7047642551455,21.8504176463531));
#30601=CARTESIAN_POINT('Ctrl Pts',(54.0162044869587,22.7356344545864,21.8464419214565));
#30602=CARTESIAN_POINT('Ctrl Pts',(54.0471568385134,22.7528177958132,21.8440955683627));
#30603=CARTESIAN_POINT('Ctrl Pts',(54.170933374695,22.8172854435037,21.8347414178948));
#30604=CARTESIAN_POINT('Ctrl Pts',(54.2669353382658,22.8580875989863,21.8275372586523));
#30605=CARTESIAN_POINT('Ctrl Pts',(54.4826811196101,22.9304507287261,21.8116734126673));
#30606=CARTESIAN_POINT('Ctrl Pts',(54.6030897518693,22.9587563664343,21.8030216820526));
#30607=CARTESIAN_POINT('Ctrl Pts',(54.7408746869787,22.977909824288,21.7938092423701));
#30608=CARTESIAN_POINT('Ctrl Pts',(54.7564237520758,22.9798848069889,21.7927795874487));
#30609=CARTESIAN_POINT('Ctrl Pts',(54.7782915916966,22.9824008463221,21.7913469835604));
#30610=CARTESIAN_POINT('Ctrl Pts',(54.7845916573608,22.9830953034037,21.7909360542432));
#30611=CARTESIAN_POINT('Ctrl Pts',(54.7947842764362,22.9841696912345,21.7902742537754));
#30612=CARTESIAN_POINT('Ctrl Pts',(54.7986747621842,22.9845682165339,21.790022358841));
#30613=CARTESIAN_POINT('Ctrl Pts',(54.8069050110589,22.9853868381767,21.7894910209665));
#30614=CARTESIAN_POINT('Ctrl Pts',(54.811245027185,22.9858041526986,21.7892117406183));
#30615=CARTESIAN_POINT('Ctrl Pts',(54.8219804263145,22.986800903384,21.788523083483));
#30616=CARTESIAN_POINT('Ctrl Pts',(54.8283773714245,22.9873636995753,21.7881146303464));
#30617=CARTESIAN_POINT('Ctrl Pts',(54.8521603123513,22.9893404070899,21.7866027453845));
#30618=CARTESIAN_POINT('Ctrl Pts',(54.8695625026795,22.9905571925582,21.7855097541409));
#30619=CARTESIAN_POINT('Ctrl Pts',(54.9794427604105,22.996792934718,21.7786794598602));
#30620=CARTESIAN_POINT('Ctrl Pts',(55.0721571717986,22.9955943612478,21.7732303855258));
#30621=CARTESIAN_POINT('Ctrl Pts',(55.1644483608155,22.9879598333782,21.7678366528264));
#30622=CARTESIAN_POINT('',(53.0052506709088,21.0016360287739,21.82180160064));
#30623=CARTESIAN_POINT('Ctrl Pts',(55.1644483516286,22.9879598341382,21.6085614209934));
#30624=CARTESIAN_POINT('Ctrl Pts',(55.1617779762643,22.9881807333834,21.6087317139713));
#30625=CARTESIAN_POINT('Ctrl Pts',(55.1591071650582,22.9883962512936,21.6089021757682));
#30626=CARTESIAN_POINT('Ctrl Pts',(55.1473710419759,22.9893194864748,21.6096518482129));
#30627=CARTESIAN_POINT('Ctrl Pts',(55.1383015064477,22.9899705857306,21.6102328283703));
#30628=CARTESIAN_POINT('Ctrl Pts',(55.1119122403895,22.9916837878414,21.6119282176947));
#30629=CARTESIAN_POINT('Ctrl Pts',(55.0945830631652,22.9925819112099,21.6130477215589));
#30630=CARTESIAN_POINT('Ctrl Pts',(54.9313800541841,22.9989065380806,21.6236519036185));
#30631=CARTESIAN_POINT('Ctrl Pts',(54.7853644296207,22.9885300440164,21.6336466817665));
#30632=CARTESIAN_POINT('Ctrl Pts',(54.5143004666532,22.9390527483187,21.6528438923881));
#30633=CARTESIAN_POINT('Ctrl Pts',(54.389346787241,22.9034016554108,21.6619515336031));
#30634=CARTESIAN_POINT('Ctrl Pts',(54.2544282853142,22.8502396124984,21.6715509014633));
#30635=CARTESIAN_POINT('Ctrl Pts',(54.2401932448406,22.8444396262404,21.6725603604724));
#30636=CARTESIAN_POINT('Ctrl Pts',(54.2202322199938,22.8360362989407,21.6739697043924));
#30637=CARTESIAN_POINT('Ctrl Pts',(54.2144497503709,22.833569712244,21.6743772386554));
#30638=CARTESIAN_POINT('Ctrl Pts',(54.2047423042156,22.8293745245944,21.6750600375736));
#30639=CARTESIAN_POINT('Ctrl Pts',(54.2008111009197,22.82766054252,21.6753361725057));
#30640=CARTESIAN_POINT('Ctrl Pts',(54.1933092774923,22.8243609575302,21.6758623518518));
#30641=CARTESIAN_POINT('Ctrl Pts',(54.1897377540319,22.8227775285375,21.6761125300098));
#30642=CARTESIAN_POINT('Ctrl Pts',(54.1807435781754,22.818758316895,21.6767417797376));
#30643=CARTESIAN_POINT('Ctrl Pts',(54.1753270735485,22.816308747576,21.677120016706));
#30644=CARTESIAN_POINT('Ctrl Pts',(54.1556958856566,22.807324784326,21.6784885678753));
#30645=CARTESIAN_POINT('Ctrl Pts',(54.1415468114881,22.8006472371079,21.679470542339));
#30646=CARTESIAN_POINT('Ctrl Pts',(54.1066583769887,22.7836771789033,21.6818844714766));
#30647=CARTESIAN_POINT('Ctrl Pts',(54.0860164315846,22.7731885591763,21.6833061211108));
#30648=CARTESIAN_POINT('Ctrl Pts',(54.0013731152529,22.728308504735,21.689127423286));
#30649=CARTESIAN_POINT('Ctrl Pts',(53.9390874315507,22.6907903806595,21.6933925329391));
#30650=CARTESIAN_POINT('Ctrl Pts',(53.7369129211323,22.553428459473,21.7076252250684));
#30651=CARTESIAN_POINT('Ctrl Pts',(53.607919748892,22.4389704164121,21.7174451561569));
#30652=CARTESIAN_POINT('Ctrl Pts',(53.4804501043683,22.292478005863,21.7294275417452));
#30653=CARTESIAN_POINT('Ctrl Pts',(53.4660047413569,22.2752998722027,21.7308234141959));
#30654=CARTESIAN_POINT('Ctrl Pts',(53.4455662760572,22.2501450886237,21.7328563263371));
#30655=CARTESIAN_POINT('Ctrl Pts',(53.4393380030701,22.2423610869161,21.7334838947135));
#30656=CARTESIAN_POINT('Ctrl Pts',(53.42847953215,22.2285798231934,21.7345925226408));
#30657=CARTESIAN_POINT('Ctrl Pts',(53.4238246312341,22.2226022113269,21.7350725873166));
#30658=CARTESIAN_POINT('Ctrl Pts',(53.4142820003185,22.2102029227855,21.73606681098));
#30659=CARTESIAN_POINT('Ctrl Pts',(53.4093989683717,22.2037778216362,21.7365811427809));
#30660=CARTESIAN_POINT('Ctrl Pts',(53.3969790068595,22.1872281033464,21.7379038696963));
#30661=CARTESIAN_POINT('Ctrl Pts',(53.3894990325579,22.1770613813856,21.7387144613357));
#30662=CARTESIAN_POINT('Ctrl Pts',(53.3584890218798,22.1340638335243,21.7421349462034));
#30663=CARTESIAN_POINT('Ctrl Pts',(53.3358639131521,22.1005951851126,21.7447790126629));
#30664=CARTESIAN_POINT('Ctrl Pts',(53.2638327535743,21.9867377216486,21.7537201551066));
#30665=CARTESIAN_POINT('Ctrl Pts',(53.2191196504964,21.9035426213686,21.7601743499628));
#30666=CARTESIAN_POINT('Ctrl Pts',(53.1476539198563,21.7444802559619,21.7722784450761));
#30667=CARTESIAN_POINT('Ctrl Pts',(53.1192701499859,21.6695461037394,21.7778895909982));
#30668=CARTESIAN_POINT('Ctrl Pts',(53.0908231470972,21.5781999293943,21.7845184947134));
#30669=CARTESIAN_POINT('Ctrl Pts',(53.0863552031951,21.5632362026823,21.7855976629879));
#30670=CARTESIAN_POINT('Ctrl Pts',(53.0784285025961,21.5355048681868,21.7875836493999));
#30671=CARTESIAN_POINT('Ctrl Pts',(53.0749201365852,21.5227523452241,21.7884915170118));
#30672=CARTESIAN_POINT('Ctrl Pts',(53.0588699559472,21.4620577684243,21.7927842349298));
#30673=CARTESIAN_POINT('Ctrl Pts',(53.0479895199753,21.4136897705801,21.7961222885044));
#30674=CARTESIAN_POINT('Ctrl Pts',(53.0373468883347,21.3565029711685,21.799935196117));
#30675=CARTESIAN_POINT('Ctrl Pts',(53.0358272605837,21.3480331324557,21.800496499402));
#30676=CARTESIAN_POINT('Ctrl Pts',(53.0334512578881,21.3342787182565,21.801402185719));
#30677=CARTESIAN_POINT('Ctrl Pts',(53.0325612827175,21.3290001701196,21.8017483727361));
#30678=CARTESIAN_POINT('Ctrl Pts',(53.0310129992354,21.319586119525,21.8023632297214));
#30679=CARTESIAN_POINT('Ctrl Pts',(53.0303464547553,21.3154520720876,21.8026323555845));
#30680=CARTESIAN_POINT('Ctrl Pts',(53.0290754110196,21.3074076804958,21.8031543239326));
#30681=CARTESIAN_POINT('Ctrl Pts',(53.0284695309719,21.3034976570394,21.8034072467288));
#30682=CARTESIAN_POINT('Ctrl Pts',(53.0271487012991,21.2948028500444,21.8039679891812));
#30683=CARTESIAN_POINT('Ctrl Pts',(53.0264395136366,21.2900171977745,21.8042754892173));
#30684=CARTESIAN_POINT('Ctrl Pts',(53.0247126304538,21.2780643332706,21.8050407911548));
#30685=CARTESIAN_POINT('Ctrl Pts',(53.0237165164829,21.2708940054424,21.8054974412499));
#30686=CARTESIAN_POINT('Ctrl Pts',(53.0111727514092,21.1768465231527,21.8114568477455));
#30687=CARTESIAN_POINT('Ctrl Pts',(53.0053225665444,21.0892957162249,21.8166699893501));
#30688=CARTESIAN_POINT('Ctrl Pts',(53.0052506709088,21.0016360287739,21.82180160064));
#30689=CARTESIAN_POINT('Ctrl Pts',(53.0052506727303,21.0016382481781,21.8218014707158));
#30690=CARTESIAN_POINT('Ctrl Pts',(53.0050980911781,20.8158532415753,21.8326773561794));
#30691=CARTESIAN_POINT('Ctrl Pts',(53.0308982462845,20.6309633578212,21.8431993114979));
#30692=CARTESIAN_POINT('Ctrl Pts',(53.0885150928867,20.429183853493,21.8561264103871));
#30693=CARTESIAN_POINT('Ctrl Pts',(53.0955337411309,20.4061870542386,21.8576200319245));
#30694=CARTESIAN_POINT('Ctrl Pts',(53.1061686196015,20.3734718070132,21.8597765417519));
#30695=CARTESIAN_POINT('Ctrl Pts',(53.1094477852777,20.3636453890307,21.8604284050087));
#30696=CARTESIAN_POINT('Ctrl Pts',(53.115269011805,20.3466435840098,21.8615636445917));
#30697=CARTESIAN_POINT('Ctrl Pts',(53.1177759042922,20.3394563185554,21.8620458524304));
#30698=CARTESIAN_POINT('Ctrl Pts',(53.1226808407823,20.3256485208664,21.8629767601612));
#30699=CARTESIAN_POINT('Ctrl Pts',(53.1250729275634,20.3190259814591,21.863425256261));
#30700=CARTESIAN_POINT('Ctrl Pts',(53.1308111808933,20.3033989682237,21.8644883886614));
#30701=CARTESIAN_POINT('Ctrl Pts',(53.1341874034381,20.2944057907627,21.865104019444));
#30702=CARTESIAN_POINT('Ctrl Pts',(53.146283442061,20.262879761762,21.8672757824595));
#30703=CARTESIAN_POINT('Ctrl Pts',(53.1553472739557,20.2404820225856,21.8688433631035));
#30704=CARTESIAN_POINT('Ctrl Pts',(53.2148410381555,20.1008174599471,21.8787782206856));
#30705=CARTESIAN_POINT('Ctrl Pts',(53.2760150411987,19.9884727899826,21.8875142622304));
#30706=CARTESIAN_POINT('Ctrl Pts',(53.3880049215924,19.8228285322391,21.9014301816578));
#30707=CARTESIAN_POINT('Ctrl Pts',(53.4317528180296,19.7651470709507,21.9064949832486));
#30708=CARTESIAN_POINT('Ctrl Pts',(53.5107039583615,19.6720320943453,21.9149388884185));
#30709=CARTESIAN_POINT('Ctrl Pts',(53.5442803056887,19.6353087153633,21.9183467338849));
#30710=CARTESIAN_POINT('Ctrl Pts',(53.598262208756,19.5805294849428,21.9235079226599));
#30711=CARTESIAN_POINT('Ctrl Pts',(53.6177222288231,19.5615724841883,21.9253094660529));
#30712=CARTESIAN_POINT('Ctrl Pts',(53.6430229066554,19.5379136217837,21.9275710145567));
#30713=CARTESIAN_POINT('Ctrl Pts',(53.6485100427259,19.5328400534064,21.9280567933379));
#30714=CARTESIAN_POINT('Ctrl Pts',(53.6569492292224,19.5251244523029,21.9287965860874));
#30715=CARTESIAN_POINT('Ctrl Pts',(53.6598807787989,19.5224602449637,21.9290522309805));
#30716=CARTESIAN_POINT('Ctrl Pts',(53.6659258925465,19.5169992062352,21.9295766097371));
#30717=CARTESIAN_POINT('Ctrl Pts',(53.6690402845746,19.5142034745889,21.9298452515595));
#30718=CARTESIAN_POINT('Ctrl Pts',(53.6761364345678,19.5078736094059,21.9304539477382));
#30719=CARTESIAN_POINT('Ctrl Pts',(53.6801235509547,19.504345606022,21.9307935454502));
#30720=CARTESIAN_POINT('Ctrl Pts',(53.6905191270377,19.4952210149287,21.9316728824456));
#30721=CARTESIAN_POINT('Ctrl Pts',(53.6969494317181,19.4896493211342,21.9322108380987));
#30722=CARTESIAN_POINT('Ctrl Pts',(53.7395565926629,19.4532059686567,21.935737745149));
#30723=CARTESIAN_POINT('Ctrl Pts',(53.7767951369329,19.4235926826868,21.9386431368235));
#30724=CARTESIAN_POINT('Ctrl Pts',(53.8301838638295,19.384168564838,21.9426244566304));
#30725=CARTESIAN_POINT('Ctrl Pts',(53.845465247139,19.3732146556651,21.9437439471052));
#30726=CARTESIAN_POINT('Ctrl Pts',(53.9898840980947,19.2727533511981,21.9541602202661));
#30727=CARTESIAN_POINT('Ctrl Pts',(54.1290172833517,19.1985817961632,21.9630325544292));
#30728=CARTESIAN_POINT('Ctrl Pts',(54.3367626858106,19.1175868952596,21.9763242863846));
#30729=CARTESIAN_POINT('Ctrl Pts',(54.3992488503363,19.0967240006669,21.9803203322845));
#30730=CARTESIAN_POINT('Ctrl Pts',(54.476875634755,19.0750099388456,21.9853390561586));
#30731=CARTESIAN_POINT('Ctrl Pts',(54.4911470622699,19.0711883175691,21.9862638429036));
#30732=CARTESIAN_POINT('Ctrl Pts',(54.5137354128136,19.0654077191829,21.9877314480522));
#30733=CARTESIAN_POINT('Ctrl Pts',(54.5220249119441,19.0633429954504,21.9882708506131));
#30734=CARTESIAN_POINT('Ctrl Pts',(54.5375822544979,19.0595739863298,21.9892848192234));
#30735=CARTESIAN_POINT('Ctrl Pts',(54.5448469207738,19.0578571221787,21.9897589710997));
#30736=CARTESIAN_POINT('Ctrl Pts',(54.5611288869914,19.0541055632396,21.9908232388005));
#30737=CARTESIAN_POINT('Ctrl Pts',(54.5701509919643,19.0520927028254,21.9914140433699));
#30738=CARTESIAN_POINT('Ctrl Pts',(54.5930854885562,19.0471430368258,21.9929187627052));
#30739=CARTESIAN_POINT('Ctrl Pts',(54.6070157058985,19.0442921830061,21.9938353942528));
#30740=CARTESIAN_POINT('Ctrl Pts',(54.6905828672312,19.0281188284701,21.9993512329737));
#30741=CARTESIAN_POINT('Ctrl Pts',(54.760851522398,19.0183692872041,22.0040624180753));
#30742=CARTESIAN_POINT('Ctrl Pts',(55.0086858164157,18.997357108006,22.0209323512635));
#30743=CARTESIAN_POINT('Ctrl Pts',(55.1870754480297,19.0060978318498,22.0336107361399));
#30744=CARTESIAN_POINT('Ctrl Pts',(55.3884195402434,19.0432467413716,22.0475121720839));
#30745=CARTESIAN_POINT('Ctrl Pts',(55.4148070987268,19.0486701271835,22.0493236396646));
#30746=CARTESIAN_POINT('Ctrl Pts',(55.4582723178746,19.0585250740111,22.0522816940782));
#30747=CARTESIAN_POINT('Ctrl Pts',(55.4754149244574,19.06265152676,22.0534416353026));
#30748=CARTESIAN_POINT('Ctrl Pts',(55.4987488004834,19.0685966858054,22.0550092454916));
#30749=CARTESIAN_POINT('Ctrl Pts',(55.5049886929585,19.0702187816143,22.0554273459321));
#30750=CARTESIAN_POINT('Ctrl Pts',(55.5154393183897,19.0729896421543,22.0561255998323));
#30751=CARTESIAN_POINT('Ctrl Pts',(55.5196542990744,19.0741220130227,22.056406678919));
#30752=CARTESIAN_POINT('Ctrl Pts',(55.527633393466,19.0762937301641,22.056937696563));
#30753=CARTESIAN_POINT('Ctrl Pts',(55.5313982174934,19.0773303077249,22.0571877969514));
#30754=CARTESIAN_POINT('Ctrl Pts',(55.541238748375,19.0800708355095,22.0578403846677));
#30755=CARTESIAN_POINT('Ctrl Pts',(55.5473095157265,19.0817925878596,22.0582418497776));
#30756=CARTESIAN_POINT('Ctrl Pts',(55.5682749531333,19.0878463053209,22.0596247413766));
#30757=CARTESIAN_POINT('Ctrl Pts',(55.5831276379326,19.0923233064311,22.060598184771));
#30758=CARTESIAN_POINT('Ctrl Pts',(55.7199499988913,19.1353126133284,22.0695205377821));
#30759=CARTESIAN_POINT('Ctrl Pts',(55.83802062457,19.1853050457379,22.0769004279614));
#30760=CARTESIAN_POINT('Ctrl Pts',(56.0802577085243,19.3165948273743,22.092885568502));
#30761=CARTESIAN_POINT('Ctrl Pts',(56.2017887384573,19.4010922930311,22.1014783269401));
#30762=CARTESIAN_POINT('Ctrl Pts',(56.3258980597828,19.5095904175426,22.1117094654506));
#30763=CARTESIAN_POINT('Ctrl Pts',(56.3387638254859,19.5211363218532,22.1127890035741));
#30764=CARTESIAN_POINT('Ctrl Pts',(56.3581554809446,19.5389990808885,22.1144462182574));
#30765=CARTESIAN_POINT('Ctrl Pts',(56.3647911966308,19.5451958959145,22.1150188160601));
#30766=CARTESIAN_POINT('Ctrl Pts',(56.376274176585,19.5560670738104,22.1160194659288));
#30767=CARTESIAN_POINT('Ctrl Pts',(56.3811405423169,19.5607211163156,22.1164466394684));
#30768=CARTESIAN_POINT('Ctrl Pts',(56.3920332459515,19.5712446773882,22.1174098950999));
#30769=CARTESIAN_POINT('Ctrl Pts',(56.3980461769483,19.5771278296098,22.1179465669647));
#30770=CARTESIAN_POINT('Ctrl Pts',(56.4140936310367,19.5930288516578,22.1193923213842));
#30771=CARTESIAN_POINT('Ctrl Pts',(56.4240587024888,19.6031158228955,22.1203044433582));
#30772=CARTESIAN_POINT('Ctrl Pts',(56.4689451736135,19.6495308816316,22.1244797993637));
#30773=CARTESIAN_POINT('Ctrl Pts',(56.5025871538981,19.6870651750828,22.1277972068187));
#30774=CARTESIAN_POINT('Ctrl Pts',(56.5516673711542,19.7461835383234,22.1329388458436));
#30775=CARTESIAN_POINT('Ctrl Pts',(56.5681576959389,19.7668703657113,22.1347232694608));
#30776=CARTESIAN_POINT('Ctrl Pts',(56.6906085573119,19.9269124462104,22.1484129697966));
#30777=CARTESIAN_POINT('Ctrl Pts',(56.7782076008204,20.079325106133,22.1608886736713));
#30778=CARTESIAN_POINT('Ctrl Pts',(56.8549747247496,20.2659610832714,22.1745882585467));
#30779=CARTESIAN_POINT('Ctrl Pts',(56.8646601625911,20.2909252622256,22.1763885421882));
#30780=CARTESIAN_POINT('Ctrl Pts',(56.8798584191307,20.3325661397942,22.179330319118));
#30781=CARTESIAN_POINT('Ctrl Pts',(56.8856586710146,20.3491336073491,22.1804849916147));
#30782=CARTESIAN_POINT('Ctrl Pts',(56.8932859935294,20.3718780928727,22.1820466944667));
#30783=CARTESIAN_POINT('Ctrl Pts',(56.8953027617215,20.3779900099763,22.1824640570668));
#30784=CARTESIAN_POINT('Ctrl Pts',(56.8986367459139,20.3882605972091,22.1831614234442));
#30785=CARTESIAN_POINT('Ctrl Pts',(56.8999699514307,20.3924139775989,22.1834423478833));
#30786=CARTESIAN_POINT('Ctrl Pts',(56.9024713724709,20.4002954874993,22.1839733301926));
#30787=CARTESIAN_POINT('Ctrl Pts',(56.9036422740737,20.4040227199068,22.1842235484473));
#30788=CARTESIAN_POINT('Ctrl Pts',(56.9066788170377,20.4137889454666,22.1848769160476));
#30789=CARTESIAN_POINT('Ctrl Pts',(56.9085267376512,20.4198334669496,22.1852790383876));
#30790=CARTESIAN_POINT('Ctrl Pts',(56.9148284310914,20.4408021778623,22.1866665286772));
#30791=CARTESIAN_POINT('Ctrl Pts',(56.9191362626855,20.4557701172069,22.1876438426298));
#30792=CARTESIAN_POINT('Ctrl Pts',(56.9564852226199,20.591504023708,22.1964012050979));
#30793=CARTESIAN_POINT('Ctrl Pts',(56.9782676272977,20.7150975577829,22.2036366071863));
#30794=CARTESIAN_POINT('Ctrl Pts',(57.0003820395373,20.9897963101217,22.2196247974323));
#30795=CARTESIAN_POINT('Ctrl Pts',(56.9954644111347,21.1405219317575,22.2283660367647));
#30796=CARTESIAN_POINT('Ctrl Pts',(56.971172018139,21.3062748612305,22.2387642985368));
#30797=CARTESIAN_POINT('Ctrl Pts',(56.9684578571297,21.3232600368203,22.2398385344605));
#30798=CARTESIAN_POINT('Ctrl Pts',(56.9639790185299,21.3491361995339,22.2414892758297));
#30799=CARTESIAN_POINT('Ctrl Pts',(56.9623727873206,21.3580540605275,22.2420607644256));
#30800=CARTESIAN_POINT('Ctrl Pts',(56.9593345936081,21.3742874246815,22.2431059023321));
#30801=CARTESIAN_POINT('Ctrl Pts',(56.9579222722598,21.381606471782,22.2435789191615));
#30802=CARTESIAN_POINT('Ctrl Pts',(56.9547757458389,21.3974352367301,22.2446058847258));
#30803=CARTESIAN_POINT('Ctrl Pts',(56.9530269290366,21.4059418609066,22.2451602909001));
#30804=CARTESIAN_POINT('Ctrl Pts',(56.9481026156856,21.4291261784821,22.2466782563411));
#30805=CARTESIAN_POINT('Ctrl Pts',(56.9448168810974,21.4437796264216,22.2476453167328));
#30806=CARTESIAN_POINT('Ctrl Pts',(56.9269837393075,21.519305565867,22.2526703123439));
#30807=CARTESIAN_POINT('Ctrl Pts',(56.9097441922972,21.5795000446673,22.2568138156584));
#30808=CARTESIAN_POINT('Ctrl Pts',(56.8341068292719,21.8032584937247,22.2727516274026));
#30809=CARTESIAN_POINT('Ctrl Pts',(56.7572835271216,21.9597465581341,22.2850865375878));
#30810=CARTESIAN_POINT('Ctrl Pts',(56.6319421699512,22.1482956386775,22.3005918544247));
#30811=CARTESIAN_POINT('Ctrl Pts',(56.6009586083271,22.1911132364786,22.3041547560605));
#30812=CARTESIAN_POINT('Ctrl Pts',(56.5626154137994,22.2398973797142,22.3082194092159));
#30813=CARTESIAN_POINT('Ctrl Pts',(56.5568719410436,22.2471015238296,22.3088197798853));
#30814=CARTESIAN_POINT('Ctrl Pts',(56.5479536706485,22.2581302378595,22.3097387385641));
#30815=CARTESIAN_POINT('Ctrl Pts',(56.5448142396232,22.2619830538696,22.3100597447509));
#30816=CARTESIAN_POINT('Ctrl Pts',(56.5390076146459,22.2690550028525,22.3106488472951));
#30817=CARTESIAN_POINT('Ctrl Pts',(56.5363447130036,22.2722774703801,22.3109172326787));
#30818=CARTESIAN_POINT('Ctrl Pts',(56.5303162798953,22.2795261551094,22.311520849531));
#30819=CARTESIAN_POINT('Ctrl Pts',(56.5269449863657,22.2835474701986,22.3118556565445));
#30820=CARTESIAN_POINT('Ctrl Pts',(56.5169631075879,22.2953589762317,22.3128390479792));
#30821=CARTESIAN_POINT('Ctrl Pts',(56.5103083770861,22.3031118768778,22.3134845163494));
#30822=CARTESIAN_POINT('Ctrl Pts',(56.4574515166504,22.3637423702608,22.3185353564067));
#30823=CARTESIAN_POINT('Ctrl Pts',(56.4085406773114,22.4142042331848,22.3227581299532));
#30824=CARTESIAN_POINT('Ctrl Pts',(56.2329790976124,22.5771663913761,22.3368967834419));
#30825=CARTESIAN_POINT('Ctrl Pts',(56.0947392657173,22.6760786430796,22.3464419036216));
#30826=CARTESIAN_POINT('Ctrl Pts',(55.9011792211822,22.7802966474929,22.359682374932));
#30827=CARTESIAN_POINT('Ctrl Pts',(55.8558038133251,22.8025480075239,22.3627726463147));
#30828=CARTESIAN_POINT('Ctrl Pts',(55.7971829979176,22.8285820949323,22.3667725602011));
#30829=CARTESIAN_POINT('Ctrl Pts',(55.784674454502,22.8339845135468,22.3676264433042));
#30830=CARTESIAN_POINT('Ctrl Pts',(55.7644676461298,22.8424672347026,22.369006888356));
#30831=CARTESIAN_POINT('Ctrl Pts',(55.756803667968,22.8456284831238,22.3695306986817));
#30832=CARTESIAN_POINT('Ctrl Pts',(55.7421638615069,22.8515606127669,22.370531842752));
#30833=CARTESIAN_POINT('Ctrl Pts',(55.7351916491895,22.8543400811375,22.3710088766293));
#30834=CARTESIAN_POINT('Ctrl Pts',(55.7192171121566,22.8606040660049,22.3721024681726));
#30835=CARTESIAN_POINT('Ctrl Pts',(55.7102049029022,22.8640626961907,22.3727198813044));
#30836=CARTESIAN_POINT('Ctrl Pts',(55.6865928764559,22.8729282338661,22.3743388514017));
#30837=CARTESIAN_POINT('Ctrl Pts',(55.6719544654871,22.8782297837889,22.3753438807442));
#30838=CARTESIAN_POINT('Ctrl Pts',(55.5437398241881,22.922974204115,22.3841601501546));
#30839=CARTESIAN_POINT('Ctrl Pts',(55.4268952292185,22.9522382108311,22.3923090568675));
#30840=CARTESIAN_POINT('Ctrl Pts',(55.2604470155227,22.978263322737,22.4039843683873));
#30841=CARTESIAN_POINT('Ctrl Pts',(55.2125158558117,22.9839835915043,22.4073508429909));
#30842=CARTESIAN_POINT('Ctrl Pts',(55.16444812056,22.9879598532527,22.4107149109706));
#30843=CARTESIAN_POINT('Origin',(55.,21.,6.22095488139522));
#30844=CARTESIAN_POINT('',(55.1644483538502,22.9879598339544,23.3702474674336));
#30845=CARTESIAN_POINT('',(55.164448305082,22.9879598379886,23.2119648302802));
#30846=CARTESIAN_POINT('',(55.1644483516311,22.987959834138,6.22095488139522));
#30847=CARTESIAN_POINT('',(53.0052508080785,20.9981768768052,22.7789686217093));
#30848=CARTESIAN_POINT('Ctrl Pts',(55.1644483538502,22.9879598339544,23.3702474674336));
#30849=CARTESIAN_POINT('Ctrl Pts',(55.1875526887303,22.9860485932075,23.368713924432));
#30850=CARTESIAN_POINT('Ctrl Pts',(55.2106221949796,22.9837346957845,23.3671685994482));
#30851=CARTESIAN_POINT('Ctrl Pts',(55.4530047006759,22.9551474869474,23.3507848761386));
#30852=CARTESIAN_POINT('Ctrl Pts',(55.6664930236811,22.89303334915,23.3348455322072));
#30853=CARTESIAN_POINT('Ctrl Pts',(55.8724179696231,22.793871326211,23.3196409044909));
#30854=CARTESIAN_POINT('Ctrl Pts',(55.879370829335,22.7904732327871,23.3191280144358));
#30855=CARTESIAN_POINT('Ctrl Pts',(55.8983085803995,22.7810808008894,23.3177326958174));
#30856=CARTESIAN_POINT('Ctrl Pts',(55.9102534002626,22.7750058860545,23.316854435342));
#30857=CARTESIAN_POINT('Ctrl Pts',(55.9268929575256,22.7663311639797,23.3156344907239));
#30858=CARTESIAN_POINT('Ctrl Pts',(55.9316394855505,22.7638322499974,23.3152868977275));
#30859=CARTESIAN_POINT('Ctrl Pts',(55.9398384892587,22.7594733741743,23.3146872511578));
#30860=CARTESIAN_POINT('Ctrl Pts',(55.943295637845,22.7576223373053,23.3144346470344));
#30861=CARTESIAN_POINT('Ctrl Pts',(55.9505742040902,22.7536975645942,23.3139033649992));
#30862=CARTESIAN_POINT('Ctrl Pts',(55.9543943387017,22.7516215094611,23.3136248424149));
#30863=CARTESIAN_POINT('Ctrl Pts',(55.9637875055941,22.7464769337867,23.3129407077181));
#30864=CARTESIAN_POINT('Ctrl Pts',(55.9693527633204,22.7433941777708,23.3125359922492));
#30865=CARTESIAN_POINT('Ctrl Pts',(55.9897621089433,22.731960912501,23.311053717938));
#30866=CARTESIAN_POINT('Ctrl Pts',(56.0045143225361,22.7234467373072,23.3099860759078));
#30867=CARTESIAN_POINT('Ctrl Pts',(56.1038199009942,22.6644245848771,23.3028123112672));
#30868=CARTESIAN_POINT('Ctrl Pts',(56.1846516218118,22.6078970473494,23.297034617931));
#30869=CARTESIAN_POINT('Ctrl Pts',(56.3899988695879,22.4403660473972,23.2816186118194));
#30870=CARTESIAN_POINT('Ctrl Pts',(56.505313221539,22.3193852197528,23.2720748873674));
#30871=CARTESIAN_POINT('Ctrl Pts',(56.6179305488844,22.1669865721406,23.2603889902156));
#30872=CARTESIAN_POINT('Ctrl Pts',(56.6312825688485,22.148248245368,23.2589586210355));
#30873=CARTESIAN_POINT('Ctrl Pts',(56.6494947927601,22.1217301194484,23.2569412544159));
#30874=CARTESIAN_POINT('Ctrl Pts',(56.6546303235663,22.1141409336612,23.2563646807037));
#30875=CARTESIAN_POINT('Ctrl Pts',(56.6639447352404,22.100169836249,23.2553045218374));
#30876=CARTESIAN_POINT('Ctrl Pts',(56.6681396669139,22.0937987929973,23.254821550069));
#30877=CARTESIAN_POINT('Ctrl Pts',(56.6765711178769,22.0808322241151,23.2538394727112));
#30878=CARTESIAN_POINT('Ctrl Pts',(56.6808055044786,22.0742354784745,23.2533402990355));
#30879=CARTESIAN_POINT('Ctrl Pts',(56.6911721142027,22.0578739978053,23.2521032644886));
#30880=CARTESIAN_POINT('Ctrl Pts',(56.6972587007716,22.0480808215462,23.25136373718));
#30881=CARTESIAN_POINT('Ctrl Pts',(56.7197103299989,22.0112481789389,23.2485853046421));
#30882=CARTESIAN_POINT('Ctrl Pts',(56.7355161604466,21.9838749746554,23.2465262670731));
#30883=CARTESIAN_POINT('Ctrl Pts',(56.7734379174398,21.9144412823184,23.2413148138363));
#30884=CARTESIAN_POINT('Ctrl Pts',(56.794712857841,21.8719461405824,23.2381351250671));
#30885=CARTESIAN_POINT('Ctrl Pts',(56.8547713207095,21.7404528777584,23.2283307252892));
#30886=CARTESIAN_POINT('Ctrl Pts',(56.888593445687,21.6493527394525,23.2215775941274));
#30887=CARTESIAN_POINT('Ctrl Pts',(56.9461673353621,21.4510445581725,23.2071740806812));
#30888=CARTESIAN_POINT('Ctrl Pts',(56.9679846630149,21.3435834236867,23.1995425786452));
#30889=CARTESIAN_POINT('Ctrl Pts',(56.9827530321108,21.2190260423238,23.1912328516155));
#30890=CARTESIAN_POINT('Ctrl Pts',(56.9844411331688,21.2031635328648,23.190184635181));
#30891=CARTESIAN_POINT('Ctrl Pts',(56.9865382697136,21.1809254785505,23.1887307203448));
#30892=CARTESIAN_POINT('Ctrl Pts',(56.9871071937269,21.174566116905,23.1883167315292));
#30893=CARTESIAN_POINT('Ctrl Pts',(56.9879760761829,21.1642986435778,23.1876513239162));
#30894=CARTESIAN_POINT('Ctrl Pts',(56.9882950611097,21.1603922516021,23.1873988602531));
#30895=CARTESIAN_POINT('Ctrl Pts',(56.9889437931303,21.1521481966832,23.1868675716016));
#30896=CARTESIAN_POINT('Ctrl Pts',(56.9892708681074,21.1478103511436,23.1865889033597));
#30897=CARTESIAN_POINT('Ctrl Pts',(56.9900421585445,21.137114515127,23.1859038948312));
#30898=CARTESIAN_POINT('Ctrl Pts',(56.9904701024633,21.1307553322432,23.1854984563951));
#30899=CARTESIAN_POINT('Ctrl Pts',(56.9919345925874,21.1073168748699,23.1840104928581));
#30900=CARTESIAN_POINT('Ctrl Pts',(56.9927818892099,21.0902259453287,23.1829379840885));
#30901=CARTESIAN_POINT('Ctrl Pts',(56.9970556815977,20.9737219898884,23.1756991873359));
#30902=CARTESIAN_POINT('Ctrl Pts',(56.9932621818815,20.8741718490033,23.1698676922224));
#30903=CARTESIAN_POINT('Ctrl Pts',(56.9634431679508,20.6111298883732,23.1544720798639));
#30904=CARTESIAN_POINT('Ctrl Pts',(56.9245085192051,20.4499181991109,23.1449954484879));
#30905=CARTESIAN_POINT('Ctrl Pts',(56.8587879331676,20.2758667397828,23.1335236801344));
#30906=CARTESIAN_POINT('Ctrl Pts',(56.8511242032126,20.2564943222127,23.1322296933896));
#30907=CARTESIAN_POINT('Ctrl Pts',(56.8388991535796,20.2269530711962,23.1302282851751));
#30908=CARTESIAN_POINT('Ctrl Pts',(56.8345535452792,20.2166961428536,23.1295281000388));
#30909=CARTESIAN_POINT('Ctrl Pts',(56.8273441564334,20.2000689599384,23.1283841970194));
#30910=CARTESIAN_POINT('Ctrl Pts',(56.8245323880571,20.1936763070465,23.1279422539157));
#30911=CARTESIAN_POINT('Ctrl Pts',(56.8185650475588,20.1803003885954,23.1270129595154));
#30912=CARTESIAN_POINT('Ctrl Pts',(56.8154026939068,20.173320290921,23.1265253818259));
#30913=CARTESIAN_POINT('Ctrl Pts',(56.8077549562634,20.1566953571391,23.1253576939694));
#30914=CARTESIAN_POINT('Ctrl Pts',(56.803232529486,20.1470679160023,23.1246763170244));
#30915=CARTESIAN_POINT('Ctrl Pts',(56.7875263593158,20.1143155713807,23.1223402741277));
#30916=CARTESIAN_POINT('Ctrl Pts',(56.775973426261,20.091371539409,23.1206728810155));
#30917=CARTESIAN_POINT('Ctrl Pts',(56.7471370084489,20.0367547738245,23.1166269036083));
#30918=CARTESIAN_POINT('Ctrl Pts',(56.7294314637788,20.0053163145938,23.1142341702073));
#30919=CARTESIAN_POINT('Ctrl Pts',(56.6060345425788,19.7994728560723,23.0981363340667));
#30920=CARTESIAN_POINT('Ctrl Pts',(56.4750119054561,19.6417183174487,23.0835243630705));
#30921=CARTESIAN_POINT('Ctrl Pts',(56.2968842411621,19.483992552103,23.0674458212872));
#30922=CARTESIAN_POINT('Ctrl Pts',(56.2708119507939,19.4620713174149,23.0651746187066));
#30923=CARTESIAN_POINT('Ctrl Pts',(56.2375992622489,19.4355682462377,23.0623949479387));
#30924=CARTESIAN_POINT('Ctrl Pts',(56.2309757686384,19.4303512146974,23.0618460732412));
#30925=CARTESIAN_POINT('Ctrl Pts',(56.2204894198042,19.4221987858299,23.0609859245855));
#30926=CARTESIAN_POINT('Ctrl Pts',(56.2166486852783,19.4192352885015,23.060672733008));
#30927=CARTESIAN_POINT('Ctrl Pts',(56.2094992228896,19.4137602808129,23.0600932109083));
#30928=CARTESIAN_POINT('Ctrl Pts',(56.2061934902591,19.4112451160129,23.0598266314776));
#30929=CARTESIAN_POINT('Ctrl Pts',(56.1985804044716,19.4054901616888,23.0592158272106));
#30930=CARTESIAN_POINT('Ctrl Pts',(56.1942677642927,19.4022574928147,23.0588720995644));
#30931=CARTESIAN_POINT('Ctrl Pts',(56.1808993120217,19.3923211384713,23.0578134421759));
#30932=CARTESIAN_POINT('Ctrl Pts',(56.1717995791893,19.3856765296031,23.0571024701889));
#30933=CARTESIAN_POINT('Ctrl Pts',(56.0844921031683,19.3230520181378,23.0503672868372));
#30934=CARTESIAN_POINT('Ctrl Pts',(56.0023772651679,19.272712385282,23.044684660013));
#30935=CARTESIAN_POINT('Ctrl Pts',(55.7671423967155,19.1509539468919,23.0292345071162));
#30936=CARTESIAN_POINT('Ctrl Pts',(55.6081307236582,19.0927370793039,23.0196200082326));
#30937=CARTESIAN_POINT('Ctrl Pts',(55.4160055260398,19.0489045509081,23.0075386372113));
#30938=CARTESIAN_POINT('Ctrl Pts',(55.388187660709,19.0431800635657,23.0057805614262));
#30939=CARTESIAN_POINT('Ctrl Pts',(55.3490479363299,19.0359931247797,23.0032905010244));
#30940=CARTESIAN_POINT('Ctrl Pts',(55.3378205130788,19.0340308343984,23.0025743410944));
#30941=CARTESIAN_POINT('Ctrl Pts',(55.3196413489024,19.031013865025,23.0014114799522));
#30942=CARTESIAN_POINT('Ctrl Pts',(55.3126996613352,19.029899517437,23.0009666743903));
#30943=CARTESIAN_POINT('Ctrl Pts',(55.2982186206325,19.0276533421696,23.0000370993482));
#30944=CARTESIAN_POINT('Ctrl Pts',(55.2906783920566,19.0265279951092,22.9995521330404));
#30945=CARTESIAN_POINT('Ctrl Pts',(55.2728200808145,19.0239672857812,22.9984012292588));
#30946=CARTESIAN_POINT('Ctrl Pts',(55.2624969200019,19.0225694843224,22.9977341190151));
#30947=CARTESIAN_POINT('Ctrl Pts',(55.227985896426,19.018171541122,22.9954975915836));
#30948=CARTESIAN_POINT('Ctrl Pts',(55.2037548481514,19.0155339549619,22.9939168674208));
#30949=CARTESIAN_POINT('Ctrl Pts',(55.1459242496455,19.0103093159642,22.9901179446026));
#30950=CARTESIAN_POINT('Ctrl Pts',(55.1122964086017,19.0081284680849,22.9878877677947));
#30951=CARTESIAN_POINT('Ctrl Pts',(54.9082050587891,19.000077133985,22.9742230755));
#30952=CARTESIAN_POINT('Ctrl Pts',(54.7376340198427,19.0152416919135,22.9621705096904));
#30953=CARTESIAN_POINT('Ctrl Pts',(54.543452890987,19.0579921827243,22.9484378914524));
#30954=CARTESIAN_POINT('Ctrl Pts',(54.5159263518666,19.0646699399603,22.9464932075839));
#30955=CARTESIAN_POINT('Ctrl Pts',(54.4478441283461,19.082729790655,22.9417018142102));
#30956=CARTESIAN_POINT('Ctrl Pts',(54.4074864741428,19.0948151077224,22.9388779976395));
#30957=CARTESIAN_POINT('Ctrl Pts',(54.3597364574703,19.110778510702,22.9355804087703));
#30958=CARTESIAN_POINT('Ctrl Pts',(54.351950357403,19.113435157266,22.9350441128625));
#30959=CARTESIAN_POINT('Ctrl Pts',(54.3392328362932,19.1178624474355,22.9341707116321));
#30960=CARTESIAN_POINT('Ctrl Pts',(54.33429165259,19.1196044540795,22.9338320026674));
#30961=CARTESIAN_POINT('Ctrl Pts',(54.3254195784695,19.1227716443559,22.9332250580764));
#30962=CARTESIAN_POINT('Ctrl Pts',(54.3214862740021,19.1241897300222,22.9329564157882));
#30963=CARTESIAN_POINT('Ctrl Pts',(54.3128782687993,19.1273238173764,22.9323694575363));
#30964=CARTESIAN_POINT('Ctrl Pts',(54.3082055328977,19.1290449564336,22.9320514501441));
#30965=CARTESIAN_POINT('Ctrl Pts',(54.2953864046925,19.13382130009,22.9311805957229));
#30966=CARTESIAN_POINT('Ctrl Pts',(54.2872533642442,19.1369123749882,22.9306298253768));
#30967=CARTESIAN_POINT('Ctrl Pts',(54.2361825597691,19.1567059173028,22.9271807199228));
#30968=CARTESIAN_POINT('Ctrl Pts',(54.1938103249119,19.1748399761501,22.9243610336628));
#30969=CARTESIAN_POINT('Ctrl Pts',(54.0408900316513,19.2466515318523,22.9142073197606));
#30970=CARTESIAN_POINT('Ctrl Pts',(53.9347345236412,19.3090426621499,22.9071894004573));
#30971=CARTESIAN_POINT('Ctrl Pts',(53.740106018739,19.4490783099857,22.893220266618));
#30972=CARTESIAN_POINT('Ctrl Pts',(53.6514202282217,19.5255448017021,22.8863070178739));
#30973=CARTESIAN_POINT('Ctrl Pts',(53.5591075622195,19.6204717614227,22.8780888329795));
#30974=CARTESIAN_POINT('Ctrl Pts',(53.5484016902059,19.6317414338212,22.8771186945713));
#30975=CARTESIAN_POINT('Ctrl Pts',(53.5312666604669,19.6502063090987,22.875537305142));
#30976=CARTESIAN_POINT('Ctrl Pts',(53.5247559517101,19.657325198205,22.8749295368323));
#30977=CARTESIAN_POINT('Ctrl Pts',(53.513271201472,19.6700671456049,22.8738449305129));
#30978=CARTESIAN_POINT('Ctrl Pts',(53.5082767490647,19.6756716201505,22.8733689638534));
#30979=CARTESIAN_POINT('Ctrl Pts',(53.4978287371467,19.6875298445927,22.8723640980562));
#30980=CARTESIAN_POINT('Ctrl Pts',(53.4923823366013,19.6937896841029,22.8718349142052));
#30981=CARTESIAN_POINT('Ctrl Pts',(53.4813976287212,19.7065752222454,22.8707565580318));
#30982=CARTESIAN_POINT('Ctrl Pts',(53.4758619542447,19.7131029444985,22.8702072929601));
#30983=CARTESIAN_POINT('Ctrl Pts',(53.4521583508878,19.741421943914,22.8678298146206));
#30984=CARTESIAN_POINT('Ctrl Pts',(53.4344152195748,19.7635629203708,22.8659845635901));
#30985=CARTESIAN_POINT('Ctrl Pts',(53.3662683598414,19.8524202091886,22.8586280152659));
#30986=CARTESIAN_POINT('Ctrl Pts',(53.3196136778135,19.921891847168,22.8529774307393));
#30987=CARTESIAN_POINT('Ctrl Pts',(53.2412710452091,20.0560457482043,22.8422826071459));
#30988=CARTESIAN_POINT('Ctrl Pts',(53.2084547445226,20.1199193115414,22.8372745521671));
#30989=CARTESIAN_POINT('Ctrl Pts',(53.1337834691278,20.2868333937937,22.8245228509604));
#30990=CARTESIAN_POINT('Ctrl Pts',(53.0969608216442,20.3918730263889,22.8168002976119));
#30991=CARTESIAN_POINT('Ctrl Pts',(53.0664944665588,20.5093986504415,22.8088293104622));
#30992=CARTESIAN_POINT('Ctrl Pts',(53.063990684449,20.5193740820848,22.8081579587824));
#30993=CARTESIAN_POINT('Ctrl Pts',(53.0603224230704,20.5344829141993,22.8071494561963));
#30994=CARTESIAN_POINT('Ctrl Pts',(53.0591009702892,20.5396021094467,22.8068091940248));
#30995=CARTESIAN_POINT('Ctrl Pts',(53.0569452083263,20.5487981258443,22.8062006102182));
#30996=CARTESIAN_POINT('Ctrl Pts',(53.0560034515358,20.5528730882056,22.8059318717448));
#30997=CARTESIAN_POINT('Ctrl Pts',(53.0539727828272,20.5617874527811,22.8053460364319));
#30998=CARTESIAN_POINT('Ctrl Pts',(53.0528891044388,20.5666279563752,22.8050292395965));
#30999=CARTESIAN_POINT('Ctrl Pts',(53.0506862507167,20.5766425950012,22.8043764255838));
#31000=CARTESIAN_POINT('Ctrl Pts',(53.0495695923727,20.5818172504558,22.8040405500336));
#31001=CARTESIAN_POINT('Ctrl Pts',(53.0467457866064,20.5951603088361,22.8031780426417));
#31002=CARTESIAN_POINT('Ctrl Pts',(53.0450692530142,20.6033351821776,22.8026530432196));
#31003=CARTESIAN_POINT('Ctrl Pts',(53.0402915204004,20.627397973566,22.8011171366485));
#31004=CARTESIAN_POINT('Ctrl Pts',(53.0373322815782,20.643313782092,22.8001133014111));
#31005=CARTESIAN_POINT('Ctrl Pts',(53.015163999816,20.7711849833125,22.7921319427207));
#31006=CARTESIAN_POINT('Ctrl Pts',(53.0053546549519,20.8845682234732,22.7855596182985));
#31007=CARTESIAN_POINT('Ctrl Pts',(53.005250832938,20.9981770887742,22.7789685690919));
#31008=CARTESIAN_POINT('Ctrl Pts',(53.0052508331338,20.9981768744968,22.7789685815233));
#31009=CARTESIAN_POINT('Ctrl Pts',(53.0051453360732,21.1136051175367,22.7722719806175));
#31010=CARTESIAN_POINT('Ctrl Pts',(53.015058653874,21.2288184959203,22.7655756215079));
#31011=CARTESIAN_POINT('Ctrl Pts',(53.041379234816,21.3798229821317,22.7562946358845));
#31012=CARTESIAN_POINT('Ctrl Pts',(53.0489400926171,21.4169241618426,22.7539745442792));
#31013=CARTESIAN_POINT('Ctrl Pts',(53.0601601337043,21.4649519739355,22.7509086422972));
#31014=CARTESIAN_POINT('Ctrl Pts',(53.062864854609,21.4760950166121,22.7501929020584));
#31015=CARTESIAN_POINT('Ctrl Pts',(53.0681980994851,21.4972690408415,22.7488240992638));
#31016=CARTESIAN_POINT('Ctrl Pts',(53.070809070488,21.5073040831553,22.7481716136797));
#31017=CARTESIAN_POINT('Ctrl Pts',(53.0754731027712,21.5246730208645,22.747035532366));
#31018=CARTESIAN_POINT('Ctrl Pts',(53.0774901615593,21.5320164240476,22.7465531087708));
#31019=CARTESIAN_POINT('Ctrl Pts',(53.081453191364,21.546127542573,22.7456219568207));
#31020=CARTESIAN_POINT('Ctrl Pts',(53.0833930499127,21.552896867841,22.7451734333469));
#31021=CARTESIAN_POINT('Ctrl Pts',(53.0880628139187,21.5688725404339,22.7441105039795));
#31022=CARTESIAN_POINT('Ctrl Pts',(53.0908234151917,21.5780696614237,22.7434951053604));
#31023=CARTESIAN_POINT('Ctrl Pts',(53.1007541000729,21.6103071679826,22.741325581283));
#31024=CARTESIAN_POINT('Ctrl Pts',(53.1082755110909,21.6332362916083,22.7397600405652));
#31025=CARTESIAN_POINT('Ctrl Pts',(53.1605709874856,21.7834043917928,22.7293539544039));
#31026=CARTESIAN_POINT('Ctrl Pts',(53.2177291450206,21.9059360388466,22.7200974280056));
#31027=CARTESIAN_POINT('Ctrl Pts',(53.3374097423015,22.1066096699775,22.7038185989115));
#31028=CARTESIAN_POINT('Ctrl Pts',(53.3942606071647,22.1876001092131,22.6968923946849));
#31029=CARTESIAN_POINT('Ctrl Pts',(53.4830875165198,22.296037913884,22.6873674253064));
#31030=CARTESIAN_POINT('Ctrl Pts',(53.5102840777869,22.327209400868,22.6845977280595));
#31031=CARTESIAN_POINT('Ctrl Pts',(53.5440408153854,22.3635535681865,22.6813519937749));
#31032=CARTESIAN_POINT('Ctrl Pts',(53.5496868286309,22.3695572975213,22.6808152743485));
#31033=CARTESIAN_POINT('Ctrl Pts',(53.5587989233984,22.379127167919,22.6799591092306));
#31034=CARTESIAN_POINT('Ctrl Pts',(53.5622413410306,22.3827155630702,22.6796379283695));
#31035=CARTESIAN_POINT('Ctrl Pts',(53.5686032623531,22.3892978181851,22.679048574456));
#31036=CARTESIAN_POINT('Ctrl Pts',(53.5715187483275,22.3922953574548,22.678780111681));
#31037=CARTESIAN_POINT('Ctrl Pts',(53.5781143711546,22.3990340808006,22.6781764009049));
#31038=CARTESIAN_POINT('Ctrl Pts',(53.5817998509754,22.4027699168376,22.6778415770493));
#31039=CARTESIAN_POINT('Ctrl Pts',(53.5927018127565,22.4137339554812,22.67685836163));
#31040=CARTESIAN_POINT('Ctrl Pts',(53.5999592466746,22.4209214560237,22.6762130835218));
#31041=CARTESIAN_POINT('Ctrl Pts',(53.6574291114675,22.4769697260454,22.6711722602938));
#31042=CARTESIAN_POINT('Ctrl Pts',(53.7101348254793,22.5232157620165,22.6669584868662));
#31043=CARTESIAN_POINT('Ctrl Pts',(53.8980658465668,22.6713475138432,22.6528330328157));
#31044=CARTESIAN_POINT('Ctrl Pts',(54.0437450344656,22.7587610030584,22.6432931665649));
#31045=CARTESIAN_POINT('Ctrl Pts',(54.2450715908759,22.8470715021673,22.6300541719681));
#31046=CARTESIAN_POINT('Ctrl Pts',(54.2921826708261,22.8656323343491,22.626958370829));
#31047=CARTESIAN_POINT('Ctrl Pts',(54.3522090215923,22.8866804943506,22.6229920844478));
#31048=CARTESIAN_POINT('Ctrl Pts',(54.3645137219724,22.8908605493942,22.6221779582407));
#31049=CARTESIAN_POINT('Ctrl Pts',(54.3849181851159,22.8975705290688,22.6208257403055));
#31050=CARTESIAN_POINT('Ctrl Pts',(54.3929949356308,22.9001695713855,22.6202899286777));
#31051=CARTESIAN_POINT('Ctrl Pts',(54.4082171215991,22.9049610097096,22.6192789294699));
#31052=CARTESIAN_POINT('Ctrl Pts',(54.4153587962142,22.9071649336191,22.6188041295629));
#31053=CARTESIAN_POINT('Ctrl Pts',(54.4314469558668,22.9120308897033,22.6177333902377));
#31054=CARTESIAN_POINT('Ctrl Pts',(54.4404000311366,22.9146703520779,22.6171367260849));
#31055=CARTESIAN_POINT('Ctrl Pts',(54.4633159294062,22.9212517446198,22.615607348649));
#31056=CARTESIAN_POINT('Ctrl Pts',(54.4773036437228,22.9251042980848,22.6146717639242));
#31057=CARTESIAN_POINT('Ctrl Pts',(54.5651231268361,22.9482642348591,22.6087838967931));
#31058=CARTESIAN_POINT('Ctrl Pts',(54.63996122882,22.963471665927,22.6037011733299));
#31059=CARTESIAN_POINT('Ctrl Pts',(54.864227588018,22.995790348985,22.5882850481216));
#31060=CARTESIAN_POINT('Ctrl Pts',(55.0148363468645,23.0003360640307,22.5776559059377));
#31061=CARTESIAN_POINT('Ctrl Pts',(55.1644483539992,22.9879598339421,22.5673314474746));
#31062=CARTESIAN_POINT('Ctrl Pts',(55.16444812056,22.9879598532527,22.4107149109706));
#31063=CARTESIAN_POINT('Ctrl Pts',(55.092998751669,22.9938702917407,22.4157153656997));
#31064=CARTESIAN_POINT('Ctrl Pts',(55.0212477053551,22.9959274312002,22.4207116381971));
#31065=CARTESIAN_POINT('Ctrl Pts',(54.9038934735875,22.9929558220811,22.4287132587244));
#31066=CARTESIAN_POINT('Ctrl Pts',(54.8583300774655,22.9902361026577,22.431777235822));
#31067=CARTESIAN_POINT('Ctrl Pts',(54.8040622238466,22.9851233423472,22.4353455123856));
#31068=CARTESIAN_POINT('Ctrl Pts',(54.7952335802668,22.9842320975303,22.4359234413858));
#31069=CARTESIAN_POINT('Ctrl Pts',(54.7815423324367,22.9827576222653,22.4368153674359));
#31070=CARTESIAN_POINT('Ctrl Pts',(54.7766755663477,22.9822153615976,22.4371315695007));
#31071=CARTESIAN_POINT('Ctrl Pts',(54.7676516610276,22.9811762515095,22.4377162346869));
#31072=CARTESIAN_POINT('Ctrl Pts',(54.7634941200175,22.980684240208,22.4379849538012));
#31073=CARTESIAN_POINT('Ctrl Pts',(54.7540349013644,22.9795346097989,22.438594886404));
#31074=CARTESIAN_POINT('Ctrl Pts',(54.7487343032689,22.9788687809919,22.4389356355363));
#31075=CARTESIAN_POINT('Ctrl Pts',(54.7349385837194,22.9770795217114,22.439819947821));
#31076=CARTESIAN_POINT('Ctrl Pts',(54.72644780779,22.9759226184039,22.4403616939125));
#31077=CARTESIAN_POINT('Ctrl Pts',(54.6696468990648,22.967810105479,22.4439705446231));
#31078=CARTESIAN_POINT('Ctrl Pts',(54.6215942770523,22.9591375037917,22.4469495944768));
#31079=CARTESIAN_POINT('Ctrl Pts',(54.5617114703128,22.9460438061985,22.4506228932857));
#31080=CARTESIAN_POINT('Ctrl Pts',(54.549543907413,22.9432634019586,22.4513672063442));
#31081=CARTESIAN_POINT('Ctrl Pts',(54.5235250428917,22.9370603304564,22.4529558992286));
#31082=CARTESIAN_POINT('Ctrl Pts',(54.5096827213903,22.9336028772246,22.4537993111489));
#31083=CARTESIAN_POINT('Ctrl Pts',(54.3674794708185,22.8964589275022,22.4624558035776));
#31084=CARTESIAN_POINT('Ctrl Pts',(54.2427479200608,22.8501917243545,22.4700054792398));
#31085=CARTESIAN_POINT('Ctrl Pts',(54.0762814461305,22.7687674941564,22.4809656359055));
#31086=CARTESIAN_POINT('Ctrl Pts',(54.0299658303962,22.7437968678231,22.4841158779019));
#31087=CARTESIAN_POINT('Ctrl Pts',(53.9650633857615,22.7054189632111,22.4887172557206));
#31088=CARTESIAN_POINT('Ctrl Pts',(53.9456344926247,22.6934759961514,22.4901196612445));
#31089=CARTESIAN_POINT('Ctrl Pts',(53.9112895465205,22.6715439544146,22.4926467932075));
#31090=CARTESIAN_POINT('Ctrl Pts',(53.8962953435343,22.6616815704203,22.4937669141107));
#31091=CARTESIAN_POINT('Ctrl Pts',(53.873806610768,22.6464510111782,22.4954736112511));
#31092=CARTESIAN_POINT('Ctrl Pts',(53.8662126013602,22.6412308223551,22.4960546231608));
#31093=CARTESIAN_POINT('Ctrl Pts',(53.852534691493,22.631688273234,22.4971097817043));
#31094=CARTESIAN_POINT('Ctrl Pts',(53.8464383258529,22.627384010214,22.4975832328444));
#31095=CARTESIAN_POINT('Ctrl Pts',(53.8333983799302,22.6180672296986,22.4986028155109));
#31096=CARTESIAN_POINT('Ctrl Pts',(53.826462659292,22.6130440186073,22.4991493525739));
#31097=CARTESIAN_POINT('Ctrl Pts',(53.8078793435547,22.5994017180392,22.5006253150456));
#31098=CARTESIAN_POINT('Ctrl Pts',(53.7962931392008,22.5907002514828,22.5015579271549));
#31099=CARTESIAN_POINT('Ctrl Pts',(53.7406877386876,22.5479841211556,22.5060951104498));
#31100=CARTESIAN_POINT('Ctrl Pts',(53.698013422705,22.5122672239427,22.5097665166));
#31101=CARTESIAN_POINT('Ctrl Pts',(53.6469821174682,22.4657932221256,22.5144024445763));
#31102=CARTESIAN_POINT('Ctrl Pts',(53.637165154185,22.4566702890569,22.5153061259929));
#31103=CARTESIAN_POINT('Ctrl Pts',(53.5050658413079,22.3314057298249,22.5276277863977));
#31104=CARTESIAN_POINT('Ctrl Pts',(53.3979186834733,22.2003307151686,22.5396048900806));
#31105=CARTESIAN_POINT('Ctrl Pts',(53.2808000484889,22.012974888698,22.554731808105));
#31106=CARTESIAN_POINT('Ctrl Pts',(53.2548129746005,21.9675173933419,22.5582606418134));
#31107=CARTESIAN_POINT('Ctrl Pts',(53.2263974495058,21.9129326649336,22.5622916535438));
#31108=CARTESIAN_POINT('Ctrl Pts',(53.222209244717,21.904749742239,22.5628906396545));
#31109=CARTESIAN_POINT('Ctrl Pts',(53.2158459801481,21.8921023768893,22.5638079327298));
#31110=CARTESIAN_POINT('Ctrl Pts',(53.2136308402978,21.8876584050031,22.5641286444772));
#31111=CARTESIAN_POINT('Ctrl Pts',(53.2095812260238,21.8794575910284,22.5647174693087));
#31112=CARTESIAN_POINT('Ctrl Pts',(53.2077419766136,21.8757032709956,22.5649858694102));
#31113=CARTESIAN_POINT('Ctrl Pts',(53.2036183348874,21.867218582008,22.5655898474871));
#31114=CARTESIAN_POINT('Ctrl Pts',(53.2013408205431,21.8624849641657,22.5659249986879));
#31115=CARTESIAN_POINT('Ctrl Pts',(53.1946777302972,21.8484951229244,22.5669103473822));
#31116=CARTESIAN_POINT('Ctrl Pts',(53.1903446376154,21.8392138887377,22.5675574102831));
#31117=CARTESIAN_POINT('Ctrl Pts',(53.1564510500299,21.7651324442052,22.5726727390936));
#31118=CARTESIAN_POINT('Ctrl Pts',(53.1303054894104,21.6988169916693,22.576953090349));
#31119=CARTESIAN_POINT('Ctrl Pts',(53.0696741379118,21.5170645829692,22.5882555807318));
#31120=CARTESIAN_POINT('Ctrl Pts',(53.0419975719998,21.3996771463598,22.5951219070059));
#31121=CARTESIAN_POINT('Ctrl Pts',(53.0118886056539,21.1876937219276,22.6076992535515));
#31122=CARTESIAN_POINT('Ctrl Pts',(53.0052664294991,21.094076959173,22.6133111086405));
#31123=CARTESIAN_POINT('Ctrl Pts',(53.0052474901953,20.9858297683454,22.6200389753441));
#31124=CARTESIAN_POINT('Ctrl Pts',(53.0054034722093,20.9713112447033,22.6209461139882));
#31125=CARTESIAN_POINT('Ctrl Pts',(53.0059201341663,20.9474622962105,22.622444642487));
#31126=CARTESIAN_POINT('Ctrl Pts',(53.0061878598199,20.9381302453841,22.6230331300854));
#31127=CARTESIAN_POINT('Ctrl Pts',(53.006787789477,20.9213331068914,22.6240963265487));
#31128=CARTESIAN_POINT('Ctrl Pts',(53.0070964514545,20.9138673118923,22.6245702906203));
#31129=CARTESIAN_POINT('Ctrl Pts',(53.0078448955458,20.8979338674464,22.6255849025647));
#31130=CARTESIAN_POINT('Ctrl Pts',(53.0082967342974,20.8894669581286,22.6261259187958));
#31131=CARTESIAN_POINT('Ctrl Pts',(53.0096664959496,20.866546442037,22.6275956496375));
#31132=CARTESIAN_POINT('Ctrl Pts',(53.0106878553721,20.852099755385,22.6285275804372));
#31133=CARTESIAN_POINT('Ctrl Pts',(53.0168683571946,20.7764061442851,22.6334406213628));
#31134=CARTESIAN_POINT('Ctrl Pts',(53.0246984402708,20.7154165809302,22.6375045289539));
#31135=CARTESIAN_POINT('Ctrl Pts',(53.0614780789679,20.5060340644227,22.6518293972231));
#31136=CARTESIAN_POINT('Ctrl Pts',(53.1044576441259,20.3606420484767,22.6624788716272));
#31137=CARTESIAN_POINT('Ctrl Pts',(53.1721614539167,20.200916347281,22.6744936219287));
#31138=CARTESIAN_POINT('Ctrl Pts',(53.181241984156,20.1804588108251,22.6760376266282));
#31139=CARTESIAN_POINT('Ctrl Pts',(53.2135241773388,20.1109108505455,22.6812957272146));
#31140=CARTESIAN_POINT('Ctrl Pts',(53.2383867657655,20.0626124866743,22.6849633921613));
#31141=CARTESIAN_POINT('Ctrl Pts',(53.2695471785789,20.0077104969352,22.6891032952618));
#31142=CARTESIAN_POINT('Ctrl Pts',(53.2739536927457,20.0000652135611,22.6896790987014));
#31143=CARTESIAN_POINT('Ctrl Pts',(53.2811478492163,19.9877726501253,22.6906034806767));
#31144=CARTESIAN_POINT('Ctrl Pts',(53.2839038913492,19.9831071483973,22.6909539836961));
#31145=CARTESIAN_POINT('Ctrl Pts',(53.2888263915764,19.9748512167794,22.6915735468317));
#31146=CARTESIAN_POINT('Ctrl Pts',(53.2909851938514,19.9712563295747,22.6918430908454));
#31147=CARTESIAN_POINT('Ctrl Pts',(53.2956621558542,19.9635234986922,22.6924223793507));
#31148=CARTESIAN_POINT('Ctrl Pts',(53.2981840531741,19.959387916135,22.6927318761022));
#31149=CARTESIAN_POINT('Ctrl Pts',(53.3052404852789,19.9479105494786,22.6935900643626));
#31150=CARTESIAN_POINT('Ctrl Pts',(53.3098076981883,19.9405888362109,22.6941366682079));
#31151=CARTESIAN_POINT('Ctrl Pts',(53.336487942343,19.8984293827333,22.6972805159877));
#31152=CARTESIAN_POINT('Ctrl Pts',(53.3596319114187,19.8642521062456,22.6998149872042));
#31153=CARTESIAN_POINT('Ctrl Pts',(53.4414075294469,19.7512126928967,22.7082374947068));
#31154=CARTESIAN_POINT('Ctrl Pts',(53.504800665623,19.6759674455647,22.7139171681438));
#31155=CARTESIAN_POINT('Ctrl Pts',(53.6682640022487,19.5087278705629,22.727484953272));
#31156=CARTESIAN_POINT('Ctrl Pts',(53.7726698597119,19.4216881707559,22.7353760782752));
#31157=CARTESIAN_POINT('Ctrl Pts',(53.9050916654885,19.3324313619997,22.7452079054729));
#31158=CARTESIAN_POINT('Ctrl Pts',(53.9253361341334,19.319313556683,22.7467055485507));
#31159=CARTESIAN_POINT('Ctrl Pts',(53.9539622803344,19.3014933613065,22.7488181931838));
#31160=CARTESIAN_POINT('Ctrl Pts',(53.9621481169816,19.2964791822796,22.7494217465351));
#31161=CARTESIAN_POINT('Ctrl Pts',(53.9763990973267,19.2878906835243,22.7504716627808));
#31162=CARTESIAN_POINT('Ctrl Pts',(53.982447609913,19.2842889955243,22.7509170201939));
#31163=CARTESIAN_POINT('Ctrl Pts',(53.9950767950381,19.2768590090452,22.7518464532058));
#31164=CARTESIAN_POINT('Ctrl Pts',(54.0016605624012,19.2730362229406,22.7523307188288));
#31165=CARTESIAN_POINT('Ctrl Pts',(54.017260190871,19.2640975006701,22.7534776134172));
#31166=CARTESIAN_POINT('Ctrl Pts',(54.0262942971588,19.2590140100602,22.7541413940337));
#31167=CARTESIAN_POINT('Ctrl Pts',(54.0564480298625,19.2423546217517,22.7563558312849));
#31168=CARTESIAN_POINT('Ctrl Pts',(54.0777369716226,19.2310911786521,22.7579174941703));
#31169=CARTESIAN_POINT('Ctrl Pts',(54.1288284968502,19.2052329650925,22.7616627450694));
#31170=CARTESIAN_POINT('Ctrl Pts',(54.1588008315016,19.1909913642154,22.7638578690015));
#31171=CARTESIAN_POINT('Ctrl Pts',(54.344011353497,19.108585232087,22.7774121086704));
#31172=CARTESIAN_POINT('Ctrl Pts',(54.5070516976254,19.0597019322775,22.7893840708762));
#31173=CARTESIAN_POINT('Ctrl Pts',(54.7436880304318,19.0205346662645,22.8059629132606));
#31174=CARTESIAN_POINT('Ctrl Pts',(54.8136763738419,19.0127243385667,22.8107589765102));
#31175=CARTESIAN_POINT('Ctrl Pts',(54.8941420691767,19.0080346050364,22.8160501696307));
#31176=CARTESIAN_POINT('Ctrl Pts',(54.9043506757875,19.0075183178579,22.8167173389075));
#31177=CARTESIAN_POINT('Ctrl Pts',(54.9198066150873,19.0068557179785,22.8177207563291));
#31178=CARTESIAN_POINT('Ctrl Pts',(54.9250511135593,19.0066516175314,22.8180600712668));
#31179=CARTESIAN_POINT('Ctrl Pts',(54.9344742892906,19.0063221374573,22.8186675790737));
#31180=CARTESIAN_POINT('Ctrl Pts',(54.9386525905587,19.0061891928523,22.8189361830087));
#31181=CARTESIAN_POINT('Ctrl Pts',(54.9477984462798,19.0059269692235,22.8195224410402));
#31182=CARTESIAN_POINT('Ctrl Pts',(54.9527660677098,19.0058031162346,22.8198397907198));
#31183=CARTESIAN_POINT('Ctrl Pts',(54.9669416105508,19.0055026897701,22.8207424276101));
#31184=CARTESIAN_POINT('Ctrl Pts',(54.9761505076584,19.0053713159823,22.8213252614499));
#31185=CARTESIAN_POINT('Ctrl Pts',(55.0381002170351,19.0049166443926,22.8252241886409));
#31186=CARTESIAN_POINT('Ctrl Pts',(55.0908400959626,19.0066213661855,22.8284369355605));
#31187=CARTESIAN_POINT('Ctrl Pts',(55.315718667367,19.0228358003474,22.8419130058105));
#31188=CARTESIAN_POINT('Ctrl Pts',(55.4856438255221,19.0575752077836,22.8515991916908));
#31189=CARTESIAN_POINT('Ctrl Pts',(55.7089713365105,19.1344136649463,22.8656898030499));
#31190=CARTESIAN_POINT('Ctrl Pts',(55.7679396950883,19.1579033322196,22.869541782155));
#31191=CARTESIAN_POINT('Ctrl Pts',(55.8394092345565,19.1904014240051,22.8744269267669));
#31192=CARTESIAN_POINT('Ctrl Pts',(55.8530621899135,19.1967973630842,22.875370146346));
#31193=CARTESIAN_POINT('Ctrl Pts',(55.8744753674274,19.2071263146197,22.8768659379682));
#31194=CARTESIAN_POINT('Ctrl Pts',(55.8822847881621,19.2109564654072,22.8774149465477));
#31195=CARTESIAN_POINT('Ctrl Pts',(55.8966752344161,19.2181314354871,22.8784331966886));
#31196=CARTESIAN_POINT('Ctrl Pts',(55.9032632490416,19.2214619605569,22.8789019324261));
#31197=CARTESIAN_POINT('Ctrl Pts',(55.9178539138087,19.228940147919,22.8799458677329));
#31198=CARTESIAN_POINT('Ctrl Pts',(55.9258472057564,19.2331056189077,22.8805216864939));
#31199=CARTESIAN_POINT('Ctrl Pts',(55.9488086334058,19.2452698890248,22.8821872527772));
#31200=CARTESIAN_POINT('Ctrl Pts',(55.963702980361,19.2534055647389,22.8832818237977));
#31201=CARTESIAN_POINT('Ctrl Pts',(56.0902572475387,19.3246443597481,22.8927066239594));
#31202=CARTESIAN_POINT('Ctrl Pts',(56.195674020134,19.3981791792827,22.9014235100781));
#31203=CARTESIAN_POINT('Ctrl Pts',(56.401201805401,19.5732024639533,22.9201683169168));
#31204=CARTESIAN_POINT('Ctrl Pts',(56.499016900732,19.6763421392218,22.9301858881024));
#31205=CARTESIAN_POINT('Ctrl Pts',(56.5878029038941,19.7925524134654,22.939926341211));
#31206=CARTESIAN_POINT('Ctrl Pts',(56.5905176511349,19.7961306806596,22.9402248516379));
#31207=CARTESIAN_POINT('Ctrl Pts',(56.6032256570252,19.8129989292799,22.9416253219826));
#31208=CARTESIAN_POINT('Ctrl Pts',(56.6130649462209,19.8264048517742,22.9427187658543));
#31209=CARTESIAN_POINT('Ctrl Pts',(56.6265134541318,19.8452170161086,22.9442244336797));
#31210=CARTESIAN_POINT('Ctrl Pts',(56.6302653132038,19.8505197836554,22.9446457263116));
#31211=CARTESIAN_POINT('Ctrl Pts',(56.6362507938172,19.8590677406693,22.9453197153147));
#31212=CARTESIAN_POINT('Ctrl Pts',(56.6385007830842,19.8623013293754,22.945573507638));
#31213=CARTESIAN_POINT('Ctrl Pts',(56.6432018901952,19.8691004329026,22.9461046583597));
#31214=CARTESIAN_POINT('Ctrl Pts',(56.6456510070594,19.8726672867907,22.9463818739079));
#31215=CARTESIAN_POINT('Ctrl Pts',(56.651616021782,19.8814154987903,22.9470583658351));
#31216=CARTESIAN_POINT('Ctrl Pts',(56.6551192039271,19.8866055536877,22.9474567902047));
#31217=CARTESIAN_POINT('Ctrl Pts',(56.6676886802169,19.9054179839502,22.9488907850934));
#31218=CARTESIAN_POINT('Ctrl Pts',(56.676611999672,19.9191357312973,22.9499172602975));
#31219=CARTESIAN_POINT('Ctrl Pts',(56.6984047254779,19.9535569273485,22.9524496949407));
#31220=CARTESIAN_POINT('Ctrl Pts',(56.7110656381577,19.9743898363287,22.9539441833923));
#31221=CARTESIAN_POINT('Ctrl Pts',(56.7632228016893,20.0638673946306,22.9602253631319));
#31222=CARTESIAN_POINT('Ctrl Pts',(56.7989971744072,20.134604110048,22.9648545623867));
#31223=CARTESIAN_POINT('Ctrl Pts',(56.8947068459724,20.3556092483932,22.9788526518921));
#31224=CARTESIAN_POINT('Ctrl Pts',(56.9406684338658,20.5111714294437,22.9881392547273));
#31225=CARTESIAN_POINT('Ctrl Pts',(56.9711531759364,20.6932257036802,22.9995173723624));
#31226=CARTESIAN_POINT('Ctrl Pts',(56.9745553031364,20.715946133555,23.000944868142));
#31227=CARTESIAN_POINT('Ctrl Pts',(56.9787959564025,20.7480425414306,23.0029740937289));
#31228=CARTESIAN_POINT('Ctrl Pts',(56.9799617716072,20.7573739994876,23.0035655512563));
#31229=CARTESIAN_POINT('Ctrl Pts',(56.9818791305782,20.7736561318084,23.0046003187129));
#31230=CARTESIAN_POINT('Ctrl Pts',(56.9826602037335,20.7806032147077,23.0050426941229));
#31231=CARTESIAN_POINT('Ctrl Pts',(56.9842197339272,20.7951630667022,23.0059717251293));
#31232=CARTESIAN_POINT('Ctrl Pts',(56.9849909328174,20.802776482892,23.0064586009335));
#31233=CARTESIAN_POINT('Ctrl Pts',(56.9867246823767,20.8209338162315,23.0076224191841));
#31234=CARTESIAN_POINT('Ctrl Pts',(56.9876471224384,20.8314812436545,23.0083006078862));
#31235=CARTESIAN_POINT('Ctrl Pts',(56.9904969979849,20.8673559553041,23.010614852929));
#31236=CARTESIAN_POINT('Ctrl Pts',(56.9920245610702,20.8927116461319,23.0122633205069));
#31237=CARTESIAN_POINT('Ctrl Pts',(56.9945275141777,20.953613520845,23.0162551983083));
#31238=CARTESIAN_POINT('Ctrl Pts',(56.995037378894,20.9891691149874,23.0186122673949));
#31239=CARTESIAN_POINT('Ctrl Pts',(56.9921803729877,21.2197163889459,23.0340688063671));
#31240=CARTESIAN_POINT('Ctrl Pts',(56.9611858366273,21.4132635714133,23.0479904204564));
#31241=CARTESIAN_POINT('Ctrl Pts',(56.889781330413,21.6399850368595,23.0641670603674));
#31242=CARTESIAN_POINT('Ctrl Pts',(56.8756340981315,21.6803320278049,23.0670339867784));
#31243=CARTESIAN_POINT('Ctrl Pts',(56.8572203117068,21.7278931206529,23.0703745713239));
#31244=CARTESIAN_POINT('Ctrl Pts',(56.8541926487967,21.735571416047,23.070912639284));
#31245=CARTESIAN_POINT('Ctrl Pts',(56.8491625288446,21.7480996127196,23.0717882834729));
#31246=CARTESIAN_POINT('Ctrl Pts',(56.8471884757789,21.7529607062207,23.0721274775284));
#31247=CARTESIAN_POINT('Ctrl Pts',(56.8436071185636,21.7616809239717,23.0727348578246));
#31248=CARTESIAN_POINT('Ctrl Pts',(56.84200684963,21.7655428168709,23.0730034543396));
#31249=CARTESIAN_POINT('Ctrl Pts',(56.8384771859602,21.7739857272321,23.0735898000635));
#31250=CARTESIAN_POINT('Ctrl Pts',(56.8365428085651,21.7785645656347,23.0739072441875));
#31251=CARTESIAN_POINT('Ctrl Pts',(56.8309728978997,21.7916127555847,23.0748104203925));
#31252=CARTESIAN_POINT('Ctrl Pts',(56.8272956978076,21.8000643400396,23.0753936944983));
#31253=CARTESIAN_POINT('Ctrl Pts',(56.8021160772697,21.8568572867254,23.0793034594482));
#31254=CARTESIAN_POINT('Ctrl Pts',(56.7787542471611,21.9043567777965,23.0825259438379));
#31255=CARTESIAN_POINT('Ctrl Pts',(56.6703689274799,22.1042323985453,23.0961143165011));
#31256=CARTESIAN_POINT('Ctrl Pts',(56.5674498107945,22.246021747285,23.1058931437571));
#31257=CARTESIAN_POINT('Ctrl Pts',(56.4049029290755,22.4174229264766,23.1200016429794));
#31258=CARTESIAN_POINT('Ctrl Pts',(56.3603616887444,22.4602242753475,23.1237536432254));
#31259=CARTESIAN_POINT('Ctrl Pts',(56.302655397468,22.5107416186355,23.1285264816614));
#31260=CARTESIAN_POINT('Ctrl Pts',(56.2912900158755,22.5204674934109,23.1294624231846));
#31261=CARTESIAN_POINT('Ctrl Pts',(56.2731653721166,22.535627782729,23.1309491977405));
#31262=CARTESIAN_POINT('Ctrl Pts',(56.2664780629372,22.5411476451347,23.1314965393039));
#31263=CARTESIAN_POINT('Ctrl Pts',(56.2539750022494,22.551331631308,23.1325177427869));
#31264=CARTESIAN_POINT('Ctrl Pts',(56.2481686622943,22.5560071094177,23.1329911350777));
#31265=CARTESIAN_POINT('Ctrl Pts',(56.2352343130173,22.5663033405105,23.1340438816937));
#31266=CARTESIAN_POINT('Ctrl Pts',(56.2280939029292,22.5719081791372,23.134623856791));
#31267=CARTESIAN_POINT('Ctrl Pts',(56.2072522369521,22.588039079482,23.1363134200241));
#31268=CARTESIAN_POINT('Ctrl Pts',(56.1934524442461,22.5984358960355,23.1374280493145));
#31269=CARTESIAN_POINT('Ctrl Pts',(56.0594988603445,22.6966553380409,23.1482116843996));
#31270=CARTESIAN_POINT('Ctrl Pts',(55.9300303282188,22.7709330836322,23.158412810211));
#31271=CARTESIAN_POINT('Ctrl Pts',(55.7879970687086,22.8325186641314,23.1692019539959));
#31272=CARTESIAN_POINT('Ctrl Pts',(55.7824454118992,22.8348959675945,23.1696229774918));
#31273=CARTESIAN_POINT('Ctrl Pts',(55.6660635245657,22.8841082213906,23.1784339184179));
#31274=CARTESIAN_POINT('Ctrl Pts',(55.5512214303481,22.9208499758922,23.1868586738788));
#31275=CARTESIAN_POINT('Ctrl Pts',(55.4183870749249,22.9504429886334,23.1958721356301));
#31276=CARTESIAN_POINT('Ctrl Pts',(55.4029742360403,22.9536855935929,23.1969068777261));
#31277=CARTESIAN_POINT('Ctrl Pts',(55.3812952865156,22.9579790055342,23.1983452503405));
#31278=CARTESIAN_POINT('Ctrl Pts',(55.3750605707958,22.9591828532656,23.1987569463429));
#31279=CARTESIAN_POINT('Ctrl Pts',(55.3649754571175,22.9610802591352,23.1994195975235));
#31280=CARTESIAN_POINT('Ctrl Pts',(55.3611286432068,22.9617922853275,23.1996715820059));
#31281=CARTESIAN_POINT('Ctrl Pts',(55.3529944451729,22.9632731486945,23.2002027400198));
#31282=CARTESIAN_POINT('Ctrl Pts',(55.3487065915121,22.9640392685493,23.2004817527859));
#31283=CARTESIAN_POINT('Ctrl Pts',(55.3381072579373,22.9658972686173,23.2011691097553));
#31284=CARTESIAN_POINT('Ctrl Pts',(55.3317928972795,22.9669728174655,23.2015765374078));
#31285=CARTESIAN_POINT('Ctrl Pts',(55.308368200945,22.9708468241331,23.2030807559671));
#31286=CARTESIAN_POINT('Ctrl Pts',(55.291226198336,22.9734526853042,23.204167241347));
#31287=CARTESIAN_POINT('Ctrl Pts',(55.2376252711634,22.9808872269974,23.2075261601569));
#31288=CARTESIAN_POINT('Ctrl Pts',(55.2010767496228,22.9849298544309,23.2097613072402));
#31289=CARTESIAN_POINT('Ctrl Pts',(55.164448305082,22.9879598379886,23.2119648302802));
#31290=CARTESIAN_POINT('Origin',(55.,21.,6.22095488139522));
#31291=CARTESIAN_POINT('',(55.1644484328881,22.9879598274162,24.1690565717028));
#31292=CARTESIAN_POINT('',(55.1644483449248,22.9879598346927,24.0089660407953));
#31293=CARTESIAN_POINT('',(55.1644483516311,22.987959834138,6.22095488139522));
#31294=CARTESIAN_POINT('Ctrl Pts',(55.1644484328881,22.9879598274162,24.1690565717028));
#31295=CARTESIAN_POINT('Ctrl Pts',(55.2278574488935,22.9827144933962,24.1653421584155));
#31296=CARTESIAN_POINT('Ctrl Pts',(55.2909969668646,22.9744369095191,24.1615920607638));
#31297=CARTESIAN_POINT('Ctrl Pts',(55.4047925019397,22.9539373158229,24.1546351819034));
#31298=CARTESIAN_POINT('Ctrl Pts',(55.4555517072851,22.9427300215604,24.1514590663388));
#31299=CARTESIAN_POINT('Ctrl Pts',(55.5191158365712,22.9260673540089,24.1473619840124));
#31300=CARTESIAN_POINT('Ctrl Pts',(55.5323825226982,22.9224425969265,24.1465002201414));
#31301=CARTESIAN_POINT('Ctrl Pts',(55.5536131967499,22.9164052844999,24.1451099885801));
#31302=CARTESIAN_POINT('Ctrl Pts',(55.5616015682748,22.9140795336627,24.1445843427756));
#31303=CARTESIAN_POINT('Ctrl Pts',(55.5767647130944,22.9095618104466,24.1435816273379));
#31304=CARTESIAN_POINT('Ctrl Pts',(55.5839421437628,22.9073791999503,24.1431048705318));
#31305=CARTESIAN_POINT('Ctrl Pts',(55.6002810082798,22.9023097901571,24.1420146380049));
#31306=CARTESIAN_POINT('Ctrl Pts',(55.6094341896089,22.8993972174951,24.1414003269731));
#31307=CARTESIAN_POINT('Ctrl Pts',(55.6332111148614,22.8916417603352,24.1397951139723));
#31308=CARTESIAN_POINT('Ctrl Pts',(55.6478002023449,22.8866954553319,24.1388008364628));
#31309=CARTESIAN_POINT('Ctrl Pts',(55.7890109192969,22.8369882496432,24.1290838788807));
#31310=CARTESIAN_POINT('Ctrl Pts',(55.9108401786786,22.7797251554187,24.1199333572215));
#31311=CARTESIAN_POINT('Ctrl Pts',(56.1181386276991,22.6553982213338,24.1031256116387));
#31312=CARTESIAN_POINT('Ctrl Pts',(56.2056874100779,22.5927637794189,24.0955716211202));
#31313=CARTESIAN_POINT('Ctrl Pts',(56.3217829935932,22.4946241422552,24.0852177535661));
#31314=CARTESIAN_POINT('Ctrl Pts',(56.3548303306389,22.4647344728215,24.0822285996259));
#31315=CARTESIAN_POINT('Ctrl Pts',(56.393189304029,22.4276305092686,24.0787353713917));
#31316=CARTESIAN_POINT('Ctrl Pts',(56.3994863396319,22.4214581597692,24.078161131154));
#31317=CARTESIAN_POINT('Ctrl Pts',(56.4092086264832,22.4118011469382,24.0772735983961));
#31318=CARTESIAN_POINT('Ctrl Pts',(56.4126622584889,22.4083454037042,24.0769581354393));
#31319=CARTESIAN_POINT('Ctrl Pts',(56.4190536744635,22.4019029145152,24.0763740425799));
#31320=CARTESIAN_POINT('Ctrl Pts',(56.4219947229854,22.3989196263637,24.076105162339));
#31321=CARTESIAN_POINT('Ctrl Pts',(56.4286784537155,22.3920970456884,24.0754938430999));
#31322=CARTESIAN_POINT('Ctrl Pts',(56.4324150654822,22.3882519189691,24.0751518762033));
#31323=CARTESIAN_POINT('Ctrl Pts',(56.4421260254281,22.378177992106,24.0742624676531));
#31324=CARTESIAN_POINT('Ctrl Pts',(56.4480756069747,22.3719253237596,24.0737168768965));
#31325=CARTESIAN_POINT('Ctrl Pts',(56.4882447178267,22.3291574504627,24.0700269729553));
#31326=CARTESIAN_POINT('Ctrl Pts',(56.5211233532755,22.2914009990119,24.0669752642144));
#31327=CARTESIAN_POINT('Ctrl Pts',(56.588221216425,22.2082254351498,24.0605778682594));
#31328=CARTESIAN_POINT('Ctrl Pts',(56.6219891695425,22.1625003741782,24.0572509093319));
#31329=CARTESIAN_POINT('Ctrl Pts',(56.7230902544962,22.0126009001958,24.046727412675));
#31330=CARTESIAN_POINT('Ctrl Pts',(56.782681589181,21.9035736458635,24.0396123859671));
#31331=CARTESIAN_POINT('Ctrl Pts',(56.8551336483146,21.7355206141634,24.0286553069179));
#31332=CARTESIAN_POINT('Ctrl Pts',(56.8760822205523,21.6803131041616,24.0250608104729));
#31333=CARTESIAN_POINT('Ctrl Pts',(56.8990300652018,21.6106694565227,24.0204924714197));
#31334=CARTESIAN_POINT('Ctrl Pts',(56.9033622962385,21.5970295855748,24.0195962418077));
#31335=CARTESIAN_POINT('Ctrl Pts',(56.9100163492697,21.575270711226,24.0181636376955));
#31336=CARTESIAN_POINT('Ctrl Pts',(56.9124340849827,21.5671813755035,24.0176304036652));
#31337=CARTESIAN_POINT('Ctrl Pts',(56.9168967570228,21.5518970309113,24.0166215907342));
#31338=CARTESIAN_POINT('Ctrl Pts',(56.9189527253857,21.5447053745374,24.0161463808844));
#31339=CARTESIAN_POINT('Ctrl Pts',(56.9235004777551,21.5284522610685,24.0150711156692));
#31340=CARTESIAN_POINT('Ctrl Pts',(56.925968756619,21.5193844661557,24.0144703096416));
#31341=CARTESIAN_POINT('Ctrl Pts',(56.9321378560755,21.4960720402998,24.0129232270118));
#31342=CARTESIAN_POINT('Ctrl Pts',(56.935745218384,21.4818034809731,24.0119739646326));
#31343=CARTESIAN_POINT('Ctrl Pts',(56.9583753609548,21.3879327638859,24.0057123054994));
#31344=CARTESIAN_POINT('Ctrl Pts',(56.9726391616497,21.3072743624777,24.00024903561));
#31345=CARTESIAN_POINT('Ctrl Pts',(56.9994110161194,21.0724741815147,23.9841229920169));
#31346=CARTESIAN_POINT('Ctrl Pts',(56.9990199022874,20.9174741845069,23.9731661659592));
#31347=CARTESIAN_POINT('Ctrl Pts',(56.9747462668238,20.7136761379846,23.9591287047738));
#31348=CARTESIAN_POINT('Ctrl Pts',(56.9668204613882,20.6635145995775,23.9557093049161));
#31349=CARTESIAN_POINT('Ctrl Pts',(56.9552215515261,20.6047538676348,23.9517864683638));
#31350=CARTESIAN_POINT('Ctrl Pts',(56.9533930810636,20.5958140289205,23.9511919427236));
#31351=CARTESIAN_POINT('Ctrl Pts',(56.9504777681279,20.5820423957456,23.9502799599097));
#31352=CARTESIAN_POINT('Ctrl Pts',(56.9494341984007,20.5772017143913,23.9499601412401));
#31353=CARTESIAN_POINT('Ctrl Pts',(56.947475845707,20.5682791521837,23.9493720669486));
#31354=CARTESIAN_POINT('Ctrl Pts',(56.9465662542278,20.564196284397,23.949103530915));
#31355=CARTESIAN_POINT('Ctrl Pts',(56.9444809133073,20.5549726428453,23.9484981256949));
#31356=CARTESIAN_POINT('Ctrl Pts',(56.9432976198474,20.5498336606666,23.9481616914997));
#31357=CARTESIAN_POINT('Ctrl Pts',(56.9401905925549,20.5365805738803,23.9472961538754));
#31358=CARTESIAN_POINT('Ctrl Pts',(56.9382363098146,20.5284736348841,23.9467687421765));
#31359=CARTESIAN_POINT('Ctrl Pts',(56.9255891212297,20.4774168997053,23.9434586574634));
#31360=CARTESIAN_POINT('Ctrl Pts',(56.9135191599593,20.4348171534066,23.9407482383574));
#31361=CARTESIAN_POINT('Ctrl Pts',(56.8411417775347,20.2083905910536,23.9264467006547));
#31362=CARTESIAN_POINT('Ctrl Pts',(56.7557530889236,20.0336707725478,23.9156868751425));
#31363=CARTESIAN_POINT('Ctrl Pts',(56.6162152604842,19.8296322137838,23.9008328584788));
#31364=CARTESIAN_POINT('Ctrl Pts',(56.58411905745,19.7865427252884,23.8975529917815));
#31365=CARTESIAN_POINT('Ctrl Pts',(56.5415794881433,19.734001016379,23.8933388227023));
#31366=CARTESIAN_POINT('Ctrl Pts',(56.5327210561125,19.7232905994466,23.8924680364628));
#31367=CARTESIAN_POINT('Ctrl Pts',(56.5183614046713,19.7062937089394,23.8910667131691));
#31368=CARTESIAN_POINT('Ctrl Pts',(56.5129312641996,19.6999475744826,23.8905390800347));
#31369=CARTESIAN_POINT('Ctrl Pts',(56.5025527829702,19.6879714648255,23.8895348209119));
#31370=CARTESIAN_POINT('Ctrl Pts',(56.4976122401817,19.6823348990479,23.889058522703));
#31371=CARTESIAN_POINT('Ctrl Pts',(56.486306265171,19.6695818664444,23.8879724688984));
#31372=CARTESIAN_POINT('Ctrl Pts',(56.4799213074308,19.6624830309295,23.887361901486));
#31373=CARTESIAN_POINT('Ctrl Pts',(56.4632312175164,19.6441927101101,23.8857728661002));
#31374=CARTESIAN_POINT('Ctrl Pts',(56.4528487337648,19.6330729577827,23.8847911332849));
#31375=CARTESIAN_POINT('Ctrl Pts',(56.3753215541541,19.5519216336571,23.8775082774481));
#31376=CARTESIAN_POINT('Ctrl Pts',(56.3032845171955,19.4867634763132,23.8709921160163));
#31377=CARTESIAN_POINT('Ctrl Pts',(56.1161180437961,19.3407795540519,23.8546778573428));
#31378=CARTESIAN_POINT('Ctrl Pts',(55.9966356774817,19.2663774826738,23.8447423161791));
#31379=CARTESIAN_POINT('Ctrl Pts',(55.8263437290236,19.1838023112513,23.8318135817867));
#31380=CARTESIAN_POINT('Ctrl Pts',(55.781577161115,19.1640925862992,23.8285237373053));
#31381=CARTESIAN_POINT('Ctrl Pts',(55.7277274570382,19.1427111163859,23.8247296097404));
#31382=CARTESIAN_POINT('Ctrl Pts',(55.7193045762337,19.1394328329818,23.8241407984635));
#31383=CARTESIAN_POINT('Ctrl Pts',(55.7062501622968,19.1344538044945,23.8232356970498));
#31384=CARTESIAN_POINT('Ctrl Pts',(55.7016342434948,19.1327128531093,23.8229170999324));
#31385=CARTESIAN_POINT('Ctrl Pts',(55.6930911279522,19.129526861767,23.822330159734));
#31386=CARTESIAN_POINT('Ctrl Pts',(55.6891658669211,19.1280770633056,23.8220615446272));
#31387=CARTESIAN_POINT('Ctrl Pts',(55.6802611863933,19.1248199179019,23.8214545596043));
#31388=CARTESIAN_POINT('Ctrl Pts',(55.6752791197591,19.1230200496571,23.8211166346995));
#31389=CARTESIAN_POINT('Ctrl Pts',(55.6604516622494,19.1177300207326,23.8201157222406));
#31390=CARTESIAN_POINT('Ctrl Pts',(55.6505857806225,19.1142972593132,23.8194560176971));
#31391=CARTESIAN_POINT('Ctrl Pts',(55.5527629968044,19.081119671006,23.812972578089));
#31392=CARTESIAN_POINT('Ctrl Pts',(55.4628453582455,19.0574687940955,23.8074703932382));
#31393=CARTESIAN_POINT('Ctrl Pts',(55.2401361014388,19.0152417635003,23.7942293860894));
#31394=CARTESIAN_POINT('Ctrl Pts',(55.1065074718338,19.0036067714459,23.7865885659887));
#31395=CARTESIAN_POINT('Ctrl Pts',(54.9114044695047,19.0062751445912,23.774923801163));
#31396=CARTESIAN_POINT('Ctrl Pts',(54.8501646632438,19.0099406494272,23.7711936969204));
#31397=CARTESIAN_POINT('Ctrl Pts',(54.7748004241117,19.0179499861071,23.7664730489652));
#31398=CARTESIAN_POINT('Ctrl Pts',(54.7604232368745,19.0196363809469,23.7655666746434));
#31399=CARTESIAN_POINT('Ctrl Pts',(54.7376559337581,19.0225584592186,23.7641215996191));
#31400=CARTESIAN_POINT('Ctrl Pts',(54.729252971863,19.0236914462918,23.7635861358629));
#31401=CARTESIAN_POINT('Ctrl Pts',(54.7134563790515,19.0259239660321,23.7625754347905));
#31402=CARTESIAN_POINT('Ctrl Pts',(54.7060611874405,19.0270115543746,23.7621005826464));
#31403=CARTESIAN_POINT('Ctrl Pts',(54.689437101637,19.0295519467769,23.7610292473917));
#31404=CARTESIAN_POINT('Ctrl Pts',(54.6802119996413,19.0310280666782,23.7604320361217));
#31405=CARTESIAN_POINT('Ctrl Pts',(54.6566608028872,19.0349663988157,23.758900323075));
#31406=CARTESIAN_POINT('Ctrl Pts',(54.6423508304461,19.0375204686403,23.7579629348897));
#31407=CARTESIAN_POINT('Ctrl Pts',(54.5523804517107,19.0545952589935,23.7520259440463));
#31408=CARTESIAN_POINT('Ctrl Pts',(54.4775957104705,19.0733308455812,23.7468933019434));
#31409=CARTESIAN_POINT('Ctrl Pts',(54.2522767857922,19.143863454152,23.7308232857337));
#31410=CARTESIAN_POINT('Ctrl Pts',(54.1067121862988,19.2093681438856,23.7195359005349));
#31411=CARTESIAN_POINT('Ctrl Pts',(53.9409992303602,19.3092221894913,23.7062986631718));
#31412=CARTESIAN_POINT('Ctrl Pts',(53.9119815592086,19.327747511516,23.7039675298469));
#31413=CARTESIAN_POINT('Ctrl Pts',(53.8659769094769,19.3588223373338,23.700266963215));
#31414=CARTESIAN_POINT('Ctrl Pts',(53.8486850809592,19.3709062231818,23.6988749161295));
#31415=CARTESIAN_POINT('Ctrl Pts',(53.8259913050678,19.3873069669499,23.6970499228626));
#31416=CARTESIAN_POINT('Ctrl Pts',(53.8204161690311,19.391380335896,23.696601738528));
#31417=CARTESIAN_POINT('Ctrl Pts',(53.8112719332227,19.3981345037371,23.695867048822));
#31418=CARTESIAN_POINT('Ctrl Pts',(53.8076905369639,19.4007984397911,23.6955794085762));
#31419=CARTESIAN_POINT('Ctrl Pts',(53.800686911998,19.4060445245249,23.6950171684617));
#31420=CARTESIAN_POINT('Ctrl Pts',(53.7972640259651,19.408625713999,23.6947425086883));
#31421=CARTESIAN_POINT('Ctrl Pts',(53.7888524726667,19.4150114857118,23.6940677826427));
#31422=CARTESIAN_POINT('Ctrl Pts',(53.7838733285206,19.4188286478513,23.693668589046));
#31423=CARTESIAN_POINT('Ctrl Pts',(53.7668232401048,19.4320279439866,23.6923020152519));
#31424=CARTESIAN_POINT('Ctrl Pts',(53.7548418393424,19.4415255927732,23.6913423672132));
#31425=CARTESIAN_POINT('Ctrl Pts',(53.6411844700034,19.5337692810685,23.6822325650844));
#31426=CARTESIAN_POINT('Ctrl Pts',(53.5477744287519,19.6262231051083,23.6746820892311));
#31427=CARTESIAN_POINT('Ctrl Pts',(53.4010029422945,19.80333143732,23.6613359711608));
#31428=CARTESIAN_POINT('Ctrl Pts',(53.3436546888174,19.8840585072693,23.6555854122675));
#31429=CARTESIAN_POINT('Ctrl Pts',(53.2656466113675,20.0132122387942,23.6465075020604));
#31430=CARTESIAN_POINT('Ctrl Pts',(53.2405141277928,20.0587558673,23.6433292366863));
#31431=CARTESIAN_POINT('Ctrl Pts',(53.2110205619976,20.1175209015712,23.6392297264973));
#31432=CARTESIAN_POINT('Ctrl Pts',(53.2049775993265,20.129878540189,23.6383677722817));
#31433=CARTESIAN_POINT('Ctrl Pts',(53.1954852936865,20.1498097436006,23.6369773067224));
#31434=CARTESIAN_POINT('Ctrl Pts',(53.1919546220124,20.1573442546834,23.6364516189851));
#31435=CARTESIAN_POINT('Ctrl Pts',(53.1853306042956,20.1717133199875,23.6354488713851));
#31436=CARTESIAN_POINT('Ctrl Pts',(53.1822284648573,20.1785436813219,23.6349721246668));
#31437=CARTESIAN_POINT('Ctrl Pts',(53.1752428417722,20.1941581319422,23.6338819823226));
#31438=CARTESIAN_POINT('Ctrl Pts',(53.1713841449312,20.2029530427416,23.6332677518921));
#31439=CARTESIAN_POINT('Ctrl Pts',(53.1615036610038,20.2259225170042,23.6316628877564));
#31440=CARTESIAN_POINT('Ctrl Pts',(53.1555823418622,20.2401393427404,23.630668880916));
#31441=CARTESIAN_POINT('Ctrl Pts',(53.1108661960963,20.3511039136503,23.6229036393757));
#31442=CARTESIAN_POINT('Ctrl Pts',(53.0795501588148,20.4506741312491,23.6158825461797));
#31443=CARTESIAN_POINT('Ctrl Pts',(53.0222733386474,20.6993170214271,23.5982938948018));
#31444=CARTESIAN_POINT('Ctrl Pts',(53.0051951726877,20.8497790334131,23.5875816050759));
#31445=CARTESIAN_POINT('Ctrl Pts',(53.005261785231,21.0327320230545,23.5752406874897));
#31446=CARTESIAN_POINT('Ctrl Pts',(53.006043736852,21.0647350499803,23.5731092580746));
#31447=CARTESIAN_POINT('Ctrl Pts',(53.0079957634069,21.1049514524451,23.5704762816586));
#31448=CARTESIAN_POINT('Ctrl Pts',(53.0084470821659,21.1131930525887,23.5699391113804));
#31449=CARTESIAN_POINT('Ctrl Pts',(53.009242377354,21.1262330720561,23.5690932542597));
#31450=CARTESIAN_POINT('Ctrl Pts',(53.0095525719062,21.1310333460878,23.5687827508951));
#31451=CARTESIAN_POINT('Ctrl Pts',(53.0101374746282,21.1396029183349,23.5682300468477));
#31452=CARTESIAN_POINT('Ctrl Pts',(53.0104055281421,21.1433725307798,23.5679874849649));
#31453=CARTESIAN_POINT('Ctrl Pts',(53.0110713778308,21.1523746519575,23.5674095525719));
#31454=CARTESIAN_POINT('Ctrl Pts',(53.0114791093999,21.1576063698247,23.5670747413607));
#31455=CARTESIAN_POINT('Ctrl Pts',(53.0127685049821,21.1733487731796,23.5660703202624));
#31456=CARTESIAN_POINT('Ctrl Pts',(53.0137129091456,21.1838543340842,23.5654041048098));
#31457=CARTESIAN_POINT('Ctrl Pts',(53.0160838316053,21.2080727197732,23.5638766749151));
#31458=CARTESIAN_POINT('Ctrl Pts',(53.0175692827296,21.2217793815065,23.5630184267433));
#31459=CARTESIAN_POINT('Ctrl Pts',(53.0230946135337,21.2682591687343,23.5601258665221));
#31460=CARTESIAN_POINT('Ctrl Pts',(53.0278062533681,21.3009484349768,23.5581215919491));
#31461=CARTESIAN_POINT('Ctrl Pts',(53.0572521287678,21.4745889248671,23.5475650709058));
#31462=CARTESIAN_POINT('Ctrl Pts',(53.0962890070089,21.6126940982866,23.5394588729822));
#31463=CARTESIAN_POINT('Ctrl Pts',(53.1849082253035,21.8326523066063,23.5255368170095));
#31464=CARTESIAN_POINT('Ctrl Pts',(53.2261626605271,21.9172599176625,23.5199133766742));
#31465=CARTESIAN_POINT('Ctrl Pts',(53.280798575232,22.0117326111282,23.5131361117721));
#31466=CARTESIAN_POINT('Ctrl Pts',(53.2885206459475,22.0247413411533,23.5121915451495));
#31467=CARTESIAN_POINT('Ctrl Pts',(53.3013431448295,22.0457930588591,23.5106437142266));
#31468=CARTESIAN_POINT('Ctrl Pts',(53.3063546173168,22.0538897220427,23.5100436910415));
#31469=CARTESIAN_POINT('Ctrl Pts',(53.3154125996122,22.0682925584727,23.508967720244));
#31470=CARTESIAN_POINT('Ctrl Pts',(53.3194370575568,22.0746124389834,23.5084925927916));
#31471=CARTESIAN_POINT('Ctrl Pts',(53.3280309105786,22.0879416043895,23.5074840631513));
#31472=CARTESIAN_POINT('Ctrl Pts',(53.3326089827357,22.094945095688,23.5069503439587));
#31473=CARTESIAN_POINT('Ctrl Pts',(53.3449460588823,22.1135614364283,23.5055213031828));
#31474=CARTESIAN_POINT('Ctrl Pts',(53.3527830799339,22.1251217811847,23.5046230642647));
#31475=CARTESIAN_POINT('Ctrl Pts',(53.3918170533879,22.1814185269128,23.5001944631864));
#31476=CARTESIAN_POINT('Ctrl Pts',(53.4247157217733,22.2249410664469,23.496599630525));
#31477=CARTESIAN_POINT('Ctrl Pts',(53.5879716613595,22.4234479175594,23.4793616150222));
#31478=CARTESIAN_POINT('Ctrl Pts',(53.7396201366567,22.5593100336184,23.4648613802283));
#31479=CARTESIAN_POINT('Ctrl Pts',(53.9387495259889,22.6893873506059,23.4487685603017));
#31480=CARTESIAN_POINT('Ctrl Pts',(53.9689168893588,22.7079666787367,23.4464040526565));
#31481=CARTESIAN_POINT('Ctrl Pts',(54.0069558825313,22.7300184746869,23.4435270539493));
#31482=CARTESIAN_POINT('Ctrl Pts',(54.0143741946855,22.7342555521636,23.442970808694));
#31483=CARTESIAN_POINT('Ctrl Pts',(54.0260697310895,22.740836343767,23.4421016689838));
#31484=CARTESIAN_POINT('Ctrl Pts',(54.0303286156587,22.7432121936547,23.4417867920909));
#31485=CARTESIAN_POINT('Ctrl Pts',(54.0382631453654,22.7476004532246,23.4412032210433));
#31486=CARTESIAN_POINT('Ctrl Pts',(54.0419363883678,22.7496168832681,23.4409342806353));
#31487=CARTESIAN_POINT('Ctrl Pts',(54.0503352261351,22.7541930514267,23.440322103096));
#31488=CARTESIAN_POINT('Ctrl Pts',(54.055064824387,22.756745274623,23.4399793433694));
#31489=CARTESIAN_POINT('Ctrl Pts',(54.0696717109687,22.7645515010465,23.438926651256));
#31490=CARTESIAN_POINT('Ctrl Pts',(54.0795831320692,22.7697416557472,23.4382206125345));
#31491=CARTESIAN_POINT('Ctrl Pts',(54.1832465969071,22.8229189610767,23.4309163007775));
#31492=CARTESIAN_POINT('Ctrl Pts',(54.2806292909887,22.8634998689112,23.4247290155489));
#31493=CARTESIAN_POINT('Ctrl Pts',(54.5407342649076,22.9484400449457,23.4088071670829));
#31494=CARTESIAN_POINT('Ctrl Pts',(54.7066419119843,22.9802219036377,23.3991702876915));
#31495=CARTESIAN_POINT('Ctrl Pts',(54.8950816066056,22.9920949487837,23.3875241719794));
#31496=CARTESIAN_POINT('Ctrl Pts',(54.9156160984686,22.993070360752,23.3862470066826));
#31497=CARTESIAN_POINT('Ctrl Pts',(54.947221891206,22.9940823686731,23.3842671893001));
#31498=CARTESIAN_POINT('Ctrl Pts',(54.9582849293128,22.9943444704469,23.3835715464159));
#31499=CARTESIAN_POINT('Ctrl Pts',(54.9763192271522,22.9946216115993,23.3824330168959));
#31500=CARTESIAN_POINT('Ctrl Pts',(54.983289494628,22.9946921841389,23.3819918711408));
#31501=CARTESIAN_POINT('Ctrl Pts',(54.9979353102157,22.9947636984397,23.3810625599421));
#31502=CARTESIAN_POINT('Ctrl Pts',(55.005610765536,22.9947568754515,23.3805741593405));
#31503=CARTESIAN_POINT('Ctrl Pts',(55.0239895699,22.9946344619003,23.3794013085571));
#31504=CARTESIAN_POINT('Ctrl Pts',(55.0346923124084,22.9944770171974,23.3787155625139));
#31505=CARTESIAN_POINT('Ctrl Pts',(55.0714859441515,22.9936395139523,23.3763483885824));
#31506=CARTESIAN_POINT('Ctrl Pts',(55.0975635324336,22.9925335635314,23.3746537710115));
#31507=CARTESIAN_POINT('Ctrl Pts',(55.1372340497878,22.9900705221096,23.3720489315753));
#31508=CARTESIAN_POINT('Ctrl Pts',(55.1508472364672,22.9890849479159,23.371150237346));
#31509=CARTESIAN_POINT('Ctrl Pts',(55.1644483538502,22.9879598339544,23.3702474674336));
#31510=CARTESIAN_POINT('',(53.0052508822312,20.9981658358939,23.4208211887813));
#31511=CARTESIAN_POINT('Ctrl Pts',(55.164448305082,22.9879598379886,23.2119648302802));
#31512=CARTESIAN_POINT('Ctrl Pts',(55.0991263259238,22.9933634123224,23.2158945217506));
#31513=CARTESIAN_POINT('Ctrl Pts',(55.033550205288,22.9955463711911,23.2197243986835));
#31514=CARTESIAN_POINT('Ctrl Pts',(54.8064007976559,22.9918972263633,23.2329283338445));
#31515=CARTESIAN_POINT('Ctrl Pts',(54.6457766981688,22.9696839662503,23.2422120601349));
#31516=CARTESIAN_POINT('Ctrl Pts',(54.4673973487199,22.9224695711337,23.2535861794245));
#31517=CARTESIAN_POINT('Ctrl Pts',(54.4453031849839,22.9162114214996,23.255013042448));
#31518=CARTESIAN_POINT('Ctrl Pts',(54.4143219137268,22.9068553022161,23.2570415141568));
#31519=CARTESIAN_POINT('Ctrl Pts',(54.4053406240195,22.9040735768447,23.2576328608777));
#31520=CARTESIAN_POINT('Ctrl Pts',(54.3897167567491,22.8991131592788,23.2586674900303));
#31521=CARTESIAN_POINT('Ctrl Pts',(54.3830652918374,22.896962833737,23.2591098385876));
#31522=CARTESIAN_POINT('Ctrl Pts',(54.3691560836983,22.8923852887287,23.2600388683995));
#31523=CARTESIAN_POINT('Ctrl Pts',(54.3619007440387,22.8899511804784,23.2605257701469));
#31524=CARTESIAN_POINT('Ctrl Pts',(54.3448392418368,22.8841177400253,23.2616762730441));
#31525=CARTESIAN_POINT('Ctrl Pts',(54.3350453223651,22.8806835319282,23.2623410176298));
#31526=CARTESIAN_POINT('Ctrl Pts',(54.3023860367182,22.8689446505354,23.2645724311521));
#31527=CARTESIAN_POINT('Ctrl Pts',(54.2796465986697,22.8602984273747,23.2661503723539));
#31528=CARTESIAN_POINT('Ctrl Pts',(54.2255913825251,22.8386053073891,23.2699615121339));
#31529=CARTESIAN_POINT('Ctrl Pts',(54.1944400246391,22.8251715215852,23.2722070828989));
#31530=CARTESIAN_POINT('Ctrl Pts',(54.0064537875455,22.7383537477567,23.2860635705158));
#31531=CARTESIAN_POINT('Ctrl Pts',(53.8593935104238,22.645602571587,23.2983126821385));
#31532=CARTESIAN_POINT('Ctrl Pts',(53.7108572168926,22.522345275487,23.3116270570718));
#31533=CARTESIAN_POINT('Ctrl Pts',(53.6957209447134,22.5093973756668,23.3129950026004));
#31534=CARTESIAN_POINT('Ctrl Pts',(53.6454872049498,22.4651063562734,23.3175666527756));
#31535=CARTESIAN_POINT('Ctrl Pts',(53.6113024340647,22.4327461086395,23.3207313592904));
#31536=CARTESIAN_POINT('Ctrl Pts',(53.5723411889971,22.3931582258712,23.3243713105746));
#31537=CARTESIAN_POINT('Ctrl Pts',(53.5664293799758,22.3870741892434,23.3249245546237));
#31538=CARTESIAN_POINT('Ctrl Pts',(53.5568760678426,22.3771162408892,23.3258198323081));
#31539=CARTESIAN_POINT('Ctrl Pts',(53.5532109955784,22.373265233944,23.3261636043928));
#31540=CARTESIAN_POINT('Ctrl Pts',(53.5466885654262,22.366356815639,23.3267758573086));
#31541=CARTESIAN_POINT('Ctrl Pts',(53.543825398956,22.3633050303755,23.3270447783194));
#31542=CARTESIAN_POINT('Ctrl Pts',(53.5376195220838,22.3566484684455,23.3276279994759));
#31543=CARTESIAN_POINT('Ctrl Pts',(53.5342805319479,22.3530403435809,23.3279420189467));
#31544=CARTESIAN_POINT('Ctrl Pts',(53.5274159744056,22.345567247119,23.3285881636097));
#31545=CARTESIAN_POINT('Ctrl Pts',(53.523892199814,22.341700671773,23.3289201560256));
#31546=CARTESIAN_POINT('Ctrl Pts',(53.5071018741299,22.3231307322401,23.3305037943368));
#31547=CARTESIAN_POINT('Ctrl Pts',(53.4940390116084,22.3082436013264,23.3317410915564));
#31548=CARTESIAN_POINT('Ctrl Pts',(53.4286731284674,22.2314723959766,23.3379744079782));
#31549=CARTESIAN_POINT('Ctrl Pts',(53.3799484704837,22.1666311447625,23.3427627309584));
#31550=CARTESIAN_POINT('Ctrl Pts',(53.2937774319601,22.0361042220352,23.3518940304228));
#31551=CARTESIAN_POINT('Ctrl Pts',(53.2558531578978,21.970906465801,23.3562377114781));
#31552=CARTESIAN_POINT('Ctrl Pts',(53.1703758829508,21.8027087107385,23.3672401135191));
#31553=CARTESIAN_POINT('Ctrl Pts',(53.1277492439044,21.6975225571349,23.3739531089497));
#31554=CARTESIAN_POINT('Ctrl Pts',(53.0896975623514,21.5744676285229,23.3819476488903));
#31555=CARTESIAN_POINT('Ctrl Pts',(53.085285662596,21.5595868515015,23.3829163660343));
#31556=CARTESIAN_POINT('Ctrl Pts',(53.078416135962,21.5353839016736,23.3844957994014));
#31557=CARTESIAN_POINT('Ctrl Pts',(53.0758515948601,21.5260925569232,23.385103045895));
#31558=CARTESIAN_POINT('Ctrl Pts',(53.0714104344116,21.5095352404554,23.3861869462143));
#31559=CARTESIAN_POINT('Ctrl Pts',(53.0695072758501,21.5022765306617,23.3866627314725));
#31560=CARTESIAN_POINT('Ctrl Pts',(53.065585955783,21.4869689153054,23.3876674457245));
#31561=CARTESIAN_POINT('Ctrl Pts',(53.063576975258,21.4789178267269,23.3881966606351));
#31562=CARTESIAN_POINT('Ctrl Pts',(53.0595976188397,21.4625358849382,23.3892751560575));
#31563=CARTESIAN_POINT('Ctrl Pts',(53.0576305228776,21.4542044211841,23.3898245298029));
#31564=CARTESIAN_POINT('Ctrl Pts',(53.0528834004297,21.4335034497103,23.3911918184686));
#31565=CARTESIAN_POINT('Ctrl Pts',(53.0501675871054,21.4211197484581,23.3920117646553));
#31566=CARTESIAN_POINT('Ctrl Pts',(53.0193000797086,21.2736644283603,23.4018000996712));
#31567=CARTESIAN_POINT('Ctrl Pts',(53.0051240058792,21.1360799458073,23.4112224742061));
#31568=CARTESIAN_POINT('Ctrl Pts',(53.0052508435975,20.9981654614968,23.4208211472388));
#31569=CARTESIAN_POINT('Ctrl Pts',(53.0052508432575,20.9981658311762,23.4208211215096));
#31570=CARTESIAN_POINT('Ctrl Pts',(53.005371052201,20.867432669888,23.429919983384));
#31571=CARTESIAN_POINT('Ctrl Pts',(53.0183428780867,20.7370158548825,23.4391245158));
#31572=CARTESIAN_POINT('Ctrl Pts',(53.0466488227188,20.5954867718677,23.4487342893852));
#31573=CARTESIAN_POINT('Ctrl Pts',(53.049446452778,20.5822050079215,23.4496321051015));
#31574=CARTESIAN_POINT('Ctrl Pts',(53.0539722639705,20.5617558432602,23.4510071637296));
#31575=CARTESIAN_POINT('Ctrl Pts',(53.0556049194828,20.554568001693,23.4514891040053));
#31576=CARTESIAN_POINT('Ctrl Pts',(53.0587334361215,20.5411395979358,23.4523866575698));
#31577=CARTESIAN_POINT('Ctrl Pts',(53.0602196369505,20.5348969076754,23.4528027775369));
#31578=CARTESIAN_POINT('Ctrl Pts',(53.0627657417058,20.5244266783544,23.4534986499897));
#31579=CARTESIAN_POINT('Ctrl Pts',(53.0638094117212,20.5201952868669,23.4537793147855));
#31580=CARTESIAN_POINT('Ctrl Pts',(53.0658157386696,20.5121741150133,23.4543102414826));
#31581=CARTESIAN_POINT('Ctrl Pts',(53.0667756814197,20.508383700906,23.4545606613191));
#31582=CARTESIAN_POINT('Ctrl Pts',(53.0693209400191,20.4984562778836,23.4552153582743));
#31583=CARTESIAN_POINT('Ctrl Pts',(53.0709243878838,20.4923238993149,23.4556186002173));
#31584=CARTESIAN_POINT('Ctrl Pts',(53.0765961963292,20.4710470028298,23.4570139235789));
#31585=CARTESIAN_POINT('Ctrl Pts',(53.0808140084591,20.4559424377483,23.4579978295762));
#31586=CARTESIAN_POINT('Ctrl Pts',(53.1195845986196,20.3231646828597,23.4666009701352));
#31587=CARTESIAN_POINT('Ctrl Pts',(53.1647481064187,20.2088445237748,23.4736985692407));
#31588=CARTESIAN_POINT('Ctrl Pts',(53.2674181349835,20.0059399127586,23.4868916015663));
#31589=CARTESIAN_POINT('Ctrl Pts',(53.3219852286993,19.9163673527866,23.4929621066318));
#31590=CARTESIAN_POINT('Ctrl Pts',(53.4147887694859,19.7879697122599,23.5024816549071));
#31591=CARTESIAN_POINT('Ctrl Pts',(53.4479927339966,19.7457333883856,23.5057610696224));
#31592=CARTESIAN_POINT('Ctrl Pts',(53.4916360087646,19.694607944774,23.5099510742376));
#31593=CARTESIAN_POINT('Ctrl Pts',(53.5005180065553,19.6844149267343,23.5107979351905));
#31594=CARTESIAN_POINT('Ctrl Pts',(53.5151292380655,19.6679872155712,23.5121820733801));
#31595=CARTESIAN_POINT('Ctrl Pts',(53.5207958575069,19.6616972170761,23.512716736701));
#31596=CARTESIAN_POINT('Ctrl Pts',(53.5315400455793,19.6499226747893,23.5137265888208));
#31597=CARTESIAN_POINT('Ctrl Pts',(53.5366087460332,19.6444302094296,23.5142013972969));
#31598=CARTESIAN_POINT('Ctrl Pts',(53.5480913277272,19.6321270923832,23.5152735186442));
#31599=CARTESIAN_POINT('Ctrl Pts',(53.5545224612008,19.6253328534108,23.515871565598));
#31600=CARTESIAN_POINT('Ctrl Pts',(53.5711000115471,19.6080642820284,23.5174071497393));
#31601=CARTESIAN_POINT('Ctrl Pts',(53.5813137887221,19.5976556645577,23.5183475994617));
#31602=CARTESIAN_POINT('Ctrl Pts',(53.6471344163324,19.5320344761336,23.5243736180764));
#31603=CARTESIAN_POINT('Ctrl Pts',(53.7058330721819,19.4800337815536,23.5295970182413));
#31604=CARTESIAN_POINT('Ctrl Pts',(53.8835586632631,19.340361215746,23.5449932789214));
#31605=CARTESIAN_POINT('Ctrl Pts',(54.009461454125,19.2622804117087,23.5554417793021));
#31606=CARTESIAN_POINT('Ctrl Pts',(54.196287797516,19.1733686297209,23.5696734898399));
#31607=CARTESIAN_POINT('Ctrl Pts',(54.2508807079937,19.1503088936273,23.5736876174422));
#31608=CARTESIAN_POINT('Ctrl Pts',(54.3159176450354,19.1261906675119,23.5782411913554));
#31609=CARTESIAN_POINT('Ctrl Pts',(54.3254380311283,19.122742360948,23.5789021393181));
#31610=CARTESIAN_POINT('Ctrl Pts',(54.3399674139916,19.1176045893399,23.5799018568847));
#31611=CARTESIAN_POINT('Ctrl Pts',(54.3449573827806,19.1158623543236,23.5802435969681));
#31612=CARTESIAN_POINT('Ctrl Pts',(54.3539085058441,19.1127769508369,23.5808536763409));
#31613=CARTESIAN_POINT('Ctrl Pts',(54.3578670000827,19.1114263933958,23.5811224425567));
#31614=CARTESIAN_POINT('Ctrl Pts',(54.366509826161,19.1085079535311,23.5817070019089));
#31615=CARTESIAN_POINT('Ctrl Pts',(54.3711957356444,19.1069450191265,23.582022503755));
#31616=CARTESIAN_POINT('Ctrl Pts',(54.3842672039095,19.1026390627224,23.5828987500165));
#31617=CARTESIAN_POINT('Ctrl Pts',(54.3926653501125,19.0999342031445,23.5834573121264));
#31618=CARTESIAN_POINT('Ctrl Pts',(54.4385349907675,19.0854957903425,23.5864855465748));
#31619=CARTESIAN_POINT('Ctrl Pts',(54.476331523129,19.0748140009854,23.5888990327003));
#31620=CARTESIAN_POINT('Ctrl Pts',(54.7069281786897,19.0169393383591,23.6032698149354));
#31621=CARTESIAN_POINT('Ctrl Pts',(54.9055766203397,18.997621295714,23.6142784303345));
#31622=CARTESIAN_POINT('Ctrl Pts',(55.1579398194784,19.0107742513284,23.629458874477));
#31623=CARTESIAN_POINT('Ctrl Pts',(55.2119142849729,19.0157984969555,23.6327671060513));
#31624=CARTESIAN_POINT('Ctrl Pts',(55.2794252266827,19.0248687892531,23.6370130942451));
#31625=CARTESIAN_POINT('Ctrl Pts',(55.2932163898071,19.0268690134407,23.6378861250292));
#31626=CARTESIAN_POINT('Ctrl Pts',(55.3152443075999,19.030299906895,23.6392901085783));
#31627=CARTESIAN_POINT('Ctrl Pts',(55.3234951524013,19.0316381650779,23.639818136255));
#31628=CARTESIAN_POINT('Ctrl Pts',(55.3391242880388,19.0342740780151,23.6408225307277));
#31629=CARTESIAN_POINT('Ctrl Pts',(55.3465041732239,19.0355615208083,23.6412985658234));
#31630=CARTESIAN_POINT('Ctrl Pts',(55.3632547980467,19.0385810432972,23.6423831653956));
#31631=CARTESIAN_POINT('Ctrl Pts',(55.372620674372,19.0403387538053,23.6429925348494));
#31632=CARTESIAN_POINT('Ctrl Pts',(55.3968498090622,19.0450658525299,23.6445767121868));
#31633=CARTESIAN_POINT('Ctrl Pts',(55.4116922382151,19.048137614523,23.6455547533047));
#31634=CARTESIAN_POINT('Ctrl Pts',(55.5194257096349,19.0717174066035,23.6527106456975));
#31635=CARTESIAN_POINT('Ctrl Pts',(55.6107655960914,19.0986748134007,23.6590948769539));
#31636=CARTESIAN_POINT('Ctrl Pts',(55.8329023582963,19.1818974140789,23.6753852741072));
#31637=CARTESIAN_POINT('Ctrl Pts',(55.9602640737285,19.2458296468731,23.6854467049082));
#31638=CARTESIAN_POINT('Ctrl Pts',(56.1210638884837,19.3493462861587,23.698512928518));
#31639=CARTESIAN_POINT('Ctrl Pts',(56.1613863401268,19.3774635310095,23.7018196737397));
#31640=CARTESIAN_POINT('Ctrl Pts',(56.2078578281129,19.4124897192678,23.7056304951447));
#31641=CARTESIAN_POINT('Ctrl Pts',(56.2150461634527,19.4179847495933,23.7062199470105));
#31642=CARTESIAN_POINT('Ctrl Pts',(56.2260967556087,19.4265519846505,23.7071257625892));
#31643=CARTESIAN_POINT('Ctrl Pts',(56.229985307592,19.4295898448149,23.7074444397174));
#31644=CARTESIAN_POINT('Ctrl Pts',(56.2371493546468,19.4352295585967,23.7080313654027));
#31645=CARTESIAN_POINT('Ctrl Pts',(56.2404279189602,19.4378272699812,23.7082998870417));
#31646=CARTESIAN_POINT('Ctrl Pts',(56.2478358076809,19.4437348027416,23.7089064506153));
#31647=CARTESIAN_POINT('Ctrl Pts',(56.2519601409186,19.4470507496263,23.7092440493147));
#31648=CARTESIAN_POINT('Ctrl Pts',(56.2641702926548,19.4569479191527,23.710243369011));
#31649=CARTESIAN_POINT('Ctrl Pts',(56.2722179154558,19.4635762824884,23.7109018214867));
#31650=CARTESIAN_POINT('Ctrl Pts',(56.3470576451503,19.5262086915572,23.7170273620546));
#31651=CARTESIAN_POINT('Ctrl Pts',(56.4101725284991,19.5864786758345,23.7222115284933));
#31652=CARTESIAN_POINT('Ctrl Pts',(56.5729915112007,19.7637586484671,23.7363018894857));
#31653=CARTESIAN_POINT('Ctrl Pts',(56.6634305585103,19.8884277457925,23.7450290716835));
#31654=CARTESIAN_POINT('Ctrl Pts',(56.7546244847892,20.0505902900363,23.7562453171472));
#31655=CARTESIAN_POINT('Ctrl Pts',(56.769873829009,20.0793304943032,23.7582263709569));
#31656=CARTESIAN_POINT('Ctrl Pts',(56.7950144539179,20.1296476191352,23.7616925939171));
#31657=CARTESIAN_POINT('Ctrl Pts',(56.8052362314239,20.1510522802272,23.7631664351786));
#31658=CARTESIAN_POINT('Ctrl Pts',(56.8193470948104,20.1820086379003,23.7652993706655));
#31659=CARTESIAN_POINT('Ctrl Pts',(56.823547836053,20.1914166690451,23.7659477745376));
#31660=CARTESIAN_POINT('Ctrl Pts',(56.8307211482963,20.2078223453816,23.7670789572054));
#31661=CARTESIAN_POINT('Ctrl Pts',(56.8337269736865,20.2148052836009,23.7675605912004));
#31662=CARTESIAN_POINT('Ctrl Pts',(56.839445028349,20.2283010164013,23.7684918066029));
#31663=CARTESIAN_POINT('Ctrl Pts',(56.8421627724346,20.2348113622403,23.7689411920937));
#31664=CARTESIAN_POINT('Ctrl Pts',(56.8485195897429,20.250269255431,23.7700086545812));
#31665=CARTESIAN_POINT('Ctrl Pts',(56.8521282942499,20.2592290237748,23.7706277455539));
#31666=CARTESIAN_POINT('Ctrl Pts',(56.8646507435292,20.2909836236564,23.7728233843142));
#31667=CARTESIAN_POINT('Ctrl Pts',(56.8732095814058,20.3139151707046,23.7744117117489));
#31668=CARTESIAN_POINT('Ctrl Pts',(56.9388318215794,20.5001256640484,23.7873367104232));
#31669=CARTESIAN_POINT('Ctrl Pts',(56.974848418882,20.6700102735432,23.7993922282362));
#31670=CARTESIAN_POINT('Ctrl Pts',(56.9962064607337,20.9394302046381,23.8182155831398));
#31671=CARTESIAN_POINT('Ctrl Pts',(56.9967845640676,21.0369432146682,23.8249461261145));
#31672=CARTESIAN_POINT('Ctrl Pts',(56.989476557572,21.1453898907522,23.8320931520076));
#31673=CARTESIAN_POINT('Ctrl Pts',(56.9886212060638,21.1566553749929,23.8328314151003));
#31674=CARTESIAN_POINT('Ctrl Pts',(56.9872160641331,21.1732887136987,23.8339146870059));
#31675=CARTESIAN_POINT('Ctrl Pts',(56.9867401520251,21.1786623458717,23.8342636085846));
#31676=CARTESIAN_POINT('Ctrl Pts',(56.9858592710022,21.1881695169784,23.834879001847));
#31677=CARTESIAN_POINT('Ctrl Pts',(56.985463186857,21.1923037860004,23.8351459607402));
#31678=CARTESIAN_POINT('Ctrl Pts',(56.9845770513471,21.201258452546,23.835722761078));
#31679=CARTESIAN_POINT('Ctrl Pts',(56.9840823497504,21.2060783056769,23.8360323399815));
#31680=CARTESIAN_POINT('Ctrl Pts',(56.9826810465643,21.2192581583034,23.8368765789452));
#31681=CARTESIAN_POINT('Ctrl Pts',(56.9817391239669,21.2276144171214,23.837409305451));
#31682=CARTESIAN_POINT('Ctrl Pts',(56.9767449314093,21.2695368788017,23.840070322094));
#31683=CARTESIAN_POINT('Ctrl Pts',(56.9718923212409,21.3030043614319,23.8421572543967));
#31684=CARTESIAN_POINT('Ctrl Pts',(56.9317712792969,21.537549487808,23.8566204574773));
#31685=CARTESIAN_POINT('Ctrl Pts',(56.8666686542478,21.7323026767777,23.8679069450745));
#31686=CARTESIAN_POINT('Ctrl Pts',(56.756598022282,21.9458823394283,23.8823356726027));
#31687=CARTESIAN_POINT('Ctrl Pts',(56.7391985440534,21.9775061173452,23.8845262736268));
#31688=CARTESIAN_POINT('Ctrl Pts',(56.7079601487604,22.0308054180066,23.8883257641648));
#31689=CARTESIAN_POINT('Ctrl Pts',(56.6945421407528,22.0527176823218,23.889920062393));
#31690=CARTESIAN_POINT('Ctrl Pts',(56.6749767388604,22.0833252542758,23.8921961650324));
#31691=CARTESIAN_POINT('Ctrl Pts',(56.6691768653315,22.0922404806152,23.8928651610198));
#31692=CARTESIAN_POINT('Ctrl Pts',(56.6590770596141,22.1074969826515,23.8940206306559));
#31693=CARTESIAN_POINT('Ctrl Pts',(56.654811338603,22.1138607126937,23.8945058171669));
#31694=CARTESIAN_POINT('Ctrl Pts',(56.6465886625499,22.1259760546985,23.8954357786244));
#31695=CARTESIAN_POINT('Ctrl Pts',(56.6426379574153,22.1317317872237,23.8958803123192));
#31696=CARTESIAN_POINT('Ctrl Pts',(56.6323084312514,22.1466127094163,23.897036791697));
#31697=CARTESIAN_POINT('Ctrl Pts',(56.6258833495972,22.1557053453652,23.8977504938186));
#31698=CARTESIAN_POINT('Ctrl Pts',(56.6072276848336,22.1816429505268,23.8998070503394));
#31699=CARTESIAN_POINT('Ctrl Pts',(56.5948093863116,22.1983504747478,23.9011570940068));
#31700=CARTESIAN_POINT('Ctrl Pts',(56.4813874369299,22.3460617449723,23.9133257239011));
#31701=CARTESIAN_POINT('Ctrl Pts',(56.3647317478751,22.464198368296,23.9248023326573));
#31702=CARTESIAN_POINT('Ctrl Pts',(56.1568487420871,22.6280659729732,23.9432593176487));
#31703=CARTESIAN_POINT('Ctrl Pts',(56.0743316354838,22.6836606898815,23.9501604704387));
#31704=CARTESIAN_POINT('Ctrl Pts',(55.9731537402961,22.7413476753729,23.957885145782));
#31705=CARTESIAN_POINT('Ctrl Pts',(55.9581908557786,22.7496257485308,23.9590095189039));
#31706=CARTESIAN_POINT('Ctrl Pts',(55.9375092430206,22.7607227396348,23.9605371875023));
#31707=CARTESIAN_POINT('Ctrl Pts',(55.9318812107387,22.763707900526,23.9609502531802));
#31708=CARTESIAN_POINT('Ctrl Pts',(55.9223875183622,22.768685313645,23.9616424581039));
#31709=CARTESIAN_POINT('Ctrl Pts',(55.9185295051924,22.7706919613483,23.9619224891895));
#31710=CARTESIAN_POINT('Ctrl Pts',(55.9111827990654,22.7744826914593,23.9624533006095));
#31711=CARTESIAN_POINT('Ctrl Pts',(55.9076953747581,22.7762691301973,23.9627042327872));
#31712=CARTESIAN_POINT('Ctrl Pts',(55.8985127412093,22.7809388435023,23.9633622845547));
#31713=CARTESIAN_POINT('Ctrl Pts',(55.892808859721,22.7838051051317,23.9637683482897));
#31714=CARTESIAN_POINT('Ctrl Pts',(55.8728050835645,22.7937372317536,23.9651833815061));
#31715=CARTESIAN_POINT('Ctrl Pts',(55.8584338480649,22.8006591395237,23.9661838665021));
#31716=CARTESIAN_POINT('Ctrl Pts',(55.7449974119872,22.8536289960962,23.9739672550977));
#31717=CARTESIAN_POINT('Ctrl Pts',(55.642370758999,22.8916468216948,23.9803390609347));
#31718=CARTESIAN_POINT('Ctrl Pts',(55.4281711025293,22.951537451725,23.9932553584661));
#31719=CARTESIAN_POINT('Ctrl Pts',(55.3168195425044,22.9726764531659,23.9997798618336));
#31720=CARTESIAN_POINT('Ctrl Pts',(55.1910139235846,22.9856281348028,24.0073582988248));
#31721=CARTESIAN_POINT('Ctrl Pts',(55.1777361368094,22.9868606397568,24.0081604816638));
#31722=CARTESIAN_POINT('Ctrl Pts',(55.1644483449248,22.9879598346927,24.0089660407953));
#31723=CARTESIAN_POINT('Origin',(55.,21.,6.22095488139522));
#31724=CARTESIAN_POINT('',(55.1644483516314,22.9879598341379,24.9666501649259));
#31725=CARTESIAN_POINT('',(55.1644480328175,22.9879598605109,24.8095189920889));
#31726=CARTESIAN_POINT('',(55.1644483516311,22.987959834138,6.22095488139522));
#31727=CARTESIAN_POINT('',(53.0052508816068,21.0013916490052,24.380394655106));
#31728=CARTESIAN_POINT('Ctrl Pts',(55.1644483516314,22.9879598341379,24.9666501649259));
#31729=CARTESIAN_POINT('Ctrl Pts',(55.1676348043784,22.9876962438517,24.9664433125484));
#31730=CARTESIAN_POINT('Ctrl Pts',(55.1708206486967,22.9874249902382,24.966236876594));
#31731=CARTESIAN_POINT('Ctrl Pts',(55.1781715296382,22.9867813051299,24.9657614465516));
#31732=CARTESIAN_POINT('Ctrl Pts',(55.1823360370128,22.9864034381216,24.965492766225));
#31733=CARTESIAN_POINT('Ctrl Pts',(55.191449129187,22.985547659663,24.9649062812653));
#31734=CARTESIAN_POINT('Ctrl Pts',(55.1963971175177,22.9850643443955,24.9645887816202));
#31735=CARTESIAN_POINT('Ctrl Pts',(55.2105127152994,22.9836322498315,24.9636855562457));
#31736=CARTESIAN_POINT('Ctrl Pts',(55.2196757710823,22.9826384111216,24.9631022880781));
#31737=CARTESIAN_POINT('Ctrl Pts',(55.2813430105057,22.9755171145529,24.9591955069159));
#31738=CARTESIAN_POINT('Ctrl Pts',(55.3335976495527,22.9673676455074,24.9559758082724));
#31739=CARTESIAN_POINT('Ctrl Pts',(55.5561161877095,22.923541406835,24.9424214907378));
#31740=CARTESIAN_POINT('Ctrl Pts',(55.7216365943301,22.8677593283082,24.9326708509641));
#31741=CARTESIAN_POINT('Ctrl Pts',(55.933732027601,22.7638161272085,24.9185683953547));
#31742=CARTESIAN_POINT('Ctrl Pts',(55.9883137784462,22.7338216591524,24.9147865747066));
#31743=CARTESIAN_POINT('Ctrl Pts',(56.0541911542102,22.6934974092091,24.9099800788978));
#31744=CARTESIAN_POINT('Ctrl Pts',(56.0668929202699,22.6855242335651,24.9090417877736));
#31745=CARTESIAN_POINT('Ctrl Pts',(56.0868036314119,22.6727106135166,24.9075520043549));
#31746=CARTESIAN_POINT('Ctrl Pts',(56.0940731091583,22.6679649150338,24.9070040260844));
#31747=CARTESIAN_POINT('Ctrl Pts',(56.1075284161863,22.6590551440066,24.9059820746544));
#31748=CARTESIAN_POINT('Ctrl Pts',(56.1137223445617,22.6549035320121,24.9055085746815));
#31749=CARTESIAN_POINT('Ctrl Pts',(56.1273992548265,22.6456247337835,24.9044561431834));
#31750=CARTESIAN_POINT('Ctrl Pts',(56.1348707988371,22.6404810604455,24.9038765942969));
#31751=CARTESIAN_POINT('Ctrl Pts',(56.1564389863986,22.6254149011974,24.9021899908399));
#31752=CARTESIAN_POINT('Ctrl Pts',(56.1704421296306,22.6153606162459,24.9010779238478));
#31753=CARTESIAN_POINT('Ctrl Pts',(56.3064204573832,22.5150315177791,24.8901077597363));
#31754=CARTESIAN_POINT('Ctrl Pts',(56.4178242737187,22.4113155304903,24.879694506376));
#31755=CARTESIAN_POINT('Ctrl Pts',(56.5967024995637,22.2020206124041,24.8605012772838));
#31756=CARTESIAN_POINT('Ctrl Pts',(56.6681227782446,22.1007652961101,24.8518336237985));
#31757=CARTESIAN_POINT('Ctrl Pts',(56.737515795382,21.9799550505251,24.8426072261192));
#31758=CARTESIAN_POINT('Ctrl Pts',(56.745159503831,21.9662770736392,24.8415779132199));
#31759=CARTESIAN_POINT('Ctrl Pts',(56.7556676119914,21.9469418984802,24.8401457023311));
#31760=CARTESIAN_POINT('Ctrl Pts',(56.7586671881259,21.9413593612169,24.8397348296448));
#31761=CARTESIAN_POINT('Ctrl Pts',(56.763474685549,21.9323089021253,24.8390730961121));
#31762=CARTESIAN_POINT('Ctrl Pts',(56.7652990727238,21.9288498479524,24.8388212118687));
#31763=CARTESIAN_POINT('Ctrl Pts',(56.7691360241086,21.9215228167533,24.8382898729361));
#31764=CARTESIAN_POINT('Ctrl Pts',(56.7711461010435,21.9176535637337,24.8380105809474));
#31765=CARTESIAN_POINT('Ctrl Pts',(56.7760855451718,21.9080688003199,24.8373218552407));
#31766=CARTESIAN_POINT('Ctrl Pts',(56.7790000571311,21.9023456152373,24.8369133455825));
#31767=CARTESIAN_POINT('Ctrl Pts',(56.7897301942436,21.8810209300242,24.8354010100674));
#31768=CARTESIAN_POINT('Ctrl Pts',(56.7973689117648,21.8653306254997,24.8343076328615));
#31769=CARTESIAN_POINT('Ctrl Pts',(56.8489967611899,21.7556502868303,24.8267843833106));
#31770=CARTESIAN_POINT('Ctrl Pts',(56.8858041596834,21.658440945814,24.8207178442405));
#31771=CARTESIAN_POINT('Ctrl Pts',(56.9596389112881,21.405424924289,24.8054029108501));
#31772=CARTESIAN_POINT('Ctrl Pts',(56.9858034823534,21.2472496426684,24.7962151320123));
#31773=CARTESIAN_POINT('Ctrl Pts',(56.9938393398452,21.0645519298029,24.7849445058906));
#31774=CARTESIAN_POINT('Ctrl Pts',(56.9944536332143,21.0414355005556,24.7835077985283));
#31775=CARTESIAN_POINT('Ctrl Pts',(56.9947525182008,21.0088830974136,24.7814675007012));
#31776=CARTESIAN_POINT('Ctrl Pts',(56.9947722207145,20.9994514944123,24.7808743325751));
#31777=CARTESIAN_POINT('Ctrl Pts',(56.9946900188627,20.9830212396635,24.779837339938));
#31778=CARTESIAN_POINT('Ctrl Pts',(56.9946181663626,20.9760225514705,24.7793944594499));
#31779=CARTESIAN_POINT('Ctrl Pts',(56.994390699841,20.9613760236692,24.7784651277143));
#31780=CARTESIAN_POINT('Ctrl Pts',(56.9942279242369,20.9537284247535,24.7779784600591));
#31781=CARTESIAN_POINT('Ctrl Pts',(56.9937356932732,20.9355244919542,24.7768165491122));
#31782=CARTESIAN_POINT('Ctrl Pts',(56.9933663814113,20.9249695520094,24.776140071492));
#31783=CARTESIAN_POINT('Ctrl Pts',(56.9918308067822,20.8892111623983,24.773838569783));
#31784=CARTESIAN_POINT('Ctrl Pts',(56.9902702405538,20.8640279362705,24.7722013215391));
#31785=CARTESIAN_POINT('Ctrl Pts',(56.985385956164,20.8037547607055,24.7682417035525));
#31786=CARTESIAN_POINT('Ctrl Pts',(56.981609132341,20.7687110400051,24.7659059669717));
#31787=CARTESIAN_POINT('Ctrl Pts',(56.9631106953068,20.6313408203308,24.7566169735997));
#31788=CARTESIAN_POINT('Ctrl Pts',(56.9413741142413,20.5301326881196,24.749470357777));
#31789=CARTESIAN_POINT('Ctrl Pts',(56.8763739140957,20.3116964289198,24.7335840601125));
#31790=CARTESIAN_POINT('Ctrl Pts',(56.8297442418331,20.1958965663062,24.7248489019185));
#31791=CARTESIAN_POINT('Ctrl Pts',(56.7654482993205,20.0713106110895,24.7155649980124));
#31792=CARTESIAN_POINT('Ctrl Pts',(56.7581197842988,20.0575104568143,24.7145385891349));
#31793=CARTESIAN_POINT('Ctrl Pts',(56.7475952794788,20.0382420418461,24.7131097115398));
#31794=CARTESIAN_POINT('Ctrl Pts',(56.7445344746864,20.0327011319146,24.7126993161964));
#31795=CARTESIAN_POINT('Ctrl Pts',(56.7395407506309,20.0237619029437,24.7120381444399));
#31796=CARTESIAN_POINT('Ctrl Pts',(56.7376241565473,20.0203545863536,24.711786347912));
#31797=CARTESIAN_POINT('Ctrl Pts',(56.7335479878515,20.0131575803304,24.7112549972677));
#31798=CARTESIAN_POINT('Ctrl Pts',(56.7313859763516,20.009369297354,24.7109756067746));
#31799=CARTESIAN_POINT('Ctrl Pts',(56.7260060383929,20.0000139680418,24.7102862971545));
#31800=CARTESIAN_POINT('Ctrl Pts',(56.7227735534764,19.9944552745603,24.7098773055863));
#31801=CARTESIAN_POINT('Ctrl Pts',(56.7106422770758,19.9738241263041,24.7083611145125));
#31802=CARTESIAN_POINT('Ctrl Pts',(56.7015717976799,19.9588528486678,24.7072644329522));
#31803=CARTESIAN_POINT('Ctrl Pts',(56.6781857806741,19.9213752335779,24.7045230780892));
#31804=CARTESIAN_POINT('Ctrl Pts',(56.6636134050195,19.8990324800545,24.7028924565857));
#31805=CARTESIAN_POINT('Ctrl Pts',(56.5510297122465,19.7337581679719,24.690805346767));
#31806=CARTESIAN_POINT('Ctrl Pts',(56.4352079441073,19.6038442236217,24.6811003423006));
#31807=CARTESIAN_POINT('Ctrl Pts',(56.2796151644102,19.4694267423815,24.668919959998));
#31808=CARTESIAN_POINT('Ctrl Pts',(56.2546815550972,19.4489218184005,24.666992528749));
#31809=CARTESIAN_POINT('Ctrl Pts',(56.1921830057454,19.4000175245283,24.6622037697784));
#31810=CARTESIAN_POINT('Ctrl Pts',(56.1540907306473,19.3723273389756,24.6593208863156));
#31811=CARTESIAN_POINT('Ctrl Pts',(56.1035759886274,19.3382721901914,24.6555229418699));
#31812=CARTESIAN_POINT('Ctrl Pts',(56.0920151840305,19.3306521934883,24.6546554227062));
#31813=CARTESIAN_POINT('Ctrl Pts',(56.0733648532688,19.3186359644834,24.6532581159843));
#31814=CARTESIAN_POINT('Ctrl Pts',(56.0663253165551,19.3141626875614,24.6527312025308));
#31815=CARTESIAN_POINT('Ctrl Pts',(56.0529048076852,19.3057523074876,24.6517275071888));
#31816=CARTESIAN_POINT('Ctrl Pts',(56.04652927229,19.3018067667803,24.651251047686));
#31817=CARTESIAN_POINT('Ctrl Pts',(56.0319670690531,19.2929080032148,24.6501635037004));
#31818=CARTESIAN_POINT('Ctrl Pts',(56.0237667498073,19.2879775837296,24.6495515990114));
#31819=CARTESIAN_POINT('Ctrl Pts',(55.9985667089958,19.2730719233735,24.6476725632003));
#31820=CARTESIAN_POINT('Ctrl Pts',(55.9814547591628,19.2632897295159,24.6463985090654));
#31821=CARTESIAN_POINT('Ctrl Pts',(55.8590042680371,19.1956775410622,24.6372920576926));
#31822=CARTESIAN_POINT('Ctrl Pts',(55.7487924046716,19.1472267404228,24.6291275942133));
#31823=CARTESIAN_POINT('Ctrl Pts',(55.5080612006935,19.0664008089282,24.6115109037598));
#31824=CARTESIAN_POINT('Ctrl Pts',(55.3772469249719,19.0366816068826,24.602060054858));
#31825=CARTESIAN_POINT('Ctrl Pts',(55.2152280364035,19.0166768406861,24.5910750875196));
#31826=CARTESIAN_POINT('Ctrl Pts',(55.1859387422817,19.0137168213038,24.5891186642995));
#31827=CARTESIAN_POINT('Ctrl Pts',(55.1485108481939,19.0107695420505,24.5866648266484));
#31828=CARTESIAN_POINT('Ctrl Pts',(55.140424838047,19.0101823809317,24.5861374395999));
#31829=CARTESIAN_POINT('Ctrl Pts',(55.1276158022245,19.0093307302018,24.5853065894854));
#31830=CARTESIAN_POINT('Ctrl Pts',(55.1228951358004,19.0090337216756,24.5850013711377));
#31831=CARTESIAN_POINT('Ctrl Pts',(55.1139636607921,19.0085036703964,24.5844258187784));
#31832=CARTESIAN_POINT('Ctrl Pts',(55.1097532181249,19.0082671920576,24.5841553074799));
#31833=CARTESIAN_POINT('Ctrl Pts',(55.0999349189261,19.0077469785543,24.5835263565206));
#31834=CARTESIAN_POINT('Ctrl Pts',(55.0943265830782,19.0074735667869,24.5831684950534));
#31835=CARTESIAN_POINT('Ctrl Pts',(55.0762663218059,19.0066695358208,24.5820203927195));
#31836=CARTESIAN_POINT('Ctrl Pts',(55.0638102625817,19.0062319191309,24.5812351347766));
#31837=CARTESIAN_POINT('Ctrl Pts',(54.9527820074298,19.0033727879327,24.5742877963379));
#31838=CARTESIAN_POINT('Ctrl Pts',(54.8541468867826,19.0081461230351,24.568478537762));
#31839=CARTESIAN_POINT('Ctrl Pts',(54.5835310230122,19.0414627817128,24.5525939473954));
#31840=CARTESIAN_POINT('Ctrl Pts',(54.4143493830394,19.0852357066642,24.542655088259));
#31841=CARTESIAN_POINT('Ctrl Pts',(54.2324333538452,19.1587067533168,24.5305455533129));
#31842=CARTESIAN_POINT('Ctrl Pts',(54.2120108156771,19.1673537273201,24.5291660051294));
#31843=CARTESIAN_POINT('Ctrl Pts',(54.182665118346,19.180360001092,24.5271525069361));
#31844=CARTESIAN_POINT('Ctrl Pts',(54.1736232014417,19.1844484541934,24.5265277712401));
#31845=CARTESIAN_POINT('Ctrl Pts',(54.157737640267,19.1917746288857,24.5254223334259));
#31846=CARTESIAN_POINT('Ctrl Pts',(54.1508811679711,19.194984187914,24.524942606874));
#31847=CARTESIAN_POINT('Ctrl Pts',(54.1436601887791,19.1984146231634,24.5244345822891));
#31848=CARTESIAN_POINT('Ctrl Pts',(54.1432772273929,19.1985967044526,24.5244076311092));
#31849=CARTESIAN_POINT('Ctrl Pts',(54.1426809112851,19.198880459691,24.5243656519631));
#31850=CARTESIAN_POINT('Ctrl Pts',(54.1424675163437,19.1989820495527,24.5243506269103));
#31851=CARTESIAN_POINT('Ctrl Pts',(54.1421208330106,19.199147168937,24.5243262128666));
#31852=CARTESIAN_POINT('Ctrl Pts',(54.141987534679,19.199210674828,24.524316824755));
#31853=CARTESIAN_POINT('Ctrl Pts',(54.1417018581962,19.1993468155217,24.5242967025858));
#31854=CARTESIAN_POINT('Ctrl Pts',(54.1415494786931,19.199419456547,24.5242859681222));
#31855=CARTESIAN_POINT('Ctrl Pts',(54.1412586991956,19.1995581197091,24.5242654814664));
#31856=CARTESIAN_POINT('Ctrl Pts',(54.1411202949939,19.1996241397018,24.5242557292091));
#31857=CARTESIAN_POINT('Ctrl Pts',(54.1408561603809,19.1997501715726,24.5242371156331));
#31858=CARTESIAN_POINT('Ctrl Pts',(54.1407304331086,19.1998101785305,24.5242282547265));
#31859=CARTESIAN_POINT('Ctrl Pts',(54.1404904830244,19.1999247324763,24.5242113419952));
#31860=CARTESIAN_POINT('Ctrl Pts',(54.140376259191,19.1999792771305,24.5242032902558));
#31861=CARTESIAN_POINT('Ctrl Pts',(54.1401582501536,19.2000834072238,24.5241879211847));
#31862=CARTESIAN_POINT('Ctrl Pts',(54.1400544640929,19.2001329907453,24.5241806039222));
#31863=CARTESIAN_POINT('Ctrl Pts',(54.139856364504,19.2002276533565,24.5241666360689));
#31864=CARTESIAN_POINT('Ctrl Pts',(54.139762050177,19.2002727309085,24.5241599855287));
#31865=CARTESIAN_POINT('Ctrl Pts',(54.1395820181777,19.2003587946248,24.5241472896687));
#31866=CARTESIAN_POINT('Ctrl Pts',(54.1394962999072,19.2003997794916,24.524141244395));
#31867=CARTESIAN_POINT('Ctrl Pts',(54.1393326664959,19.2004780326435,24.5241297033616));
#31868=CARTESIAN_POINT('Ctrl Pts',(54.1392547507871,19.2005152998936,24.5241242076346));
#31869=CARTESIAN_POINT('Ctrl Pts',(54.1391060031611,19.2005864580724,24.5241137151684));
#31870=CARTESIAN_POINT('Ctrl Pts',(54.1390351708357,19.2006203481178,24.5241087184605));
#31871=CARTESIAN_POINT('Ctrl Pts',(54.1388999382049,19.2006850605928,24.5240991782298));
#31872=CARTESIAN_POINT('Ctrl Pts',(54.1388355375489,19.2007158822997,24.5240946347319));
#31873=CARTESIAN_POINT('Ctrl Pts',(54.1387125771048,19.2007747384283,24.5240859593593));
#31874=CARTESIAN_POINT('Ctrl Pts',(54.1386540171968,19.200802772172,24.5240818275173));
#31875=CARTESIAN_POINT('Ctrl Pts',(54.1385422028668,19.2008563065322,24.5240739378007));
#31876=CARTESIAN_POINT('Ctrl Pts',(54.1384889481523,19.2008818066812,24.5240701799395));
#31877=CARTESIAN_POINT('Ctrl Pts',(54.138356359029,19.2009453020512,24.5240608235276));
#31878=CARTESIAN_POINT('Ctrl Pts',(54.1382770258726,19.2009833002168,24.5240552248676));
#31879=CARTESIAN_POINT('Ctrl Pts',(54.1381200143869,19.2010585167052,24.5240441436185));
#31880=CARTESIAN_POINT('Ctrl Pts',(54.138042336046,19.2010957347679,24.5240386610433));
#31881=CARTESIAN_POINT('Ctrl Pts',(54.1378885930604,19.2011694099667,24.5240278091049));
#31882=CARTESIAN_POINT('Ctrl Pts',(54.1378125281441,19.2012058669793,24.5240224397366));
#31883=CARTESIAN_POINT('Ctrl Pts',(54.137661971134,19.2012780389131,24.5240118113688));
#31884=CARTESIAN_POINT('Ctrl Pts',(54.1375874790808,19.2013137535728,24.5240065523855));
#31885=CARTESIAN_POINT('Ctrl Pts',(54.1374400285605,19.2013844588914,24.5239961420579));
#31886=CARTESIAN_POINT('Ctrl Pts',(54.1373670700523,19.2014194493387,24.5239909907236));
#31887=CARTESIAN_POINT('Ctrl Pts',(54.1372226485801,19.2014887237887,24.523980793046));
#31888=CARTESIAN_POINT('Ctrl Pts',(54.1371511854602,19.2015230076452,24.5239757467042));
#31889=CARTESIAN_POINT('Ctrl Pts',(54.129139970632,19.2053669108682,24.5234100049145));
#31890=CARTESIAN_POINT('Ctrl Pts',(54.1212256391666,19.2092290112937,24.5228474909823));
#31891=CARTESIAN_POINT('Ctrl Pts',(54.0987980336851,19.2203578964112,24.5212429899138));
#31892=CARTESIAN_POINT('Ctrl Pts',(54.0843477890384,19.227749452343,24.5201966661263));
#31893=CARTESIAN_POINT('Ctrl Pts',(54.052012585362,19.2447905080663,24.5178263664843));
#31894=CARTESIAN_POINT('Ctrl Pts',(54.0341818652593,19.2545385196946,24.5164990160639));
#31895=CARTESIAN_POINT('Ctrl Pts',(53.977745987031,19.2865214054872,24.512231668133));
#31896=CARTESIAN_POINT('Ctrl Pts',(53.9397375655378,19.309776571731,24.5092568699223));
#31897=CARTESIAN_POINT('Ctrl Pts',(53.7622871645128,19.4266898488615,24.4948827916702));
#31898=CARTESIAN_POINT('Ctrl Pts',(53.6342863563278,19.5364246014618,24.4829603438867));
#31899=CARTESIAN_POINT('Ctrl Pts',(53.4858322569959,19.7003249974754,24.4678051562642));
#31900=CARTESIAN_POINT('Ctrl Pts',(53.4516989011861,19.7411815575075,24.464212847805));
#31901=CARTESIAN_POINT('Ctrl Pts',(53.4138815496365,19.7903170097563,24.460147068855));
#31902=CARTESIAN_POINT('Ctrl Pts',(53.4085714737221,19.7973113753004,24.4595740827152));
#31903=CARTESIAN_POINT('Ctrl Pts',(53.4000668303537,19.8086685398365,24.4586532766773));
#31904=CARTESIAN_POINT('Ctrl Pts',(53.3968435780148,19.8130095688568,24.4583035563238));
#31905=CARTESIAN_POINT('Ctrl Pts',(53.3911519094315,19.820740500493,24.4576847805924));
#31906=CARTESIAN_POINT('Ctrl Pts',(53.3886764929846,19.824125133102,24.4574152467923));
#31907=CARTESIAN_POINT('Ctrl Pts',(53.3833583866539,19.8314449002278,24.4568353008663));
#31908=CARTESIAN_POINT('Ctrl Pts',(53.3805193859416,19.8353826082748,24.4565251408301));
#31909=CARTESIAN_POINT('Ctrl Pts',(53.3726479290097,19.8463847996819,24.4556634875886));
#31910=CARTESIAN_POINT('Ctrl Pts',(53.3676470595739,19.8534719027567,24.4551141087919));
#31911=CARTESIAN_POINT('Ctrl Pts',(53.338710218839,19.8950535738245,24.4519222368892));
#31912=CARTESIAN_POINT('Ctrl Pts',(53.315819971952,19.9302670635964,24.4493447741032));
#31913=CARTESIAN_POINT('Ctrl Pts',(53.2044242995398,20.114084992578,24.436378115828));
#31914=CARTESIAN_POINT('Ctrl Pts',(53.1344013522111,20.2730269760886,24.426690984179));
#31915=CARTESIAN_POINT('Ctrl Pts',(53.0719163302744,20.4862464912673,24.413516415007));
#31916=CARTESIAN_POINT('Ctrl Pts',(53.0598299291023,20.5339647139773,24.4105622547277));
#31917=CARTESIAN_POINT('Ctrl Pts',(53.0428007465075,20.6134415502945,24.4055961776215));
#31918=CARTESIAN_POINT('Ctrl Pts',(53.036838485273,20.6449605074253,24.4036151909408));
#31919=CARTESIAN_POINT('Ctrl Pts',(53.0296972914166,20.688426197937,24.4008615200558));
#31920=CARTESIAN_POINT('Ctrl Pts',(53.0278621601364,20.7002612334259,24.4001095449652));
#31921=CARTESIAN_POINT('Ctrl Pts',(53.0251033542933,20.7191766150367,24.3989039156715));
#31922=CARTESIAN_POINT('Ctrl Pts',(53.024110909842,20.7262467607354,24.3984524378235));
#31923=CARTESIAN_POINT('Ctrl Pts',(53.022195379038,20.740446300345,24.3975439456216));
#31924=CARTESIAN_POINT('Ctrl Pts',(53.0212728355989,20.7475756581781,24.3970869214274));
#31925=CARTESIAN_POINT('Ctrl Pts',(53.0194871914024,20.7619866730898,24.3961612614836));
#31926=CARTESIAN_POINT('Ctrl Pts',(53.0186256639307,20.7692684096212,24.3956925836446));
#31927=CARTESIAN_POINT('Ctrl Pts',(53.0167383165913,20.7860111692049,24.3946127106645));
#31928=CARTESIAN_POINT('Ctrl Pts',(53.0157400204477,20.7954750555062,24.3940006604504));
#31929=CARTESIAN_POINT('Ctrl Pts',(53.0124488889824,20.8289709548609,24.3918283909596));
#31930=CARTESIAN_POINT('Ctrl Pts',(53.0105247093562,20.8530362748832,24.3902567394274));
#31931=CARTESIAN_POINT('Ctrl Pts',(53.0064843855035,20.9185047798876,24.3859498910358));
#31932=CARTESIAN_POINT('Ctrl Pts',(53.0052215183626,20.9599462506629,24.3831895681168));
#31933=CARTESIAN_POINT('Ctrl Pts',(53.0052504872089,21.001394173412,24.3803951722837));
#31934=CARTESIAN_POINT('Ctrl Pts',(53.0052504854785,21.0013916954035,24.3803953393496));
#31935=CARTESIAN_POINT('Ctrl Pts',(53.0053744414124,21.1790606296367,24.3684170045932));
#31936=CARTESIAN_POINT('Ctrl Pts',(53.0292322017107,21.3558945387234,24.3557807860037));
#31937=CARTESIAN_POINT('Ctrl Pts',(53.0895213675535,21.575885919755,24.3401825258644));
#31938=CARTESIAN_POINT('Ctrl Pts',(53.104699482229,21.6240273304911,24.3367843651265));
#31939=CARTESIAN_POINT('Ctrl Pts',(53.1247556485663,21.6801243933373,24.3328825920221));
#31940=CARTESIAN_POINT('Ctrl Pts',(53.1278816459156,21.6886823969914,24.3322889815137));
#31941=CARTESIAN_POINT('Ctrl Pts',(53.1327959925183,21.7018555748569,24.3313781003643));
#31942=CARTESIAN_POINT('Ctrl Pts',(53.1345430171888,21.7064858810228,24.3310584769951));
#31943=CARTESIAN_POINT('Ctrl Pts',(53.1377985616489,21.7150180871364,24.3304705848655));
#31944=CARTESIAN_POINT('Ctrl Pts',(53.1393021148868,21.7189217223319,24.3302020370318));
#31945=CARTESIAN_POINT('Ctrl Pts',(53.1427302050711,21.7277391835431,24.3295963830438));
#31946=CARTESIAN_POINT('Ctrl Pts',(53.1446619645514,21.7326501117046,24.329259713464));
#31947=CARTESIAN_POINT('Ctrl Pts',(53.1504406494992,21.7471712820239,24.3282659829877));
#31948=CARTESIAN_POINT('Ctrl Pts',(53.1543429876387,21.7567594857693,24.3276121357559));
#31949=CARTESIAN_POINT('Ctrl Pts',(53.1891104480686,21.8403156779393,24.3219307536087));
#31950=CARTESIAN_POINT('Ctrl Pts',(53.2243369692337,21.9124009079606,24.317141991972));
#31951=CARTESIAN_POINT('Ctrl Pts',(53.3271700845343,22.094178252436,24.3048786505637));
#31952=CARTESIAN_POINT('Ctrl Pts',(53.4012172397528,22.1997834794396,24.2975450830677));
#31953=CARTESIAN_POINT('Ctrl Pts',(53.5182633119268,22.3364547943455,24.2868913638562));
#31954=CARTESIAN_POINT('Ctrl Pts',(53.5530917736207,22.3740855300647,24.2838183989105));
#31955=CARTESIAN_POINT('Ctrl Pts',(53.6051688545557,22.4261751522309,24.2793209128481));
#31956=CARTESIAN_POINT('Ctrl Pts',(53.6212740665945,22.441750404861,24.2779425824143));
#31957=CARTESIAN_POINT('Ctrl Pts',(53.6504332651493,22.4690146540765,24.2754662147029));
#31958=CARTESIAN_POINT('Ctrl Pts',(53.6633855149432,22.4808092765275,24.2743727118282));
#31959=CARTESIAN_POINT('Ctrl Pts',(53.6832977336752,22.4984677074687,24.2727003881602));
#31960=CARTESIAN_POINT('Ctrl Pts',(53.6901454809844,22.5044571988141,24.2721268239649));
#31961=CARTESIAN_POINT('Ctrl Pts',(53.6971155062008,22.5104699831316,24.2715444946886));
#31962=CARTESIAN_POINT('Ctrl Pts',(53.6971971478378,22.5105404008242,24.271537673925));
#31963=CARTESIAN_POINT('Ctrl Pts',(53.6973638001637,22.510684118529,24.2715237513458));
#31964=CARTESIAN_POINT('Ctrl Pts',(53.6974488114816,22.5107574181148,24.2715166494947));
#31965=CARTESIAN_POINT('Ctrl Pts',(53.6976224265456,22.5109070892501,24.2715021461315));
#31966=CARTESIAN_POINT('Ctrl Pts',(53.6977110307563,22.5109834601244,24.2714947445996));
#31967=CARTESIAN_POINT('Ctrl Pts',(53.6978920745766,22.5111394799748,24.271479621636));
#31968=CARTESIAN_POINT('Ctrl Pts',(53.6979845148122,22.5112191282935,24.2714719001731));
#31969=CARTESIAN_POINT('Ctrl Pts',(53.698173496219,22.5113819281663,24.2714561152316));
#31970=CARTESIAN_POINT('Ctrl Pts',(53.6982700380402,22.5114650789451,24.2714480517222));
#31971=CARTESIAN_POINT('Ctrl Pts',(53.6984675130052,22.5116351297639,24.2714315585051));
#31972=CARTESIAN_POINT('Ctrl Pts',(53.6985684468999,22.5117220289573,24.271423128761));
#31973=CARTESIAN_POINT('Ctrl Pts',(53.6987750242842,22.5118998460546,24.2714058765732));
#31974=CARTESIAN_POINT('Ctrl Pts',(53.6988806686358,22.5119907630264,24.2713970540869));
#31975=CARTESIAN_POINT('Ctrl Pts',(53.6990970164859,22.5121769113792,24.271378987313));
#31976=CARTESIAN_POINT('Ctrl Pts',(53.699207720944,22.5122721417036,24.2713697429782));
#31977=CARTESIAN_POINT('Ctrl Pts',(53.6994345737779,22.5124672419858,24.2713508004779));
#31978=CARTESIAN_POINT('Ctrl Pts',(53.6995507231692,22.5125671106945,24.2713411022649));
#31979=CARTESIAN_POINT('Ctrl Pts',(53.6997888900893,22.5127718459999,24.2713212167001));
#31980=CARTESIAN_POINT('Ctrl Pts',(53.6999109087731,22.512876711189,24.2713110292941));
#31981=CARTESIAN_POINT('Ctrl Pts',(53.7001612832108,22.5130918351072,24.2712901263204));
#31982=CARTESIAN_POINT('Ctrl Pts',(53.7002896402545,22.5132020922211,24.2712794106928));
#31983=CARTESIAN_POINT('Ctrl Pts',(53.7004997078298,22.5133824912249,24.2712618744412));
#31984=CARTESIAN_POINT('Ctrl Pts',(53.7005814100934,22.5134526429002,24.2712550542114));
#31985=CARTESIAN_POINT('Ctrl Pts',(53.70076751334,22.5136124097792,24.2712395193977));
#31986=CARTESIAN_POINT('Ctrl Pts',(53.700871917902,22.5137020207871,24.2712308046424));
#31987=CARTESIAN_POINT('Ctrl Pts',(53.7011103999963,22.5139066684285,24.2712108990488));
#31988=CARTESIAN_POINT('Ctrl Pts',(53.701244483496,22.5140216980151,24.2711997079253));
#31989=CARTESIAN_POINT('Ctrl Pts',(53.7070512557002,22.5190019608301,24.2707150758491));
#31990=CARTESIAN_POINT('Ctrl Pts',(53.712751161316,22.5238352395217,24.2702403301013));
#31991=CARTESIAN_POINT('Ctrl Pts',(53.7256242359562,22.5346272949989,24.2691702151703));
#31992=CARTESIAN_POINT('Ctrl Pts',(53.7328122628395,22.5405679979953,24.2685741248451));
#31993=CARTESIAN_POINT('Ctrl Pts',(53.7512670760165,22.5556038394103,24.2670471959981));
#31994=CARTESIAN_POINT('Ctrl Pts',(53.7625915668127,22.5646269752729,24.2661135016873));
#31995=CARTESIAN_POINT('Ctrl Pts',(53.8344515100184,22.6206154765686,24.2602080822056));
#31996=CARTESIAN_POINT('Ctrl Pts',(53.8975452624156,22.664178116476,24.2551047954707));
#31997=CARTESIAN_POINT('Ctrl Pts',(54.0992766138642,22.7869475617343,24.2390355902647));
#31998=CARTESIAN_POINT('Ctrl Pts',(54.2450143737752,22.8532332362195,24.2277139411983));
#31999=CARTESIAN_POINT('Ctrl Pts',(54.4299260009135,22.911865703729,24.2144412050943));
#32000=CARTESIAN_POINT('Ctrl Pts',(54.4630375121495,22.9214282185605,24.2121074398105));
#32001=CARTESIAN_POINT('Ctrl Pts',(54.5168080274741,22.9354582685018,24.2084031773435));
#32002=CARTESIAN_POINT('Ctrl Pts',(54.5373184057796,22.9404636096017,24.2070100140868));
#32003=CARTESIAN_POINT('Ctrl Pts',(54.564640113532,22.9466733243871,24.2051837964063));
#32004=CARTESIAN_POINT('Ctrl Pts',(54.5713829081274,22.9481690518494,24.2047354786657));
#32005=CARTESIAN_POINT('Ctrl Pts',(54.5824963742723,22.9505738159128,24.2040006271888));
#32006=CARTESIAN_POINT('Ctrl Pts',(54.5868625033272,22.9515032407408,24.2037129576162));
#32007=CARTESIAN_POINT('Ctrl Pts',(54.5954274801637,22.9532964481474,24.2031507079015));
#32008=CARTESIAN_POINT('Ctrl Pts',(54.599626040789,22.9541613626998,24.2028760675952));
#32009=CARTESIAN_POINT('Ctrl Pts',(54.6099746599695,22.9562584536195,24.2022014625306));
#32010=CARTESIAN_POINT('Ctrl Pts',(54.6161278707485,22.9574751835347,24.2018023697279));
#32011=CARTESIAN_POINT('Ctrl Pts',(54.6372889189158,22.9615559300947,24.2004365018136));
#32012=CARTESIAN_POINT('Ctrl Pts',(54.6523243013168,22.964276619309,24.1994774481572));
#32013=CARTESIAN_POINT('Ctrl Pts',(54.7968129741785,22.9887111235441,24.1903574965546));
#32014=CARTESIAN_POINT('Ctrl Pts',(54.9280997295243,22.9977730564976,24.1827979213669));
#32015=CARTESIAN_POINT('Ctrl Pts',(55.0944337379504,22.9928227445012,24.1731426277646));
#32016=CARTESIAN_POINT('Ctrl Pts',(55.1294820511752,22.9908523238325,24.1711048544396));
#32017=CARTESIAN_POINT('Ctrl Pts',(55.1644484328881,22.9879598274162,24.1690565717028));
#32018=CARTESIAN_POINT('Ctrl Pts',(55.1644483449248,22.9879598346927,24.0089660407953));
#32019=CARTESIAN_POINT('Ctrl Pts',(55.1201504546627,22.9916242521574,24.0116515562158));
#32020=CARTESIAN_POINT('Ctrl Pts',(55.075741393938,22.9938071064991,24.014374972811));
#32021=CARTESIAN_POINT('Ctrl Pts',(55.0170795277407,22.9947275452425,24.0180305829984));
#32022=CARTESIAN_POINT('Ctrl Pts',(55.0028624442198,22.9947986063458,24.0189210070507));
#32023=CARTESIAN_POINT('Ctrl Pts',(54.9802255455821,22.994669757504,24.0203463745895));
#32024=CARTESIAN_POINT('Ctrl Pts',(54.9718054848462,22.9945685088112,24.0208782316466));
#32025=CARTESIAN_POINT('Ctrl Pts',(54.9559071143158,22.9942766455062,24.0218857287375));
#32026=CARTESIAN_POINT('Ctrl Pts',(54.9484287242451,22.9940972700442,24.0223610088173));
#32027=CARTESIAN_POINT('Ctrl Pts',(54.931529604813,22.9935968046183,24.0234381795587));
#32028=CARTESIAN_POINT('Ctrl Pts',(54.9221098397583,22.9932509958099,24.0240408331336));
#32029=CARTESIAN_POINT('Ctrl Pts',(54.8978916526339,22.9921899880803,24.0255961357955));
#32030=CARTESIAN_POINT('Ctrl Pts',(54.8830983204186,22.9913766697587,24.0265518256977));
#32031=CARTESIAN_POINT('Ctrl Pts',(54.7839848515052,22.9848193485508,24.0329939884227));
#32032=CARTESIAN_POINT('Ctrl Pts',(54.7001052303843,22.9738870615148,24.0386417614492));
#32033=CARTESIAN_POINT('Ctrl Pts',(54.468031614072,22.9285054502434,24.0547998883235));
#32034=CARTESIAN_POINT('Ctrl Pts',(54.3227183528229,22.8823942503079,24.0655744578728));
#32035=CARTESIAN_POINT('Ctrl Pts',(54.1531881242769,22.8064001350005,24.0782787290817));
#32036=CARTESIAN_POINT('Ctrl Pts',(54.1226759940034,22.7917797451871,24.0805685456348));
#32037=CARTESIAN_POINT('Ctrl Pts',(54.0739988975599,22.7669135280702,24.0842109271548));
#32038=CARTESIAN_POINT('Ctrl Pts',(54.0555976420066,22.7571470418782,24.0855852944508));
#32039=CARTESIAN_POINT('Ctrl Pts',(54.0313340174825,22.7437777916207,24.0873907948999));
#32040=CARTESIAN_POINT('Ctrl Pts',(54.02533320286,22.7404308116502,24.0878367711843));
#32041=CARTESIAN_POINT('Ctrl Pts',(54.0154700277099,22.7348625724343,24.0885687269228));
#32042=CARTESIAN_POINT('Ctrl Pts',(54.0115976609762,22.7326592938996,24.0888558256824));
#32043=CARTESIAN_POINT('Ctrl Pts',(54.0040105454273,22.7283087045995,24.0894177505274));
#32044=CARTESIAN_POINT('Ctrl Pts',(54.0002952983333,22.7261623568016,24.0896926324532));
#32045=CARTESIAN_POINT('Ctrl Pts',(53.9911447006593,22.7208364823964,24.0903690409796));
#32046=CARTESIAN_POINT('Ctrl Pts',(53.9857173669071,22.7176431401592,24.0907696842096));
#32047=CARTESIAN_POINT('Ctrl Pts',(53.9670408126773,22.7065348116988,24.0921468241187));
#32048=CARTESIAN_POINT('Ctrl Pts',(53.953867992275,22.6984915669489,24.0931154259836));
#32049=CARTESIAN_POINT('Ctrl Pts',(53.8318463418225,22.6220276629111,24.1020751439746));
#32050=CARTESIAN_POINT('Ctrl Pts',(53.7297423064452,22.5433766629365,24.1094906789742));
#32051=CARTESIAN_POINT('Ctrl Pts',(53.5625076910332,22.3866377073119,24.1227884230327));
#32052=CARTESIAN_POINT('Ctrl Pts',(53.4944186815043,22.312391369064,24.1286328948172));
#32053=CARTESIAN_POINT('Ctrl Pts',(53.399743874035,22.192043435566,24.1378421023001));
#32054=CARTESIAN_POINT('Ctrl Pts',(53.3689097527057,22.1494916681885,24.1410519184223));
#32055=CARTESIAN_POINT('Ctrl Pts',(53.332143639312,22.094291147485,24.1451868901259));
#32056=CARTESIAN_POINT('Ctrl Pts',(53.3246141777311,22.0827281684426,24.1460514580284));
#32057=CARTESIAN_POINT('Ctrl Pts',(53.3127334098542,22.0640622069451,24.1474450373972));
#32058=CARTESIAN_POINT('Ctrl Pts',(53.3083054923293,22.05700833288,24.1479712009774));
#32059=CARTESIAN_POINT('Ctrl Pts',(53.2999757072047,22.0435521920616,24.1489741358482));
#32060=CARTESIAN_POINT('Ctrl Pts',(53.2960654985755,22.0371552371698,24.1494505894083));
#32061=CARTESIAN_POINT('Ctrl Pts',(53.2872398690975,22.0225322120775,24.1505390518519));
#32062=CARTESIAN_POINT('Ctrl Pts',(53.2823475057463,22.0142925093043,24.1511518874507));
#32063=CARTESIAN_POINT('Ctrl Pts',(53.2697813902583,21.9927770409265,24.1527510288973));
#32064=CARTESIAN_POINT('Ctrl Pts',(53.2622011283673,21.9794476762148,24.1537406698523));
#32065=CARTESIAN_POINT('Ctrl Pts',(53.2055781965782,21.8771532657491,24.1613289756606));
#32066=CARTESIAN_POINT('Ctrl Pts',(53.1632499850094,21.7846598743356,24.1681643887401));
#32067=CARTESIAN_POINT('Ctrl Pts',(53.1196806768405,21.666354097067,24.1768459592815));
#32068=CARTESIAN_POINT('Ctrl Pts',(53.1116336426709,21.6431959226837,24.1785419117466));
#32069=CARTESIAN_POINT('Ctrl Pts',(53.0807085948919,21.5486100075613,24.1854484365023));
#32070=CARTESIAN_POINT('Ctrl Pts',(53.0614407213508,21.4760674420471,24.1907015752486));
#32071=CARTESIAN_POINT('Ctrl Pts',(53.0310087615182,21.3283949953725,24.2011662044374));
#32072=CARTESIAN_POINT('Ctrl Pts',(53.0199540427219,21.2533577871977,24.2063680862179));
#32073=CARTESIAN_POINT('Ctrl Pts',(53.0118574211865,21.1629169455024,24.212373208555));
#32074=CARTESIAN_POINT('Ctrl Pts',(53.0106877976602,21.1479521507097,24.2133581532773));
#32075=CARTESIAN_POINT('Ctrl Pts',(53.009283810642,21.126937882553,24.214727757282));
#32076=CARTESIAN_POINT('Ctrl Pts',(53.0089079248541,21.1208988139083,24.2151197907483));
#32077=CARTESIAN_POINT('Ctrl Pts',(53.0083127110249,21.1105788312556,24.2157869493336));
#32078=CARTESIAN_POINT('Ctrl Pts',(53.008079693714,21.1062987758672,24.2160628272749));
#32079=CARTESIAN_POINT('Ctrl Pts',(53.0076282017065,21.0974823332571,24.2166293846024));
#32080=CARTESIAN_POINT('Ctrl Pts',(53.0074114209899,21.0929459183311,24.2169199693291));
#32081=CARTESIAN_POINT('Ctrl Pts',(53.0068882495684,21.0811532989728,24.2176730277907));
#32082=CARTESIAN_POINT('Ctrl Pts',(53.0066059870503,21.0738960125848,24.2181341749747));
#32083=CARTESIAN_POINT('Ctrl Pts',(53.0056294460151,21.0446800850045,24.21998199044));
#32084=CARTESIAN_POINT('Ctrl Pts',(53.0052582849255,21.0227112526261,24.2213518101054));
#32085=CARTESIAN_POINT('Ctrl Pts',(53.0051869685036,20.8303971244324,24.2332061857491));
#32086=CARTESIAN_POINT('Ctrl Pts',(53.0269430638565,20.6607262184238,24.2427735846008));
#32087=CARTESIAN_POINT('Ctrl Pts',(53.0946009687021,20.4017082946576,24.2584692867371));
#32088=CARTESIAN_POINT('Ctrl Pts',(53.1260505416986,20.3094869824277,24.2642804424908));
#32089=CARTESIAN_POINT('Ctrl Pts',(53.1700519439094,20.2059286616253,24.2712670480698));
#32090=CARTESIAN_POINT('Ctrl Pts',(53.1761634107087,20.1919905607599,24.2722172114739));
#32091=CARTESIAN_POINT('Ctrl Pts',(53.1863676500479,20.1694240381615,24.2737722998942));
#32092=CARTESIAN_POINT('Ctrl Pts',(53.1903640222102,20.1607525085169,24.2743739309471));
#32093=CARTESIAN_POINT('Ctrl Pts',(53.1976076149501,20.1453273113667,24.2754515629388));
#32094=CARTESIAN_POINT('Ctrl Pts',(53.2008309476769,20.1385625774085,24.2759267324222));
#32095=CARTESIAN_POINT('Ctrl Pts',(53.2077256015357,20.1243004331026,24.2769340675041));
#32096=CARTESIAN_POINT('Ctrl Pts',(53.211406016372,20.1168076035813,24.2774665422779));
#32097=CARTESIAN_POINT('Ctrl Pts',(53.2213337221065,20.0969126995134,24.2788891833555));
#32098=CARTESIAN_POINT('Ctrl Pts',(53.2276635825834,20.0845525641883,24.2797822226333));
#32099=CARTESIAN_POINT('Ctrl Pts',(53.2590477756434,20.0248153019157,24.2841440429888));
#32100=CARTESIAN_POINT('Ctrl Pts',(53.2858734333657,19.9783987803166,24.2876749726932));
#32101=CARTESIAN_POINT('Ctrl Pts',(53.3702046389756,19.845171328773,24.2982431385995));
#32102=CARTESIAN_POINT('Ctrl Pts',(53.432668764797,19.7617227869511,24.3054418134468));
#32103=CARTESIAN_POINT('Ctrl Pts',(53.5828752659126,19.5907289870585,24.3213082969186));
#32104=CARTESIAN_POINT('Ctrl Pts',(53.6728526841473,19.5056865407901,24.3299684805561));
#32105=CARTESIAN_POINT('Ctrl Pts',(53.7824634150558,19.4198488194517,24.3391882590102));
#32106=CARTESIAN_POINT('Ctrl Pts',(53.794913901926,19.4103331726723,24.3402176745465));
#32107=CARTESIAN_POINT('Ctrl Pts',(53.8125550764452,19.3971767826822,24.3416499322326));
#32108=CARTESIAN_POINT('Ctrl Pts',(53.817652576768,19.3934128452296,24.3420607514116));
#32109=CARTESIAN_POINT('Ctrl Pts',(53.8259242133656,19.3873658520242,24.3427223694111));
#32110=CARTESIAN_POINT('Ctrl Pts',(53.8290872275258,19.3850677636875,24.342974191508));
#32111=CARTESIAN_POINT('Ctrl Pts',(53.8357906859715,19.3802274132129,24.3435053672755));
#32112=CARTESIAN_POINT('Ctrl Pts',(53.8393327448244,19.3776874273995,24.3437845584957));
#32113=CARTESIAN_POINT('Ctrl Pts',(53.8481118863605,19.371435435325,24.3444729754754));
#32114=CARTESIAN_POINT('Ctrl Pts',(53.8533586698706,19.3677370216715,24.3448812783426));
#32115=CARTESIAN_POINT('Ctrl Pts',(53.8729217829715,19.3540880276946,24.3463924737536));
#32116=CARTESIAN_POINT('Ctrl Pts',(53.8873510154334,19.3442996001751,24.3474849361285));
#32117=CARTESIAN_POINT('Ctrl Pts',(53.9884010859737,19.2776675062381,24.3549970223303));
#32118=CARTESIAN_POINT('Ctrl Pts',(54.079218351292,19.2274515108908,24.3610544309121));
#32119=CARTESIAN_POINT('Ctrl Pts',(54.3191469521964,19.1182287589057,24.3763727757744));
#32120=CARTESIAN_POINT('Ctrl Pts',(54.4721846627788,19.0697076193825,24.3855721550808));
#32121=CARTESIAN_POINT('Ctrl Pts',(54.6520710515779,19.0356917618733,24.3968553359351));
#32122=CARTESIAN_POINT('Ctrl Pts',(54.6748459090992,19.0317936704078,24.3982909124424));
#32123=CARTESIAN_POINT('Ctrl Pts',(54.7070005718512,19.0268634707939,24.4003297633327));
#32124=CARTESIAN_POINT('Ctrl Pts',(54.7163283966702,19.0255008624061,24.4009226332413));
#32125=CARTESIAN_POINT('Ctrl Pts',(54.7325954193293,19.0232422243168,24.4019591643541));
#32126=CARTESIAN_POINT('Ctrl Pts',(54.7395303771718,19.0223164846107,24.4024018828136));
#32127=CARTESIAN_POINT('Ctrl Pts',(54.7540554412726,19.020455274477,24.4033309331839));
#32128=CARTESIAN_POINT('Ctrl Pts',(54.7616463305098,19.0195269323018,24.4038174816814));
#32129=CARTESIAN_POINT('Ctrl Pts',(54.7797318788632,19.0174206090636,24.4049792154059));
#32130=CARTESIAN_POINT('Ctrl Pts',(54.7902308382829,19.0162822836284,24.4056556351956));
#32131=CARTESIAN_POINT('Ctrl Pts',(54.8258480083624,19.0127064874755,24.4079574508394));
#32132=CARTESIAN_POINT('Ctrl Pts',(54.8510024075139,19.0106624113426,24.4095950781105));
#32133=CARTESIAN_POINT('Ctrl Pts',(54.9113754114096,19.0069078809627,24.4135559498465));
#32134=CARTESIAN_POINT('Ctrl Pts',(54.9466128382667,19.0056529713029,24.415892575055));
#32135=CARTESIAN_POINT('Ctrl Pts',(55.0853077001173,19.0043918750168,24.4251877403351));
#32136=CARTESIAN_POINT('Ctrl Pts',(55.1886572786616,19.0114997699508,24.4323399416086));
#32137=CARTESIAN_POINT('Ctrl Pts',(55.4140974886809,19.0447407386672,24.4482246769193));
#32138=CARTESIAN_POINT('Ctrl Pts',(55.5352584213596,19.074378183792,24.4569523608459));
#32139=CARTESIAN_POINT('Ctrl Pts',(55.6676432703045,19.1202329160133,24.4662298844263));
#32140=CARTESIAN_POINT('Ctrl Pts',(55.682351326863,19.1255217980751,24.4672566075729));
#32141=CARTESIAN_POINT('Ctrl Pts',(55.7029269232083,19.1331948768822,24.4686857742312));
#32142=CARTESIAN_POINT('Ctrl Pts',(55.7088471473249,19.1354348090135,24.4690961502209));
#32143=CARTESIAN_POINT('Ctrl Pts',(55.7184056169918,19.1391033860441,24.4697572461807));
#32144=CARTESIAN_POINT('Ctrl Pts',(55.7220504428948,19.1405145881404,24.4700089863843));
#32145=CARTESIAN_POINT('Ctrl Pts',(55.7297524269464,19.1435226993168,24.4705401722585));
#32146=CARTESIAN_POINT('Ctrl Pts',(55.7338085422907,19.1451222152031,24.4708194546238));
#32147=CARTESIAN_POINT('Ctrl Pts',(55.7438298504644,19.1491121015627,24.4715084118892));
#32148=CARTESIAN_POINT('Ctrl Pts',(55.7497888599526,19.151518047898,24.4719171606612));
#32149=CARTESIAN_POINT('Ctrl Pts',(55.7719170798269,19.1605769156864,24.473431921239));
#32150=CARTESIAN_POINT('Ctrl Pts',(55.7880107871393,19.1674137646631,24.4745274388747));
#32151=CARTESIAN_POINT('Ctrl Pts',(55.8283880728196,19.1851969399015,24.4772654219345));
#32152=CARTESIAN_POINT('Ctrl Pts',(55.8525467468859,19.1964199130238,24.4788938772922));
#32153=CARTESIAN_POINT('Ctrl Pts',(56.0316276992867,19.2840151981439,24.4909441445611));
#32154=CARTESIAN_POINT('Ctrl Pts',(56.1762777001333,19.3797402981935,24.5006186912474));
#32155=CARTESIAN_POINT('Ctrl Pts',(56.3326308301585,19.5153142183306,24.5128740032492));
#32156=CARTESIAN_POINT('Ctrl Pts',(56.3578841520877,19.5383751275753,24.5149160073336));
#32157=CARTESIAN_POINT('Ctrl Pts',(56.4157110278066,19.593974244281,24.5197606758156));
#32158=CARTESIAN_POINT('Ctrl Pts',(56.4477742930153,19.6270122962901,24.522580664548));
#32159=CARTESIAN_POINT('Ctrl Pts',(56.4878816687065,19.6713073041469,24.5263064439513));
#32160=CARTESIAN_POINT('Ctrl Pts',(56.4969932466944,19.6815814987274,24.5271669406076));
#32161=CARTESIAN_POINT('Ctrl Pts',(56.5114497059954,19.6982256451391,24.528555515134));
#32162=CARTESIAN_POINT('Ctrl Pts',(56.5168622077254,19.704536482911,24.5290807819553));
#32163=CARTESIAN_POINT('Ctrl Pts',(56.527082284277,19.7166046917551,24.5300830273523));
#32164=CARTESIAN_POINT('Ctrl Pts',(56.531897157794,19.7223557163277,24.5305596949737));
#32165=CARTESIAN_POINT('Ctrl Pts',(56.5428062621453,19.7355361867768,24.531650077597));
#32166=CARTESIAN_POINT('Ctrl Pts',(56.5488794362536,19.742982743128,24.5322646300916));
#32167=CARTESIAN_POINT('Ctrl Pts',(56.5673820186913,19.7660071614647,24.5341604733343));
#32168=CARTESIAN_POINT('Ctrl Pts',(56.5796316632102,19.7817272559743,24.5354488705616));
#32169=CARTESIAN_POINT('Ctrl Pts',(56.6811813476548,19.9161539162316,24.54641962589));
#32170=CARTESIAN_POINT('Ctrl Pts',(56.7571826535879,20.044287776389,24.5566264820719));
#32171=CARTESIAN_POINT('Ctrl Pts',(56.8686209598344,20.2912798885625,24.5755180412968));
#32172=CARTESIAN_POINT('Ctrl Pts',(56.9086066661541,20.4073327590701,24.584100975454));
#32173=CARTESIAN_POINT('Ctrl Pts',(56.9414193521452,20.5415630888679,24.5932521286237));
#32174=CARTESIAN_POINT('Ctrl Pts',(56.944963652324,20.556840965103,24.5942824240086));
#32175=CARTESIAN_POINT('Ctrl Pts',(56.9496870534991,20.5783506981071,24.5957156917872));
#32176=CARTESIAN_POINT('Ctrl Pts',(56.9510170823219,20.5845483331275,24.5961266557924));
#32177=CARTESIAN_POINT('Ctrl Pts',(56.953119766704,20.594579196344,24.5967884444127));
#32178=CARTESIAN_POINT('Ctrl Pts',(56.9539107201787,20.5984084794924,24.597040293299));
#32179=CARTESIAN_POINT('Ctrl Pts',(56.9555594390969,20.6065106916597,24.5975714659817));
#32180=CARTESIAN_POINT('Ctrl Pts',(56.9564144705416,20.6107841527528,24.5978506276065));
#32181=CARTESIAN_POINT('Ctrl Pts',(56.958493790088,20.6213566161494,24.5985388688223));
#32182=CARTESIAN_POINT('Ctrl Pts',(56.9597017150029,20.6276588541642,24.5989470265737));
#32183=CARTESIAN_POINT('Ctrl Pts',(56.9640754850284,20.6510896180521,24.6004570629606));
#32184=CARTESIAN_POINT('Ctrl Pts',(56.9670474576904,20.6682541431399,24.601548532192));
#32185=CARTESIAN_POINT('Ctrl Pts',(56.9860985927904,20.7875596366002,24.6090468857285));
#32186=CARTESIAN_POINT('Ctrl Pts',(56.9944415430899,20.8907899121634,24.6150929570007));
#32187=CARTESIAN_POINT('Ctrl Pts',(56.9952065330458,21.1544603789626,24.6304148984246));
#32188=CARTESIAN_POINT('Ctrl Pts',(56.9763613361714,21.3141605022672,24.6396280555755));
#32189=CARTESIAN_POINT('Ctrl Pts',(56.9331801189221,21.4923160557855,24.6509262513412));
#32190=CARTESIAN_POINT('Ctrl Pts',(56.9273534283053,21.5146544128928,24.6523605894061));
#32191=CARTESIAN_POINT('Ctrl Pts',(56.9186042750282,21.545961535097,24.6543979654552));
#32192=CARTESIAN_POINT('Ctrl Pts',(56.9160037429072,21.5550189314289,24.6549906192823));
#32193=CARTESIAN_POINT('Ctrl Pts',(56.9113610036103,21.5707675668143,24.656026880526));
#32194=CARTESIAN_POINT('Ctrl Pts',(56.909347575784,21.5774671715941,24.6564695464577));
#32195=CARTESIAN_POINT('Ctrl Pts',(56.9050592124056,21.5914688960616,24.657398593521));
#32196=CARTESIAN_POINT('Ctrl Pts',(56.9027774422238,21.5987687871518,24.6578851917919));
#32197=CARTESIAN_POINT('Ctrl Pts',(56.8972439708907,21.6161205149528,24.6590472428152));
#32198=CARTESIAN_POINT('Ctrl Pts',(56.8939543100859,21.6261599142584,24.6597239319087));
#32199=CARTESIAN_POINT('Ctrl Pts',(56.8825287762426,21.6601144508086,24.662027636207));
#32200=CARTESIAN_POINT('Ctrl Pts',(56.8740187063137,21.6839001920939,24.6636669100598));
#32201=CARTESIAN_POINT('Ctrl Pts',(56.8525387016752,21.7405228395673,24.6676324875115));
#32202=CARTESIAN_POINT('Ctrl Pts',(56.8391445797303,21.7731886433931,24.6699722138506));
#32203=CARTESIAN_POINT('Ctrl Pts',(56.7830255071102,21.9003316902037,24.6792863832323));
#32204=CARTESIAN_POINT('Ctrl Pts',(56.7338327749072,21.9917643565053,24.686455361212));
#32205=CARTESIAN_POINT('Ctrl Pts',(56.610624479092,22.1833528612105,24.7023341584585));
#32206=CARTESIAN_POINT('Ctrl Pts',(56.5338803441178,22.2812695787954,24.7110381176753));
#32207=CARTESIAN_POINT('Ctrl Pts',(56.4377750938679,22.3827779463659,24.7202948658823));
#32208=CARTESIAN_POINT('Ctrl Pts',(56.426891045618,22.3940064740992,24.7213221078798));
#32209=CARTESIAN_POINT('Ctrl Pts',(56.4114161461479,22.4095999808155,24.7227518702476));
#32210=CARTESIAN_POINT('Ctrl Pts',(56.4069351640366,22.4140725194842,24.7231623316721));
#32211=CARTESIAN_POINT('Ctrl Pts',(56.3996533229827,22.4212717599659,24.7238235282743));
#32212=CARTESIAN_POINT('Ctrl Pts',(56.396865654455,22.4240116517299,24.7240752842722));
#32213=CARTESIAN_POINT('Ctrl Pts',(56.3909515979916,22.4297902720865,24.7246064681429));
#32214=CARTESIAN_POINT('Ctrl Pts',(56.3878232667474,22.4328269787615,24.7248857328756));
#32215=CARTESIAN_POINT('Ctrl Pts',(56.3800602550646,22.4403133456851,24.7255745857494));
#32216=CARTESIAN_POINT('Ctrl Pts',(56.3754139374104,22.444750962926,24.725983248388));
#32217=CARTESIAN_POINT('Ctrl Pts',(56.3580510251904,22.4611743013001,24.7274973198924));
#32218=CARTESIAN_POINT('Ctrl Pts',(56.3451981077814,22.4730156231024,24.7285922469728));
#32219=CARTESIAN_POINT('Ctrl Pts',(56.3123815466474,22.5024615056038,24.73132845339));
#32220=CARTESIAN_POINT('Ctrl Pts',(56.2922176330935,22.5198386848212,24.7329557458309));
#32221=CARTESIAN_POINT('Ctrl Pts',(56.1388915735912,22.6467162438117,24.7449856958899));
#32222=CARTESIAN_POINT('Ctrl Pts',(55.9923762343565,22.7389505321152,24.7546434375773));
#32223=CARTESIAN_POINT('Ctrl Pts',(55.7665585067778,22.8431584765607,24.76936898023));
#32224=CARTESIAN_POINT('Ctrl Pts',(55.6955352478824,22.8711156685095,24.7739701783918));
#32225=CARTESIAN_POINT('Ctrl Pts',(55.6093184682002,22.8994653899005,24.7796112167173));
#32226=CARTESIAN_POINT('Ctrl Pts',(55.5954969675613,22.9038437717777,24.7805170669479));
#32227=CARTESIAN_POINT('Ctrl Pts',(55.5727051384031,22.9107913090369,24.7820138994928));
#32228=CARTESIAN_POINT('Ctrl Pts',(55.563762179779,22.9134489285392,24.7826019909393));
#32229=CARTESIAN_POINT('Ctrl Pts',(55.5476241899227,22.9181217726163,24.7836647579728));
#32230=CARTESIAN_POINT('Ctrl Pts',(55.5404358141173,22.9201595028303,24.7841386913768));
#32231=CARTESIAN_POINT('Ctrl Pts',(55.5250616953261,22.9244245229243,24.7851535501004));
#32232=CARTESIAN_POINT('Ctrl Pts',(55.5168728748607,22.9266400691092,24.7856948456783));
#32233=CARTESIAN_POINT('Ctrl Pts',(55.4946475188633,22.9325014122606,24.7871661207754));
#32234=CARTESIAN_POINT('Ctrl Pts',(55.480585169007,22.9360464233084,24.7880993280154));
#32235=CARTESIAN_POINT('Ctrl Pts',(55.4064525763073,22.9538772592639,24.7930319914985));
#32236=CARTESIAN_POINT('Ctrl Pts',(55.3457874409596,22.9655202155769,24.797115040149));
#32237=CARTESIAN_POINT('Ctrl Pts',(55.2447304996243,22.9800919459253,24.8039962631807));
#32238=CARTESIAN_POINT('Ctrl Pts',(55.2046327693612,22.9846356983861,24.8067466482639));
#32239=CARTESIAN_POINT('Ctrl Pts',(55.1644480328175,22.9879598605109,24.8095189920889));
#32240=CARTESIAN_POINT('Origin',(55.,21.,6.22095488139522));
#32241=CARTESIAN_POINT('',(55.1644486115703,22.9879598126352,25.7694502499567));
#32242=CARTESIAN_POINT('',(55.1644483516311,22.987959834138,25.6104387285779));
#32243=CARTESIAN_POINT('',(55.1644483516311,22.987959834138,6.22095488139522));
#32244=CARTESIAN_POINT('Ctrl Pts',(55.1644486115703,22.9879598126352,25.7694502499567));
#32245=CARTESIAN_POINT('Ctrl Pts',(55.1987137427014,22.9851253221169,25.7670853474462));
#32246=CARTESIAN_POINT('Ctrl Pts',(55.2329147190426,22.9814041745798,25.7647034036361));
#32247=CARTESIAN_POINT('Ctrl Pts',(55.3633286894365,22.963788417207,25.7555552787918));
#32248=CARTESIAN_POINT('Ctrl Pts',(55.4585615134211,22.9437578732887,25.7487310203176));
#32249=CARTESIAN_POINT('Ctrl Pts',(55.6050887325483,22.9015657588654,25.7382731815912));
#32250=CARTESIAN_POINT('Ctrl Pts',(55.6575678444106,22.8840622241677,25.7345385385399));
#32251=CARTESIAN_POINT('Ctrl Pts',(55.717963738037,22.8610863550257,25.7303047097285));
#32252=CARTESIAN_POINT('Ctrl Pts',(55.7266478402137,22.8577129149717,25.7296975411362));
#32253=CARTESIAN_POINT('Ctrl Pts',(55.7399491257513,22.8524383333742,25.7287703605073));
#32254=CARTESIAN_POINT('Ctrl Pts',(55.7445831968322,22.8505805445787,25.728447864191));
#32255=CARTESIAN_POINT('Ctrl Pts',(55.7530843413423,22.8471353524798,25.7278572826226));
#32256=CARTESIAN_POINT('Ctrl Pts',(55.7569533865524,22.8455531980367,25.7275888985259));
#32257=CARTESIAN_POINT('Ctrl Pts',(55.7656455325285,22.8419668180063,25.7269868381286));
#32258=CARTESIAN_POINT('Ctrl Pts',(55.7704657422825,22.8399558096826,25.7266535755869));
#32259=CARTESIAN_POINT('Ctrl Pts',(55.7845835491554,22.8340006043129,25.7256791212905));
#32260=CARTESIAN_POINT('Ctrl Pts',(55.7938593205844,22.8300046315442,25.7250409613763));
#32261=CARTESIAN_POINT('Ctrl Pts',(55.8634704866508,22.799387470929,25.7202646175037));
#32262=CARTESIAN_POINT('Ctrl Pts',(55.9224895619041,22.7698563481475,25.7162873093644));
#32263=CARTESIAN_POINT('Ctrl Pts',(56.1304996229599,22.6525362883027,25.7021549861658));
#32264=CARTESIAN_POINT('Ctrl Pts',(56.2693784417955,22.5484145214144,25.6924300500915));
#32265=CARTESIAN_POINT('Ctrl Pts',(56.4298277762251,22.3918524716028,25.6789358331926));
#32266=CARTESIAN_POINT('Ctrl Pts',(56.4651557658104,22.3546138452156,25.675798456889));
#32267=CARTESIAN_POINT('Ctrl Pts',(56.5080429290298,22.3057647825805,25.6717451898777));
#32268=CARTESIAN_POINT('Ctrl Pts',(56.5169725906122,22.2953799781264,25.6708869403508));
#32269=CARTESIAN_POINT('Ctrl Pts',(56.531145310657,22.2785501968891,25.6695010653625));
#32270=CARTESIAN_POINT('Ctrl Pts',(56.5364563791508,22.2721628668902,25.6689762306133));
#32271=CARTESIAN_POINT('Ctrl Pts',(56.5464887966712,22.2599429637516,25.6679742004703));
#32272=CARTESIAN_POINT('Ctrl Pts',(56.5512174436157,22.2541165457146,25.6674973121549));
#32273=CARTESIAN_POINT('Ctrl Pts',(56.5619372666742,22.2407546949579,25.6664055664006));
#32274=CARTESIAN_POINT('Ctrl Pts',(56.5679069560941,22.2332023393362,25.6657898645808));
#32275=CARTESIAN_POINT('Ctrl Pts',(56.583331447765,22.2133955043724,25.6641785133988));
#32276=CARTESIAN_POINT('Ctrl Pts',(56.5926985545834,22.2010738592288,25.6631794451923));
#32277=CARTESIAN_POINT('Ctrl Pts',(56.6808603046209,22.0822594111258,25.6535753605125));
#32278=CARTESIAN_POINT('Ctrl Pts',(56.7489906850262,21.9682955440858,25.6445549407022));
#32279=CARTESIAN_POINT('Ctrl Pts',(56.8458512198371,21.7621958737475,25.6287258172756));
#32280=CARTESIAN_POINT('Ctrl Pts',(56.8801527438242,21.67315338539,25.6220354076973));
#32281=CARTESIAN_POINT('Ctrl Pts',(56.9247054453855,21.5270969724586,25.6115500348712));
#32282=CARTESIAN_POINT('Ctrl Pts',(56.9390768902927,21.471491709778,25.6076682751786));
#32283=CARTESIAN_POINT('Ctrl Pts',(56.9529873697942,21.4061479941851,25.6032903264984));
#32284=CARTESIAN_POINT('Ctrl Pts',(56.9548789845702,21.3969433508574,25.6026778295513));
#32285=CARTESIAN_POINT('Ctrl Pts',(56.9576792288291,21.3828115646912,25.6017442603133));
#32286=CARTESIAN_POINT('Ctrl Pts',(56.9586344287251,21.3778939441162,25.6014206511083));
#32287=CARTESIAN_POINT('Ctrl Pts',(56.9603525654504,21.3688669805552,25.6008289916017));
#32288=CARTESIAN_POINT('Ctrl Pts',(56.9611211109768,21.3647588504085,25.6005606350281));
#32289=CARTESIAN_POINT('Ctrl Pts',(56.9628175290375,21.3555305690075,25.5999598280195));
#32290=CARTESIAN_POINT('Ctrl Pts',(56.9637382805708,21.3504091960823,25.59962778303));
#32291=CARTESIAN_POINT('Ctrl Pts',(56.9660426973824,21.3372972523279,25.5987810653452));
#32292=CARTESIAN_POINT('Ctrl Pts',(56.9673977110284,21.3293016493912,25.5982679634477));
#32293=CARTESIAN_POINT('Ctrl Pts',(56.9751916531498,21.2815454477942,25.5952213143963));
#32294=CARTESIAN_POINT('Ctrl Pts',(56.9804743545328,21.2416024641927,25.592747454608));
#32295=CARTESIAN_POINT('Ctrl Pts',(57.0025758128941,21.0239542000424,25.5795369209107));
#32296=CARTESIAN_POINT('Ctrl Pts',(56.9966960605877,20.8447574200326,25.5695615310469));
#32297=CARTESIAN_POINT('Ctrl Pts',(56.9592821020438,20.6226031753363,25.5561728113888));
#32298=CARTESIAN_POINT('Ctrl Pts',(56.9498962616782,20.5767756674893,25.5533593531232));
#32299=CARTESIAN_POINT('Ctrl Pts',(56.9315693366514,20.5009575520206,25.548587276673));
#32300=CARTESIAN_POINT('Ctrl Pts',(56.9235174912562,20.4707705961186,25.5466557194962));
#32301=CARTESIAN_POINT('Ctrl Pts',(56.9115422466572,20.4297670794274,25.54398315837));
#32302=CARTESIAN_POINT('Ctrl Pts',(56.9082290077694,20.4187759557905,25.5432619206835));
#32303=CARTESIAN_POINT('Ctrl Pts',(56.9024970348965,20.4003385270025,25.5420436159648));
#32304=CARTESIAN_POINT('Ctrl Pts',(56.9001289704138,20.3928766657925,25.5415482128943));
#32305=CARTESIAN_POINT('Ctrl Pts',(56.8953641778733,20.3781635919909,25.5405666753345));
#32306=CARTESIAN_POINT('Ctrl Pts',(56.8929696090625,20.3709118173179,25.540080618982));
#32307=CARTESIAN_POINT('Ctrl Pts',(56.8875997098284,20.3549577699148,25.5390061791335));
#32308=CARTESIAN_POINT('Ctrl Pts',(56.8846057331062,20.346262002641,25.53841718838));
#32309=CARTESIAN_POINT('Ctrl Pts',(56.8738423888088,20.315689231853,25.5363343199171));
#32310=CARTESIAN_POINT('Ctrl Pts',(56.8657515919242,20.2939281571805,25.5348298505742));
#32311=CARTESIAN_POINT('Ctrl Pts',(56.7973254741935,20.1192832269913,25.5225725790334));
#32312=CARTESIAN_POINT('Ctrl Pts',(56.7186950303505,19.9742771673024,25.5111737305711));
#32313=CARTESIAN_POINT('Ctrl Pts',(56.5649908452727,19.7590884269826,25.4927338148515));
#32314=CARTESIAN_POINT('Ctrl Pts',(56.5007184611168,19.6820827106578,25.4857743850951));
#32315=CARTESIAN_POINT('Ctrl Pts',(56.4189681743203,19.5979117277289,25.4779914188751));
#32316=CARTESIAN_POINT('Ctrl Pts',(56.4068500416963,19.5857527758847,25.4768626104906));
#32317=CARTESIAN_POINT('Ctrl Pts',(56.3900130935428,19.5692897261254,25.4753298587012));
#32318=CARTESIAN_POINT('Ctrl Pts',(56.3854287439169,19.564850012639,25.474916065421));
#32319=CARTESIAN_POINT('Ctrl Pts',(56.3776823586011,19.5574197349651,25.4742229149952));
#32320=CARTESIAN_POINT('Ctrl Pts',(56.3745317290066,19.5544174083192,25.4739426615991));
#32321=CARTESIAN_POINT('Ctrl Pts',(56.3685260029905,19.5487317640814,25.4734116438554));
#32322=CARTESIAN_POINT('Ctrl Pts',(56.3656727959931,19.5460465178075,25.4731607263745));
#32323=CARTESIAN_POINT('Ctrl Pts',(56.3581548400927,19.5390127785168,25.472503081986));
#32324=CARTESIAN_POINT('Ctrl Pts',(56.3534770713746,19.5346781749595,25.4720974077733));
#32325=CARTESIAN_POINT('Ctrl Pts',(56.3370595480313,19.5196107480058,25.4706855223959));
#32326=CARTESIAN_POINT('Ctrl Pts',(56.3252119162404,19.5089956448969,25.4696877441147));
#32327=CARTESIAN_POINT('Ctrl Pts',(56.2277076935532,19.4237154408265,25.4616338473089));
#32328=CARTESIAN_POINT('Ctrl Pts',(56.1359294820986,19.3563423914512,25.45502332415));
#32329=CARTESIAN_POINT('Ctrl Pts',(55.945094257375,19.239914863322,25.4420474701758));
#32330=CARTESIAN_POINT('Ctrl Pts',(55.8467243269586,19.1905363247235,25.435699930808));
#32331=CARTESIAN_POINT('Ctrl Pts',(55.6920528987658,19.1282835835363,25.4257026965543));
#32332=CARTESIAN_POINT('Ctrl Pts',(55.6384346344294,19.1093229080778,25.4222367430073));
#32333=CARTESIAN_POINT('Ctrl Pts',(55.5705552912544,19.0885360601271,25.4178129543353));
#32334=CARTESIAN_POINT('Ctrl Pts',(55.5569838004522,19.0845374544169,25.4169267859392));
#32335=CARTESIAN_POINT('Ctrl Pts',(55.5352820159186,19.0783935352728,25.4155065511723));
#32336=CARTESIAN_POINT('Ctrl Pts',(55.5271785438499,19.0761546264718,25.4149755307995));
#32337=CARTESIAN_POINT('Ctrl Pts',(55.511833707776,19.0720192299842,25.4139685514591));
#32338=CARTESIAN_POINT('Ctrl Pts',(55.5045953311176,19.0701121423055,25.4134929453715));
#32339=CARTESIAN_POINT('Ctrl Pts',(55.4881900153905,19.0658884547582,25.4124135802196));
#32340=CARTESIAN_POINT('Ctrl Pts',(55.4790170467408,19.0635962134906,25.4118090471561));
#32341=CARTESIAN_POINT('Ctrl Pts',(55.455341513841,19.0578584345586,25.4102459849503));
#32342=CARTESIAN_POINT('Ctrl Pts',(55.4408162099327,19.0545101379141,25.4092843650881));
#32343=CARTESIAN_POINT('Ctrl Pts',(55.3413278626324,19.0327479598299,25.4026785576816));
#32344=CARTESIAN_POINT('Ctrl Pts',(55.2552889208056,19.0197451693043,25.3968633144754));
#32345=CARTESIAN_POINT('Ctrl Pts',(55.0195324630175,18.9997367425953,25.3806764698064));
#32346=CARTESIAN_POINT('Ctrl Pts',(54.8694411485365,19.0039076819948,25.3700669397672));
#32347=CARTESIAN_POINT('Ctrl Pts',(54.6715682255119,19.0318343432153,25.3564043538794));
#32348=CARTESIAN_POINT('Ctrl Pts',(54.6221786573854,19.0407155730788,25.3530266801714));
#32349=CARTESIAN_POINT('Ctrl Pts',(54.564285719063,19.0533969622904,25.3491452445288));
#32350=CARTESIAN_POINT('Ctrl Pts',(54.5554124616931,19.0554043480942,25.3485525293237));
#32351=CARTESIAN_POINT('Ctrl Pts',(54.5417366368638,19.0585967151658,25.3476427285455));
#32352=CARTESIAN_POINT('Ctrl Pts',(54.5369243614921,19.0597389405891,25.3473232987571));
#32353=CARTESIAN_POINT('Ctrl Pts',(54.5280496332209,19.0618803146879,25.3467355908434));
#32354=CARTESIAN_POINT('Ctrl Pts',(54.5239860976243,19.0628743384554,25.3464670349452));
#32355=CARTESIAN_POINT('Ctrl Pts',(54.5148001264134,19.0651520651995,25.3458611472473));
#32356=CARTESIAN_POINT('Ctrl Pts',(54.5096796513578,19.0664433275995,25.3455242535553));
#32357=CARTESIAN_POINT('Ctrl Pts',(54.4964631959368,19.0698320819651,25.344656732413));
#32358=CARTESIAN_POINT('Ctrl Pts',(54.4883750737319,19.0719602064619,25.3441278097276));
#32359=CARTESIAN_POINT('Ctrl Pts',(54.4371322928298,19.0857882318441,25.3407879589516));
#32360=CARTESIAN_POINT('Ctrl Pts',(54.3943642813671,19.0988864291551,25.3380507863272));
#32361=CARTESIAN_POINT('Ctrl Pts',(54.3294702529646,19.1211736710106,25.3339244024836));
#32362=CARTESIAN_POINT('Ctrl Pts',(54.3070118619256,19.1293407513215,25.3325014201927));
#32363=CARTESIAN_POINT('Ctrl Pts',(54.221587247276,19.1621553775841,25.327089607174));
#32364=CARTESIAN_POINT('Ctrl Pts',(54.1597407705482,19.1895955265956,25.3231719037584));
#32365=CARTESIAN_POINT('Ctrl Pts',(53.9663797051667,19.2874337849833,25.3105997711783));
#32366=CARTESIAN_POINT('Ctrl Pts',(53.841338140746,19.3694329476286,25.3019263243817));
#32367=CARTESIAN_POINT('Ctrl Pts',(53.71334315765,19.4755858480685,25.2916052019623));
#32368=CARTESIAN_POINT('Ctrl Pts',(53.7002263401399,19.4867542365627,25.2905293215721));
#32369=CARTESIAN_POINT('Ctrl Pts',(53.680428187019,19.5040588145211,25.2888764750155));
#32370=CARTESIAN_POINT('Ctrl Pts',(53.6736411084337,19.5100731942793,25.2883045442814));
#32371=CARTESIAN_POINT('Ctrl Pts',(53.6613486404189,19.5211167395031,25.2872588180134));
#32372=CARTESIAN_POINT('Ctrl Pts',(53.6558299623056,19.5261309189819,25.2867856571914));
#32373=CARTESIAN_POINT('Ctrl Pts',(53.6439457020634,19.5370510252227,25.285758631805));
#32374=CARTESIAN_POINT('Ctrl Pts',(53.6375903322752,19.5429677920137,25.2852043111359));
#32375=CARTESIAN_POINT('Ctrl Pts',(53.6203584925594,19.5592217292458,25.2836872151279));
#32376=CARTESIAN_POINT('Ctrl Pts',(53.609559883736,19.5696402630136,25.2827209465972));
#32377=CARTESIAN_POINT('Ctrl Pts',(53.5544839065643,19.6239908258312,25.2777105893766));
#32378=CARTESIAN_POINT('Ctrl Pts',(53.5121715471467,19.6698559806677,25.2735815415471));
#32379=CARTESIAN_POINT('Ctrl Pts',(53.3603285933521,19.850773098871,25.2576460762852));
#32380=CARTESIAN_POINT('Ctrl Pts',(53.2664787650186,19.9979343331679,25.2452961260464));
#32381=CARTESIAN_POINT('Ctrl Pts',(53.1705139197744,20.2032558780712,25.2297746884592));
#32382=CARTESIAN_POINT('Ctrl Pts',(53.1500459799559,20.2520082043859,25.2262102003987));
#32383=CARTESIAN_POINT('Ctrl Pts',(53.1283100090884,20.3101528623972,25.2221438568295));
#32384=CARTESIAN_POINT('Ctrl Pts',(53.1251427658284,20.3188077696421,25.2215433009778));
#32385=CARTESIAN_POINT('Ctrl Pts',(53.1203595096896,20.3321647632041,25.2206240643528));
#32386=CARTESIAN_POINT('Ctrl Pts',(53.1187009518077,20.3368513221767,25.2203029639187));
#32387=CARTESIAN_POINT('Ctrl Pts',(53.1156795724806,20.3454913483539,25.2197136871885));
#32388=CARTESIAN_POINT('Ctrl Pts',(53.1143116678404,20.3494428824373,25.2194452217143));
#32389=CARTESIAN_POINT('Ctrl Pts',(53.1112546477196,20.358364503779,25.218841417915));
#32390=CARTESIAN_POINT('Ctrl Pts',(53.1095727210666,20.3633369648263,25.2185065043475));
#32391=CARTESIAN_POINT('Ctrl Pts',(53.1052949474696,20.3761502256042,25.217647497414));
#32392=CARTESIAN_POINT('Ctrl Pts',(53.102728103208,20.384000704284,25.2171250533664));
#32393=CARTESIAN_POINT('Ctrl Pts',(53.0871510780936,20.4326628863885,25.2139091086782));
#32394=CARTESIAN_POINT('Ctrl Pts',(53.075408468489,20.4738722174298,25.2112832282967));
#32395=CARTESIAN_POINT('Ctrl Pts',(53.0634629608103,20.5215734599231,25.2083209097801));
#32396=CARTESIAN_POINT('Ctrl Pts',(53.0619539879243,20.5277232644443,25.2079404568527));
#32397=CARTESIAN_POINT('Ctrl Pts',(53.0577687344165,20.5451381152892,25.2068669610492));
#32398=CARTESIAN_POINT('Ctrl Pts',(53.0551611882988,20.5564195364914,25.2061761029616));
#32399=CARTESIAN_POINT('Ctrl Pts',(53.0429075624966,20.6116204474346,25.2028151583015));
#32400=CARTESIAN_POINT('Ctrl Pts',(53.0346498716367,20.655836300039,25.2001828725965));
#32401=CARTESIAN_POINT('Ctrl Pts',(53.0128925837776,20.7990026686966,25.1917507212868));
#32402=CARTESIAN_POINT('Ctrl Pts',(53.0053239422665,20.898694736625,25.1860104863481));
#32403=CARTESIAN_POINT('Ctrl Pts',(53.0051907103367,21.0799090277027,25.1753093433157));
#32404=CARTESIAN_POINT('Ctrl Pts',(53.0101103656949,21.1612031272879,25.170412390646));
#32405=CARTESIAN_POINT('Ctrl Pts',(53.0217625348664,21.2565544136016,25.1644434531611));
#32406=CARTESIAN_POINT('Ctrl Pts',(53.0237067659709,21.2711248247565,25.1635252310404));
#32407=CARTESIAN_POINT('Ctrl Pts',(53.0271569043668,21.294967622256,25.1620120252493));
#32408=CARTESIAN_POINT('Ctrl Pts',(53.0285676134974,21.3042533791974,25.1614200419647));
#32409=CARTESIAN_POINT('Ctrl Pts',(53.0312194072802,21.3209150676238,25.1603529121146));
#32410=CARTESIAN_POINT('Ctrl Pts',(53.0324365059465,21.3282946805478,25.1598785326594));
#32411=CARTESIAN_POINT('Ctrl Pts',(53.0351164056717,21.3439932658364,25.1588656081408));
#32412=CARTESIAN_POINT('Ctrl Pts',(53.0365905973743,21.3523101194445,25.158326710118));
#32413=CARTESIAN_POINT('Ctrl Pts',(53.0407076951347,21.3747085536115,25.1568691401507));
#32414=CARTESIAN_POINT('Ctrl Pts',(53.043449526565,21.3887712221637,25.1559473436282));
#32415=CARTESIAN_POINT('Ctrl Pts',(53.0583059357758,21.4608271560232,25.1511888790892));
#32416=CARTESIAN_POINT('Ctrl Pts',(53.07284720207,21.5182840795158,25.1472755411651));
#32417=CARTESIAN_POINT('Ctrl Pts',(53.125923392249,21.6945952213958,25.1348865795288));
#32418=CARTESIAN_POINT('Ctrl Pts',(53.1730731901187,21.8105290853614,25.1261688925054));
#32419=CARTESIAN_POINT('Ctrl Pts',(53.2539703931561,21.9658869139979,25.1139607142313));
#32420=CARTESIAN_POINT('Ctrl Pts',(53.2788777314909,22.0096016120363,25.1104654592546));
#32421=CARTESIAN_POINT('Ctrl Pts',(53.3344303282074,22.0990591336827,25.1032411605051));
#32422=CARTESIAN_POINT('Ctrl Pts',(53.3653726540244,22.1445732597396,25.0995237832423));
#32423=CARTESIAN_POINT('Ctrl Pts',(53.4034361443054,22.1958636218789,25.0953349161264));
#32424=CARTESIAN_POINT('Ctrl Pts',(53.4087597193454,22.2029382043951,25.0947571572306));
#32425=CARTESIAN_POINT('Ctrl Pts',(53.4174230406902,22.2142928793373,25.0938302017551));
#32426=CARTESIAN_POINT('Ctrl Pts',(53.4207333938952,22.2185950998905,25.0934790645787));
#32427=CARTESIAN_POINT('Ctrl Pts',(53.4266332646917,22.2261983034915,25.0928587328654));
#32428=CARTESIAN_POINT('Ctrl Pts',(53.4292156757261,22.2295046852513,25.0925890507336));
#32429=CARTESIAN_POINT('Ctrl Pts',(53.4347998581858,22.2366080643972,25.0920098571577));
#32430=CARTESIAN_POINT('Ctrl Pts',(53.4378050199245,22.2404022872835,25.0917005911911));
#32431=CARTESIAN_POINT('Ctrl Pts',(53.446193135112,22.2509140212713,25.0908439607375));
#32432=CARTESIAN_POINT('Ctrl Pts',(53.4516058827614,22.2576077791068,25.0902986707892));
#32433=CARTESIAN_POINT('Ctrl Pts',(53.4829738471706,22.2958899211716,25.0871799037485));
#32434=CARTESIAN_POINT('Ctrl Pts',(53.5098540068613,22.326711911013,25.0846680261461));
#32435=CARTESIAN_POINT('Ctrl Pts',(53.6033336616256,22.4274709490318,25.0763677402079));
#32436=CARTESIAN_POINT('Ctrl Pts',(53.6740605271425,22.4933980095581,25.0707809079501));
#32437=CARTESIAN_POINT('Ctrl Pts',(53.856592186776,22.6403105570128,25.0571873701118));
#32438=CARTESIAN_POINT('Ctrl Pts',(53.9725373406965,22.7153176723617,25.0491798743587));
#32439=CARTESIAN_POINT('Ctrl Pts',(54.1167541340739,22.7887104366737,25.0392170930963));
#32440=CARTESIAN_POINT('Ctrl Pts',(54.1384267072222,22.7992497517744,25.0377208913161));
#32441=CARTESIAN_POINT('Ctrl Pts',(54.1689895627996,22.8134335723434,25.0356098561294));
#32442=CARTESIAN_POINT('Ctrl Pts',(54.1777238551143,22.8174106867839,25.0350064454044));
#32443=CARTESIAN_POINT('Ctrl Pts',(54.1929147417576,22.8241958547521,25.033956621114));
#32444=CARTESIAN_POINT('Ctrl Pts',(54.1993581850637,22.8270330628305,25.0335112117328));
#32445=CARTESIAN_POINT('Ctrl Pts',(54.2128031623955,22.8328684379433,25.0325815182322));
#32446=CARTESIAN_POINT('Ctrl Pts',(54.219807106966,22.8358607297286,25.0320970431942));
#32447=CARTESIAN_POINT('Ctrl Pts',(54.2363917697655,22.8428341410072,25.0309493763775));
#32448=CARTESIAN_POINT('Ctrl Pts',(54.2459866761908,22.8467807399175,25.0302850298756));
#32449=CARTESIAN_POINT('Ctrl Pts',(54.2779932371539,22.8596547451663,25.0280674125708));
#32450=CARTESIAN_POINT('Ctrl Pts',(54.3005352996268,22.8682501398506,25.0265030946542));
#32451=CARTESIAN_POINT('Ctrl Pts',(54.3545044763139,22.8877151893424,25.0227505152921));
#32452=CARTESIAN_POINT('Ctrl Pts',(54.3860575962214,22.8982116896339,25.0205506601696));
#32453=CARTESIAN_POINT('Ctrl Pts',(54.5799959784933,22.9573862062563,25.006992035006));
#32454=CARTESIAN_POINT('Ctrl Pts',(54.7477669732928,22.9859824683103,24.9950210163085));
#32455=CARTESIAN_POINT('Ctrl Pts',(54.9872897546912,22.9959464872326,24.9784515668118));
#32456=CARTESIAN_POINT('Ctrl Pts',(55.0576018867768,22.9951561742846,24.9736629886231));
#32457=CARTESIAN_POINT('Ctrl Pts',(55.1379314968794,22.9900017360129,24.968378859988));
#32458=CARTESIAN_POINT('Ctrl Pts',(55.148125421962,22.9892689303293,24.9677117846586));
#32459=CARTESIAN_POINT('Ctrl Pts',(55.1603587101088,22.9882949619975,24.9669158040825));
#32460=CARTESIAN_POINT('Ctrl Pts',(55.1624036561328,22.9881289757869,24.966782898771));
#32461=CARTESIAN_POINT('Ctrl Pts',(55.1644483516314,22.9879598341379,24.9666501649259));
#32462=CARTESIAN_POINT('',(53.0052505171966,21.0014364385374,25.0209548813952));
#32463=CARTESIAN_POINT('Ctrl Pts',(55.1644480328175,22.9879598605109,24.8095189920889));
#32464=CARTESIAN_POINT('Ctrl Pts',(55.0694986482504,22.9958142643243,24.8160695474148));
#32465=CARTESIAN_POINT('Ctrl Pts',(54.9740639845202,22.9968597274719,24.8227495899263));
#32466=CARTESIAN_POINT('Ctrl Pts',(54.7885947631868,22.9855771526695,24.8356719559787));
#32467=CARTESIAN_POINT('Ctrl Pts',(54.6987781032876,22.973949870372,24.8418996449565));
#32468=CARTESIAN_POINT('Ctrl Pts',(54.599810923806,22.9542224305118,24.8485268780842));
#32469=CARTESIAN_POINT('Ctrl Pts',(54.5895859910395,22.9521006524244,24.8492086813215));
#32470=CARTESIAN_POINT('Ctrl Pts',(54.5742014826202,22.948781985647,24.8502296723462));
#32471=CARTESIAN_POINT('Ctrl Pts',(54.5690294295359,22.9476447247763,24.8505720851651));
#32472=CARTESIAN_POINT('Ctrl Pts',(54.5597799131597,22.9455722388945,24.8511828822077));
#32473=CARTESIAN_POINT('Ctrl Pts',(54.5557008192255,22.9446447749193,24.8514516977496));
#32474=CARTESIAN_POINT('Ctrl Pts',(54.5468190821993,22.9425959280332,24.85203580544));
#32475=CARTESIAN_POINT('Ctrl Pts',(54.5420176780389,22.9414695665684,24.8523508098508));
#32476=CARTESIAN_POINT('Ctrl Pts',(54.5284320347866,22.9382293069453,24.8532400930335));
#32477=CARTESIAN_POINT('Ctrl Pts',(54.5196577760865,22.9360734870835,24.8538120311549));
#32478=CARTESIAN_POINT('Ctrl Pts',(54.4635245733565,22.92187655774,24.8574573507342));
#32479=CARTESIAN_POINT('Ctrl Pts',(54.4166026810043,22.9081571823331,24.8604422002779));
#32480=CARTESIAN_POINT('Ctrl Pts',(54.2372081337404,22.8484667656616,24.8717785910531));
#32481=CARTESIAN_POINT('Ctrl Pts',(54.1092171139349,22.790305046343,24.8797290338978));
#32482=CARTESIAN_POINT('Ctrl Pts',(53.9046806401534,22.6699501066238,24.8936436136888));
#32483=CARTESIAN_POINT('Ctrl Pts',(53.8247038376438,22.61466193902,24.8994424917228));
#32484=CARTESIAN_POINT('Ctrl Pts',(53.7371820630214,22.5441993382042,24.9064188352943));
#32485=CARTESIAN_POINT('Ctrl Pts',(53.7253983161695,22.534487297231,24.9073721427187));
#32486=CARTESIAN_POINT('Ctrl Pts',(53.7064178262241,22.5184742945385,24.9089313584512));
#32487=CARTESIAN_POINT('Ctrl Pts',(53.6991527158156,22.5122550583766,24.9095339433015));
#32488=CARTESIAN_POINT('Ctrl Pts',(53.6862740296592,22.5010688909484,24.9106126359956));
#32489=CARTESIAN_POINT('Ctrl Pts',(53.6806431615453,22.4961220775187,24.9110879060852));
#32490=CARTESIAN_POINT('Ctrl Pts',(53.6748282058459,22.4909551834413,24.9115825483667));
#32491=CARTESIAN_POINT('Ctrl Pts',(53.6746160832492,22.4907666203233,24.9116005976465));
#32492=CARTESIAN_POINT('Ctrl Pts',(53.6742405962284,22.4904326934249,24.9116325568571));
#32493=CARTESIAN_POINT('Ctrl Pts',(53.6740772154313,22.4902873480239,24.9116464660165));
#32494=CARTESIAN_POINT('Ctrl Pts',(53.6737870509912,22.4900291289757,24.911671174316));
#32495=CARTESIAN_POINT('Ctrl Pts',(53.6736602577595,22.4899162659251,24.9116819730149));
#32496=CARTESIAN_POINT('Ctrl Pts',(53.6734344933636,22.4897152535529,24.9117012042656));
#32497=CARTESIAN_POINT('Ctrl Pts',(53.6733355166616,22.4896271106267,24.9117096365444));
#32498=CARTESIAN_POINT('Ctrl Pts',(53.6731589276725,22.489469819127,24.911724683045));
#32499=CARTESIAN_POINT('Ctrl Pts',(53.6730813119391,22.4894006742915,24.9117312971128));
#32500=CARTESIAN_POINT('Ctrl Pts',(53.6728778291622,22.4892193708762,24.9117486388872));
#32501=CARTESIAN_POINT('Ctrl Pts',(53.6727519710279,22.4891072024914,24.9117593670015));
#32502=CARTESIAN_POINT('Ctrl Pts',(53.6725064295371,22.4888883130017,24.9117803005684));
#32503=CARTESIAN_POINT('Ctrl Pts',(53.6723867447892,22.488781593385,24.9117905059603));
#32504=CARTESIAN_POINT('Ctrl Pts',(53.6721531002008,22.4885732083161,24.9118104319152));
#32505=CARTESIAN_POINT('Ctrl Pts',(53.6720391391556,22.4884715441983,24.9118201524226));
#32506=CARTESIAN_POINT('Ctrl Pts',(53.6718165342088,22.4882729134487,24.9118391429239));
#32507=CARTESIAN_POINT('Ctrl Pts',(53.6717078892287,22.4881759479876,24.9118484128694));
#32508=CARTESIAN_POINT('Ctrl Pts',(53.6714955459617,22.4879863902022,24.9118665334425));
#32509=CARTESIAN_POINT('Ctrl Pts',(53.6713918467396,22.4878937989375,24.9118753840251));
#32510=CARTESIAN_POINT('Ctrl Pts',(53.6711890577208,22.4877126939811,24.9118926942909));
#32511=CARTESIAN_POINT('Ctrl Pts',(53.6710899671371,22.4876241812735,24.9119011539303));
#32512=CARTESIAN_POINT('Ctrl Pts',(53.6708960880452,22.4874509638594,24.9119177082222));
#32513=CARTESIAN_POINT('Ctrl Pts',(53.6708012987304,22.4873662599383,24.9119258028445));
#32514=CARTESIAN_POINT('Ctrl Pts',(53.6706157412565,22.4872004135045,24.9119416507998));
#32515=CARTESIAN_POINT('Ctrl Pts',(53.6705249723595,22.4871192716804,24.911949404107));
#32516=CARTESIAN_POINT('Ctrl Pts',(53.6703471985066,22.4869603234802,24.9119645911416));
#32517=CARTESIAN_POINT('Ctrl Pts',(53.670260192947,22.4868825177742,24.9119720248409));
#32518=CARTESIAN_POINT('Ctrl Pts',(53.6700897096876,22.4867300342585,24.9119865925954));
#32519=CARTESIAN_POINT('Ctrl Pts',(53.670006231586,22.4866553571777,24.9119937266134));
#32520=CARTESIAN_POINT('Ctrl Pts',(53.6698425869416,22.4865089406253,24.9120077132792));
#32521=CARTESIAN_POINT('Ctrl Pts',(53.6697624198444,22.4864372016385,24.9120145659098));
#32522=CARTESIAN_POINT('Ctrl Pts',(53.6628926127019,22.4802886287659,24.9126018584426));
#32523=CARTESIAN_POINT('Ctrl Pts',(53.6561447796106,22.4741654356619,24.9131842453037));
#32524=CARTESIAN_POINT('Ctrl Pts',(53.6365165287981,22.4561073891668,24.9148947291948));
#32525=CARTESIAN_POINT('Ctrl Pts',(53.623751736778,22.4440486800239,24.9160280814115));
#32526=CARTESIAN_POINT('Ctrl Pts',(53.5950020375112,22.4161618084909,24.9186298075048));
#32527=CARTESIAN_POINT('Ctrl Pts',(53.5791225752763,22.4002288450258,24.9201026320038));
#32528=CARTESIAN_POINT('Ctrl Pts',(53.5277394391093,22.3468983816586,24.9249893124848));
#32529=CARTESIAN_POINT('Ctrl Pts',(53.493418431436,22.3083950639374,24.9284503096402));
#32530=CARTESIAN_POINT('Ctrl Pts',(53.3771548011107,22.1673169959474,24.9408916577074));
#32531=CARTESIAN_POINT('Ctrl Pts',(53.303885422737,22.0580386044249,24.9501299119466));
#32532=CARTESIAN_POINT('Ctrl Pts',(53.2054529529215,21.8744003200238,24.9645672612726));
#32533=CARTESIAN_POINT('Ctrl Pts',(53.1729875878152,21.8043652286845,24.9698421783664));
#32534=CARTESIAN_POINT('Ctrl Pts',(53.1408593093562,21.7230009508422,24.975585963564));
#32535=CARTESIAN_POINT('Ctrl Pts',(53.1371363652526,21.7133537494606,24.9762610072975));
#32536=CARTESIAN_POINT('Ctrl Pts',(53.1316281004472,21.6987430289135,24.9772738854839));
#32537=CARTESIAN_POINT('Ctrl Pts',(53.1297872393542,21.6938008409931,24.9776148714347));
#32538=CARTESIAN_POINT('Ctrl Pts',(53.1265218522209,21.6849267698452,24.9782241486304));
#32539=CARTESIAN_POINT('Ctrl Pts',(53.1250900755792,21.6809976700276,24.9784928618732));
#32540=CARTESIAN_POINT('Ctrl Pts',(53.1219909440572,21.6724091293542,24.9790779379945));
#32541=CARTESIAN_POINT('Ctrl Pts',(53.1203285708724,21.6677479848315,24.9793940055533));
#32542=CARTESIAN_POINT('Ctrl Pts',(53.1156539637337,21.6544850198008,24.980289331709));
#32543=CARTESIAN_POINT('Ctrl Pts',(53.1126832644326,21.6458685413581,24.9808661989606));
#32544=CARTESIAN_POINT('Ctrl Pts',(53.0936183491421,21.5893160550945,24.9846228963687));
#32545=CARTESIAN_POINT('Ctrl Pts',(53.079291264784,21.5407987876339,24.9877078373612));
#32546=CARTESIAN_POINT('Ctrl Pts',(53.0260467787715,21.3314979314074,25.0006390514469));
#32547=CARTESIAN_POINT('Ctrl Pts',(53.0053636459116,21.1667638399575,25.0099340749681));
#32548=CARTESIAN_POINT('Ctrl Pts',(53.0052504670078,21.0013649643292,25.019750596888));
#32549=CARTESIAN_POINT('Ctrl Pts',(53.0052505171966,21.0014364385374,25.0209548813952));
#32550=CARTESIAN_POINT('Ctrl Pts',(53.0052001533975,20.9314973777562,25.0254037518945));
#32551=CARTESIAN_POINT('Ctrl Pts',(53.0088323744059,20.8615259841515,25.0298526223938));
#32552=CARTESIAN_POINT('Ctrl Pts',(53.016130795315,20.7919362088143,25.0343014928931));
#32553=CARTESIAN_POINT('Ctrl Pts',(53.0234288322359,20.7223500947698,25.0387501293261));
#32554=CARTESIAN_POINT('Ctrl Pts',(53.0343926343225,20.6531460421601,25.0431987657592));
#32555=CARTESIAN_POINT('Ctrl Pts',(53.048953970378,20.5847326730935,25.0476474021923));
#32556=CARTESIAN_POINT('Ctrl Pts',(53.0642055004891,20.5130765726949,25.0523068999371));
#32557=CARTESIAN_POINT('Ctrl Pts',(53.0834039916007,20.4422885516444,25.056966397682));
#32558=CARTESIAN_POINT('Ctrl Pts',(53.1064115872689,20.3728234015283,25.0616258954268));
#32559=CARTESIAN_POINT('Ctrl Pts',(53.1284128967115,20.3063964577825,25.0660816001084));
#32560=CARTESIAN_POINT('Ctrl Pts',(53.1538968136819,20.2411795245564,25.0705373047901));
#32561=CARTESIAN_POINT('Ctrl Pts',(53.1826932359489,20.1775501912979,25.0749930094717));
#32562=CARTESIAN_POINT('Ctrl Pts',(53.2115124075885,20.1138705904264,25.0794522341908));
#32563=CARTESIAN_POINT('Ctrl Pts',(53.2436490666211,20.0517815147258,25.0839114589099));
#32564=CARTESIAN_POINT('Ctrl Pts',(53.2788875824894,19.9916351807055,25.088370683629));
#32565=CARTESIAN_POINT('Ctrl Pts',(53.3141870948961,19.9313847356555,25.0928376270975));
#32566=CARTESIAN_POINT('Ctrl Pts',(53.3525989041981,19.8730841418326,25.097304570566));
#32567=CARTESIAN_POINT('Ctrl Pts',(53.3938652082761,19.8170551182265,25.1017715140344));
#32568=CARTESIAN_POINT('Ctrl Pts',(53.3993768780767,19.8095716887248,25.1023681343998));
#32569=CARTESIAN_POINT('Ctrl Pts',(53.4049394140699,19.8021287303179,25.1029647547651));
#32570=CARTESIAN_POINT('Ctrl Pts',(53.4105521515587,19.7947269605664,25.1035613751305));
#32571=CARTESIAN_POINT('Ctrl Pts',(53.4524588730015,19.739462679318,25.1080159578556));
#32572=CARTESIAN_POINT('Ctrl Pts',(53.4973340371494,19.6862774989079,25.1124705405806));
#32573=CARTESIAN_POINT('Ctrl Pts',(53.5449437481546,19.6355078356892,25.1169251233057));
#32574=CARTESIAN_POINT('Ctrl Pts',(53.5924820341012,19.5848143381537,25.121373023175));
#32575=CARTESIAN_POINT('Ctrl Pts',(53.6427463924562,19.5365295194779,25.1258209230443));
#32576=CARTESIAN_POINT('Ctrl Pts',(53.6954616143976,19.4909581970701,25.1302688229135));
#32577=CARTESIAN_POINT('Ctrl Pts',(53.748114857069,19.4454404545809,25.1347114932196));
#32578=CARTESIAN_POINT('Ctrl Pts',(53.8032128716403,19.402630190384,25.1391541635256));
#32579=CARTESIAN_POINT('Ctrl Pts',(53.8604436771806,19.362795385536,25.1435968338317));
#32580=CARTESIAN_POINT('Ctrl Pts',(53.9176384992424,19.3229856265497,25.1480367108391));
#32581=CARTESIAN_POINT('Ctrl Pts',(53.9769630512782,19.2861478945724,25.1524765878465));
#32582=CARTESIAN_POINT('Ctrl Pts',(54.0380735607145,19.2525089162163,25.1569164648539));
#32583=CARTESIAN_POINT('Ctrl Pts',(54.0991663979844,19.2188796657061,25.161355057921));
#32584=CARTESIAN_POINT('Ctrl Pts',(54.1620437388259,19.1884475683449,25.1657936509881));
#32585=CARTESIAN_POINT('Ctrl Pts',(54.2263357484426,19.1613942270399,25.1702322440552));
#32586=CARTESIAN_POINT('Ctrl Pts',(54.2906309961562,19.1343395231808,25.1746710606741));
#32587=CARTESIAN_POINT('Ctrl Pts',(54.3563406020663,19.1106641008342,25.179109877293));
#32588=CARTESIAN_POINT('Ctrl Pts',(54.4230748723272,19.0905013852951,25.1835486939119));
#32589=CARTESIAN_POINT('Ctrl Pts',(54.4898797455656,19.0703173381712,25.1879922066737));
#32590=CARTESIAN_POINT('Ctrl Pts',(54.5577109774409,19.0536535572182,25.1924357194355));
#32591=CARTESIAN_POINT('Ctrl Pts',(54.6261647640543,19.0405932584414,25.1968792321974));
#32592=CARTESIAN_POINT('Ctrl Pts',(54.6946585840436,19.0275253216963,25.2013253436294));
#32593=CARTESIAN_POINT('Ctrl Pts',(54.7637751984106,19.0180651280658,25.2057714550614));
#32594=CARTESIAN_POINT('Ctrl Pts',(54.8331044622872,19.0122441191153,25.2102175664935));
#32595=CARTESIAN_POINT('Ctrl Pts',(54.9025542274361,19.0064129926626,25.2146714057168));
#32596=CARTESIAN_POINT('Ctrl Pts',(54.9722168907849,19.0042336923204,25.2191252449402));
#32597=CARTESIAN_POINT('Ctrl Pts',(55.0416818868452,19.0056855356266,25.2235790841636));
#32598=CARTESIAN_POINT('Ctrl Pts',(55.078155111173,19.006447839083,25.2259176127222));
#32599=CARTESIAN_POINT('Ctrl Pts',(55.1145739153244,19.0082103327259,25.2282561412809));
#32600=CARTESIAN_POINT('Ctrl Pts',(55.1508797507476,19.0109643383503,25.2305946698395));
#32601=CARTESIAN_POINT('Ctrl Pts',(55.2200375291387,19.0162103520679,25.2350492551131));
#32602=CARTESIAN_POINT('Ctrl Pts',(55.2890579270999,19.0250778938475,25.2395038403867));
#32603=CARTESIAN_POINT('Ctrl Pts',(55.3575314519216,19.0375528482563,25.2439584256602));
#32604=CARTESIAN_POINT('Ctrl Pts',(55.4259022511927,19.0500090874527,25.2484063280629));
#32605=CARTESIAN_POINT('Ctrl Pts',(55.4937273281079,19.0660619108251,25.2528542304656));
#32606=CARTESIAN_POINT('Ctrl Pts',(55.5606013397307,19.0856453566823,25.2573021328683));
#32607=CARTESIAN_POINT('Ctrl Pts',(55.6273967245928,19.105205777408,25.2617448056735));
#32608=CARTESIAN_POINT('Ctrl Pts',(55.6932427976504,19.1282884390331,25.2661874784788));
#32609=CARTESIAN_POINT('Ctrl Pts',(55.7577452285476,19.1547765091693,25.2706301512841));
#32610=CARTESIAN_POINT('Ctrl Pts',(55.8222071036778,19.1812479249875,25.2750700307682));
#32611=CARTESIAN_POINT('Ctrl Pts',(55.885326560898,19.2111203162352,25.2795099102524));
#32612=CARTESIAN_POINT('Ctrl Pts',(55.9467266951757,19.2442277690026,25.2839497897365));
#32613=CARTESIAN_POINT('Ctrl Pts',(56.0081090731831,19.2773256474444,25.2883883852544));
#32614=CARTESIAN_POINT('Ctrl Pts',(56.0677726847449,19.3136564979985,25.2928269807723));
#32615=CARTESIAN_POINT('Ctrl Pts',(56.1253644078508,19.3530080412939,25.2972655762902));
#32616=CARTESIAN_POINT('Ctrl Pts',(56.1829590312068,19.3923615662858,25.3017043953304));
#32617=CARTESIAN_POINT('Ctrl Pts',(56.2384811562253,19.4347358079341,25.3061432143706));
#32618=CARTESIAN_POINT('Ctrl Pts',(56.2916073734096,19.4798756776323,25.3105820334109));
#32619=CARTESIAN_POINT('Ctrl Pts',(56.3447897958764,19.5250633033963,25.3150255485332));
#32620=CARTESIAN_POINT('Ctrl Pts',(56.3955708776067,19.5730220795878,25.3194690636556));
#32621=CARTESIAN_POINT('Ctrl Pts',(56.4436617459362,19.6234578372529,25.3239125787779));
#32622=CARTESIAN_POINT('Ctrl Pts',(56.4917807385802,19.6739230905616,25.3283586925395));
#32623=CARTESIAN_POINT('Ctrl Pts',(56.5372060676061,19.7268678370387,25.332804806301));
#32624=CARTESIAN_POINT('Ctrl Pts',(56.5796889248339,19.7819645065693,25.3372509200626));
#32625=CARTESIAN_POINT('Ctrl Pts',(56.6222456208304,19.8371569387321,25.3417047615427));
#32626=CARTESIAN_POINT('Ctrl Pts',(56.6618493581873,19.8945083572998,25.3461586030229));
#32627=CARTESIAN_POINT('Ctrl Pts',(56.6982948970917,19.9536625759287,25.350612444503));
#32628=CARTESIAN_POINT('Ctrl Pts',(56.7174307681436,19.9847217270316,25.3529509511848));
#32629=CARTESIAN_POINT('Ctrl Pts',(56.7356967523851,20.0162774680169,25.3552894578666));
#32630=CARTESIAN_POINT('Ctrl Pts',(56.7530683958959,20.048275900373,25.3576279645484));
#32631=CARTESIAN_POINT('Ctrl Pts',(56.7861594011771,20.1092292749587,25.3620825538283));
#32632=CARTESIAN_POINT('Ctrl Pts',(56.8161329725906,20.1720308909635,25.3665371431082));
#32633=CARTESIAN_POINT('Ctrl Pts',(56.842778934709,20.2363290235365,25.3709917323881));
#32634=CARTESIAN_POINT('Ctrl Pts',(56.8693849222466,20.3005306953068,25.3754396388416));
#32635=CARTESIAN_POINT('Ctrl Pts',(56.8926730228657,20.3662239791824,25.3798875452951));
#32636=CARTESIAN_POINT('Ctrl Pts',(56.9124788743392,20.4330325250015,25.3843354517486));
#32637=CARTESIAN_POINT('Ctrl Pts',(56.9322614394135,20.499762521788,25.3887781286503));
#32638=CARTESIAN_POINT('Ctrl Pts',(56.9485697485646,20.5676047092078,25.393220805552));
#32639=CARTESIAN_POINT('Ctrl Pts',(56.9612881542128,20.6361644071224,25.3976634824538));
#32640=CARTESIAN_POINT('Ctrl Pts',(56.9739985632717,20.7046809987109,25.4021033660602));
#32641=CARTESIAN_POINT('Ctrl Pts',(56.9831234574383,20.7739137257499,25.4065432496667));
#32642=CARTESIAN_POINT('Ctrl Pts',(56.9885978775687,20.8434559364608,25.4109831332731));
#32643=CARTESIAN_POINT('Ctrl Pts',(56.9940707145801,20.9129780366231,25.4154217329329));
#32644=CARTESIAN_POINT('Ctrl Pts',(56.9958951348644,20.9828089551278,25.4198603325926));
#32645=CARTESIAN_POINT('Ctrl Pts',(56.9940580328572,21.0525368832141,25.4242989322523));
#32646=CARTESIAN_POINT('Ctrl Pts',(56.9922208383303,21.1222683229188,25.4287377554475));
#32647=CARTESIAN_POINT('Ctrl Pts',(56.9867217707048,21.1918962727284,25.4331765786427));
#32648=CARTESIAN_POINT('Ctrl Pts',(56.9775998050228,21.2610106773175,25.437615401838));
#32649=CARTESIAN_POINT('Ctrl Pts',(56.9684681887157,21.3301982018052,25.4420589211064));
#32650=CARTESIAN_POINT('Ctrl Pts',(56.9557060884259,21.3988706105079,25.4465024403748));
#32651=CARTESIAN_POINT('Ctrl Pts',(56.9394040425061,21.4666256769734,25.4509459596432));
#32652=CARTESIAN_POINT('Ctrl Pts',(56.9230924628923,21.5344203676728,25.4553920775519));
#32653=CARTESIAN_POINT('Ctrl Pts',(56.9032369564458,21.6012961790338,25.4598381954606));
#32654=CARTESIAN_POINT('Ctrl Pts',(56.8799778501924,21.6668664373665,25.4642843133693));
#32655=CARTESIAN_POINT('Ctrl Pts',(56.8566783179238,21.7325506615686,25.4687381589537));
#32656=CARTESIAN_POINT('Ctrl Pts',(56.8299635648336,21.7969243512478,25.4731920045381));
#32657=CARTESIAN_POINT('Ctrl Pts',(56.8000215860336,21.8596219240533,25.4776458501225));
#32658=CARTESIAN_POINT('Ctrl Pts',(56.7843006973762,21.892540976189,25.4799843198342));
#32659=CARTESIAN_POINT('Ctrl Pts',(56.7676909130401,21.9249983947807,25.4823227895458));
#32660=CARTESIAN_POINT('Ctrl Pts',(56.7502242594158,21.9569444102206,25.4846612592574));
#32661=CARTESIAN_POINT('Ctrl Pts',(56.7169516615478,22.0177990506161,25.4891158596643));
#32662=CARTESIAN_POINT('Ctrl Pts',(56.6804357450355,22.0770364677886,25.4935704600712));
#32663=CARTESIAN_POINT('Ctrl Pts',(56.6408580806643,22.1342893465156,25.498025060478));
#32664=CARTESIAN_POINT('Ctrl Pts',(56.6013398682158,22.1914562223474,25.5024729693693));
#32665=CARTESIAN_POINT('Ctrl Pts',(56.5587693124784,22.2466440772406,25.5069208782606));
#32666=CARTESIAN_POINT('Ctrl Pts',(56.5133735161578,22.2995107398911,25.5113687871518));
#32667=CARTESIAN_POINT('Ctrl Pts',(56.468031430981,22.35231485206,25.5158114333911));
#32668=CARTESIAN_POINT('Ctrl Pts',(56.4198710620093,22.4028028573868,25.5202540796305));
#32669=CARTESIAN_POINT('Ctrl Pts',(56.3691613222879,22.4506635847263,25.5246967258698));
#32670=CARTESIAN_POINT('Ctrl Pts',(56.3184836056079,22.4984940881667,25.529136566592));
#32671=CARTESIAN_POINT('Ctrl Pts',(56.2652600671528,22.5437002699515,25.5335764073142));
#32672=CARTESIAN_POINT('Ctrl Pts',(56.2097971603903,22.5860070596349,25.5380162480364));
#32673=CARTESIAN_POINT('Ctrl Pts',(56.1543504450653,22.6283014985818,25.5424547926238));
#32674=CARTESIAN_POINT('Ctrl Pts',(56.0966660482703,22.6676979292194,25.5468933372112));
#32675=CARTESIAN_POINT('Ctrl Pts',(56.0370828691747,22.7039620550248,25.5513318817986));
#32676=CARTESIAN_POINT('Ctrl Pts',(55.9774968527151,22.7402279077358,25.5557706377505));
#32677=CARTESIAN_POINT('Ctrl Pts',(55.9160122938274,22.7733609072408,25.5602093937023));
#32678=CARTESIAN_POINT('Ctrl Pts',(55.8529948537301,22.8031714677229,25.5646481496542));
#32679=CARTESIAN_POINT('Ctrl Pts',(55.7899127541798,22.8330126155239,25.5690914600204));
#32680=CARTESIAN_POINT('Ctrl Pts',(55.7252950778109,22.8595243114278,25.5735347703865));
#32681=CARTESIAN_POINT('Ctrl Pts',(55.6595288283531,22.8825645505722,25.5779780807527));
#32682=CARTESIAN_POINT('Ctrl Pts',(55.5937241886818,22.9056182391639,25.582423984845));
#32683=CARTESIAN_POINT('Ctrl Pts',(55.526770111227,22.9251963003124,25.5868698889372));
#32684=CARTESIAN_POINT('Ctrl Pts',(55.4590675248692,22.9412069879615,25.5913157930294));
#32685=CARTESIAN_POINT('Ctrl Pts',(55.3912521515552,22.9572443481031,25.5957691036332));
#32686=CARTESIAN_POINT('Ctrl Pts',(55.3226862619325,22.9697023868234,25.600222414237));
#32687=CARTESIAN_POINT('Ctrl Pts',(55.2537788206309,22.9785408443343,25.6046757248408));
#32688=CARTESIAN_POINT('Ctrl Pts',(55.2240545789698,22.9823534434093,25.6065967260865));
#32689=CARTESIAN_POINT('Ctrl Pts',(55.1942668153676,22.9854931861074,25.6085177273322));
#32690=CARTESIAN_POINT('Ctrl Pts',(55.1644483516311,22.987959834138,25.6104387285779));
#32691=CARTESIAN_POINT('Origin',(55.,21.,6.22095488139522));
#32692=CARTESIAN_POINT('',(55.1644483516311,22.987959834138,26.5685072087751));
#32693=CARTESIAN_POINT('',(55.1643728891593,22.9868942741083,26.4105573801158));
#32694=CARTESIAN_POINT('',(55.1644483516311,22.987959834138,6.22095488139522));
#32695=CARTESIAN_POINT('',(53.005250049757,20.9995544605957,25.9790451186048));
#32696=CARTESIAN_POINT('Ctrl Pts',(53.005250049757,20.9995544605957,25.9790451186048));
#32697=CARTESIAN_POINT('Ctrl Pts',(53.0052554859099,20.9752159494636,25.9806079598459));
#32698=CARTESIAN_POINT('Ctrl Pts',(53.0057063467274,20.9508829793038,25.982170801087));
#32699=CARTESIAN_POINT('Ctrl Pts',(53.0066021269694,20.9265664770214,25.9837336423282));
#32700=CARTESIAN_POINT('Ctrl Pts',(53.0091549439874,20.8572686984656,25.9881874665249));
#32701=CARTESIAN_POINT('Ctrl Pts',(53.0153306838428,20.78796709998,25.9926412907217));
#32702=CARTESIAN_POINT('Ctrl Pts',(53.0251312383553,20.7190712959132,25.9970951149184));
#32703=CARTESIAN_POINT('Ctrl Pts',(53.0349170842458,20.6502788903161,26.0015422548387));
#32704=CARTESIAN_POINT('Ctrl Pts',(53.0483168791449,20.5818915511762,26.0059893947589));
#32705=CARTESIAN_POINT('Ctrl Pts',(53.0652805461648,20.5143167725238,26.0104365346791));
#32706=CARTESIAN_POINT('Ctrl Pts',(53.0822242708594,20.4468214341374,26.014878446584));
#32707=CARTESIAN_POINT('Ctrl Pts',(53.1027234278885,20.3801372316042,26.0193203584889));
#32708=CARTESIAN_POINT('Ctrl Pts',(53.1266766784958,20.3146626410238,26.0237622703938));
#32709=CARTESIAN_POINT('Ctrl Pts',(53.1506148735093,20.2492292038907,26.0282013903761));
#32710=CARTESIAN_POINT('Ctrl Pts',(53.178002687431,20.1850043292041,26.0326405103585));
#32711=CARTESIAN_POINT('Ctrl Pts',(53.2086890578424,20.1223709946644,26.0370796303408));
#32712=CARTESIAN_POINT('Ctrl Pts',(53.2393665699213,20.059755740689,26.0415174688682));
#32713=CARTESIAN_POINT('Ctrl Pts',(53.2733405328967,19.9987315542473,26.0459553073956));
#32714=CARTESIAN_POINT('Ctrl Pts',(53.3104126278366,19.9396594536065,26.050393145923));
#32715=CARTESIAN_POINT('Ctrl Pts',(53.347486620293,19.88058432939,26.054831211599));
#32716=CARTESIAN_POINT('Ctrl Pts',(53.3876587972494,19.8234619027611,26.0592692772749));
#32717=CARTESIAN_POINT('Ctrl Pts',(53.430686907246,19.7686251669736,26.0637073429508));
#32718=CARTESIAN_POINT('Ctrl Pts',(53.4737606498378,19.7137302751906,26.0681501153279));
#32719=CARTESIAN_POINT('Ctrl Pts',(53.5196960678683,19.6611262983735,26.072592887705));
#32720=CARTESIAN_POINT('Ctrl Pts',(53.5682105163276,19.6111132382569,26.0770356600821));
#32721=CARTESIAN_POINT('Ctrl Pts',(53.6167533952926,19.5610708694161,26.081481036019));
#32722=CARTESIAN_POINT('Ctrl Pts',(53.6678779538738,19.5136227724311,26.0859264119558));
#32723=CARTESIAN_POINT('Ctrl Pts',(53.7212666166781,19.4690302103313,26.0903717878927));
#32724=CARTESIAN_POINT('Ctrl Pts',(53.7747482750312,19.4243599742542,26.0948249070497));
#32725=CARTESIAN_POINT('Ctrl Pts',(53.8305015182019,19.3825554953541,26.0992780262068));
#32726=CARTESIAN_POINT('Ctrl Pts',(53.8881784858555,19.3438356110623,26.1037311453639));
#32727=CARTESIAN_POINT('Ctrl Pts',(53.9185544324252,19.3234435345665,26.106076409255));
#32728=CARTESIAN_POINT('Ctrl Pts',(53.9494635164362,19.3039062662285,26.1084216731461));
#32729=CARTESIAN_POINT('Ctrl Pts',(53.9808523549507,19.2852505605511,26.1107669370371));
#32730=CARTESIAN_POINT('Ctrl Pts',(54.0404847602063,19.2498085163744,26.1152224611471));
#32731=CARTESIAN_POINT('Ctrl Pts',(54.1020857201306,19.2174109949132,26.119677985257));
#32732=CARTESIAN_POINT('Ctrl Pts',(54.1653117999386,19.1882817075554,26.1241335093669));
#32733=CARTESIAN_POINT('Ctrl Pts',(54.2284429897427,19.1591961375719,26.1285823466049));
#32734=CARTESIAN_POINT('Ctrl Pts',(54.2931940178165,19.1333692693402,26.1330311838428));
#32735=CARTESIAN_POINT('Ctrl Pts',(54.3591950686674,19.110979988862,26.1374800210808));
#32736=CARTESIAN_POINT('Ctrl Pts',(54.4251183823711,19.0886170788547,26.1419236184034));
#32737=CARTESIAN_POINT('Ctrl Pts',(54.4922883335603,19.0696838712695,26.1463672157261));
#32738=CARTESIAN_POINT('Ctrl Pts',(54.5603149029982,19.0543112844099,26.1508108130488));
#32739=CARTESIAN_POINT('Ctrl Pts',(54.6282986042985,19.038948384856,26.1552516101606));
#32740=CARTESIAN_POINT('Ctrl Pts',(54.6971373768873,19.0271417623195,26.1596924072723));
#32741=CARTESIAN_POINT('Ctrl Pts',(54.7664272707845,19.0189721499517,26.1641332043841));
#32742=CARTESIAN_POINT('Ctrl Pts',(54.8356970030509,19.0108049147374,26.1685727093346));
#32743=CARTESIAN_POINT('Ctrl Pts',(54.9054171104519,19.0062726460233,26.1730122142852));
#32744=CARTESIAN_POINT('Ctrl Pts',(54.9751764736149,19.0054044632964,26.1774517192358));
#32745=CARTESIAN_POINT('Ctrl Pts',(55.0449391996525,19.0045362387172,26.1818914382006));
#32746=CARTESIAN_POINT('Ctrl Pts',(55.114740696023,19.0073324544971,26.1863311571655));
#32747=CARTESIAN_POINT('Ctrl Pts',(55.184169567371,19.0137701208182,26.1907708761303));
#32748=CARTESIAN_POINT('Ctrl Pts',(55.2536715568894,19.0202145668893,26.1952152707311));
#32749=CARTESIAN_POINT('Ctrl Pts',(55.3227996500613,19.0303080725577,26.1996596653319));
#32750=CARTESIAN_POINT('Ctrl Pts',(55.3911482661161,19.043975819062,26.2041040599327));
#32751=CARTESIAN_POINT('Ctrl Pts',(55.4595366871907,19.057651525419,26.20855104287));
#32752=CARTESIAN_POINT('Ctrl Pts',(55.5271442534278,19.0749054948847,26.2129980258072));
#32753=CARTESIAN_POINT('Ctrl Pts',(55.5935789799403,19.0956125506943,26.2174450087445));
#32754=CARTESIAN_POINT('Ctrl Pts',(55.6601287766886,19.1163554727733,26.2218996942103));
#32755=CARTESIAN_POINT('Ctrl Pts',(55.7255012199284,19.1405632503944,26.2263543796761));
#32756=CARTESIAN_POINT('Ctrl Pts',(55.7893235384156,19.1680622515481,26.2308090651418));
#32757=CARTESIAN_POINT('Ctrl Pts',(55.8227110405595,19.1824478611865,26.2331394540099));
#32758=CARTESIAN_POINT('Ctrl Pts',(55.8556747182556,19.197733397104,26.235469842878));
#32759=CARTESIAN_POINT('Ctrl Pts',(55.8881641213877,19.2138891255077,26.2378002317461));
#32760=CARTESIAN_POINT('Ctrl Pts',(55.9502810579926,19.2447774847976,26.2422557342678));
#32761=CARTESIAN_POINT('Ctrl Pts',(56.010906875813,19.2789708724776,26.2467112367896));
#32762=CARTESIAN_POINT('Ctrl Pts',(56.0696674020691,19.3163019239036,26.2511667393113));
#32763=CARTESIAN_POINT('Ctrl Pts',(56.128339977417,19.3535770993855,26.2556155729769));
#32764=CARTESIAN_POINT('Ctrl Pts',(56.1851523930307,19.3939803570567,26.2600644066425));
#32765=CARTESIAN_POINT('Ctrl Pts',(56.239753849348,19.4372978673059,26.2645132403082));
#32766=CARTESIAN_POINT('Ctrl Pts',(56.2942913182649,19.4805646138015,26.2689568603894));
#32767=CARTESIAN_POINT('Ctrl Pts',(56.3466225926864,19.5267385271277,26.2734004804706));
#32768=CARTESIAN_POINT('Ctrl Pts',(56.3964262326221,19.5755627990871,26.2778441005518));
#32769=CARTESIAN_POINT('Ctrl Pts',(56.4461986700604,19.6243564821331,26.2822849366589));
#32770=CARTESIAN_POINT('Ctrl Pts',(56.4934462660713,19.6757968880417,26.286725772766));
#32771=CARTESIAN_POINT('Ctrl Pts',(56.5378822056027,19.7295883013013,26.2911666088731));
#32772=CARTESIAN_POINT('Ctrl Pts',(56.5823053758943,19.7833642569052,26.2956061688487));
#32773=CARTESIAN_POINT('Ctrl Pts',(56.6239181823223,19.8394895017036,26.3000457288243));
#32774=CARTESIAN_POINT('Ctrl Pts',(56.6624732994973,19.8976343206729,26.3044852888));
#32775=CARTESIAN_POINT('Ctrl Pts',(56.701030412825,19.9557821500321,26.3089250786294));
#32776=CARTESIAN_POINT('Ctrl Pts',(56.7365292542682,20.0159493521424,26.3133648684588));
#32777=CARTESIAN_POINT('Ctrl Pts',(56.7687661404784,20.07777773677,26.3178046582882));
#32778=CARTESIAN_POINT('Ctrl Pts',(56.8010371446848,20.1396715576366,26.3222491469812));
#32779=CARTESIAN_POINT('Ctrl Pts',(56.8300390765395,20.2032296354737,26.3266936356742));
#32780=CARTESIAN_POINT('Ctrl Pts',(56.8556149590916,20.2680705730089,26.3311381243673));
#32781=CARTESIAN_POINT('Ctrl Pts',(56.8812058129006,20.3329494662366,26.3355852147137));
#32782=CARTESIAN_POINT('Ctrl Pts',(56.9033664702261,20.3991122498787,26.3400323050602));
#32783=CARTESIAN_POINT('Ctrl Pts',(56.9219896428977,20.4661616582768,26.3444793954066));
#32784=CARTESIAN_POINT('Ctrl Pts',(56.9406451526124,20.5333274904253,26.3489342076249));
#32785=CARTESIAN_POINT('Ctrl Pts',(56.9557508104675,20.601382542975,26.3533890198431));
#32786=CARTESIAN_POINT('Ctrl Pts',(56.9672504622757,20.6699194322955,26.3578438320614));
#32787=CARTESIAN_POINT('Ctrl Pts',(56.9732648610753,20.7057647075902,26.3601737301926));
#32788=CARTESIAN_POINT('Ctrl Pts',(56.9782937493876,20.7417416945414,26.3625036283239));
#32789=CARTESIAN_POINT('Ctrl Pts',(56.9823347679958,20.7777919216255,26.3648335264551));
#32790=CARTESIAN_POINT('Ctrl Pts',(56.9900512974037,20.84663165349,26.3692825847718));
#32791=CARTESIAN_POINT('Ctrl Pts',(56.9941931550845,20.9160117809082,26.3737316430885));
#32792=CARTESIAN_POINT('Ctrl Pts',(56.9946975038501,20.9855282815713,26.3781807014052));
#32793=CARTESIAN_POINT('Ctrl Pts',(56.9952010934743,21.0549401466075,26.3826230630384));
#32794=CARTESIAN_POINT('Ctrl Pts',(56.9920780367055,21.1244874908298,26.3870654246715));
#32795=CARTESIAN_POINT('Ctrl Pts',(56.9853171987077,21.1937606332963,26.3915077863047));
#32796=CARTESIAN_POINT('Ctrl Pts',(56.9785643105686,21.262952319633,26.3959449243032));
#32797=CARTESIAN_POINT('Ctrl Pts',(56.9681821837198,21.3318699584875,26.4003820623017));
#32798=CARTESIAN_POINT('Ctrl Pts',(56.9542117163663,21.4001051488253,26.4048192003002));
#32799=CARTESIAN_POINT('Ctrl Pts',(56.9402500230965,21.4682974843858,26.4092535515759));
#32800=CARTESIAN_POINT('Ctrl Pts',(56.9227045578704,21.5358077419548,26.4136879028516));
#32801=CARTESIAN_POINT('Ctrl Pts',(56.9016676942168,21.6022354550108,26.4181222541273));
#32802=CARTESIAN_POINT('Ctrl Pts',(56.8806368525617,21.6686441525142,26.4225553360286));
#32803=CARTESIAN_POINT('Ctrl Pts',(56.8561167444901,21.7339704530156,26.4269884179299));
#32804=CARTESIAN_POINT('Ctrl Pts',(56.8282497352792,21.7978285955966,26.4314214998312));
#32805=CARTESIAN_POINT('Ctrl Pts',(56.8003811789297,21.8616902834951,26.4358548278512));
#32806=CARTESIAN_POINT('Ctrl Pts',(56.7691655510603,21.924083202831,26.4402881558712));
#32807=CARTESIAN_POINT('Ctrl Pts',(56.734792814888,21.9846428042255,26.4447214838912));
#32808=CARTESIAN_POINT('Ctrl Pts',(56.7003831145663,22.0452675309024,26.4491595794746));
#32809=CARTESIAN_POINT('Ctrl Pts',(56.6628097724314,22.1040545770526,26.453597675058));
#32810=CARTESIAN_POINT('Ctrl Pts',(56.6223075820728,22.1606660465651,26.4580357706414));
#32811=CARTESIAN_POINT('Ctrl Pts',(56.5817813814332,22.217311076171,26.4624764971916));
#32812=CARTESIAN_POINT('Ctrl Pts',(56.5383231833967,22.2717775788078,26.4669172237419));
#32813=CARTESIAN_POINT('Ctrl Pts',(56.492208042573,22.3237608243866,26.4713579502922));
#32814=CARTESIAN_POINT('Ctrl Pts',(56.4460115334723,22.3758357922726,26.4758065123226));
#32815=CARTESIAN_POINT('Ctrl Pts',(56.3971490682769,22.4254184076707,26.480255074353));
#32816=CARTESIAN_POINT('Ctrl Pts',(56.3459319110476,22.4722414385296,26.4847036363833));
#32817=CARTESIAN_POINT('Ctrl Pts',(56.3184415326082,22.4973733065915,26.4870913646436));
#32818=CARTESIAN_POINT('Ctrl Pts',(56.2902733482307,22.5217108604893,26.4894790929038));
#32819=CARTESIAN_POINT('Ctrl Pts',(56.2614790088167,22.5452178722804,26.4918668211641));
#32820=CARTESIAN_POINT('Ctrl Pts',(56.2076670278864,22.5891486897944,26.4963291005642));
#32821=CARTESIAN_POINT('Ctrl Pts',(56.1514529776905,22.6303505042149,26.5007913799643));
#32822=CARTESIAN_POINT('Ctrl Pts',(56.0931444860463,22.6685510765711,26.5052536593645));
#32823=CARTESIAN_POINT('Ctrl Pts',(56.0349188706141,22.7066973529124,26.5097095963469));
#32824=CARTESIAN_POINT('Ctrl Pts',(55.974605124732,22.7418505863297,26.5141655333292));
#32825=CARTESIAN_POINT('Ctrl Pts',(55.9125436069833,22.7737789399624,26.5186214703116));
#32826=CARTESIAN_POINT('Ctrl Pts',(55.8505532127707,22.8056707031683,26.5230723007157));
#32827=CARTESIAN_POINT('Ctrl Pts',(55.7868194557606,22.8343447041128,26.5275231311199));
#32828=CARTESIAN_POINT('Ctrl Pts',(55.7217097632358,22.8596135566698,26.531973961524));
#32829=CARTESIAN_POINT('Ctrl Pts',(55.6566446468541,22.8848651093757,26.5364217447497));
#32830=CARTESIAN_POINT('Ctrl Pts',(55.5902059183537,22.9067159657897,26.5408695279754));
#32831=CARTESIAN_POINT('Ctrl Pts',(55.5227821248716,22.9250263407067,26.5453173112011));
#32832=CARTESIAN_POINT('Ctrl Pts',(55.4553656706266,22.9433347224968,26.5497646102752));
#32833=CARTESIAN_POINT('Ctrl Pts',(55.3869648314726,22.9581032488662,26.5542119093493));
#32834=CARTESIAN_POINT('Ctrl Pts',(55.3179831069597,22.9692420638886,26.5586592084234));
#32835=CARTESIAN_POINT('Ctrl Pts',(55.2670659071085,22.9774639121333,26.5619418752073));
#32836=CARTESIAN_POINT('Ctrl Pts',(55.2158325719834,22.9837092199195,26.5652245419912));
#32837=CARTESIAN_POINT('Ctrl Pts',(55.1644483516311,22.987959834138,26.5685072087751));
#32838=CARTESIAN_POINT('Ctrl Pts',(53.0052500783576,20.9994408866902,25.9772229232566));
#32839=CARTESIAN_POINT('Ctrl Pts',(53.0052168943837,21.1178314313542,25.969843828915));
#32840=CARTESIAN_POINT('Ctrl Pts',(53.0157237467158,21.2360116493196,25.9629670122793));
#32841=CARTESIAN_POINT('Ctrl Pts',(53.0553516448135,21.4566802688221,25.9499560771908));
#32842=CARTESIAN_POINT('Ctrl Pts',(53.0822955029543,21.5591258510858,25.9438400738149));
#32843=CARTESIAN_POINT('Ctrl Pts',(53.1364684850564,21.7139110708629,25.9340161240978));
#32844=CARTESIAN_POINT('Ctrl Pts',(53.1581014789727,21.7680023374757,25.9304683168702));
#32845=CARTESIAN_POINT('Ctrl Pts',(53.1879357837986,21.8340587940084,25.9259522809833));
#32846=CARTESIAN_POINT('Ctrl Pts',(53.1939427273713,21.8469875481996,25.9250594539539));
#32847=CARTESIAN_POINT('Ctrl Pts',(53.2037225485487,21.8674595027399,25.9236309183512));
#32848=CARTESIAN_POINT('Ctrl Pts',(53.2074056508731,21.8750452373608,25.9230983165377));
#32849=CARTESIAN_POINT('Ctrl Pts',(53.2144482759667,21.8893191886766,25.9220898341636));
#32850=CARTESIAN_POINT('Ctrl Pts',(53.2177975671835,21.8960123126986,25.921614316845));
#32851=CARTESIAN_POINT('Ctrl Pts',(53.2254481267374,21.9110883516037,25.9205371818387));
#32852=CARTESIAN_POINT('Ctrl Pts',(53.2297712575822,21.9194599120203,25.9199348046992));
#32853=CARTESIAN_POINT('Ctrl Pts',(53.2410333087816,21.9408945370596,25.9183813406902));
#32854=CARTESIAN_POINT('Ctrl Pts',(53.2480584153073,21.953911429301,25.9174272288736));
#32855=CARTESIAN_POINT('Ctrl Pts',(53.2958130772659,22.0400893611099,25.9110375353348));
#32856=CARTESIAN_POINT('Ctrl Pts',(53.3409644880603,22.110692046266,25.9054438100963));
#32857=CARTESIAN_POINT('Ctrl Pts',(53.4720711051744,22.2897958207562,25.8902834373139));
#32858=CARTESIAN_POINT('Ctrl Pts',(53.565104899898,22.3925557241909,25.8805199323808));
#32859=CARTESIAN_POINT('Ctrl Pts',(53.7002336413577,22.5137733837179,25.8680133646231));
#32860=CARTESIAN_POINT('Ctrl Pts',(53.7334004786974,22.5416317930085,25.8650600155022));
#32861=CARTESIAN_POINT('Ctrl Pts',(53.7804983565995,22.5786445834628,25.8610505370502));
#32862=CARTESIAN_POINT('Ctrl Pts',(53.7936747974107,22.5887361405098,25.8599479137013));
#32863=CARTESIAN_POINT('Ctrl Pts',(53.8137836131362,22.6037426216574,25.8582956442951));
#32864=CARTESIAN_POINT('Ctrl Pts',(53.8206236377335,22.6087793866882,25.8577388534942));
#32865=CARTESIAN_POINT('Ctrl Pts',(53.8318289221935,22.6169207103406,25.8568354870571));
#32866=CARTESIAN_POINT('Ctrl Pts',(53.8361748006287,22.6200515909781,25.856487250934));
#32867=CARTESIAN_POINT('Ctrl Pts',(53.8445488857416,22.6260334061561,25.8558203920828));
#32868=CARTESIAN_POINT('Ctrl Pts',(53.848575158784,22.6288869671294,25.855501597135));
#32869=CARTESIAN_POINT('Ctrl Pts',(53.8526311622533,22.6317390456855,25.8551823180915));
#32870=CARTESIAN_POINT('Ctrl Pts',(53.8526502916636,22.6317524964979,25.8551808123111));
#32871=CARTESIAN_POINT('Ctrl Pts',(53.8526886932853,22.631779497524,25.8551777895932));
#32872=CARTESIAN_POINT('Ctrl Pts',(53.8527079662335,22.6317930482481,25.8551762725984));
#32873=CARTESIAN_POINT('Ctrl Pts',(53.8527466579178,22.631820251175,25.8551732272186));
#32874=CARTESIAN_POINT('Ctrl Pts',(53.8527660765872,22.631833903323,25.8551716988395));
#32875=CARTESIAN_POINT('Ctrl Pts',(53.8528050628986,22.6318613113132,25.8551686304424));
#32876=CARTESIAN_POINT('Ctrl Pts',(53.8528246305032,22.6318750671212,25.855167090428));
#32877=CARTESIAN_POINT('Ctrl Pts',(53.8528639174295,22.6319026843368,25.8551639985463));
#32878=CARTESIAN_POINT('Ctrl Pts',(53.85288363709,22.6319165459744,25.855162446653));
#32879=CARTESIAN_POINT('Ctrl Pts',(53.8529232313168,22.631944377066,25.8551593307646));
#32880=CARTESIAN_POINT('Ctrl Pts',(53.852943105864,22.6319583464983,25.8551577667717));
#32881=CARTESIAN_POINT('Ctrl Pts',(53.8529830131672,22.6319863954753,25.8551546264264));
#32882=CARTESIAN_POINT('Ctrl Pts',(53.853003045852,22.6320004749616,25.8551530500802));
#32883=CARTESIAN_POINT('Ctrl Pts',(53.8530432727706,22.6320287463683,25.8551498847675));
#32884=CARTESIAN_POINT('Ctrl Pts',(53.8530634667852,22.6320429381259,25.8551482958191));
#32885=CARTESIAN_POINT('Ctrl Pts',(53.8564102213836,22.6343948457042,25.8548849670434));
#32886=CARTESIAN_POINT('Ctrl Pts',(53.8597438809084,22.6367223579057,25.8546239353481));
#32887=CARTESIAN_POINT('Ctrl Pts',(53.8673711701042,22.6420130054644,25.8540295736486));
#32888=CARTESIAN_POINT('Ctrl Pts',(53.8716693145569,22.6449694958284,25.8536966943792));
#32889=CARTESIAN_POINT('Ctrl Pts',(53.8842961897082,22.6535821503281,25.8527246308436));
#32890=CARTESIAN_POINT('Ctrl Pts',(53.8926563477196,22.6591922631115,25.8520884545075));
#32891=CARTESIAN_POINT('Ctrl Pts',(53.9556345587976,22.7007659572642,25.8473485004364));
#32892=CARTESIAN_POINT('Ctrl Pts',(54.0119551749834,22.734091500109,25.843402885128));
#32893=CARTESIAN_POINT('Ctrl Pts',(54.2231724667732,22.8454320255768,25.8292679487586));
#32894=CARTESIAN_POINT('Ctrl Pts',(54.3864080176575,22.9059352033324,25.819517022989));
#32895=CARTESIAN_POINT('Ctrl Pts',(54.6055034078439,22.9560265693039,25.8059888965488));
#32896=CARTESIAN_POINT('Ctrl Pts',(54.6560113960928,22.965537751984,25.8028475902073));
#32897=CARTESIAN_POINT('Ctrl Pts',(54.7203812286329,22.9751021933107,25.7987898157386));
#32898=CARTESIAN_POINT('Ctrl Pts',(54.7339554159447,22.9769763771404,25.7979311357743));
#32899=CARTESIAN_POINT('Ctrl Pts',(54.755789988905,22.9797621261863,25.7965446833748));
#32900=CARTESIAN_POINT('Ctrl Pts',(54.7640387927685,22.9807622045808,25.7960197047885));
#32901=CARTESIAN_POINT('Ctrl Pts',(54.7797491121106,22.9825673831855,25.7950174766231));
#32902=CARTESIAN_POINT('Ctrl Pts',(54.7872094100477,22.9833819714796,25.7945405346773));
#32903=CARTESIAN_POINT('Ctrl Pts',(54.8042491035216,22.9851452875238,25.7934487733241));
#32904=CARTESIAN_POINT('Ctrl Pts',(54.8138310678165,22.9860668038534,25.7928331102182));
#32905=CARTESIAN_POINT('Ctrl Pts',(54.8388317759815,22.9882886586392,25.7912220810086));
#32906=CARTESIAN_POINT('Ctrl Pts',(54.8542594048445,22.9894789878342,25.7902232993738));
#32907=CARTESIAN_POINT('Ctrl Pts',(54.9679368844923,22.9969205199647,25.7828282501797));
#32908=CARTESIAN_POINT('Ctrl Pts',(55.0664554171434,22.9960660352381,25.7762135204845));
#32909=CARTESIAN_POINT('Ctrl Pts',(55.1644486115703,22.9879598126352,25.7694502499567));
#32910=CARTESIAN_POINT('',(53.0052505021471,20.9985846147351,25.8209548813952));
#32911=CARTESIAN_POINT('Ctrl Pts',(55.1644483516311,22.987959834138,25.6104387285779));
#32912=CARTESIAN_POINT('Ctrl Pts',(55.1579505623676,22.9884973453669,25.6108573370408));
#32913=CARTESIAN_POINT('Ctrl Pts',(55.1514513148831,22.9890029011531,25.6112759455036));
#32914=CARTESIAN_POINT('Ctrl Pts',(55.1449509479891,22.9894765103356,25.6116945539665));
#32915=CARTESIAN_POINT('Ctrl Pts',(55.0757777214915,22.9945163912813,25.6161491483744));
#32916=CARTESIAN_POINT('Ctrl Pts',(55.0062047534237,22.9959542399979,25.6206037427823));
#32917=CARTESIAN_POINT('Ctrl Pts',(54.9366391221284,22.9937434543229,25.6250583371902));
#32918=CARTESIAN_POINT('Ctrl Pts',(54.8671778558954,22.9915359853544,25.6295062486426));
#32919=CARTESIAN_POINT('Ctrl Pts',(54.7977243897905,22.9856907617156,25.6339541600949));
#32920=CARTESIAN_POINT('Ctrl Pts',(54.7286893658636,22.9762130710793,25.6384020715472));
#32921=CARTESIAN_POINT('Ctrl Pts',(54.6597355119215,22.9667465241198,25.6428447532353));
#32922=CARTESIAN_POINT('Ctrl Pts',(54.5911996055224,22.9536560591925,25.6472874349233));
#32923=CARTESIAN_POINT('Ctrl Pts',(54.5234889208121,22.936998903952,25.6517301166113));
#32924=CARTESIAN_POINT('Ctrl Pts',(54.4558208106123,22.9203522222465,25.6561700048702));
#32925=CARTESIAN_POINT('Ctrl Pts',(54.3889773669066,22.9001434157983,25.6606098931291));
#32926=CARTESIAN_POINT('Ctrl Pts',(54.3233558891505,22.8764808311711,25.665049781388));
#32927=CARTESIAN_POINT('Ctrl Pts',(54.2577533901692,22.8528250901396,25.6694883855606));
#32928=CARTESIAN_POINT('Ctrl Pts',(54.1933726157074,22.8257177198506,25.6739269897332));
#32929=CARTESIAN_POINT('Ctrl Pts',(54.1305942010773,22.7953164398789,25.6783655939059));
#32930=CARTESIAN_POINT('Ctrl Pts',(54.0678126268779,22.7649136298439,25.6828044214686));
#32931=CARTESIAN_POINT('Ctrl Pts',(54.0066340120517,22.7312167964684,25.6872432490314));
#32932=CARTESIAN_POINT('Ctrl Pts',(53.9474159375527,22.6944303921914,25.6916820765941));
#32933=CARTESIAN_POINT('Ctrl Pts',(53.8881352163903,22.6576050716627,25.6961255999822));
#32934=CARTESIAN_POINT('Ctrl Pts',(53.8308195917504,22.6176839154238,25.7005691233703));
#32935=CARTESIAN_POINT('Ctrl Pts',(53.7757982674691,22.5749151344019,25.7050126467584));
#32936=CARTESIAN_POINT('Ctrl Pts',(53.7207447675428,22.5321213428386,25.7094587686524));
#32937=CARTESIAN_POINT('Ctrl Pts',(53.667988608646,22.4864769323068,25.7139048905463));
#32938=CARTESIAN_POINT('Ctrl Pts',(53.6178243107435,22.4382690730626,25.7183510124402));
#32939=CARTESIAN_POINT('Ctrl Pts',(53.5675728265466,22.3899774278434,25.72280486176));
#32940=CARTESIAN_POINT('Ctrl Pts',(53.5199225298912,22.339113797589,25.7272587110798));
#32941=CARTESIAN_POINT('Ctrl Pts',(53.4751290838272,22.2860000977879,25.7317125603996));
#32942=CARTESIAN_POINT('Ctrl Pts',(53.451610930245,22.2581135148387,25.7340509898248));
#32943=CARTESIAN_POINT('Ctrl Pts',(53.4288796015844,22.2296071906273,25.7363894192501));
#32944=CARTESIAN_POINT('Ctrl Pts',(53.4069672511891,22.200530809149,25.7387278486753));
#32945=CARTESIAN_POINT('Ctrl Pts',(53.3650931932104,22.1449664328104,25.7431965399643));
#32946=CARTESIAN_POINT('Ctrl Pts',(53.3260457686232,22.087097308453,25.7476652312533));
#32947=CARTESIAN_POINT('Ctrl Pts',(53.2900869513704,22.0272414169154,25.7521339225422));
#32948=CARTESIAN_POINT('Ctrl Pts',(53.2541821620369,21.9674754585159,25.7565958996478));
#32949=CARTESIAN_POINT('Ctrl Pts',(53.2213570194895,21.9057290678154,25.7610578767534));
#32950=CARTESIAN_POINT('Ctrl Pts',(53.1918320278417,21.8423515578194,25.765519853859));
#32951=CARTESIAN_POINT('Ctrl Pts',(53.1612641374524,21.7767353909527,25.770139439487));
#32952=CARTESIAN_POINT('Ctrl Pts',(53.1342342429006,21.7093711268831,25.7747590251151));
#32953=CARTESIAN_POINT('Ctrl Pts',(53.1109365293977,21.6406768034945,25.7793786107431));
#32954=CARTESIAN_POINT('Ctrl Pts',(53.0884794010214,21.5744609819775,25.7838315210032));
#32955=CARTESIAN_POINT('Ctrl Pts',(53.0694899032742,21.5070099421813,25.7882844312633));
#32956=CARTESIAN_POINT('Ctrl Pts',(53.0540931529504,21.438718708406,25.7927373415233));
#32957=CARTESIAN_POINT('Ctrl Pts',(53.0387034612457,21.3704587826533,25.7971882103528));
#32958=CARTESIAN_POINT('Ctrl Pts',(53.0269033496652,21.3013599010742,25.8016390791823));
#32959=CARTESIAN_POINT('Ctrl Pts',(53.0187674350936,21.2318298648886,25.8060899480117));
#32960=CARTESIAN_POINT('Ctrl Pts',(53.0106315145687,21.1622997778266,25.810540820098));
#32961=CARTESIAN_POINT('Ctrl Pts',(53.0061598545227,21.0923390168737,25.8149916921842));
#32962=CARTESIAN_POINT('Ctrl Pts',(53.0053753430082,21.02236157911,25.8194425642705));
#32963=CARTESIAN_POINT('Ctrl Pts',(53.0052864892454,21.014435935519,25.8199466699787));
#32964=CARTESIAN_POINT('Ctrl Pts',(53.0052448785904,21.0065100799959,25.820450775687));
#32965=CARTESIAN_POINT('Ctrl Pts',(53.0052505021471,20.9985846147351,25.8209548813952));
#32966=CARTESIAN_POINT('Ctrl Pts',(53.0073840846254,20.9985711856803,25.8209558328711));
#32967=CARTESIAN_POINT('Ctrl Pts',(53.005850056014,20.7640139712392,25.8358909363755));
#32968=CARTESIAN_POINT('Ctrl Pts',(53.1526219523583,19.8662942493302,25.8931704714496));
#32969=CARTESIAN_POINT('Ctrl Pts',(54.4827630389435,18.6996030104917,25.9927944380933));
#32970=CARTESIAN_POINT('Ctrl Pts',(56.6523991680059,19.3180745080547,26.1198277328024));
#32971=CARTESIAN_POINT('Ctrl Pts',(57.3092165337547,21.4764259740402,26.2468610275113));
#32972=CARTESIAN_POINT('Ctrl Pts',(56.1973412839694,22.7902337162283,26.3437709099491));
#32973=CARTESIAN_POINT('Ctrl Pts',(55.355531775765,22.972868043151,26.3983363608173));
#32974=CARTESIAN_POINT('Ctrl Pts',(55.164372889159,22.9868942741083,26.4105573801159));
#32975=CARTESIAN_POINT('Origin',(55.,21.,7.5));
#32976=CARTESIAN_POINT('',(52.5495004857877,21.0015429988506,7.95782749621206));
#32977=CARTESIAN_POINT('',(56.0772665381941,23.205491718641,7.70002485738492));
#32978=CARTESIAN_POINT('Ctrl Pts',(52.5465050492984,21.0015448849783,7.95782749621206));
#32979=CARTESIAN_POINT('Ctrl Pts',(52.5459443844546,21.0835112770769,7.95355359535896));
#32980=CARTESIAN_POINT('Ctrl Pts',(52.5868459923412,21.9769760028613,7.9069352629362));
#32981=CARTESIAN_POINT('Ctrl Pts',(53.6445503233722,23.5238918290192,7.82100104999381));
#32982=CARTESIAN_POINT('Ctrl Pts',(55.3982288713416,23.5326747575202,7.73934073790454));
#32983=CARTESIAN_POINT('Ctrl Pts',(56.0772665381941,23.205491718641,7.70002485738492));
#32984=CARTESIAN_POINT('',(53.9249115396487,23.2020751695661,7.7));
#32985=CARTESIAN_POINT('Origin',(55.,21.,7.7));
#32986=CARTESIAN_POINT('',(52.5493075430995,21.0024481883259,7.84217250378794));
#32987=CARTESIAN_POINT('Ctrl Pts',(53.9249115396487,23.2020751695661,7.7));
#32988=CARTESIAN_POINT('Ctrl Pts',(53.1925621422827,22.8445304331579,7.74234443156966));
#32989=CARTESIAN_POINT('Ctrl Pts',(52.5954013728997,22.0066433600949,7.78973526616564));
#32990=CARTESIAN_POINT('Ctrl Pts',(52.5465178413277,21.0991960387036,7.83712610076162));
#32991=CARTESIAN_POINT('Ctrl Pts',(52.5472668131576,21.0024502269706,7.84217250378794));
#32992=CARTESIAN_POINT('',(52.5495002427347,21.0010907074207,8.64217250373997));
#32993=CARTESIAN_POINT('Ctrl Pts',(52.5495012227464,21.0024479948441,7.84217250378794));
#32994=CARTESIAN_POINT('Ctrl Pts',(52.549422118682,20.9232630187398,7.84630671022257));
#32995=CARTESIAN_POINT('Ctrl Pts',(52.5531853006392,20.8439028055671,7.85044091665719));
#32996=CARTESIAN_POINT('Ctrl Pts',(52.5608151121287,20.7647823714506,7.85457512309182));
#32997=CARTESIAN_POINT('Ctrl Pts',(52.5684657252199,20.6854462266639,7.85872060085541));
#32998=CARTESIAN_POINT('Ctrl Pts',(52.5800041470203,20.6063516605387,7.862866078619));
#32999=CARTESIAN_POINT('Ctrl Pts',(52.5954022533773,20.5279195757744,7.86701155638259));
#33000=CARTESIAN_POINT('Ctrl Pts',(52.6107230540881,20.4498812565067,7.87113622192226));
#33001=CARTESIAN_POINT('Ctrl Pts',(52.6298648063395,20.3724992676908,7.87526088746194));
#33002=CARTESIAN_POINT('Ctrl Pts',(52.6527479093513,20.2961833527507,7.87938555300161));
#33003=CARTESIAN_POINT('Ctrl Pts',(52.6756198352345,20.2199047139087,7.8835082038706));
#33004=CARTESIAN_POINT('Ctrl Pts',(52.702229348838,20.144691581996,7.88763085473958));
#33005=CARTESIAN_POINT('Ctrl Pts',(52.7324463126037,20.0709410541977,7.89175350560856));
#33006=CARTESIAN_POINT('Ctrl Pts',(52.7626586529099,19.9972018108742,7.89587552567596));
#33007=CARTESIAN_POINT('Ctrl Pts',(52.796477162552,19.9249251776549,7.89999754574336));
#33008=CARTESIAN_POINT('Ctrl Pts',(52.8337232570441,19.8544890559543,7.90411956581076));
#33009=CARTESIAN_POINT('Ctrl Pts',(52.8713328823099,19.7833654608913,7.90828181777803));
#33010=CARTESIAN_POINT('Ctrl Pts',(52.9124371517035,19.7141189594769,7.91244406974529));
#33011=CARTESIAN_POINT('Ctrl Pts',(52.9568052803081,19.6471121305064,7.91660632171256));
#33012=CARTESIAN_POINT('Ctrl Pts',(53.0008010424648,19.5806676668117,7.92073364133022));
#33013=CARTESIAN_POINT('Ctrl Pts',(53.0480057411504,19.5164257812278,7.92486096094788));
#33014=CARTESIAN_POINT('Ctrl Pts',(53.0981527312477,19.4547080481865,7.92898828056554));
#33015=CARTESIAN_POINT('Ctrl Pts',(53.148936364137,19.3922067755989,7.93316799870761));
#33016=CARTESIAN_POINT('Ctrl Pts',(53.2027371757151,19.3322945787699,7.93734771684968));
#33017=CARTESIAN_POINT('Ctrl Pts',(53.2592401587572,19.2752665640406,7.94152743499175));
#33018=CARTESIAN_POINT('Ctrl Pts',(53.3157431417993,19.2182385493112,7.94570715313382));
#33019=CARTESIAN_POINT('Ctrl Pts',(53.3749478683294,19.1640950033771,7.94988687127589));
#33020=CARTESIAN_POINT('Ctrl Pts',(53.4365070735543,19.1130871459036,7.95406658941796));
#33021=CARTESIAN_POINT('Ctrl Pts',(53.4988934139118,19.0613939256025,7.95830246799464));
#33022=CARTESIAN_POINT('Ctrl Pts',(53.5639619311142,19.0127020952609,7.96253834657133));
#33023=CARTESIAN_POINT('Ctrl Pts',(53.6313921892293,18.9673015692687,7.96677422514801));
#33024=CARTESIAN_POINT('Ctrl Pts',(53.6987256512506,18.9219662157035,7.97100402312361));
#33025=CARTESIAN_POINT('Ctrl Pts',(53.7684137389447,18.8799130391827,7.97523382109922));
#33026=CARTESIAN_POINT('Ctrl Pts',(53.8401027657429,18.8413919633331,7.97946361907482));
#33027=CARTESIAN_POINT('Ctrl Pts',(53.911877321831,18.8028249295399,7.98369846345199));
#33028=CARTESIAN_POINT('Ctrl Pts',(53.985657222653,18.7677987134624,7.98793330782917));
#33029=CARTESIAN_POINT('Ctrl Pts',(54.0610580981629,18.7365207412095,7.99216815220634));
#33030=CARTESIAN_POINT('Ctrl Pts',(54.1362325494697,18.7053366947883,7.99639027960567));
#33031=CARTESIAN_POINT('Ctrl Pts',(54.2130178316279,18.6778786080508,8.000612407005));
#33032=CARTESIAN_POINT('Ctrl Pts',(54.2910097948158,18.6543054037337,8.00483453440433));
#33033=CARTESIAN_POINT('Ctrl Pts',(54.3689753494903,18.630740181435,8.00905523216779));
#33034=CARTESIAN_POINT('Ctrl Pts',(54.4481463301967,18.6110573631241,8.01327592993125));
#33035=CARTESIAN_POINT('Ctrl Pts',(54.5281021875988,18.5953664094813,8.01749662769471));
#33036=CARTESIAN_POINT('Ctrl Pts',(54.6080553125754,18.5796759920639,8.02171718121931));
#33037=CARTESIAN_POINT('Ctrl Pts',(54.6887928056727,18.5679772563439,8.02593773474391));
#33038=CARTESIAN_POINT('Ctrl Pts',(54.7698840529587,18.5603285260271,8.03015828826851));
#33039=CARTESIAN_POINT('Ctrl Pts',(54.8514475556846,18.5526352513899,8.03440342125671));
#33040=CARTESIAN_POINT('Ctrl Pts',(54.9333684758368,18.5490393671079,8.03864855424491));
#33041=CARTESIAN_POINT('Ctrl Pts',(55.0152053631808,18.5495471751265,8.04289368723312));
#33042=CARTESIAN_POINT('Ctrl Pts',(55.0966835794971,18.550052757547,8.04712021484346));
#33043=CARTESIAN_POINT('Ctrl Pts',(55.1780780341992,18.554626057633,8.0513467424538));
#33044=CARTESIAN_POINT('Ctrl Pts',(55.2589568338114,18.563221058811,8.05557327006414));
#33045=CARTESIAN_POINT('Ctrl Pts',(55.3403696819735,18.5718728134019,8.05982770574128));
#33046=CARTESIAN_POINT('Ctrl Pts',(55.4212595698563,18.5845994999149,8.06408214141841));
#33047=CARTESIAN_POINT('Ctrl Pts',(55.5011968970607,18.6013020364421,8.06833657709554));
#33048=CARTESIAN_POINT('Ctrl Pts',(55.581134224265,18.6180045729694,8.07259101277268));
#33049=CARTESIAN_POINT('Ctrl Pts',(55.660118549111,18.6386827804699,8.07684544844981));
#33050=CARTESIAN_POINT('Ctrl Pts',(55.7377380125337,18.66318745406,8.08109988412694));
#33051=CARTESIAN_POINT('Ctrl Pts',(55.8150631561192,18.687599210085,8.08533818770575));
#33052=CARTESIAN_POINT('Ctrl Pts',(55.8913147918291,18.7158971420639,8.08957649128455));
#33053=CARTESIAN_POINT('Ctrl Pts',(55.9660753525726,18.7479678814121,8.09381479486336));
#33054=CARTESIAN_POINT('Ctrl Pts',(56.0407314205827,18.7799937955317,8.09804717457105));
#33055=CARTESIAN_POINT('Ctrl Pts',(56.1139001310483,18.8157818615719,8.10227955427875));
#33056=CARTESIAN_POINT('Ctrl Pts',(56.1851796564499,18.8551691367529,8.10651193398644));
#33057=CARTESIAN_POINT('Ctrl Pts',(56.2564901504259,18.8945735243902,8.11074615252184));
#33058=CARTESIAN_POINT('Ctrl Pts',(56.3259093825185,18.9375800833776,8.11498037105723));
#33059=CARTESIAN_POINT('Ctrl Pts',(56.393055648912,18.9839776268518,8.11921458959263));
#33060=CARTESIAN_POINT('Ctrl Pts',(56.4600568949614,19.0302749624053,8.12343966319916));
#33061=CARTESIAN_POINT('Ctrl Pts',(56.5247945892955,19.0799484052375,8.12766473680569));
#33062=CARTESIAN_POINT('Ctrl Pts',(56.5869162490708,19.1327434379724,8.13188981041223));
#33063=CARTESIAN_POINT('Ctrl Pts',(56.6490188187896,19.1855222467338,8.13611358564884));
#33064=CARTESIAN_POINT('Ctrl Pts',(56.7085065979807,19.2414204405044,8.14033736088546));
#33065=CARTESIAN_POINT('Ctrl Pts',(56.7650598860866,19.3001429917408,8.14456113612207));
#33066=CARTESIAN_POINT('Ctrl Pts',(56.8216129508396,19.358865311057,8.14878489467721));
#33067=CARTESIAN_POINT('Ctrl Pts',(56.875231227228,19.4204116312256,8.15300865323234));
#33068=CARTESIAN_POINT('Ctrl Pts',(56.925632619831,19.4844508376688,8.15723241178748));
#33069=CARTESIAN_POINT('Ctrl Pts',(56.9762484696386,19.5487625300193,8.16147414237485));
#33070=CARTESIAN_POINT('Ctrl Pts',(57.0236196989971,19.6155880078858,8.16571587296222));
#33071=CARTESIAN_POINT('Ctrl Pts',(57.0675032574135,19.6845607081342,8.16995760354959));
#33072=CARTESIAN_POINT('Ctrl Pts',(57.1112656105149,19.7533429074715,8.17418761858083));
#33073=CARTESIAN_POINT('Ctrl Pts',(57.1515593395479,19.8242600576247,8.17841763361206));
#33074=CARTESIAN_POINT('Ctrl Pts',(57.188189379129,19.8969236241008,8.1826476486433));
#33075=CARTESIAN_POINT('Ctrl Pts',(57.2249715959299,19.9698890668417,8.18689523700874));
#33076=CARTESIAN_POINT('Ctrl Pts',(57.2580594326714,20.0446150352548,8.19114282537418));
#33077=CARTESIAN_POINT('Ctrl Pts',(57.2873047354194,20.1206893055762,8.19539041373961));
#33078=CARTESIAN_POINT('Ctrl Pts',(57.3165500381673,20.1967635758976,8.19963800210505));
#33079=CARTESIAN_POINT('Ctrl Pts',(57.3419527204521,20.2741856860223,8.20388559047049));
#33080=CARTESIAN_POINT('Ctrl Pts',(57.3634158799239,20.3525313686954,8.20813317883593));
#33081=CARTESIAN_POINT('Ctrl Pts',(57.384771145699,20.4304832134837,8.21235941489247));
#33082=CARTESIAN_POINT('Ctrl Pts',(57.4023066169024,20.5096422156924,8.216585650949));
#33083=CARTESIAN_POINT('Ctrl Pts',(57.4158893440379,20.5895990651033,8.22081188700554));
#33084=CARTESIAN_POINT('Ctrl Pts',(57.4294523479186,20.6694398104875,8.22503198621417));
#33085=CARTESIAN_POINT('Ctrl Pts',(57.4390739289214,20.7500756467217,8.22925208542279));
#33086=CARTESIAN_POINT('Ctrl Pts',(57.444671222262,20.8310832600236,8.23347218463142));
#33087=CARTESIAN_POINT('Ctrl Pts',(57.450291279378,20.9124203252604,8.23770944666948));
#33088=CARTESIAN_POINT('Ctrl Pts',(57.451854115726,20.9941317396832,8.24194670870754));
#33089=CARTESIAN_POINT('Ctrl Pts',(57.449328003338,21.0757798262361,8.24618397074561));
#33090=CARTESIAN_POINT('Ctrl Pts',(57.4468167335279,21.1569481763784,8.25039633607185));
#33091=CARTESIAN_POINT('Ctrl Pts',(57.4402644461553,21.2380534699362,8.2546087013981));
#33092=CARTESIAN_POINT('Ctrl Pts',(57.4296921086673,21.3186636268545,8.25882106672435));
#33093=CARTESIAN_POINT('Ctrl Pts',(57.4191233632417,21.3992463956271,8.26303200085533));
#33094=CARTESIAN_POINT('Ctrl Pts',(57.4045373404319,21.4793338999595,8.26724293498631));
#33095=CARTESIAN_POINT('Ctrl Pts',(57.3860068412155,21.5584994213718,8.27145386911729));
#33096=CARTESIAN_POINT('Ctrl Pts',(57.3674769238625,21.6376624569624,8.27566467102364));
#33097=CARTESIAN_POINT('Ctrl Pts',(57.3450028836156,21.7159031135083,8.27987547292999));
#33098=CARTESIAN_POINT('Ctrl Pts',(57.3187082729761,21.7928065305181,8.28408627483635));
#33099=CARTESIAN_POINT('Ctrl Pts',(57.2921271536252,21.8705478948629,8.28834295806206));
#33100=CARTESIAN_POINT('Ctrl Pts',(57.2616418377762,21.946922234669,8.29259964128777));
#33101=CARTESIAN_POINT('Ctrl Pts',(57.2274305212793,22.021520201892,8.29685632451349));
#33102=CARTESIAN_POINT('Ctrl Pts',(57.1935388937509,22.0954210855287,8.30107323099837));
#33103=CARTESIAN_POINT('Ctrl Pts',(57.1559908843481,22.16757826781,8.30529013748324));
#33104=CARTESIAN_POINT('Ctrl Pts',(57.1150058694171,22.2376188518002,8.30950704396812));
#33105=CARTESIAN_POINT('Ctrl Pts',(57.0734409565243,22.3086504416974,8.31378361556425));
#33106=CARTESIAN_POINT('Ctrl Pts',(57.0283412900334,22.3775046540551,8.31806018716038));
#33107=CARTESIAN_POINT('Ctrl Pts',(56.979979776086,22.4438248980712,8.32233675875652));
#33108=CARTESIAN_POINT('Ctrl Pts',(56.9316182621387,22.5101451420873,8.32661333035265));
#33109=CARTESIAN_POINT('Ctrl Pts',(56.8799952623039,22.573931076411,8.33088990194878));
#33110=CARTESIAN_POINT('Ctrl Pts',(56.8254230573828,22.6348641875016,8.33516647354491));
#33111=CARTESIAN_POINT('Ctrl Pts',(56.7714178366747,22.6951642270115,8.33939861320753));
#33112=CARTESIAN_POINT('Ctrl Pts',(56.7143205495057,22.7528981716161,8.34363075287014));
#33113=CARTESIAN_POINT('Ctrl Pts',(56.6544045728723,22.8077322144774,8.34786289253276));
#33114=CARTESIAN_POINT('Ctrl Pts',(56.5945744576463,22.8624876784961,8.35208896741119));
#33115=CARTESIAN_POINT('Ctrl Pts',(56.5319340152705,22.9143511832187,8.35631504228962));
#33116=CARTESIAN_POINT('Ctrl Pts',(56.4667954483278,22.9630235257798,8.36054111716805));
#33117=CARTESIAN_POINT('Ctrl Pts',(56.4015073358401,23.011807610621,8.36477689429662));
#33118=CARTESIAN_POINT('Ctrl Pts',(56.3337099361628,23.0573855189617,8.3690126714252));
#33119=CARTESIAN_POINT('Ctrl Pts',(56.2637532666214,23.0994946847048,8.37324844855378));
#33120=CARTESIAN_POINT('Ctrl Pts',(56.1940823883991,23.141431823476,8.37746692142328));
#33121=CARTESIAN_POINT('Ctrl Pts',(56.1222702433406,23.1799282560506,8.38168539429279));
#33122=CARTESIAN_POINT('Ctrl Pts',(56.048692467878,23.2147673371747,8.38590386716229));
#33123=CARTESIAN_POINT('Ctrl Pts',(55.9751390238809,23.2495948973484,8.39012094502323));
#33124=CARTESIAN_POINT('Ctrl Pts',(55.8998215286527,23.2807673092017,8.39433802288417));
#33125=CARTESIAN_POINT('Ctrl Pts',(55.8231391481475,23.3081144236773,8.3985551007451));
#33126=CARTESIAN_POINT('Ctrl Pts',(55.7464586626518,23.3354608623386,8.40277207439171));
#33127=CARTESIAN_POINT('Ctrl Pts',(55.6684137970017,23.3589820365267,8.40698904803832));
#33128=CARTESIAN_POINT('Ctrl Pts',(55.5894212164372,23.3785568901361,8.41120602168493));
#33129=CARTESIAN_POINT('Ctrl Pts',(55.5098197460523,23.3982826304364,8.41545550056567));
#33130=CARTESIAN_POINT('Ctrl Pts',(55.4292563476232,23.4140008172801,8.41970497944642));
#33131=CARTESIAN_POINT('Ctrl Pts',(55.3481684974395,23.4256399047243,8.42395445832717));
#33132=CARTESIAN_POINT('Ctrl Pts',(55.2675842978785,23.4372066997889,8.42817754296168));
#33133=CARTESIAN_POINT('Ctrl Pts',(55.186482615642,23.4447449399005,8.43240062759619));
#33134=CARTESIAN_POINT('Ctrl Pts',(55.105296749555,23.4482366806608,8.43662371223071));
#33135=CARTESIAN_POINT('Ctrl Pts',(55.0233497669174,23.4517611564502,8.44088638823457));
#33136=CARTESIAN_POINT('Ctrl Pts',(54.9413174975649,23.4511628672211,8.44514906423844));
#33137=CARTESIAN_POINT('Ctrl Pts',(54.8596423428699,23.4464770544775,8.4494117402423));
#33138=CARTESIAN_POINT('Ctrl Pts',(54.7779671881749,23.4417912417339,8.45367441624616));
#33139=CARTESIAN_POINT('Ctrl Pts',(54.6966496184479,23.4330180203266,8.45793709225003));
#33140=CARTESIAN_POINT('Ctrl Pts',(54.6161216682733,23.4202453752524,8.46219976825389));
#33141=CARTESIAN_POINT('Ctrl Pts',(54.536172916678,23.4075645976338,8.4664317848919));
#33142=CARTESIAN_POINT('Ctrl Pts',(54.4567039432331,23.3908944354196,8.47066380152991));
#33143=CARTESIAN_POINT('Ctrl Pts',(54.3781434386056,23.3702836680555,8.47489581816792));
#33144=CARTESIAN_POINT('Ctrl Pts',(54.2996952454205,23.3497023661974,8.4791217846425));
#33145=CARTESIAN_POINT('Ctrl Pts',(54.2221533873162,23.3251917649516,8.48334775111707));
#33146=CARTESIAN_POINT('Ctrl Pts',(54.1459385201734,23.2968520280324,8.48757371759165));
#33147=CARTESIAN_POINT('Ctrl Pts',(54.0695461971795,23.2684463059278,8.49180952364878));
#33148=CARTESIAN_POINT('Ctrl Pts',(53.9944875157402,23.236193678747,8.49604532970592));
#33149=CARTESIAN_POINT('Ctrl Pts',(53.9211728758895,23.2002459604061,8.50028113576305));
#33150=CARTESIAN_POINT('Ctrl Pts',(53.8481594848187,23.1644459507127,8.50449953695521));
#33151=CARTESIAN_POINT('Ctrl Pts',(53.7768762549463,23.1249813533276,8.50871793814738));
#33152=CARTESIAN_POINT('Ctrl Pts',(53.7077088482683,23.082050390638,8.51293633933954));
#33153=CARTESIAN_POINT('Ctrl Pts',(53.6385640843698,23.0391334819136,8.51715335958751));
#33154=CARTESIAN_POINT('Ctrl Pts',(53.571534162698,22.9927527062658,8.52137037983549));
#33155=CARTESIAN_POINT('Ctrl Pts',(53.5069784244422,22.9431512614614,8.52558740008347));
#33156=CARTESIAN_POINT('Ctrl Pts',(53.4424240640287,22.8935508753231,8.52980433032567));
#33157=CARTESIAN_POINT('Ctrl Pts',(53.38034414985,22.8407302407367,8.53402126056788));
#33158=CARTESIAN_POINT('Ctrl Pts',(53.3210662513842,22.7849738703295,8.53823819081009));
#33159=CARTESIAN_POINT('Ctrl Pts',(53.2613294942306,22.7287859006985,8.54248776348949));
#33160=CARTESIAN_POINT('Ctrl Pts',(53.204438681225,22.6696168635082,8.54673733616889));
#33161=CARTESIAN_POINT('Ctrl Pts',(53.1506910796216,22.6077956235196,8.55098690884829));
#33162=CARTESIAN_POINT('Ctrl Pts',(53.097278590771,22.5463598348871,8.55520998572217));
#33163=CARTESIAN_POINT('Ctrl Pts',(53.0469704719098,22.482305228034,8.55943306259605));
#33164=CARTESIAN_POINT('Ctrl Pts',(53.0000166551467,22.4159861829514,8.56365613946993));
#33165=CARTESIAN_POINT('Ctrl Pts',(52.9526209523248,22.3490430041248,8.56791896005209));
#33166=CARTESIAN_POINT('Ctrl Pts',(52.9086432780434,22.2797929500265,8.57218178063425));
#33167=CARTESIAN_POINT('Ctrl Pts',(52.8682938210179,22.2086269136873,8.57644460121641));
#33168=CARTESIAN_POINT('Ctrl Pts',(52.8279443639923,22.1374608773482,8.58070742179856));
#33169=CARTESIAN_POINT('Ctrl Pts',(52.7912232825414,22.0643793163929,8.58497024238072));
#33170=CARTESIAN_POINT('Ctrl Pts',(52.7582908137182,21.9897929956006,8.58923306296287));
#33171=CARTESIAN_POINT('Ctrl Pts',(52.7223976386163,21.9085011894265,8.59387912112526));
#33172=CARTESIAN_POINT('Ctrl Pts',(52.690888228178,21.8251600641242,8.59852517928764));
#33173=CARTESIAN_POINT('Ctrl Pts',(52.6639779262701,21.7402372059325,8.60317123745003));
#33174=CARTESIAN_POINT('Ctrl Pts',(52.6371426068781,21.6555509756903,8.60780434989627));
#33175=CARTESIAN_POINT('Ctrl Pts',(52.6148809649752,21.5692920834761,8.61243746234251));
#33176=CARTESIAN_POINT('Ctrl Pts',(52.5973604478986,21.481947541417,8.61707057478874));
#33177=CARTESIAN_POINT('Ctrl Pts',(52.5799228403308,21.3950163258056,8.62168176270639));
#33178=CARTESIAN_POINT('Ctrl Pts',(52.5671817197313,21.3070099981626,8.62629295062405));
#33179=CARTESIAN_POINT('Ctrl Pts',(52.5592542932496,21.2184276653249,8.6309041385417));
#33180=CARTESIAN_POINT('Ctrl Pts',(52.5527968728571,21.1462714159045,8.63466026027446));
#33181=CARTESIAN_POINT('Ctrl Pts',(52.5495325756989,21.0737333974149,8.63841638200722));
#33182=CARTESIAN_POINT('Ctrl Pts',(52.5495002427347,21.0010907074207,8.64217250373998));
#33183=CARTESIAN_POINT('',(52.5495009513656,20.9978406848801,9.44217250382341));
#33184=CARTESIAN_POINT('Ctrl Pts',(52.5495002427343,21.0010907064931,8.64217250378794));
#33185=CARTESIAN_POINT('Ctrl Pts',(52.5494633039605,20.9181000424275,8.64646368624462));
#33186=CARTESIAN_POINT('Ctrl Pts',(52.5536466572638,20.8351255123515,8.6507548687013));
#33187=CARTESIAN_POINT('Ctrl Pts',(52.562019055815,20.752615348514,8.65504605115798));
#33188=CARTESIAN_POINT('Ctrl Pts',(52.5703955399197,20.6700649214614,8.65933932762095));
#33189=CARTESIAN_POINT('Ctrl Pts',(52.5829650897535,20.587979750338,8.66363260408392));
#33190=CARTESIAN_POINT('Ctrl Pts',(52.5996448073063,20.5068010554466,8.6679258805469));
#33191=CARTESIAN_POINT('Ctrl Pts',(52.6163507093547,20.4254949229552,8.67222589676899));
#33192=CARTESIAN_POINT('Ctrl Pts',(52.6371795746486,20.3450985416839,8.67652591299108));
#33193=CARTESIAN_POINT('Ctrl Pts',(52.6619977589626,20.2660410291411,8.68082592921317));
#33194=CARTESIAN_POINT('Ctrl Pts',(52.6868364033699,20.1869183416418,8.68512949036554));
#33195=CARTESIAN_POINT('Ctrl Pts',(52.7156707645301,20.1091371353627,8.6894330515179));
#33196=CARTESIAN_POINT('Ctrl Pts',(52.7483187471438,20.0331071488858,8.69373661267027));
#33197=CARTESIAN_POINT('Ctrl Pts',(52.7810346800022,19.9569189212014,8.69804913082428));
#33198=CARTESIAN_POINT('Ctrl Pts',(52.8175798980594,19.8824895922892,8.70236164897828));
#33199=CARTESIAN_POINT('Ctrl Pts',(52.8577259346309,19.8102050265499,8.70667416713229));
#33200=CARTESIAN_POINT('Ctrl Pts',(52.8874910987764,19.756611642292,8.70987156397881));
#33201=CARTESIAN_POINT('Ctrl Pts',(52.9192346953156,19.7041967242502,8.71306896082534));
#33202=CARTESIAN_POINT('Ctrl Pts',(52.9528488415688,19.6531063945012,8.71626635767186));
#33203=CARTESIAN_POINT('Ctrl Pts',(52.9973333307875,19.5854941694044,8.72049774776804));
#33204=CARTESIAN_POINT('Ctrl Pts',(53.0452543647997,19.5199614369122,8.72472913786422));
#33205=CARTESIAN_POINT('Ctrl Pts',(53.0963910874101,19.456878696308,8.7289605279604));
#33206=CARTESIAN_POINT('Ctrl Pts',(53.1474545003025,19.3938863912592,8.73318585192644));
#33207=CARTESIAN_POINT('Ctrl Pts',(53.2017241556532,19.3333374604473,8.73741117589249));
#33208=CARTESIAN_POINT('Ctrl Pts',(53.2589356744407,19.2755739319226,8.74163649985853));
#33209=CARTESIAN_POINT('Ctrl Pts',(53.3162912702017,19.2176649362868,8.74587246454696));
#33210=CARTESIAN_POINT('Ctrl Pts',(53.3766033000059,19.1625557800068,8.75010842923539));
#33211=CARTESIAN_POINT('Ctrl Pts',(53.4395643536709,19.1105580602555,8.75434439392382));
#33212=CARTESIAN_POINT('Ctrl Pts',(53.5022542940963,19.0587842451155,8.75856211835035));
#33213=CARTESIAN_POINT('Ctrl Pts',(53.567570136524,19.0100954301877,8.76277984277687));
#33214=CARTESIAN_POINT('Ctrl Pts',(53.6351725367441,18.9647613787218,8.76699756720339));
#33215=CARTESIAN_POINT('Ctrl Pts',(53.7027526198979,18.9194422930416,8.77121389926462));
#33216=CARTESIAN_POINT('Ctrl Pts',(53.7726173760282,18.8774760302271,8.77543023132585));
#33217=CARTESIAN_POINT('Ctrl Pts',(53.8443973110694,18.8390898502398,8.77964656338708));
#33218=CARTESIAN_POINT('Ctrl Pts',(53.9161755347366,18.8007045854542,8.78386279492271));
#33219=CARTESIAN_POINT('Ctrl Pts',(53.9898684360633,18.7658994520344,8.78807902645834));
#33220=CARTESIAN_POINT('Ctrl Pts',(54.0650819530737,18.7348557450945,8.79229525799397));
#33221=CARTESIAN_POINT('Ctrl Pts',(54.1409043996592,18.7035607079147,8.79654562419287));
#33222=CARTESIAN_POINT('Ctrl Pts',(54.2182717590573,18.6760884781144,8.80079599039178));
#33223=CARTESIAN_POINT('Ctrl Pts',(54.2967615807266,18.6525746070092,8.80504635659068));
#33224=CARTESIAN_POINT('Ctrl Pts',(54.37473421048,18.6292156755356,8.80926871590933));
#33225=CARTESIAN_POINT('Ctrl Pts',(54.4538140839922,18.6097631464843,8.81349107522797));
#33226=CARTESIAN_POINT('Ctrl Pts',(54.5335754404777,18.5942987757674,8.81771343454661));
#33227=CARTESIAN_POINT('Ctrl Pts',(54.614130381755,18.5786805424539,8.82197780418565));
#33228=CARTESIAN_POINT('Ctrl Pts',(54.6953799615533,18.5671303369363,8.82624217382469));
#33229=CARTESIAN_POINT('Ctrl Pts',(54.7768808099841,18.5596786938916,8.83050654346373));
#33230=CARTESIAN_POINT('Ctrl Pts',(54.8583816584149,18.5522270508469,8.83477091310277));
#33231=CARTESIAN_POINT('Ctrl Pts',(54.9401332918113,18.5488739258957,8.8390352827418));
#33232=CARTESIAN_POINT('Ctrl Pts',(55.0216948174201,18.5495960363856,8.84329965238084));
#33233=CARTESIAN_POINT('Ctrl Pts',(55.1026239270472,18.5503125477378,8.84753095672971));
#33234=CARTESIAN_POINT('Ctrl Pts',(55.1836691614056,18.5550439596971,8.85176226107857));
#33235=CARTESIAN_POINT('Ctrl Pts',(55.2643994752335,18.5638055973514,8.85599356542743));
#33236=CARTESIAN_POINT('Ctrl Pts',(55.3450140680852,18.5725546758416,8.86021880451225));
#33237=CARTESIAN_POINT('Ctrl Pts',(55.425314178663,18.5853224566516,8.86444404359707));
#33238=CARTESIAN_POINT('Ctrl Pts',(55.5048690847785,18.6020722577119,8.86866928268188));
#33239=CARTESIAN_POINT('Ctrl Pts',(55.5846263394862,18.6188646620361,8.87290526869888));
#33240=CARTESIAN_POINT('Ctrl Pts',(55.6636341222117,18.639659358033,8.87714125471588));
#33241=CARTESIAN_POINT('Ctrl Pts',(55.7414639155221,18.6643669997239,8.88137724073288));
#33242=CARTESIAN_POINT('Ctrl Pts',(55.8189566713769,18.6889676463897,8.8855948830554));
#33243=CARTESIAN_POINT('Ctrl Pts',(55.8952811706885,18.7174472858186,8.88981252537793));
#33244=CARTESIAN_POINT('Ctrl Pts',(55.970026763108,18.7496670626651,8.89403016770045));
#33245=CARTESIAN_POINT('Ctrl Pts',(56.0447477017894,18.7818762122905,8.89824641889548));
#33246=CARTESIAN_POINT('Ctrl Pts',(56.1178903411844,18.817822865629,8.90246267009049));
#33247=CARTESIAN_POINT('Ctrl Pts',(56.1890633963501,18.8573197883351,8.90667892128552));
#33248=CARTESIAN_POINT('Ctrl Pts',(56.2602347774529,18.8968157820332,8.91089507331002));
#33249=CARTESIAN_POINT('Ctrl Pts',(56.3294362604733,18.9398616525109,8.91511122533452));
#33250=CARTESIAN_POINT('Ctrl Pts',(56.396301861268,18.9862245998574,8.91932737735901));
#33251=CARTESIAN_POINT('Ctrl Pts',(56.4637116313637,19.0329648606857,8.92357784150325));
#33252=CARTESIAN_POINT('Ctrl Pts',(56.528746921495,19.0830761764581,8.92782830564748));
#33253=CARTESIAN_POINT('Ctrl Pts',(56.5910647494884,19.1362770557469,8.93207876979172));
#33254=CARTESIAN_POINT('Ctrl Pts',(56.6529694163975,19.1891252184266,8.93630105377578));
#33255=CARTESIAN_POINT('Ctrl Pts',(56.7121922461191,19.2450217344356,8.94052333775984));
#33256=CARTESIAN_POINT('Ctrl Pts',(56.7684337064739,19.3036531970712,8.9447456217439));
#33257=CARTESIAN_POINT('Ctrl Pts',(56.8252382128131,19.3628716325446,8.94901017596822));
#33258=CARTESIAN_POINT('Ctrl Pts',(56.8790010037236,19.4248797141324,8.95327473019254));
#33259=CARTESIAN_POINT('Ctrl Pts',(56.9294559916372,19.4893214020397,8.95753928441686));
#33260=CARTESIAN_POINT('Ctrl Pts',(56.9799109795508,19.5537630899469,8.96180383864118));
#33261=CARTESIAN_POINT('Ctrl Pts',(57.0270579394572,19.6206379535486,8.9660683928655));
#33262=CARTESIAN_POINT('Ctrl Pts',(57.0706773591257,19.689562849884,8.97033294708982));
#33263=CARTESIAN_POINT('Ctrl Pts',(57.113954896683,19.7579475237852,8.97456407641275));
#33264=CARTESIAN_POINT('Ctrl Pts',(57.1539223370878,19.8286066506894,8.97879520573567));
#33265=CARTESIAN_POINT('Ctrl Pts',(57.1903330678364,19.90118641165,8.98302633505859));
#33266=CARTESIAN_POINT('Ctrl Pts',(57.2266915748675,19.9736620718456,8.98725139569523));
#33267=CARTESIAN_POINT('Ctrl Pts',(57.2595032972075,20.0480524828814,8.99147645633188));
#33268=CARTESIAN_POINT('Ctrl Pts',(57.2885654926829,20.1239758931964,8.99570151696852));
#33269=CARTESIAN_POINT('Ctrl Pts',(57.3177031426095,20.2000964241749,8.99993754716978));
#33270=CARTESIAN_POINT('Ctrl Pts',(57.3430715233589,20.2777575227887,9.00417357737104));
#33271=CARTESIAN_POINT('Ctrl Pts',(57.3645133119766,20.3565506643989,9.0084096075723));
#33272=CARTESIAN_POINT('Ctrl Pts',(57.3858610866042,20.4349983284111,9.01262706441161));
#33273=CARTESIAN_POINT('Ctrl Pts',(57.4033164994337,20.5145676796993,9.01684452125091));
#33274=CARTESIAN_POINT('Ctrl Pts',(57.416773540449,20.5948384221257,9.02106197809021));
#33275=CARTESIAN_POINT('Ctrl Pts',(57.4302261355124,20.6750826446162,9.0252780415615));
#33276=CARTESIAN_POINT('Ctrl Pts',(57.4396829052383,20.7560273398839,9.02949410503279));
#33277=CARTESIAN_POINT('Ctrl Pts',(57.4450889889884,20.8372422477182,9.03371016850408));
#33278=CARTESIAN_POINT('Ctrl Pts',(57.4504949430223,20.9184552068436,9.03792613081315));
#33279=CARTESIAN_POINT('Ctrl Pts',(57.4518503745512,20.9999379016525,9.04214209312222));
#33280=CARTESIAN_POINT('Ctrl Pts',(57.449152427175,21.0812566210407,9.04635805543129));
#33281=CARTESIAN_POINT('Ctrl Pts',(57.4464322612815,21.1632450278314,9.05060873762859));
#33282=CARTESIAN_POINT('Ctrl Pts',(57.4395916443802,21.2450662657673,9.05485941982588));
#33283=CARTESIAN_POINT('Ctrl Pts',(57.4286811215174,21.3262794201067,9.05911010202317));
#33284=CARTESIAN_POINT('Ctrl Pts',(57.4178439849383,21.4069463190864,9.06333219331112));
#33285=CARTESIAN_POINT('Ctrl Pts',(57.402991671001,21.4870128391883,9.06755428459908));
#33286=CARTESIAN_POINT('Ctrl Pts',(57.3842250890649,21.5660573952115,9.07177637588703));
#33287=CARTESIAN_POINT('Ctrl Pts',(57.3652678834759,21.6459048551444,9.07604135353899));
#33288=CARTESIAN_POINT('Ctrl Pts',(57.3423165757122,21.7247090052469,9.08030633119095));
#33289=CARTESIAN_POINT('Ctrl Pts',(57.3155261021999,21.8020530655954,9.08457130884292));
#33290=CARTESIAN_POINT('Ctrl Pts',(57.2887356286876,21.8793971259439,9.08883628649488));
#33291=CARTESIAN_POINT('Ctrl Pts',(57.2581062294484,21.9552806736383,9.09310126414684));
#33292=CARTESIAN_POINT('Ctrl Pts',(57.2238408955478,22.0293113820847,9.0973662417988));
#33293=CARTESIAN_POINT('Ctrl Pts',(57.1898465433513,22.1027566309648,9.10159749058312));
#33294=CARTESIAN_POINT('Ctrl Pts',(57.1521461140952,22.1746536964031,9.10582873936745));
#33295=CARTESIAN_POINT('Ctrl Pts',(57.1109032105033,22.2446035054936,9.11005998815177));
#33296=CARTESIAN_POINT('Ctrl Pts',(57.069719443434,22.3144530163967,9.11428516992049));
#33297=CARTESIAN_POINT('Ctrl Pts',(57.0250035242599,22.3823604191509,9.1185103516892));
#33298=CARTESIAN_POINT('Ctrl Pts',(56.9769663118386,22.4479483595264,9.12273553345791));
#33299=CARTESIAN_POINT('Ctrl Pts',(56.9288061026312,22.513704234415,9.12697153358499));
#33300=CARTESIAN_POINT('Ctrl Pts',(56.8773077746333,22.5771283284492,9.13120753371207));
#33301=CARTESIAN_POINT('Ctrl Pts',(56.8227292797739,22.6378669734307,9.13544353383915));
#33302=CARTESIAN_POINT('Ctrl Pts',(56.7683881032024,22.6983415145509,9.13966111498454));
#33303=CARTESIAN_POINT('Ctrl Pts',(56.7109937969682,22.756153558255,9.14387869612993));
#33304=CARTESIAN_POINT('Ctrl Pts',(56.6508420524642,22.8109861313151,9.14809627727531));
#33305=CARTESIAN_POINT('Ctrl Pts',(56.5907101672733,22.8658006012057,9.15231246597124));
#33306=CARTESIAN_POINT('Ctrl Pts',(56.5278229950112,22.9176372409537,9.15652865466716));
#33307=CARTESIAN_POINT('Ctrl Pts',(56.4625123322713,22.9662166533611,9.16074484336308));
#33308=CARTESIAN_POINT('Ctrl Pts',(56.3972032249617,23.0147949088074,9.1649609316468));
#33309=CARTESIAN_POINT('Ctrl Pts',(56.3294711156287,23.0601158145682,9.16917701993052));
#33310=CARTESIAN_POINT('Ctrl Pts',(56.2596788971637,23.1019417989184,9.17339310821423));
#33311=CARTESIAN_POINT('Ctrl Pts',(56.1893164437269,23.1441095210659,9.17764364390536));
#33312=CARTESIAN_POINT('Ctrl Pts',(56.1168604651603,23.1827246880677,9.18189417959649));
#33313=CARTESIAN_POINT('Ctrl Pts',(56.0427087845393,23.2175907288417,9.18614471528762));
#33314=CARTESIAN_POINT('Ctrl Pts',(55.9690511163499,23.2522244854997,9.19036693311118));
#33315=CARTESIAN_POINT('Ctrl Pts',(55.8937207293832,23.2831587976864,9.19458915093473));
#33316=CARTESIAN_POINT('Ctrl Pts',(55.8171265895045,23.3102498537441,9.19881136875829));
#33317=CARTESIAN_POINT('Ctrl Pts',(55.739761889176,23.3376134541032,9.2030760633832));
#33318=CARTESIAN_POINT('Ctrl Pts',(55.6611083311514,23.3610558966466,9.20734075800812));
#33319=CARTESIAN_POINT('Ctrl Pts',(55.5816000133454,23.3804813955326,9.21160545263304));
#33320=CARTESIAN_POINT('Ctrl Pts',(55.5020916955393,23.3999068944186,9.21587014725795));
#33321=CARTESIAN_POINT('Ctrl Pts',(55.421729103167,23.4153154220188,9.22013484188287));
#33322=CARTESIAN_POINT('Ctrl Pts',(55.3409518431461,23.4266648080555,9.22439953650778));
#33323=CARTESIAN_POINT('Ctrl Pts',(55.260808466249,23.437925132093,9.22863076480876));
#33324=CARTESIAN_POINT('Ctrl Pts',(55.1799564086001,23.4452320607928,9.23286199310974));
#33325=CARTESIAN_POINT('Ctrl Pts',(55.098819690326,23.4485066711781,9.23709322141072));
#33326=CARTESIAN_POINT('Ctrl Pts',(55.0177993118685,23.4517765861853,9.24131838266418));
#33327=CARTESIAN_POINT('Ctrl Pts',(54.9364955440597,23.4510256474488,9.24554354391765));
#33328=CARTESIAN_POINT('Ctrl Pts',(54.8553397818511,23.4462264145588,9.24976870517112));
#33329=CARTESIAN_POINT('Ctrl Pts',(54.7739757310339,23.4414148642989,9.25400471042302));
#33330=CARTESIAN_POINT('Ctrl Pts',(54.6927609148197,23.4325341538951,9.25824071567493));
#33331=CARTESIAN_POINT('Ctrl Pts',(54.6121323693784,23.419609255875,9.26247672092683));
#33332=CARTESIAN_POINT('Ctrl Pts',(54.5318548992027,23.406740635839,9.26669428163579));
#33333=CARTESIAN_POINT('Ctrl Pts',(54.4521590681906,23.3898630393969,9.27091184234475));
#33334=CARTESIAN_POINT('Ctrl Pts',(54.373471535494,23.3690530456627,9.27512940305371));
#33335=CARTESIAN_POINT('Ctrl Pts',(54.2948099804698,23.3482499220791,9.27934557138949));
#33336=CARTESIAN_POINT('Ctrl Pts',(54.217156511829,23.3235170980812,9.28356173972527));
#33337=CARTESIAN_POINT('Ctrl Pts',(54.1409257931169,23.2949818642134,9.28777790806105));
#33338=CARTESIAN_POINT('Ctrl Pts',(54.064696888021,23.2664473092315,9.29199397608936));
#33339=CARTESIAN_POINT('Ctrl Pts',(53.9898911005788,23.2341106882708,9.29621004411767));
#33340=CARTESIAN_POINT('Ctrl Pts',(53.9169048121914,23.1981480987745,9.30042611214597));
#33341=CARTESIAN_POINT('Ctrl Pts',(53.8433214187941,23.1618912972716,9.30467667206854));
#33342=CARTESIAN_POINT('Ctrl Pts',(53.7715878700404,23.1219491226593,9.3089272319911));
#33343=CARTESIAN_POINT('Ctrl Pts',(53.7020850487283,23.0785492607262,9.31317779191367));
#33344=CARTESIAN_POINT('Ctrl Pts',(53.6330459854035,23.0354389846292,9.31739998994994));
#33345=CARTESIAN_POINT('Ctrl Pts',(53.5662083210735,22.9889173426043,9.32162218798621));
#33346=CARTESIAN_POINT('Ctrl Pts',(53.5019146379084,22.9392499833407,9.32584438602249));
#33347=CARTESIAN_POINT('Ctrl Pts',(53.43697313217,22.8890821762118,9.3301091268882));
#33348=CARTESIAN_POINT('Ctrl Pts',(53.3746275312274,22.8357052187734,9.33437386775391));
#33349=CARTESIAN_POINT('Ctrl Pts',(53.3151937054493,22.7794319317811,9.33863860861962));
#33350=CARTESIAN_POINT('Ctrl Pts',(53.2557598796711,22.7231586447889,9.34290334948534));
#33351=CARTESIAN_POINT('Ctrl Pts',(53.1992381153865,22.663989420995,9.34716809035105));
#33352=CARTESIAN_POINT('Ctrl Pts',(53.1459022174421,22.6022707832055,9.35143283121676));
#33353=CARTESIAN_POINT('Ctrl Pts',(53.0934104411699,22.5415289366906,9.35563007607454));
#33354=CARTESIAN_POINT('Ctrl Pts',(53.0437996775331,22.4780807482771,9.35982732093232));
#33355=CARTESIAN_POINT('Ctrl Pts',(52.9973646295413,22.4122329209403,9.36402456579009));
#33356=CARTESIAN_POINT('Ctrl Pts',(52.9509918326174,22.346473369545,9.36821618379948));
#33357=CARTESIAN_POINT('Ctrl Pts',(52.9077865744021,22.2783209440572,9.37240780180887));
#33358=CARTESIAN_POINT('Ctrl Pts',(52.8680047304671,22.2081168903254,9.37659941981826));
#33359=CARTESIAN_POINT('Ctrl Pts',(52.8282635509888,22.1379845982169,9.38078675321307));
#33360=CARTESIAN_POINT('Ctrl Pts',(52.7919390721948,22.065805249046,9.38497408660787));
#33361=CARTESIAN_POINT('Ctrl Pts',(52.759244187876,21.9919494142508,9.38916142000267));
#33362=CARTESIAN_POINT('Ctrl Pts',(52.7265723169706,21.9181455654128,9.39334580599953));
#33363=CARTESIAN_POINT('Ctrl Pts',(52.6975251579487,21.842668005412,9.3975301919964));
#33364=CARTESIAN_POINT('Ctrl Pts',(52.6722691891804,21.7659109101985,9.40171457799326));
#33365=CARTESIAN_POINT('Ctrl Pts',(52.6470180173743,21.689168393752,9.40589816923378));
#33366=CARTESIAN_POINT('Ctrl Pts',(52.6255567618322,21.6111472707469,9.4100817604743));
#33367=CARTESIAN_POINT('Ctrl Pts',(52.6080028976971,21.5322594410385,9.41426535171482));
#33368=CARTESIAN_POINT('Ctrl Pts',(52.5904506362686,21.4533788139631,9.41844856098422));
#33369=CARTESIAN_POINT('Ctrl Pts',(52.5768051527144,21.3736321005787,9.42263177025363));
#33370=CARTESIAN_POINT('Ctrl Pts',(52.5671329872607,21.2934422401849,9.42681497952303));
#33371=CARTESIAN_POINT('Ctrl Pts',(52.5574557755994,21.2132105427607,9.43100037127602));
#33372=CARTESIAN_POINT('Ctrl Pts',(52.5517560652642,21.1325357075258,9.435185763029));
#33373=CARTESIAN_POINT('Ctrl Pts',(52.5500485115664,21.0518454850662,9.43937115478199));
#33374=CARTESIAN_POINT('Ctrl Pts',(52.5496675473193,21.0338430703327,9.44030493778397));
#33375=CARTESIAN_POINT('Ctrl Pts',(52.5494850909459,21.0158398899857,9.44123872078596));
#33376=CARTESIAN_POINT('Ctrl Pts',(52.549500951365,20.9978406855638,9.44217250378794));
#33377=CARTESIAN_POINT('',(52.5495000065655,21.0001793810522,10.2421725038327));
#33378=CARTESIAN_POINT('Ctrl Pts',(52.5495009513656,20.9978406848801,9.44217250382341));
#33379=CARTESIAN_POINT('Ctrl Pts',(52.5495886065576,20.8983651786185,9.44733320619029));
#33380=CARTESIAN_POINT('Ctrl Pts',(52.5557371744544,20.7991567821712,9.45249390855717));
#33381=CARTESIAN_POINT('Ctrl Pts',(52.5678270520411,20.7008595627187,9.45765461092406));
#33382=CARTESIAN_POINT('Ctrl Pts',(52.580109737472,20.6009947115979,9.46289761552193));
#33383=CARTESIAN_POINT('Ctrl Pts',(52.5985246902829,20.5020702618922,9.46814062011981));
#33384=CARTESIAN_POINT('Ctrl Pts',(52.6228978721534,20.4047389448427,9.47338362471768));
#33385=CARTESIAN_POINT('Ctrl Pts',(52.6307735551381,20.3732883693027,9.47507779178704));
#33386=CARTESIAN_POINT('Ctrl Pts',(52.6392709797487,20.3420039670236,9.47677195885639));
#33387=CARTESIAN_POINT('Ctrl Pts',(52.6483832195965,20.3109072862634,9.47846612592574));
#33388=CARTESIAN_POINT('Ctrl Pts',(52.6711412674524,20.2332425451333,9.4826973507271));
#33389=CARTESIAN_POINT('Ctrl Pts',(52.6977935641045,20.1565608183473,9.48692857552846));
#33390=CARTESIAN_POINT('Ctrl Pts',(52.7282373323909,20.0812809830761,9.49115980032983));
#33391=CARTESIAN_POINT('Ctrl Pts',(52.7586374468349,20.0061090928542,9.49538495790524));
#33392=CARTESIAN_POINT('Ctrl Pts',(52.7928180624719,19.9323355291198,9.49961011548066));
#33393=CARTESIAN_POINT('Ctrl Pts',(52.830626453431,19.8603646787473,9.50383527305608));
#33394=CARTESIAN_POINT('Ctrl Pts',(52.8685319217436,19.7882090350127,9.50807127920519));
#33395=CARTESIAN_POINT('Ctrl Pts',(52.9100836797597,19.7178658249795,9.5123072853543));
#33396=CARTESIAN_POINT('Ctrl Pts',(52.9550789186719,19.6497229835549,9.51654329150341));
#33397=CARTESIAN_POINT('Ctrl Pts',(52.999878185035,19.5818769318943,9.52076084812446));
#33398=CARTESIAN_POINT('Ctrl Pts',(53.0480907483382,19.5162125167468,9.52497840474551));
#33399=CARTESIAN_POINT('Ctrl Pts',(53.0994710522777,19.4530869549747,9.52919596136656));
#33400=CARTESIAN_POINT('Ctrl Pts',(53.150834391881,19.3899822354937,9.53341212546864));
#33401=CARTESIAN_POINT('Ctrl Pts',(53.2053631018543,19.3294150650192,9.53762828957072));
#33402=CARTESIAN_POINT('Ctrl Pts',(53.262770360231,19.2717108376466,9.54184445367279));
#33403=CARTESIAN_POINT('Ctrl Pts',(53.3201762509071,19.2140079850499,9.54606051732676));
#33404=CARTESIAN_POINT('Ctrl Pts',(53.3804602249465,19.159168268753,9.55027658098073));
#33405=CARTESIAN_POINT('Ctrl Pts',(53.4432985200949,19.107480316493,9.5544926446347));
#33406=CARTESIAN_POINT('Ctrl Pts',(53.5066510353778,19.0553693899034,9.55874320930137));
#33407=CARTESIAN_POINT('Ctrl Pts',(53.5725995095767,19.0064623657227,9.56299377396804));
#33408=CARTESIAN_POINT('Ctrl Pts',(53.6407795565335,18.9610124973255,9.56724433863471));
#33409=CARTESIAN_POINT('Ctrl Pts',(53.7085045211023,18.9158659938505,9.57146653199327));
#33410=CARTESIAN_POINT('Ctrl Pts',(53.7784309240605,18.8741308231446,9.57568872535183));
#33411=CARTESIAN_POINT('Ctrl Pts',(53.8501755696681,18.8360096974774,9.5799109187104));
#33412=CARTESIAN_POINT('Ctrl Pts',(53.9226433546275,18.7975043356644,9.58417566903112));
#33413=CARTESIAN_POINT('Ctrl Pts',(53.9969658019666,18.7626864893385,9.58844041935184));
#33414=CARTESIAN_POINT('Ctrl Pts',(54.0727277340705,18.7317150983975,9.59270516967257));
#33415=CARTESIAN_POINT('Ctrl Pts',(54.1484896661744,18.7007437074564,9.59696991999329));
#33416=CARTESIAN_POINT('Ctrl Pts',(54.2256906071985,18.6736188709929,9.60123467031401));
#33417=CARTESIAN_POINT('Ctrl Pts',(54.3039020009561,18.6504473136941,9.60549942063474));
#33418=CARTESIAN_POINT('Ctrl Pts',(54.3814984979045,18.6274579308327,9.60973064155215));
#33419=CARTESIAN_POINT('Ctrl Pts',(54.4603805779328,18.608273637356,9.61396186246957));
#33420=CARTESIAN_POINT('Ctrl Pts',(54.5401405584574,18.5930352009171,9.61819308338698));
#33421=CARTESIAN_POINT('Ctrl Pts',(54.6197861692198,18.5778186152402,9.62241823705454));
#33422=CARTESIAN_POINT('Ctrl Pts',(54.7003067275132,18.5665367357808,9.6266433907221));
#33423=CARTESIAN_POINT('Ctrl Pts',(54.7812796426594,18.5592805045879,9.63086854438966));
#33424=CARTESIAN_POINT('Ctrl Pts',(54.8624605587454,18.552005633793,9.63510455151275));
#33425=CARTESIAN_POINT('Ctrl Pts',(54.9440957042696,18.5487772476019,9.63934055863584));
#33426=CARTESIAN_POINT('Ctrl Pts',(55.0257491544411,18.5496352861165,9.64357656575892));
#33427=CARTESIAN_POINT('Ctrl Pts',(55.1070468760822,18.5504895865308,9.64779411844333));
#33428=CARTESIAN_POINT('Ctrl Pts',(55.188362275281,18.5553947836171,9.65201167112774));
#33429=CARTESIAN_POINT('Ctrl Pts',(55.2692620604703,18.5643382433533,9.65622922381215));
#33430=CARTESIAN_POINT('Ctrl Pts',(55.3501351347561,18.573278750203,9.66044538397565));
#33431=CARTESIAN_POINT('Ctrl Pts',(55.4305924057973,18.5862548208621,9.66466154413915));
#33432=CARTESIAN_POINT('Ctrl Pts',(55.5102049454675,18.6032018934377,9.66887770430264));
#33433=CARTESIAN_POINT('Ctrl Pts',(55.5898155884708,18.620148562271,9.67309376402152));
#33434=CARTESIAN_POINT('Ctrl Pts',(55.6685810856139,18.6410659470403,9.67730982374039));
#33435=CARTESIAN_POINT('Ctrl Pts',(55.7460833713172,18.6658385117897,9.68152588345927));
#33436=CARTESIAN_POINT('Ctrl Pts',(55.8242200344799,18.6908138467742,9.68577645278297));
#33437=CARTESIAN_POINT('Ctrl Pts',(55.9010722494636,18.7197076336754,9.69002702210667));
#33438=CARTESIAN_POINT('Ctrl Pts',(55.9762296438501,18.7523510210737,9.69427759143038));
#33439=CARTESIAN_POINT('Ctrl Pts',(56.0508852335377,18.7847764577925,9.69849978090301));
#33440=CARTESIAN_POINT('Ctrl Pts',(56.1238681720284,18.8209013137562,9.70272197037564));
#33441=CARTESIAN_POINT('Ctrl Pts',(56.194800356877,18.8605135295575,9.70694415984827));
#33442=CARTESIAN_POINT('Ctrl Pts',(56.2664477079404,18.9005251313145,9.71120891909751));
#33443=CARTESIAN_POINT('Ctrl Pts',(56.3360023079129,18.9440945526786,9.71547367834675));
#33444=CARTESIAN_POINT('Ctrl Pts',(56.4031054890392,18.9909591251973,9.71973843759599));
#33445=CARTESIAN_POINT('Ctrl Pts',(56.4702086701655,19.037823697716,9.72400319684523));
#33446=CARTESIAN_POINT('Ctrl Pts',(56.5348600911658,19.0879830752915,9.72826795609447));
#33447=CARTESIAN_POINT('Ctrl Pts',(56.5967377036965,19.1411350356752,9.73253271534371));
#33448=CARTESIAN_POINT('Ctrl Pts',(56.6581286759659,19.1938689792217,9.73676393413348));
#33449=CARTESIAN_POINT('Ctrl Pts',(56.7170195532931,19.2497463153063,9.74099515292325));
#33450=CARTESIAN_POINT('Ctrl Pts',(56.7730710033144,19.308500822582,9.74522637171302));
#33451=CARTESIAN_POINT('Ctrl Pts',(56.8290420791093,19.3671710796186,9.74945152320325));
#33452=CARTESIAN_POINT('Ctrl Pts',(56.8821814958066,19.4287099803759,9.75367667469348));
#33453=CARTESIAN_POINT('Ctrl Pts',(56.9321837027249,19.4928117606204,9.75790182618371));
#33454=CARTESIAN_POINT('Ctrl Pts',(56.9823143861035,19.5570782449916,9.76213783384492));
#33455=CARTESIAN_POINT('Ctrl Pts',(57.0292913635986,19.6239204834868,9.76637384150613));
#33456=CARTESIAN_POINT('Ctrl Pts',(57.0728447075579,19.6929938529796,9.77060984916733));
#33457=CARTESIAN_POINT('Ctrl Pts',(57.1162082795827,19.7617662539184,9.77482739956911));
#33458=CARTESIAN_POINT('Ctrl Pts',(57.1561777345011,19.8327499918985,9.77904494997088));
#33459=CARTESIAN_POINT('Ctrl Pts',(57.1925287476046,19.9055741501008,9.78326250037265));
#33460=CARTESIAN_POINT('Ctrl Pts',(57.2288677582892,19.97837426314,9.78747865821884));
#33461=CARTESIAN_POINT('Ctrl Pts',(57.2615904922698,20.0530131739984,9.79169481606503));
#33462=CARTESIAN_POINT('Ctrl Pts',(57.2905186224002,20.1290954757048,9.79591097391123));
#33463=CARTESIAN_POINT('Ctrl Pts',(57.3194460631376,20.2051759642761,9.80012703128118));
#33464=CARTESIAN_POINT('Ctrl Pts',(57.3445789156268,20.2826993403403,9.80434308865113));
#33465=CARTESIAN_POINT('Ctrl Pts',(57.3657875728272,20.361251684733,9.80855914602108));
#33466=CARTESIAN_POINT('Ctrl Pts',(57.3871698540912,20.440447095639,9.81280971802372));
#33467=CARTESIAN_POINT('Ctrl Pts',(57.4045632523075,20.5206879409317,9.81706029002635));
#33468=CARTESIAN_POINT('Ctrl Pts',(57.417887129105,20.6015378551122,9.82131086202899));
#33469=CARTESIAN_POINT('Ctrl Pts',(57.4311220302655,20.6818478609222,9.82553304909854));
#33470=CARTESIAN_POINT('Ctrl Pts',(57.4403416045215,20.7627583522951,9.82975523616809));
#33471=CARTESIAN_POINT('Ctrl Pts',(57.4455190161863,20.8438366513195,9.83397742323764));
#33472=CARTESIAN_POINT('Ctrl Pts',(57.4507486379313,20.925732560526,9.83824218770682));
#33473=CARTESIAN_POINT('Ctrl Pts',(57.4518541076335,21.0077991950925,9.84250695217599));
#33474=CARTESIAN_POINT('Ctrl Pts',(57.4488616512167,21.0895927631027,9.84677171664517));
#33475=CARTESIAN_POINT('Ctrl Pts',(57.4458691947999,21.1713863311129,9.85103648111434));
#33476=CARTESIAN_POINT('Ctrl Pts',(57.4387789180195,21.2529063581448,9.85530124558352));
#33477=CARTESIAN_POINT('Ctrl Pts',(57.4276701375239,21.3337183743441,9.85956601005269));
#33478=CARTESIAN_POINT('Ctrl Pts',(57.4166487304825,21.4138947829709,9.86379723103763));
#33479=CARTESIAN_POINT('Ctrl Pts',(57.4016305233529,21.4936749372697,9.86802845202257));
#33480=CARTESIAN_POINT('Ctrl Pts',(57.3826552117956,21.5726293667839,9.8722596730075));
#33481=CARTESIAN_POINT('Ctrl Pts',(57.3637071094665,21.6514705813405,9.8764848267267));
#33482=CARTESIAN_POINT('Ctrl Pts',(57.3408132798271,21.7294879744486,9.8807099804459));
#33483=CARTESIAN_POINT('Ctrl Pts',(57.3140649610287,21.8062590192608,9.8849351341651));
#33484=CARTESIAN_POINT('Ctrl Pts',(57.2872479323257,21.8832272701554,9.88917114127329));
#33485=CARTESIAN_POINT('Ctrl Pts',(57.2565566572777,21.9589422946898,9.89340714838148));
#33486=CARTESIAN_POINT('Ctrl Pts',(57.2221343399255,22.0329904284763,9.89764315548967));
#33487=CARTESIAN_POINT('Ctrl Pts',(57.1878619854026,22.1067159672578,9.90186070818633));
#33488=CARTESIAN_POINT('Ctrl Pts',(57.1498912195992,22.1787886810994,9.90607826088299));
#33489=CARTESIAN_POINT('Ctrl Pts',(57.1084120666089,22.2488189650138,9.91029581357964));
#33490=CARTESIAN_POINT('Ctrl Pts',(57.0669466090509,22.3188261265896,9.91451197374045));
#33491=CARTESIAN_POINT('Ctrl Pts',(57.0219753014447,22.3867917977215,9.91872813390126));
#33492=CARTESIAN_POINT('Ctrl Pts',(56.973733686242,22.4523517431372,9.92294429406206));
#33493=CARTESIAN_POINT('Ctrl Pts',(56.9254932205056,22.5179101264378,9.92716035376325));
#33494=CARTESIAN_POINT('Ctrl Pts',(56.8739828785433,22.5810625241831,9.93137641346443));
#33495=CARTESIAN_POINT('Ctrl Pts',(56.8194801744949,22.6414755997639,9.93559247316562));
#33496=CARTESIAN_POINT('Ctrl Pts',(56.7645313509494,22.7023831728445,9.93984304246529));
#33497=CARTESIAN_POINT('Ctrl Pts',(56.7065412620411,22.7605060056448,9.94409361176496));
#33498=CARTESIAN_POINT('Ctrl Pts',(56.6458328328143,22.8155397369462,9.94834418106463));
#33499=CARTESIAN_POINT('Ctrl Pts',(56.585529737066,22.8702060231657,9.9525663704826));
#33500=CARTESIAN_POINT('Ctrl Pts',(56.5225448920022,22.9218240826417,9.95678855990056));
#33501=CARTESIAN_POINT('Ctrl Pts',(56.4572272983366,22.9701367594618,9.96101074931852));
#33502=CARTESIAN_POINT('Ctrl Pts',(56.3912511462556,23.0189365442432,9.96527550855905));
#33503=CARTESIAN_POINT('Ctrl Pts',(56.3228953459908,23.0643636499391,9.96954026779957));
#33504=CARTESIAN_POINT('Ctrl Pts',(56.2525470057195,23.1061994797414,9.9738050270401));
#33505=CARTESIAN_POINT('Ctrl Pts',(56.1821986654482,23.1480353095437,9.97806978628062));
#33506=CARTESIAN_POINT('Ctrl Pts',(56.1098582411348,23.1862796950713,9.98233454552115));
#33507=CARTESIAN_POINT('Ctrl Pts',(56.0359337950515,23.220763702484,9.98659930476167));
#33508=CARTESIAN_POINT('Ctrl Pts',(55.9625907055436,23.2549765207904,9.99083052508566));
#33509=CARTESIAN_POINT('Ctrl Pts',(55.8874134108726,23.2856162299238,9.99506174540966));
#33510=CARTESIAN_POINT('Ctrl Pts',(55.8107842910035,23.3124833152829,9.99929296573365));
#33511=CARTESIAN_POINT('Ctrl Pts',(55.7342650518872,23.3393118751367,10.0035181187862));
#33512=CARTESIAN_POINT('Ctrl Pts',(55.6562985572485,23.3623784027111,10.0077432718387));
#33513=CARTESIAN_POINT('Ctrl Pts',(55.5772893002634,23.3815304561986,10.0119684248912));
#33514=CARTESIAN_POINT('Ctrl Pts',(55.4980770721725,23.4007317104206,10.0162044321653));
#33515=CARTESIAN_POINT('Ctrl Pts',(55.4178171477371,23.4159981588874,10.0204404394394));
#33516=CARTESIAN_POINT('Ctrl Pts',(55.3369347508858,23.4272258287282,10.0246764467136));
#33517=CARTESIAN_POINT('Ctrl Pts',(55.2564047389614,23.4384045823429,10.0288939987345));
#33518=CARTESIAN_POINT('Ctrl Pts',(55.1752581295352,23.4455796034614,10.0331115507555));
#33519=CARTESIAN_POINT('Ctrl Pts',(55.09392531759,23.448699304675,10.0373291027764));
#33520=CARTESIAN_POINT('Ctrl Pts',(55.0126193598504,23.4518179758356,10.0415452622596));
#33521=CARTESIAN_POINT('Ctrl Pts',(54.9311277858973,23.4508839682967,10.0457614217428));
#33522=CARTESIAN_POINT('Ctrl Pts',(54.8498843552359,23.445897696797,10.0499775812261));
#33523=CARTESIAN_POINT('Ctrl Pts',(54.7686428604029,23.4409115441078,10.0541936402487));
#33524=CARTESIAN_POINT('Ctrl Pts',(54.6876499610865,23.4318733490222,10.0584096992714));
#33525=CARTESIAN_POINT('Ctrl Pts',(54.6073362126123,23.4188355463062,10.062625758294));
#33526=CARTESIAN_POINT('Ctrl Pts',(54.5263650459627,23.4056910210348,10.0668763283921));
#33527=CARTESIAN_POINT('Ctrl Pts',(54.4460846761135,23.3884811683558,10.0711268984901));
#33528=CARTESIAN_POINT('Ctrl Pts',(54.3669259354745,23.367312290093,10.0753774685882));
#33529=CARTESIAN_POINT('Ctrl Pts',(54.2882957432863,23.3462847579117,10.0795996573322));
#33530=CARTESIAN_POINT('Ctrl Pts',(54.2107726755594,23.3213511111254,10.0838218460763));
#33531=CARTESIAN_POINT('Ctrl Pts',(54.1347620394814,23.2926651569031,10.0880440348203));
#33532=CARTESIAN_POINT('Ctrl Pts',(54.0579849935265,23.2636899642298,10.0923087955954));
#33533=CARTESIAN_POINT('Ctrl Pts',(53.9827514956785,23.230886563881,10.0965735563704));
#33534=CARTESIAN_POINT('Ctrl Pts',(53.9094551176978,23.1944616901839,10.1008383171455));
#33535=CARTESIAN_POINT('Ctrl Pts',(53.8361587397172,23.1580368164868,10.1051030779206));
#33536=CARTESIAN_POINT('Ctrl Pts',(53.7647998703185,23.1179907612598,10.1093678386956));
#33537=CARTESIAN_POINT('Ctrl Pts',(53.6957417143754,23.0745747936335,10.1136325994707));
#33538=CARTESIAN_POINT('Ctrl Pts',(53.6272266735438,23.0315002754389,10.1178638195872));
#33539=CARTESIAN_POINT('Ctrl Pts',(53.5607193389105,22.984947175665,10.1220950397038));
#33540=CARTESIAN_POINT('Ctrl Pts',(53.4965946844597,22.9351286022394,10.1263262598204));
#33541=CARTESIAN_POINT('Ctrl Pts',(53.4325619803304,22.8853814652042,10.1305514126598));
#33542=CARTESIAN_POINT('Ctrl Pts',(53.3709055348076,22.8323784370686,10.1347765654993));
#33543=CARTESIAN_POINT('Ctrl Pts',(53.3119727599222,22.7763767299633,10.1390017183387));
#33544=CARTESIAN_POINT('Ctrl Pts',(53.2528885857669,22.7202311535497,10.1432377256654));
#33545=CARTESIAN_POINT('Ctrl Pts',(53.1965424906567,22.6610717277937,10.1474737329921));
#33546=CARTESIAN_POINT('Ctrl Pts',(53.1432524020399,22.5991993645163,10.1517097403188));
#33547=CARTESIAN_POINT('Ctrl Pts',(53.090194488868,22.5375965681292,10.1559272921145));
#33548=CARTESIAN_POINT('Ctrl Pts',(53.0401663202996,22.4733047736645,10.1601448439101));
#33549=CARTESIAN_POINT('Ctrl Pts',(52.9934446114649,22.4066576423355,10.1643623957058));
#33550=CARTESIAN_POINT('Ctrl Pts',(52.9467383290998,22.3400325164075,10.1685785549596));
#33551=CARTESIAN_POINT('Ctrl Pts',(52.9033366051359,22.2710539783736,10.1727947142134));
#33552=CARTESIAN_POINT('Ctrl Pts',(52.8634742849804,22.200086713142,10.1770108734672));
#33553=CARTESIAN_POINT('Ctrl Pts',(52.8236129146808,22.1291211389477,10.1812269322566));
#33554=CARTESIAN_POINT('Ctrl Pts',(52.7872910072233,22.0561673376716,10.185442991046));
#33555=CARTESIAN_POINT('Ctrl Pts',(52.7546979615751,21.9816155083559,10.1896590498354));
#33556=CARTESIAN_POINT('Ctrl Pts',(52.7218381176401,21.906453416945,10.1939096201974));
#33557=CARTESIAN_POINT('Ctrl Pts',(52.692768671173,21.8296674477605,10.1981601905594));
#33558=CARTESIAN_POINT('Ctrl Pts',(52.6676339104245,21.751677240708,10.2024107609215));
#33559=CARTESIAN_POINT('Ctrl Pts',(52.6426669792038,21.6742077889456,10.2066329494252));
#33560=CARTESIAN_POINT('Ctrl Pts',(52.6215824103021,21.5955506016873,10.210855137929));
#33561=CARTESIAN_POINT('Ctrl Pts',(52.6044707359118,21.5161296299351,10.2150773264328));
#33562=CARTESIAN_POINT('Ctrl Pts',(52.5871865226414,21.4359078478586,10.2193420877239));
#33563=CARTESIAN_POINT('Ctrl Pts',(52.5739558514078,21.3549072713918,10.2236068490151));
#33564=CARTESIAN_POINT('Ctrl Pts',(52.5648184199452,21.273570689515,10.2278716103062));
#33565=CARTESIAN_POINT('Ctrl Pts',(52.5556809884825,21.1922341076383,10.2321363715974));
#33566=CARTESIAN_POINT('Ctrl Pts',(52.5506367623642,21.1105620051941,10.2364011328885));
#33567=CARTESIAN_POINT('Ctrl Pts',(52.5496715539799,21.0289958035729,10.2406658941797));
#33568=CARTESIAN_POINT('Ctrl Pts',(52.5495578944551,21.0193908562159,10.2411680973824));
#33569=CARTESIAN_POINT('Ctrl Pts',(52.5495007097351,21.0097852392485,10.2416703005852));
#33570=CARTESIAN_POINT('Ctrl Pts',(52.5495000065656,21.0001793819091,10.2421725037879));
#33571=CARTESIAN_POINT('',(52.5495008566119,21.0020489641339,11.0421724789485));
#33572=CARTESIAN_POINT('Ctrl Pts',(52.5495000065655,21.0001793810522,10.2421725038327));
#33573=CARTESIAN_POINT('Ctrl Pts',(52.5494940944825,20.9194152249059,10.246394929427));
#33574=CARTESIAN_POINT('Ctrl Pts',(52.5534852447008,20.8384964272295,10.2506173550213));
#33575=CARTESIAN_POINT('Ctrl Pts',(52.5614933360761,20.7578523177923,10.2548397806156));
#33576=CARTESIAN_POINT('Ctrl Pts',(52.5694899518793,20.6773237711335,10.2590561554861));
#33577=CARTESIAN_POINT('Ctrl Pts',(52.5814920319619,20.597069591859,10.2632725303566));
#33578=CARTESIAN_POINT('Ctrl Pts',(52.5974674466584,20.5175193473994,10.2674889052271));
#33579=CARTESIAN_POINT('Ctrl Pts',(52.6134244530256,20.4380607679841,10.271700421606));
#33580=CARTESIAN_POINT('Ctrl Pts',(52.6333456042126,20.3593049670456,10.275911937985));
#33581=CARTESIAN_POINT('Ctrl Pts',(52.657147118386,20.2816751256477,10.280123454364));
#33582=CARTESIAN_POINT('Ctrl Pts',(52.6809336462747,20.2040941627753,10.2843323190215));
#33583=CARTESIAN_POINT('Ctrl Pts',(52.7085955512577,20.127638197695,10.2885411836791));
#33584=CARTESIAN_POINT('Ctrl Pts',(52.7399985197093,20.052717803881,10.2927500483367));
#33585=CARTESIAN_POINT('Ctrl Pts',(52.7713914438852,19.9778213734416,10.296957566784));
#33586=CARTESIAN_POINT('Ctrl Pts',(52.8065228750273,19.9044599694482,10.3011650852314));
#33587=CARTESIAN_POINT('Ctrl Pts',(52.8452099382239,19.8330252617683,10.3053726036787));
#33588=CARTESIAN_POINT('Ctrl Pts',(52.883896611826,19.761591273465,10.3095800797546));
#33589=CARTESIAN_POINT('Ctrl Pts',(52.9261386226279,19.6920843529753,10.3137875558306));
#33590=CARTESIAN_POINT('Ctrl Pts',(52.9717073065553,19.6248712788546,10.3179950319065));
#33591=CARTESIAN_POINT('Ctrl Pts',(53.0173211902005,19.5575915358789,10.3222066813909));
#33592=CARTESIAN_POINT('Ctrl Pts',(53.0662680755153,19.4926105716875,10.3264183308752));
#33593=CARTESIAN_POINT('Ctrl Pts',(53.1182764588268,19.4302653840235,10.3306299803596));
#33594=CARTESIAN_POINT('Ctrl Pts',(53.1703098516973,19.3678902160844,10.3348436551232));
#33595=CARTESIAN_POINT('Ctrl Pts',(53.2254073578391,19.3081536930189,10.3390573298867));
#33596=CARTESIAN_POINT('Ctrl Pts',(53.2832594495177,19.2513570597947,10.3432710046503));
#33597=CARTESIAN_POINT('Ctrl Pts',(53.3412157186426,19.1944581497464,10.34749226721));
#33598=CARTESIAN_POINT('Ctrl Pts',(53.4019361342735,19.1405100181646,10.3517135297697));
#33599=CARTESIAN_POINT('Ctrl Pts',(53.4650769767002,19.0897744733817,10.3559347923293));
#33600=CARTESIAN_POINT('Ctrl Pts',(53.5237335120291,19.0426422027211,10.3598562578491));
#33601=CARTESIAN_POINT('Ctrl Pts',(53.5844782987549,18.9982821328772,10.3637777233688));
#33602=CARTESIAN_POINT('Ctrl Pts',(53.6470151067306,18.9568695272732,10.3676991888886));
#33603=CARTESIAN_POINT('Ctrl Pts',(53.7144916687481,18.9121857587728,10.3719304091876));
#33604=CARTESIAN_POINT('Ctrl Pts',(53.7843107156218,18.870764532508,10.3761616294866));
#33605=CARTESIAN_POINT('Ctrl Pts',(53.8561235800349,18.8328597216959,10.3803928497857));
#33606=CARTESIAN_POINT('Ctrl Pts',(53.9278334698295,18.7950092637281,10.3846180028111));
#33607=CARTESIAN_POINT('Ctrl Pts',(54.0015310912931,18.7606654220311,10.3888431558365));
#33608=CARTESIAN_POINT('Ctrl Pts',(54.0768389451719,18.7300387851665,10.3930683088619));
#33609=CARTESIAN_POINT('Ctrl Pts',(54.1523402620237,18.6993334696525,10.3973043161426));
#33610=CARTESIAN_POINT('Ctrl Pts',(54.2294596980397,18.6723647373858,10.4015403234232));
#33611=CARTESIAN_POINT('Ctrl Pts',(54.3077920827892,18.649298307026,10.4057763307039));
#33612=CARTESIAN_POINT('Ctrl Pts',(54.3857831916818,18.6263323717018,10.4099938826928));
#33613=CARTESIAN_POINT('Ctrl Pts',(54.4649762557747,18.6072349463723,10.4142114346817));
#33614=CARTESIAN_POINT('Ctrl Pts',(54.5449532428255,18.5921207051048,10.4184289866706));
#33615=CARTESIAN_POINT('Ctrl Pts',(54.6249038232982,18.5770114542153,10.42264514612));
#33616=CARTESIAN_POINT('Ctrl Pts',(54.7056373562451,18.5658828619374,10.4268613055693));
#33617=CARTESIAN_POINT('Ctrl Pts',(54.7867247909581,18.5587986696693,10.4310774650187));
#33618=CARTESIAN_POINT('Ctrl Pts',(54.8678102935257,18.5517146462029,10.4352935240057));
#33619=CARTESIAN_POINT('Ctrl Pts',(54.9492492178389,18.5486748704977,10.4395095829928));
#33620=CARTESIAN_POINT('Ctrl Pts',(55.0306079885442,18.5496911621109,10.4437256419798));
#33621=CARTESIAN_POINT('Ctrl Pts',(55.1126327329865,18.550715772723,10.4479762121146));
#33622=CARTESIAN_POINT('Ctrl Pts',(55.1945755256662,18.5558631702371,10.4522267822494));
#33623=CARTESIAN_POINT('Ctrl Pts',(55.2759945504124,18.5650919405155,10.4564773523842));
#33624=CARTESIAN_POINT('Ctrl Pts',(55.3568699331744,18.5742590894835,10.4606995410887));
#33625=CARTESIAN_POINT('Ctrl Pts',(55.4372280679039,18.5874531367582,10.4649217297931));
#33626=CARTESIAN_POINT('Ctrl Pts',(55.5166453570889,18.604581910188,10.4691439184976));
#33627=CARTESIAN_POINT('Ctrl Pts',(55.5968634073559,18.6218833922973,10.4734086793476));
#33628=CARTESIAN_POINT('Ctrl Pts',(55.6761210631514,18.6431992683482,10.4776734401976));
#33629=CARTESIAN_POINT('Ctrl Pts',(55.7539985055505,18.6683832854374,10.4819382010476));
#33630=CARTESIAN_POINT('Ctrl Pts',(55.8318759479495,18.6935673025266,10.4862029618976));
#33631=CARTESIAN_POINT('Ctrl Pts',(55.9083727493533,18.7226192295344,10.4904677227476));
#33632=CARTESIAN_POINT('Ctrl Pts',(55.9830925372282,18.7553442773454,10.4947324835976));
#33633=CARTESIAN_POINT('Ctrl Pts',(56.0572246850924,18.7878119562854,10.4989637038798));
#33634=CARTESIAN_POINT('Ctrl Pts',(56.1298856760451,18.8240168954734,10.503194924162));
#33635=CARTESIAN_POINT('Ctrl Pts',(56.2006731417975,18.8638037879057,10.5074261444442));
#33636=CARTESIAN_POINT('Ctrl Pts',(56.2713591032709,18.9035336287146,10.5116512974522));
#33637=CARTESIAN_POINT('Ctrl Pts',(56.3401764732719,18.9468349958729,10.5158764504602));
#33638=CARTESIAN_POINT('Ctrl Pts',(56.4067436195039,18.9935048868774,10.5201016034682));
#33639=CARTESIAN_POINT('Ctrl Pts',(56.4734817745108,19.0402946712727,10.5243376107531));
#33640=CARTESIAN_POINT('Ctrl Pts',(56.5379576996635,19.0904701136743,10.528573618038));
#33641=CARTESIAN_POINT('Ctrl Pts',(56.5998124600216,19.1437806318327,10.532809625323));
#33642=CARTESIAN_POINT('Ctrl Pts',(56.6613977333373,19.1968588882575,10.5370271772931));
#33643=CARTESIAN_POINT('Ctrl Pts',(56.7203842741128,19.2530446605368,10.5412447292632));
#33644=CARTESIAN_POINT('Ctrl Pts',(56.7764490629299,19.3120488819828,10.5454622812334));
#33645=CARTESIAN_POINT('Ctrl Pts',(56.8324953404255,19.3710336215733,10.5496784406635));
#33646=CARTESIAN_POINT('Ctrl Pts',(56.8856214617184,19.4328346255407,10.5538946000936));
#33647=CARTESIAN_POINT('Ctrl Pts',(56.9355412283676,19.497125952287,10.5581107595237));
#33648=CARTESIAN_POINT('Ctrl Pts',(56.9854598055269,19.5614157470974,10.5623268184911));
#33649=CARTESIAN_POINT('Ctrl Pts',(57.0321718956901,19.6281953788033,10.5665428774584));
#33650=CARTESIAN_POINT('Ctrl Pts',(57.0754324736214,19.6971069508829,10.5707589364258));
#33651=CARTESIAN_POINT('Ctrl Pts',(57.1190471675672,19.7665826090756,10.5750095065825));
#33652=CARTESIAN_POINT('Ctrl Pts',(57.1591533140597,19.8382248736267,10.5792600767392));
#33653=CARTESIAN_POINT('Ctrl Pts',(57.1955461483394,19.911640059304,10.583510646896));
#33654=CARTESIAN_POINT('Ctrl Pts',(57.2316959841033,19.9845650446023,10.5877328355798));
#33655=CARTESIAN_POINT('Ctrl Pts',(57.2641818143274,20.0592388920022,10.5919550242637));
#33656=CARTESIAN_POINT('Ctrl Pts',(57.2928514014913,20.1352557021412,10.5961772129475));
#33657=CARTESIAN_POINT('Ctrl Pts',(57.3218100632935,20.2120389876313,10.6004419738407));
#33658=CARTESIAN_POINT('Ctrl Pts',(57.346874942372,20.2901920078152,10.6047067347339));
#33659=CARTESIAN_POINT('Ctrl Pts',(57.3679412905953,20.3692827144483,10.608971495627));
#33660=CARTESIAN_POINT('Ctrl Pts',(57.3890076388186,20.4483734210814,10.6132362565202));
#33661=CARTESIAN_POINT('Ctrl Pts',(57.4060754185282,20.5284013295618,10.6175010174134));
#33662=CARTESIAN_POINT('Ctrl Pts',(57.4190933765831,20.6089277747377,10.6217657783066));
#33663=CARTESIAN_POINT('Ctrl Pts',(57.4320089538018,20.6888209128491,10.6259969986256));
#33664=CARTESIAN_POINT('Ctrl Pts',(57.4409866592818,20.7695043569888,10.6302282189447));
#33665=CARTESIAN_POINT('Ctrl Pts',(57.4459388145949,20.8505558122309,10.6344594392638));
#33666=CARTESIAN_POINT('Ctrl Pts',(57.4508838688641,20.9314910453629,10.6386845923093));
#33667=CARTESIAN_POINT('Ctrl Pts',(57.4518148091863,21.0127927813999,10.6429097453547));
#33668=CARTESIAN_POINT('Ctrl Pts',(57.4486952760865,21.09403028699,10.6471348984002));
#33669=CARTESIAN_POINT('Ctrl Pts',(57.4455677290451,21.1754764881169,10.6513709056759));
#33670=CARTESIAN_POINT('Ctrl Pts',(57.4383688019827,21.2568576613764,10.6556069129515));
#33671=CARTESIAN_POINT('Ctrl Pts',(57.4271144206118,21.3377363457759,10.6598429202271));
#33672=CARTESIAN_POINT('Ctrl Pts',(57.4159090718788,21.4182626611637,10.664060472236));
#33673=CARTESIAN_POINT('Ctrl Pts',(57.4006835888085,21.498290392473,10.6682780242449));
#33674=CARTESIAN_POINT('Ctrl Pts',(57.3815057072802,21.5773913890871,10.6724955762537));
#33675=CARTESIAN_POINT('Ctrl Pts',(57.3623341578516,21.6564662683536,10.676711735723));
#33676=CARTESIAN_POINT('Ctrl Pts',(57.3392129109556,21.7346145690944,10.6809278951922));
#33677=CARTESIAN_POINT('Ctrl Pts',(57.3122606512133,21.8114190845986,10.6851440546614));
#33678=CARTESIAN_POINT('Ctrl Pts',(57.2853090336881,21.8882217700085,10.6893601136682));
#33679=CARTESIAN_POINT('Ctrl Pts',(57.254526739808,21.9636802955179,10.693576172675));
#33680=CARTESIAN_POINT('Ctrl Pts',(57.220081628862,22.0373947229428,10.6977922316818));
#33681=CARTESIAN_POINT('Ctrl Pts',(57.1853545629394,22.1117125494883,10.702042801793));
#33682=CARTESIAN_POINT('Ctrl Pts',(57.1469046267709,22.1842571516632,10.7062933719041));
#33683=CARTESIAN_POINT('Ctrl Pts',(57.1049515806814,22.2546430141626,10.7105439420153));
#33684=CARTESIAN_POINT('Ctrl Pts',(57.0632786583457,22.32455890478,10.7147661307389));
#33685=CARTESIAN_POINT('Ctrl Pts',(57.0181495763465,22.3923444395174,10.7189883194626));
#33686=CARTESIAN_POINT('Ctrl Pts',(56.9698228391822,22.4576516155228,10.7232105081863));
#33687=CARTESIAN_POINT('Ctrl Pts',(56.9210088263624,22.5236172799522,10.7274752689912));
#33688=CARTESIAN_POINT('Ctrl Pts',(56.8689326201312,22.5870539505716,10.7317400297961));
#33689=CARTESIAN_POINT('Ctrl Pts',(56.8139004459577,22.6476393483267,10.736004790601));
#33690=CARTESIAN_POINT('Ctrl Pts',(56.7588682717842,22.7082247460818,10.7402695514058));
#33691=CARTESIAN_POINT('Ctrl Pts',(56.7008805164288,22.7659585765689,10.7445343122107));
#33692=CARTESIAN_POINT('Ctrl Pts',(56.6402779712684,22.8205599212802,10.7487990730156));
#33693=CARTESIAN_POINT('Ctrl Pts',(56.5801520389524,22.8747318499968,10.7530302933186));
#33694=CARTESIAN_POINT('Ctrl Pts',(56.5172268635239,22.9260235608084,10.7572615136216));
#33695=CARTESIAN_POINT('Ctrl Pts',(56.4518097309541,22.9741324056676,10.7614927339246));
#33696=CARTESIAN_POINT('Ctrl Pts',(56.3864864019737,23.0221722658106,10.7657178869539));
#33697=CARTESIAN_POINT('Ctrl Pts',(56.3186785840612,23.0670380513405,10.7699430399832));
#33698=CARTESIAN_POINT('Ctrl Pts',(56.2487284797095,23.1084656587107,10.7741681930124));
#33699=CARTESIAN_POINT('Ctrl Pts',(56.1785986763164,23.1499996919598,10.7784042002921));
#33700=CARTESIAN_POINT('Ctrl Pts',(56.1063159204699,23.1880775481734,10.7826402075718));
#33701=CARTESIAN_POINT('Ctrl Pts',(56.0322564176405,23.222475407792,10.7868762148514));
#33702=CARTESIAN_POINT('Ctrl Pts',(55.9585195746456,23.2567234040268,10.7910937668437));
#33703=CARTESIAN_POINT('Ctrl Pts',(55.8830218550091,23.2873231980491,10.795311318836));
#33704=CARTESIAN_POINT('Ctrl Pts',(55.8061597338934,23.3140995513264,10.7995288708283));
#33705=CARTESIAN_POINT('Ctrl Pts',(55.7293229909011,23.3408670636611,10.8037450302809));
#33706=CARTESIAN_POINT('Ctrl Pts',(55.6511231797466,23.3638134893972,10.8079611897335));
#33707=CARTESIAN_POINT('Ctrl Pts',(55.5719752056556,23.3828123329619,10.8121773491861));
#33708=CARTESIAN_POINT('Ctrl Pts',(55.4928291175002,23.4018107238227,10.8163934081761));
#33709=CARTESIAN_POINT('Ctrl Pts',(55.4127353636673,23.4168616120932,10.8206094671662));
#33710=CARTESIAN_POINT('Ctrl Pts',(55.3321210033346,23.4278891838682,10.8248255261562));
#33711=CARTESIAN_POINT('Ctrl Pts',(55.2508467628784,23.4390070233746,10.8290760962869));
#33712=CARTESIAN_POINT('Ctrl Pts',(55.1690438267035,23.4460352946014,10.8333266664176));
#33713=CARTESIAN_POINT('Ctrl Pts',(55.0871552772608,23.4489496131292,10.8375772365483));
#33714=CARTESIAN_POINT('Ctrl Pts',(55.0058135047322,23.4518444725006,10.8417994252553));
#33715=CARTESIAN_POINT('Ctrl Pts',(54.9243877273233,23.4506802188239,10.8460216139623));
#33716=CARTESIAN_POINT('Ctrl Pts',(54.8433105161209,23.4454853619766,10.8502438026693));
#33717=CARTESIAN_POINT('Ctrl Pts',(54.7614158071071,23.4402381256253,10.8545085635118));
#33718=CARTESIAN_POINT('Ctrl Pts',(54.679877215646,23.4308786032364,10.8587733243544));
#33719=CARTESIAN_POINT('Ctrl Pts',(54.5991315741485,23.4174893495433,10.8630380851969));
#33720=CARTESIAN_POINT('Ctrl Pts',(54.5183859326511,23.4041000958502,10.8673028460395));
#33721=CARTESIAN_POINT('Ctrl Pts',(54.4384336981956,23.3866812761905,10.871567606882));
#33722=CARTESIAN_POINT('Ctrl Pts',(54.3596956929881,23.3653669153901,10.8758323677246));
#33723=CARTESIAN_POINT('Ctrl Pts',(54.2815769288897,23.3442201830226,10.8800635880269));
#33724=CARTESIAN_POINT('Ctrl Pts',(54.204360415008,23.319159710537,10.8842948083291));
#33725=CARTESIAN_POINT('Ctrl Pts',(54.1284670641012,23.2902795880948,10.8885260286314));
#33726=CARTESIAN_POINT('Ctrl Pts',(54.0526825389488,23.2614408777272,10.8927511816599));
#33727=CARTESIAN_POINT('Ctrl Pts',(53.9782178394031,23.2287935593128,10.8969763346883));
#33728=CARTESIAN_POINT('Ctrl Pts',(53.90548042427,23.1924819607796,10.9012014877168));
#33729=CARTESIAN_POINT('Ctrl Pts',(53.8325561495876,23.1560770791826,10.9054374949967));
#33730=CARTESIAN_POINT('Ctrl Pts',(53.7613684992649,23.1159891961191,10.9096735022765));
#33731=CARTESIAN_POINT('Ctrl Pts',(53.6923095212342,23.0724130528795,10.9139095095564));
#33732=CARTESIAN_POINT('Ctrl Pts',(53.6235514169462,23.0290267606582,10.9181270615477));
#33733=CARTESIAN_POINT('Ctrl Pts',(53.55690387543,22.9821827826933,10.9223446135391));
#33734=CARTESIAN_POINT('Ctrl Pts',(53.4927291157899,22.9321192332805,10.9265621655304));
#33735=CARTESIAN_POINT('Ctrl Pts',(53.428575545196,22.8820722137133,10.930778324982));
#33736=CARTESIAN_POINT('Ctrl Pts',(53.3668935013947,22.8288080194679,10.9349944844336));
#33737=CARTESIAN_POINT('Ctrl Pts',(53.3080142411145,22.7726066799289,10.9392106438852));
#33738=CARTESIAN_POINT('Ctrl Pts',(53.2491363838083,22.7164066795545,10.9434267028742));
#33739=CARTESIAN_POINT('Ctrl Pts',(53.1930615127808,22.6572699948515,10.9476427618633));
#33740=CARTESIAN_POINT('Ctrl Pts',(53.140084890369,22.5955143480916,10.9518588208523));
#33741=CARTESIAN_POINT('Ctrl Pts',(53.0866746203768,22.5332531918152,10.956109390984));
#33742=CARTESIAN_POINT('Ctrl Pts',(53.0364138799446,22.4683303534671,10.9603599611158));
#33743=CARTESIAN_POINT('Ctrl Pts',(52.9895634067052,22.401104904831,10.9646105312476));
#33744=CARTESIAN_POINT('Ctrl Pts',(52.9430257581448,22.3343283263541,10.9688327199534));
#33745=CARTESIAN_POINT('Ctrl Pts',(52.8998531706619,22.2652802242718,10.9730549086592));
#33746=CARTESIAN_POINT('Ctrl Pts',(52.8602562387386,22.1943395187897,10.9772770973651));
#33747=CARTESIAN_POINT('Ctrl Pts',(52.8202600527306,22.1226835213632,10.9815418582098));
#33748=CARTESIAN_POINT('Ctrl Pts',(52.7839122496268,22.0490969752077,10.9858066190546));
#33749=CARTESIAN_POINT('Ctrl Pts',(52.7513803240931,21.9739916853465,10.9900713798993));
#33750=CARTESIAN_POINT('Ctrl Pts',(52.7188483985593,21.8988863954853,10.9943361407441));
#33751=CARTESIAN_POINT('Ctrl Pts',(52.6901324595109,21.8222628356214,10.9986009015888));
#33752=CARTESIAN_POINT('Ctrl Pts',(52.6653480735384,21.7445472666455,11.0028656624336));
#33753=CARTESIAN_POINT('Ctrl Pts',(52.6357253635559,21.6516603271242,11.0079629754672));
#33754=CARTESIAN_POINT('Ctrl Pts',(52.6116270588092,21.5569317973583,11.0130602885009));
#33755=CARTESIAN_POINT('Ctrl Pts',(52.5932460894767,21.4609618901612,11.0181576015345));
#33756=CARTESIAN_POINT('Ctrl Pts',(52.5750889287308,21.3661605224948,11.0231928491567));
#33757=CARTESIAN_POINT('Ctrl Pts',(52.5625107684555,21.2701478592151,11.0282280967789));
#33758=CARTESIAN_POINT('Ctrl Pts',(52.5556514284901,21.1735232288698,11.0332633444011));
#33759=CARTESIAN_POINT('Ctrl Pts',(52.5516058953972,21.1165355096989,11.0362330559169));
#33760=CARTESIAN_POINT('Ctrl Pts',(52.549548756107,21.0593353118622,11.0392027674327));
#33761=CARTESIAN_POINT('Ctrl Pts',(52.5495008566119,21.0020489641339,11.0421724789485));
#33762=CARTESIAN_POINT('',(52.5495290836882,20.9986540030259,11.8421725323987));
#33763=CARTESIAN_POINT('Ctrl Pts',(52.5512711617411,21.0020470050971,11.0421725037879));
#33764=CARTESIAN_POINT('Ctrl Pts',(52.5557259539615,20.4383632669047,11.0714146549061));
#33765=CARTESIAN_POINT('Ctrl Pts',(53.0293753351344,19.0516701821435,11.143001237594));
#33766=CARTESIAN_POINT('Ctrl Pts',(55.3350226443368,18.1229073326861,11.2569322518514));
#33767=CARTESIAN_POINT('Ctrl Pts',(57.5990916197438,19.7214754048292,11.3839655465605));
#33768=CARTESIAN_POINT('Ctrl Pts',(57.4835458207409,22.4906047579764,11.5109988412695));
#33769=CARTESIAN_POINT('Ctrl Pts',(55.094173934607,23.8950014953986,11.6380321359785));
#33770=CARTESIAN_POINT('Ctrl Pts',(52.942897126316,22.812112652436,11.748423356818));
#33771=CARTESIAN_POINT('Ctrl Pts',(52.5552276006745,21.4948623786468,11.8164701460878));
#33772=CARTESIAN_POINT('Ctrl Pts',(52.5527567710893,20.9986563282935,11.8421725037879));
#33773=CARTESIAN_POINT('',(52.5495003638158,20.9986646869211,12.6421725037591));
#33774=CARTESIAN_POINT('Ctrl Pts',(52.5495003696722,20.9986539823399,11.8421725326532));
#33775=CARTESIAN_POINT('Ctrl Pts',(52.5495501121537,20.9080950425036,11.846857062966));
#33776=CARTESIAN_POINT('Ctrl Pts',(52.5546239307066,20.8177144413065,11.8515415932788));
#33777=CARTESIAN_POINT('Ctrl Pts',(52.5646380792273,20.7280394057033,11.8562261235917));
#33778=CARTESIAN_POINT('Ctrl Pts',(52.5746897537974,20.6380283305641,11.8609282082593));
#33779=CARTESIAN_POINT('Ctrl Pts',(52.5897187232734,20.5487283771237,11.865630292927));
#33780=CARTESIAN_POINT('Ctrl Pts',(52.6095903921718,20.4606558085949,11.8703323775946));
#33781=CARTESIAN_POINT('Ctrl Pts',(52.6295615247038,20.3721424105744,11.8750579975994));
#33782=CARTESIAN_POINT('Ctrl Pts',(52.6544238258674,20.2848689666113,11.8797836176042));
#33783=CARTESIAN_POINT('Ctrl Pts',(52.683992309623,20.199338630809,11.884509237609));
#33784=CARTESIAN_POINT('Ctrl Pts',(52.6998216008856,20.153550533983,11.8870390668714));
#33785=CARTESIAN_POINT('Ctrl Pts',(52.7169988381724,20.108261620341,11.8895688961339));
#33786=CARTESIAN_POINT('Ctrl Pts',(52.7354901934547,20.0635462712658,11.8920987253964));
#33787=CARTESIAN_POINT('Ctrl Pts',(52.7664175762218,19.9887584206568,11.8963299457013));
#33788=CARTESIAN_POINT('Ctrl Pts',(52.8011118491665,19.9153641107187,11.9005611660062));
#33789=CARTESIAN_POINT('Ctrl Pts',(52.8394260610957,19.8437688360335,11.9047923863112));
#33790=CARTESIAN_POINT('Ctrl Pts',(52.8776853331266,19.7722762239611,11.9090175393423));
#33791=CARTESIAN_POINT('Ctrl Pts',(52.919554017429,19.7025779301395,11.9132426923735));
#33792=CARTESIAN_POINT('Ctrl Pts',(52.9648370486113,19.635059704128,11.9174678454046));
#33793=CARTESIAN_POINT('Ctrl Pts',(53.0102364100779,19.567368026512,11.9217038526838));
#33794=CARTESIAN_POINT('Ctrl Pts',(53.0590674972057,19.5018680657897,11.925939859963));
#33795=CARTESIAN_POINT('Ctrl Pts',(53.1110872055688,19.4389238631527,11.9301758672422));
#33796=CARTESIAN_POINT('Ctrl Pts',(53.1628802763265,19.376253893567,11.9343934192363));
#33797=CARTESIAN_POINT('Ctrl Pts',(53.217833950369,19.3161178246963,11.9386109712305));
#33798=CARTESIAN_POINT('Ctrl Pts',(53.2756659041834,19.2588445859131,11.9428285232246));
#33799=CARTESIAN_POINT('Ctrl Pts',(53.3334787632022,19.2015902574503,11.9470446826791));
#33800=CARTESIAN_POINT('Ctrl Pts',(53.3941676846644,19.1471972088512,11.9512608421335));
#33801=CARTESIAN_POINT('Ctrl Pts',(53.4574127164301,19.0959583191095,11.9554770015879));
#33802=CARTESIAN_POINT('Ctrl Pts',(53.5206562411948,19.0447206502867,11.9596930605798));
#33803=CARTESIAN_POINT('Ctrl Pts',(53.5864553932218,18.9966372826957,11.9639091195717));
#33804=CARTESIAN_POINT('Ctrl Pts',(53.6544574206571,18.9519605918891,11.9681251785636));
#33805=CARTESIAN_POINT('Ctrl Pts',(53.723016088135,18.9069181938233,11.9723757486921));
#33806=CARTESIAN_POINT('Ctrl Pts',(53.7938134692512,18.8653387784438,11.9766263188205));
#33807=CARTESIAN_POINT('Ctrl Pts',(53.8664601983647,18.8274352096868,11.980876888949));
#33808=CARTESIAN_POINT('Ctrl Pts',(53.9386218590641,18.7897847262952,11.9850990776578));
#33809=CARTESIAN_POINT('Ctrl Pts',(54.0126077940697,18.7557612911305,11.9893212663665));
#33810=CARTESIAN_POINT('Ctrl Pts',(54.0880153397349,18.7255255047723,11.9935434550753));
#33811=CARTESIAN_POINT('Ctrl Pts',(54.1641832161262,18.6949848524064,11.9978082159136));
#33812=CARTESIAN_POINT('Ctrl Pts',(54.2418010731814,18.6683088180263,12.002072976752));
#33813=CARTESIAN_POINT('Ctrl Pts',(54.3204391217192,18.6456110638405,12.0063377375903));
#33814=CARTESIAN_POINT('Ctrl Pts',(54.399077170257,18.6229133096547,12.0106024984287));
#33815=CARTESIAN_POINT('Ctrl Pts',(54.4787349265582,18.6041938833373,12.014867259267));
#33816=CARTESIAN_POINT('Ctrl Pts',(54.5589748794589,18.589513100419,12.0191320201054));
#33817=CARTESIAN_POINT('Ctrl Pts',(54.6385837791951,18.5749477756257,12.0233632404103));
#33818=CARTESIAN_POINT('Ctrl Pts',(54.7190642668798,18.5643031333827,12.0275944607152));
#33819=CARTESIAN_POINT('Ctrl Pts',(54.7999959514765,18.5576755681167,12.0318256810201));
#33820=CARTESIAN_POINT('Ctrl Pts',(54.8808115857021,18.5510575063153,12.0360508340513));
#33821=CARTESIAN_POINT('Ctrl Pts',(54.962076672418,18.5484451189129,12.0402759870824));
#33822=CARTESIAN_POINT('Ctrl Pts',(55.0433613224848,18.5498836669023,12.0445011401136));
#33823=CARTESIAN_POINT('Ctrl Pts',(55.1248547895454,18.5513259104635,12.0487371473928));
#33824=CARTESIAN_POINT('Ctrl Pts',(55.2063674551396,18.5568400080709,12.052973154672));
#33825=CARTESIAN_POINT('Ctrl Pts',(55.2874616224533,18.5664190858703,12.0572091619512));
#33826=CARTESIAN_POINT('Ctrl Pts',(55.3682024815986,18.575956429886,12.0614267139453));
#33827=CARTESIAN_POINT('Ctrl Pts',(55.4485280158544,18.5895233608773,12.0656442659395));
#33828=CARTESIAN_POINT('Ctrl Pts',(55.5280087651534,18.6070610133308,12.0698618179336));
#33829=CARTESIAN_POINT('Ctrl Pts',(55.6074632717172,18.6245928752506,12.0740779773881));
#33830=CARTESIAN_POINT('Ctrl Pts',(55.6860730935931,18.6460927549896,12.0782941368425));
#33831=CARTESIAN_POINT('Ctrl Pts',(55.7634186584541,18.6714506228288,12.0825102962969));
#33832=CARTESIAN_POINT('Ctrl Pts',(55.8407623803269,18.6968078864415,12.0867263552888));
#33833=CARTESIAN_POINT('Ctrl Pts',(55.9168414636413,18.7260228094845,12.0909424142807));
#33834=CARTESIAN_POINT('Ctrl Pts',(55.9912525837727,18.7589358409086,12.0951584732726));
#33835=CARTESIAN_POINT('Ctrl Pts',(56.0662728064653,18.7921182865238,12.0994090434011));
#33836=CARTESIAN_POINT('Ctrl Pts',(56.1395971880355,18.8290594833582,12.1036596135296));
#33837=CARTESIAN_POINT('Ctrl Pts',(56.2108357501217,18.8695476921021,12.1079101836581));
#33838=CARTESIAN_POINT('Ctrl Pts',(56.2815986462453,18.9097655576188,12.1121323723668));
#33839=CARTESIAN_POINT('Ctrl Pts',(56.3503031295201,18.9534829076873,12.1163545610756));
#33840=CARTESIAN_POINT('Ctrl Pts',(56.4165959246362,19.0004484912101,12.1205767497843));
#33841=CARTESIAN_POINT('Ctrl Pts',(56.4835571468785,19.0478876264962,12.1248415106226));
#33842=CARTESIAN_POINT('Ctrl Pts',(56.5480573915711,19.0986405670876,12.129106271461));
#33843=CARTESIAN_POINT('Ctrl Pts',(56.6097681146265,19.1524078190434,12.1333710322993));
#33844=CARTESIAN_POINT('Ctrl Pts',(56.6714788376818,19.2061750709992,12.1376357931377));
#33845=CARTESIAN_POINT('Ctrl Pts',(56.7303997367595,19.2629562537313,12.141900553976));
#33846=CARTESIAN_POINT('Ctrl Pts',(56.7862429045101,19.3224164592822,12.1461653148144));
#33847=CARTESIAN_POINT('Ctrl Pts',(56.8416468894543,19.3814090355599,12.1503965351193));
#33848=CARTESIAN_POINT('Ctrl Pts',(56.8942291722578,19.443259830556,12.1546277554242));
#33849=CARTESIAN_POINT('Ctrl Pts',(56.9436808137138,19.5076678840148,12.1588589757292));
#33850=CARTESIAN_POINT('Ctrl Pts',(56.9930615449771,19.5719835808329,12.1630841287603));
#33851=CARTESIAN_POINT('Ctrl Pts',(57.0393202698788,19.6388488876622,12.1673092817915));
#33852=CARTESIAN_POINT('Ctrl Pts',(57.0821858632528,19.7079271379406,12.1715344348226));
#33853=CARTESIAN_POINT('Ctrl Pts',(57.1251615766104,19.7771828474629,12.1757704421018));
#33854=CARTESIAN_POINT('Ctrl Pts',(57.164726384035,19.8486625364532,12.180006449381));
#33855=CARTESIAN_POINT('Ctrl Pts',(57.2006487324116,19.9219947094122,12.1842424566602));
#33856=CARTESIAN_POINT('Ctrl Pts',(57.2364145755853,19.9950073913825,12.1884600086544));
#33857=CARTESIAN_POINT('Ctrl Pts',(57.2685694190252,20.0698560327421,12.1926775606486));
#33858=CARTESIAN_POINT('Ctrl Pts',(57.296929860991,20.1461478677852,12.1968951126427));
#33859=CARTESIAN_POINT('Ctrl Pts',(57.3252809389841,20.222414513,12.2011112720972));
#33860=CARTESIAN_POINT('Ctrl Pts',(57.3498399415676,20.3001229701735,12.2053274315516));
#33861=CARTESIAN_POINT('Ctrl Pts',(57.3704718183253,20.3788610392792,12.209543591006));
#33862=CARTESIAN_POINT('Ctrl Pts',(57.3911032034673,20.4575972322162,12.2137596499979));
#33863=CARTESIAN_POINT('Ctrl Pts',(57.4078075320624,20.537362538287,12.2179757089898));
#33864=CARTESIAN_POINT('Ctrl Pts',(57.420500173127,20.617731557813,12.2221917679817));
#33865=CARTESIAN_POINT('Ctrl Pts',(57.4332967115683,20.698758449113,12.2264423381102));
#33866=CARTESIAN_POINT('Ctrl Pts',(57.442015492194,20.7803985117083,12.2306929082387));
#33867=CARTESIAN_POINT('Ctrl Pts',(57.446622971078,20.8622092623081,12.2349434783671));
#33868=CARTESIAN_POINT('Ctrl Pts',(57.451199685432,20.9434737555402,12.2391656670759));
#33869=CARTESIAN_POINT('Ctrl Pts',(57.4517198926874,21.0249061944298,12.2433878557847));
#33870=CARTESIAN_POINT('Ctrl Pts',(57.448203149316,21.106073510734,12.2476100444934));
#33871=CARTESIAN_POINT('Ctrl Pts',(57.444650946787,21.1880592332594,12.2518748053317));
#33872=CARTESIAN_POINT('Ctrl Pts',(57.4369799720587,21.2697739729991,12.2561395661701));
#33873=CARTESIAN_POINT('Ctrl Pts',(57.4252637267549,21.3507792834349,12.2604043270084));
#33874=CARTESIAN_POINT('Ctrl Pts',(57.413547481451,21.4317845938708,12.2646690878467));
#33875=CARTESIAN_POINT('Ctrl Pts',(57.3977861214198,21.5120800146024,12.268933848685));
#33876=CARTESIAN_POINT('Ctrl Pts',(57.3781049385212,21.5912420412833,12.2731986095234));
#33877=CARTESIAN_POINT('Ctrl Pts',(57.3585785397706,21.6697814922325,12.2774298298283));
#33878=CARTESIAN_POINT('Ctrl Pts',(57.3351205760353,21.7474998378392,12.2816610501332));
#33879=CARTESIAN_POINT('Ctrl Pts',(57.3078164111831,21.8239743092317,12.2858922704381));
#33880=CARTESIAN_POINT('Ctrl Pts',(57.2805513985923,21.9003391215847,12.2901174234693));
#33881=CARTESIAN_POINT('Ctrl Pts',(57.2494512934621,21.9754631679865,12.2943425765005));
#33882=CARTESIAN_POINT('Ctrl Pts',(57.2146519649609,22.0489360915208,12.2985677295316));
#33883=CARTESIAN_POINT('Ctrl Pts',(57.1797632383856,22.1225977640378,12.3028037368108));
#33884=CARTESIAN_POINT('Ctrl Pts',(57.1411563779152,22.1945993629736,12.30703974409));
#33885=CARTESIAN_POINT('Ctrl Pts',(57.0990179740528,22.2645448962386,12.3112757513692));
#33886=CARTESIAN_POINT('Ctrl Pts',(57.0570631572817,22.3341856933054,12.3154933033634));
#33887=CARTESIAN_POINT('Ctrl Pts',(57.0116077395819,22.4017878979421,12.3197108553575));
#33888=CARTESIAN_POINT('Ctrl Pts',(56.9628822921637,22.466984443377,12.3239284073517));
#33889=CARTESIAN_POINT('Ctrl Pts',(56.9141729327799,22.5321594623956,12.3281445668061));
#33890=CARTESIAN_POINT('Ctrl Pts',(56.8621959658948,22.5949300274527,12.3323607262605));
#33891=CARTESIAN_POINT('Ctrl Pts',(56.807224509266,22.654959160556,12.336576885715));
#33892=CARTESIAN_POINT('Ctrl Pts',(56.7522543624956,22.7149868632868,12.3407929447069));
#33893=CARTESIAN_POINT('Ctrl Pts',(56.6942901826542,22.7722729218149,12.3450090036988));
#33894=CARTESIAN_POINT('Ctrl Pts',(56.6336435168314,22.8265155651991,12.3492250626907));
#33895=CARTESIAN_POINT('Ctrl Pts',(56.5725004193003,22.8812022192763,12.3534756328191));
#33896=CARTESIAN_POINT('Ctrl Pts',(56.5086310642246,22.9327950718666,12.3577262029476));
#33897=CARTESIAN_POINT('Ctrl Pts',(56.4423890534673,22.981026014074,12.3619767730761));
#33898=CARTESIAN_POINT('Ctrl Pts',(56.3765893462725,23.0289349141615,12.3661989617848));
#33899=CARTESIAN_POINT('Ctrl Pts',(56.308448998465,23.0735264573031,12.3704211504936));
#33900=CARTESIAN_POINT('Ctrl Pts',(56.2383424932468,23.1145822564798,12.3746433392023));
#33901=CARTESIAN_POINT('Ctrl Pts',(56.1675291074434,23.156052019343,12.3789081000407));
#33902=CARTESIAN_POINT('Ctrl Pts',(56.0947101227336,23.1939141113333,12.383172860879));
#33903=CARTESIAN_POINT('Ctrl Pts',(56.0202937915758,23.2279925558385,12.3874376217173));
#33904=CARTESIAN_POINT('Ctrl Pts',(55.9458774604181,23.2620710003437,12.3917023825557));
#33905=CARTESIAN_POINT('Ctrl Pts',(55.8698642541614,23.2923656786736,12.395967143394));
#33906=CARTESIAN_POINT('Ctrl Pts',(55.7926779521201,23.3187522321763,12.4002319042323));
#33907=CARTESIAN_POINT('Ctrl Pts',(55.7160986875752,23.344931266638,12.4044631245373));
#33908=CARTESIAN_POINT('Ctrl Pts',(55.6380775643946,23.3673616398872,12.4086943448422));
#33909=CARTESIAN_POINT('Ctrl Pts',(55.5590160940915,23.3858858431507,12.4129255651471));
#33910=CARTESIAN_POINT('Ctrl Pts',(55.4800679924032,23.4043834840032,12.4171507181783));
#33911=CARTESIAN_POINT('Ctrl Pts',(55.4000829552331,23.4189859740579,12.4213758712094));
#33912=CARTESIAN_POINT('Ctrl Pts',(55.3194794502073,23.4295849709148,12.4256010242406));
#33913=CARTESIAN_POINT('Ctrl Pts',(55.2386688780221,23.440211196168,12.4298370315198));
#33914=CARTESIAN_POINT('Ctrl Pts',(55.1572371049882,23.4468131856598,12.434073038799));
#33915=CARTESIAN_POINT('Ctrl Pts',(55.0756180311116,23.4493330037728,12.4383090460782));
#33916=CARTESIAN_POINT('Ctrl Pts',(54.9943545522976,23.4518418436324,12.4425265980723));
#33917=CARTESIAN_POINT('Ctrl Pts',(54.9129058686852,23.450303985438,12.4467441500665));
#33918=CARTESIAN_POINT('Ctrl Pts',(54.8317054235051,23.4447141316568,12.4509617020606));
#33919=CARTESIAN_POINT('Ctrl Pts',(54.7505317888649,23.4391261235182,12.4551778615151));
#33920=CARTESIAN_POINT('Ctrl Pts',(54.6696066933503,23.4294888085328,12.4593940209695));
#33921=CARTESIAN_POINT('Ctrl Pts',(54.5893613682022,23.4158489530753,12.4636101804239));
#33922=CARTESIAN_POINT('Ctrl Pts',(54.5091179551376,23.402209422628,12.4678262394158));
#33923=CARTESIAN_POINT('Ctrl Pts',(54.4295547383962,23.3845676203351,12.4720422984077));
#33924=CARTESIAN_POINT('Ctrl Pts',(54.3510942042322,23.363021692287,12.4762583573996));
#33925=CARTESIAN_POINT('Ctrl Pts',(54.2719914204661,23.3412993970517,12.4805089275281));
#33926=CARTESIAN_POINT('Ctrl Pts',(54.1940099217676,23.3156088770702,12.4847594976566));
#33927=CARTESIAN_POINT('Ctrl Pts',(54.1175667133664,23.286101866637,12.489010067785));
#33928=CARTESIAN_POINT('Ctrl Pts',(54.0416339227954,23.2567918770321,12.4932322564938));
#33929=CARTESIAN_POINT('Ctrl Pts',(53.9672193464176,23.2237164550153,12.4974544452025));
#33930=CARTESIAN_POINT('Ctrl Pts',(53.8947095337005,23.1870718404084,12.5016766339113));
#33931=CARTESIAN_POINT('Ctrl Pts',(53.8214686079623,23.150057739881,12.5059413947496));
#33932=CARTESIAN_POINT('Ctrl Pts',(53.7501714953767,23.1094023062835,12.5102061555879));
#33933=CARTESIAN_POINT('Ctrl Pts',(53.6811874211161,23.06535314941,12.5144709164263));
#33934=CARTESIAN_POINT('Ctrl Pts',(53.6122033468556,23.0213039925365,12.5187356772646));
#33935=CARTESIAN_POINT('Ctrl Pts',(53.5455326662232,22.9738614440747,12.5230004381029));
#33936=CARTESIAN_POINT('Ctrl Pts',(53.4815096521556,22.9233141484176,12.5272651989413));
#33937=CARTESIAN_POINT('Ctrl Pts',(53.4187616329917,22.8737734836619,12.5314450286277));
#33938=CARTESIAN_POINT('Ctrl Pts',(53.3583090111805,22.8210547669303,12.5356248583141));
#33939=CARTESIAN_POINT('Ctrl Pts',(53.3004973656926,22.765401100595,12.5398046880005));
#33940=CARTESIAN_POINT('Ctrl Pts',(53.2415032168275,22.7086090710834,12.5440700136571));
#33941=CARTESIAN_POINT('Ctrl Pts',(53.1852597290091,22.648760927074,12.5483353393137));
#33942=CARTESIAN_POINT('Ctrl Pts',(53.132101510513,22.5861606107114,12.5526006649703));
#33943=CARTESIAN_POINT('Ctrl Pts',(53.0801443795852,22.5249747221433,12.5567696173894));
#33944=CARTESIAN_POINT('Ctrl Pts',(53.0311349011389,22.4611600990071,12.5609385698084));
#33945=CARTESIAN_POINT('Ctrl Pts',(52.9853493218512,22.3950386715194,12.5651075222274));
#33946=CARTESIAN_POINT('Ctrl Pts',(52.9395912881483,22.3289570240981,12.5692739665154));
#33947=CARTESIAN_POINT('Ctrl Pts',(52.8970535765444,22.260571717223,12.5734404108034));
#33948=CARTESIAN_POINT('Ctrl Pts',(52.8579712424293,22.1902365528499,12.5776068550914));
#33949=CARTESIAN_POINT('Ctrl Pts',(52.8188997481619,22.1199208965868,12.5817721437774));
#33950=CARTESIAN_POINT('Ctrl Pts',(52.783281960016,22.0476568737207,12.5859374324635));
#33951=CARTESIAN_POINT('Ctrl Pts',(52.7513079523275,21.9738245862241,12.5901027211495));
#33952=CARTESIAN_POINT('Ctrl Pts',(52.7179993440694,21.8969105263733,12.5944418697003));
#33953=CARTESIAN_POINT('Ctrl Pts',(52.6886456301591,21.8182949040314,12.5987810182511));
#33954=CARTESIAN_POINT('Ctrl Pts',(52.663406240258,21.7384306683331,12.6031201668019));
#33955=CARTESIAN_POINT('Ctrl Pts',(52.6391545882402,21.6616919016508,12.6072895037439));
#33956=CARTESIAN_POINT('Ctrl Pts',(52.6187013072694,21.5838009235815,12.6114588406859));
#33957=CARTESIAN_POINT('Ctrl Pts',(52.6021362891922,21.5051731132901,12.6156281776278));
#33958=CARTESIAN_POINT('Ctrl Pts',(52.5855617474506,21.426500097803,12.6197999116312));
#33959=CARTESIAN_POINT('Ctrl Pts',(52.5728799892526,21.3470898783097,12.6239716456347));
#33960=CARTESIAN_POINT('Ctrl Pts',(52.5641292380657,21.2673646969099,12.6281433796381));
#33961=CARTESIAN_POINT('Ctrl Pts',(52.5553661774599,21.1875273684912,12.6323209818945));
#33962=CARTESIAN_POINT('Ctrl Pts',(52.550545175321,21.1073746695339,12.6364985841508));
#33963=CARTESIAN_POINT('Ctrl Pts',(52.5496524038118,21.0273296149722,12.6406761864072));
#33964=CARTESIAN_POINT('Ctrl Pts',(52.5495458140011,21.0177728727134,12.6411749588579));
#33965=CARTESIAN_POINT('Ctrl Pts',(52.5494951582618,21.0082176587128,12.6416737313085));
#33966=CARTESIAN_POINT('Ctrl Pts',(52.5495003638158,20.9986646869211,12.6421725037591));
#33967=CARTESIAN_POINT('',(52.5495009651831,21.0021749394239,13.4421725037879));
#33968=CARTESIAN_POINT('Ctrl Pts',(52.5495003638161,20.9986646863694,12.6421725037879));
#33969=CARTESIAN_POINT('Ctrl Pts',(52.5495425490658,20.9212484624948,12.6462145004087));
#33970=CARTESIAN_POINT('Ctrl Pts',(52.5532530208526,20.843934384163,12.6502564970295));
#33971=CARTESIAN_POINT('Ctrl Pts',(52.5606047961666,20.7669736291435,12.6542984936503));
#33972=CARTESIAN_POINT('Ctrl Pts',(52.5683007404991,20.6864100018396,12.6585297139552));
#33973=CARTESIAN_POINT('Ctrl Pts',(52.5800064524164,20.6060769848732,12.6627609342602));
#33974=CARTESIAN_POINT('Ctrl Pts',(52.5957000328985,20.5264053228807,12.6669921545651));
#33975=CARTESIAN_POINT('Ctrl Pts',(52.6113711098846,20.4468479044752,12.6712173075962));
#33976=CARTESIAN_POINT('Ctrl Pts',(52.6310186093195,20.3679504098838,12.6754424606274));
#33977=CARTESIAN_POINT('Ctrl Pts',(52.6545688466119,20.2901387778469,12.6796676136585));
#33978=CARTESIAN_POINT('Ctrl Pts',(52.678179583516,20.2121272508595,12.6839036209377));
#33979=CARTESIAN_POINT('Ctrl Pts',(52.7057130846198,20.1352076419053,12.6881396282169));
#33980=CARTESIAN_POINT('Ctrl Pts',(52.7370433772792,20.0597991843845,12.6923756354961));
#33981=CARTESIAN_POINT('Ctrl Pts',(52.7682371712398,19.9847192637351,12.6965931874903));
#33982=CARTESIAN_POINT('Ctrl Pts',(52.8031945703391,19.9111377897203,12.7008107394844));
#33983=CARTESIAN_POINT('Ctrl Pts',(52.8417418269329,19.8394518931172,12.7050282914786));
#33984=CARTESIAN_POINT('Ctrl Pts',(52.8802763560995,19.7677896655664,12.709244450933));
#33985=CARTESIAN_POINT('Ctrl Pts',(52.9223981689301,19.6980221816789,12.7134606103874));
#33986=CARTESIAN_POINT('Ctrl Pts',(52.9678869890961,19.6305231068341,12.7176767698418));
#33987=CARTESIAN_POINT('Ctrl Pts',(53.0133747253557,19.5630256403556,12.7218928288337));
#33988=CARTESIAN_POINT('Ctrl Pts',(53.062229048691,19.4977968603748,12.7261088878256));
#33989=CARTESIAN_POINT('Ctrl Pts',(53.1141864690518,19.4351812959667,12.7303249468175));
#33990=CARTESIAN_POINT('Ctrl Pts',(53.1665691940953,19.3720531831569,12.7345755169459));
#33991=CARTESIAN_POINT('Ctrl Pts',(53.2221057583337,19.3115816444894,12.7388260870744));
#33992=CARTESIAN_POINT('Ctrl Pts',(53.2804861009244,19.2540841369396,12.7430766572029));
#33993=CARTESIAN_POINT('Ctrl Pts',(53.3384766329819,19.1969705451581,12.7472988459116));
#33994=CARTESIAN_POINT('Ctrl Pts',(53.3992726910952,19.1427916559399,12.7515210346204));
#33995=CARTESIAN_POINT('Ctrl Pts',(53.4625362090209,19.091818839463,12.7557432233291));
#33996=CARTESIAN_POINT('Ctrl Pts',(53.5264376100142,19.0403320664816,12.7600079841674));
#33997=CARTESIAN_POINT('Ctrl Pts',(53.5928561163172,18.9921166688931,12.7642727450058));
#33998=CARTESIAN_POINT('Ctrl Pts',(53.6614139914404,18.9474070672224,12.7685375058442));
#33999=CARTESIAN_POINT('Ctrl Pts',(53.7299718665635,18.9026974655518,12.7728022666825));
#34000=CARTESIAN_POINT('Ctrl Pts',(53.8006686618954,18.8614938468948,12.7770670275209));
#34001=CARTESIAN_POINT('Ctrl Pts',(53.8731036507204,18.8239818778374,12.7813317883592));
#34002=CARTESIAN_POINT('Ctrl Pts',(53.9449689691098,18.7867649244912,12.7855630086642));
#34003=CARTESIAN_POINT('Ctrl Pts',(54.0188147040824,18.7530421616621,12.7897942289691));
#34004=CARTESIAN_POINT('Ctrl Pts',(54.0942670546318,18.7230287481669,12.794025449274));
#34005=CARTESIAN_POINT('Ctrl Pts',(54.1696112117913,18.6930583718059,12.7982506023052));
#34006=CARTESIAN_POINT('Ctrl Pts',(54.2465569807047,18.6667869513411,12.8024757553363));
#34007=CARTESIAN_POINT('Ctrl Pts',(54.3247065191816,18.644383527659,12.8067009083675));
#34008=CARTESIAN_POINT('Ctrl Pts',(54.4030568206766,18.6219225504834,12.8109369156467));
#34009=CARTESIAN_POINT('Ctrl Pts',(54.4826166624278,18.6033496803442,12.8151729229259));
#34010=CARTESIAN_POINT('Ctrl Pts',(54.562965484585,18.5887863880743,12.8194089302051));
#34011=CARTESIAN_POINT('Ctrl Pts',(54.642964245867,18.5742865446353,12.8236264821992));
#34012=CARTESIAN_POINT('Ctrl Pts',(54.7237446681765,18.5637615058452,12.8278440341934));
#34013=CARTESIAN_POINT('Ctrl Pts',(54.8048788584204,18.5572806157668,12.8320615861876));
#34014=CARTESIAN_POINT('Ctrl Pts',(54.8859862600005,18.5508018655309,12.836277745642));
#34015=CARTESIAN_POINT('Ctrl Pts',(54.9674467344728,18.5483646493068,12.8404939050965));
#34016=CARTESIAN_POINT('Ctrl Pts',(55.048826876333,18.5499864926602,12.8447100645509));
#34017=CARTESIAN_POINT('Ctrl Pts',(55.1302050790693,18.5516082973683,12.8489261235428));
#34018=CARTESIAN_POINT('Ctrl Pts',(55.2115024881918,18.5572889589791,12.8531421825347));
#34019=CARTESIAN_POINT('Ctrl Pts',(55.2922867481265,18.5669938950201,12.8573582415266));
#34020=CARTESIAN_POINT('Ctrl Pts',(55.3737322788434,18.5767782721632,12.8616088116551));
#34021=CARTESIAN_POINT('Ctrl Pts',(55.4546557424809,18.5906530690653,12.8658593817836));
#34022=CARTESIAN_POINT('Ctrl Pts',(55.5346222786994,18.6085298937435,12.870109951912));
#34023=CARTESIAN_POINT('Ctrl Pts',(55.6140548715271,18.6262873533369,12.8743321406208));
#34024=CARTESIAN_POINT('Ctrl Pts',(55.6925428409481,18.6479933749729,12.8785543293296));
#34025=CARTESIAN_POINT('Ctrl Pts',(55.7696748652404,18.6735110462723,12.8827765180383));
#34026=CARTESIAN_POINT('Ctrl Pts',(55.8475846080949,18.6992860110476,12.8870412788767));
#34027=CARTESIAN_POINT('Ctrl Pts',(55.9241104550958,18.7289497479128,12.891306039715));
#34028=CARTESIAN_POINT('Ctrl Pts',(55.9988506208529,18.762311977236,12.8955708005533));
#34029=CARTESIAN_POINT('Ctrl Pts',(56.0735907866101,18.7956742065591,12.8998355613916));
#34030=CARTESIAN_POINT('Ctrl Pts',(56.1465448706722,18.8327346528485,12.90410032223));
#34031=CARTESIAN_POINT('Ctrl Pts',(56.2173395866305,18.8732572838206,12.9083650830683));
#34032=CARTESIAN_POINT('Ctrl Pts',(56.2875775322036,18.9134612215039,12.9125963033732));
#34033=CARTESIAN_POINT('Ctrl Pts',(56.3559533604273,18.9572238016516,12.9168275236782));
#34034=CARTESIAN_POINT('Ctrl Pts',(56.4220836041848,19.004347607245,12.9210587439831));
#34035=CARTESIAN_POINT('Ctrl Pts',(56.4881190218013,19.0514038405995,12.9252838970142));
#34036=CARTESIAN_POINT('Ctrl Pts',(56.5519148747036,19.1018114594618,12.9295090500454));
#34037=CARTESIAN_POINT('Ctrl Pts',(56.6131134100363,19.1553278404114,12.9337342030766));
#34038=CARTESIAN_POINT('Ctrl Pts',(56.6744691619425,19.2089817027893,12.9379702103558));
#34039=CARTESIAN_POINT('Ctrl Pts',(56.7332138279284,19.2657600802133,12.9422062176349));
#34040=CARTESIAN_POINT('Ctrl Pts',(56.7890173071687,19.3253754675597,12.9464422249141));
#34041=CARTESIAN_POINT('Ctrl Pts',(56.8445776638061,19.3847311247183,12.9506597769083));
#34042=CARTESIAN_POINT('Ctrl Pts',(56.8972220826611,19.4468987869988,12.9548773289025));
#34043=CARTESIAN_POINT('Ctrl Pts',(56.9466602854203,19.5115565233549,12.9590948808966));
#34044=CARTESIAN_POINT('Ctrl Pts',(56.9960821648095,19.5761929111972,12.963311040351));
#34045=CARTESIAN_POINT('Ctrl Pts',(57.0422996481992,19.6433173713685,12.9675271998055));
#34046=CARTESIAN_POINT('Ctrl Pts',(57.0850630080604,19.7125752439781,12.9717433592599));
#34047=CARTESIAN_POINT('Ctrl Pts',(57.1278253489575,19.781831466313,12.9759594182518));
#34048=CARTESIAN_POINT('Ctrl Pts',(57.1671334866555,19.8532206038417,12.9801754772437));
#34049=CARTESIAN_POINT('Ctrl Pts',(57.2027820459374,19.9263606247459,12.9843915362356));
#34050=CARTESIAN_POINT('Ctrl Pts',(57.2387224114536,20.0000993434519,12.9886421063641));
#34051=CARTESIAN_POINT('Ctrl Pts',(57.2709427854333,20.0756173178473,12.9928926764925));
#34052=CARTESIAN_POINT('Ctrl Pts',(57.2992816471748,20.1525012348298,12.997143246621));
#34053=CARTESIAN_POINT('Ctrl Pts',(57.3274312879166,20.2288717913333,13.0013654353298));
#34054=CARTESIAN_POINT('Ctrl Pts',(57.3517510117247,20.3065896384019,13.0055876240385));
#34055=CARTESIAN_POINT('Ctrl Pts',(57.3721328296035,20.385234932094,13.0098098127473));
#34056=CARTESIAN_POINT('Ctrl Pts',(57.3927201563904,20.4646732025724,13.0140745735856));
#34057=CARTESIAN_POINT('Ctrl Pts',(57.4092896207638,20.5450572519506,13.0183393344239));
#34058=CARTESIAN_POINT('Ctrl Pts',(57.4217832455885,20.6259463121602,13.0226040952622));
#34059=CARTESIAN_POINT('Ctrl Pts',(57.4342768704133,20.7068353723697,13.0268688561006));
#34060=CARTESIAN_POINT('Ctrl Pts',(57.442694670034,20.7882289575597,13.0311336169389));
#34061=CARTESIAN_POINT('Ctrl Pts',(57.4470325630816,20.8696854374275,13.0353983777772));
#34062=CARTESIAN_POINT('Ctrl Pts',(57.451336340442,20.9505012966632,13.0396295980822));
#34063=CARTESIAN_POINT('Ctrl Pts',(57.4516403398395,21.0316821126902,13.0438608183871));
#34064=CARTESIAN_POINT('Ctrl Pts',(57.4479025137916,21.1127986390549,13.048092038692));
#34065=CARTESIAN_POINT('Ctrl Pts',(57.4441700475247,21.1937988499981,13.0523171917231));
#34066=CARTESIAN_POINT('Ctrl Pts',(57.4364072877171,21.2747344938583,13.0565423447543));
#34067=CARTESIAN_POINT('Ctrl Pts',(57.4246241137385,21.3551734183153,13.0607674977855));
#34068=CARTESIAN_POINT('Ctrl Pts',(57.4128106692603,21.435818987131,13.0650035050646));
#34069=CARTESIAN_POINT('Ctrl Pts',(57.3969561089172,21.5159648094864,13.0692395123438));
#34070=CARTESIAN_POINT('Ctrl Pts',(57.377123016808,21.5951776314357,13.073475519623));
#34071=CARTESIAN_POINT('Ctrl Pts',(57.3573763328054,21.6740453417949,13.0776930716172));
#34072=CARTESIAN_POINT('Ctrl Pts',(57.3336858174935,21.7519877086711,13.0819106236113));
#34073=CARTESIAN_POINT('Ctrl Pts',(57.3061645734845,21.8285862719143,13.0861281756055));
#34074=CARTESIAN_POINT('Ctrl Pts',(57.2786524163643,21.9051595440545,13.0903443350599));
#34075=CARTESIAN_POINT('Ctrl Pts',(57.2473121993811,21.9803894564804,13.0945604945144));
#34076=CARTESIAN_POINT('Ctrl Pts',(57.2123065126005,22.0538738749516,13.0987766539688));
#34077=CARTESIAN_POINT('Ctrl Pts',(57.1773016599345,22.127356542438,13.1029927129607));
#34078=CARTESIAN_POINT('Ctrl Pts',(57.1386317120743,22.1990933794108,13.1072087719526));
#34079=CARTESIAN_POINT('Ctrl Pts',(57.0965063067393,22.2687046763539,13.1114248309445));
#34080=CARTESIAN_POINT('Ctrl Pts',(57.0540360780468,22.3388857862387,13.1156754010729));
#34081=CARTESIAN_POINT('Ctrl Pts',(57.0080537951447,22.4069059789412,13.1199259712014));
#34082=CARTESIAN_POINT('Ctrl Pts',(56.9588191582693,22.4724054316652,13.1241765413299));
#34083=CARTESIAN_POINT('Ctrl Pts',(56.9099132652687,22.53746753895,13.1283987300386));
#34084=CARTESIAN_POINT('Ctrl Pts',(56.8577986664844,22.6000421449226,13.1326209187474));
#34085=CARTESIAN_POINT('Ctrl Pts',(56.8027695756549,22.6598108648557,13.1368431074561));
#34086=CARTESIAN_POINT('Ctrl Pts',(56.7471856290984,22.7201822299724,13.1411078682945));
#34087=CARTESIAN_POINT('Ctrl Pts',(56.6886284329182,22.7776904669439,13.1453726291328));
#34088=CARTESIAN_POINT('Ctrl Pts',(56.627436899567,22.8320478672589,13.1496373899712));
#34089=CARTESIAN_POINT('Ctrl Pts',(56.5662453662158,22.8864052675738,13.1539021508095));
#34090=CARTESIAN_POINT('Ctrl Pts',(56.5024199117009,22.937611579846,13.1581669116478));
#34091=CARTESIAN_POINT('Ctrl Pts',(56.4363293964162,22.9854239131708,13.1624316724862));
#34092=CARTESIAN_POINT('Ctrl Pts',(56.3707586549759,23.0328602227926,13.1666628927911));
#34093=CARTESIAN_POINT('Ctrl Pts',(56.3027124969757,23.0771336650337,13.170894113096));
#34094=CARTESIAN_POINT('Ctrl Pts',(56.232528791406,23.1179761633114,13.175125333401));
#34095=CARTESIAN_POINT('Ctrl Pts',(56.162445724358,23.1587600963051,13.1793504864321));
#34096=CARTESIAN_POINT('Ctrl Pts',(56.0902315956899,23.1961226244261,13.1835756394633));
#34097=CARTESIAN_POINT('Ctrl Pts',(56.0162548718767,23.2298377262453,13.1878007924944));
#34098=CARTESIAN_POINT('Ctrl Pts',(55.9420881048381,23.2636394408038,13.1920367997736));
#34099=CARTESIAN_POINT('Ctrl Pts',(55.8661500611846,23.2937746934287,13.1962728070528));
#34100=CARTESIAN_POINT('Ctrl Pts',(55.7888387106711,23.320061149743,13.200508814332));
#34101=CARTESIAN_POINT('Ctrl Pts',(55.711864187485,23.3462330821644,13.2047263663262));
#34102=CARTESIAN_POINT('Ctrl Pts',(55.6335287391667,23.3685895265775,13.2089439183203));
#34103=CARTESIAN_POINT('Ctrl Pts',(55.5542452974421,23.3869986175663,13.2131614703145));
#34104=CARTESIAN_POINT('Ctrl Pts',(55.4749880333063,23.405401630292,13.2173776297689));
#34105=CARTESIAN_POINT('Ctrl Pts',(55.3947838498681,23.4198597727448,13.2215937892234));
#34106=CARTESIAN_POINT('Ctrl Pts',(55.3140587944245,23.430291612882,13.2258099486778));
#34107=CARTESIAN_POINT('Ctrl Pts',(55.2333356624953,23.4407232044496,13.2300260076697));
#34108=CARTESIAN_POINT('Ctrl Pts',(55.1520921444674,23.4471286259672,13.2342420666616));
#34109=CARTESIAN_POINT('Ctrl Pts',(55.0707609558563,23.4494781356702,13.2384581256535));
#34110=CARTESIAN_POINT('Ctrl Pts',(54.9887640195022,23.4518468776113,13.242708695782));
#34111=CARTESIAN_POINT('Ctrl Pts',(54.9066784497142,23.4500929708947,13.2469592659104));
#34112=CARTESIAN_POINT('Ctrl Pts',(54.8249473974727,23.4442395210675,13.2512098360389));
#34113=CARTESIAN_POINT('Ctrl Pts',(54.7437620704464,23.4384251552247,13.2554320247477));
#34114=CARTESIAN_POINT('Ctrl Pts',(54.6629269996648,23.4285659437547,13.2596542134564));
#34115=CARTESIAN_POINT('Ctrl Pts',(54.5828692323513,23.4147364602956,13.2638764021652));
#34116=CARTESIAN_POINT('Ctrl Pts',(54.5020042463466,23.4007675348072,13.2681411630035));
#34117=CARTESIAN_POINT('Ctrl Pts',(54.4219328010098,23.3827479292142,13.2724059238418));
#34118=CARTESIAN_POINT('Ctrl Pts',(54.3430804049416,23.3608064079099,13.2766706846802));
#34119=CARTESIAN_POINT('Ctrl Pts',(54.2642280088733,23.3388648866055,13.2809354455185));
#34120=CARTESIAN_POINT('Ctrl Pts',(54.1865950988654,23.3130016628266,13.2852002063568));
#34121=CARTESIAN_POINT('Ctrl Pts',(54.1105857646076,23.2833949653709,13.2894649671952));
#34122=CARTESIAN_POINT('Ctrl Pts',(54.0351742114943,23.2540211120213,13.2936961875001));
#34123=CARTESIAN_POINT('Ctrl Pts',(53.9610779865151,23.2208523503577,13.297927407805));
#34124=CARTESIAN_POINT('Ctrl Pts',(53.8887055370419,23.1840272128796,13.30215862811));
#34125=CARTESIAN_POINT('Ctrl Pts',(53.8164368645958,23.1472548800712,13.3063837811411));
#34126=CARTESIAN_POINT('Ctrl Pts',(53.7458874693976,23.1068367934756,13.3106089341723));
#34127=CARTESIAN_POINT('Ctrl Pts',(53.6774470532155,23.0629599979039,13.3148340872034));
#34128=CARTESIAN_POINT('Ctrl Pts',(53.6088308163596,23.0189704846107,13.3190700944826));
#34129=CARTESIAN_POINT('Ctrl Pts',(53.5423348456485,22.9715046463281,13.3233061017618));
#34130=CARTESIAN_POINT('Ctrl Pts',(53.4783281327667,22.92079800564,13.327542109041));
#34131=CARTESIAN_POINT('Ctrl Pts',(53.4146002820429,22.870312281831,13.3317596610352));
#34132=CARTESIAN_POINT('Ctrl Pts',(53.3533404159781,22.8166142196711,13.3359772130293));
#34133=CARTESIAN_POINT('Ctrl Pts',(53.2948832331578,22.7599792786943,13.3401947650235));
#34134=CARTESIAN_POINT('Ctrl Pts',(53.2364453515694,22.7033630372866,13.3444109244779));
#34135=CARTESIAN_POINT('Ctrl Pts',(53.1808086491966,22.643812165981,13.3486270839323));
#34136=CARTESIAN_POINT('Ctrl Pts',(53.12827256027,22.5816404905546,13.3528432433868));
#34137=CARTESIAN_POINT('Ctrl Pts',(53.075737723172,22.5194702965533,13.3570593023787));
#34138=CARTESIAN_POINT('Ctrl Pts',(53.0263036518553,22.4546797784244,13.3612753613706));
#34139=CARTESIAN_POINT('Ctrl Pts',(52.980229964204,22.3876163924157,13.3654914203625));
#34140=CARTESIAN_POINT('Ctrl Pts',(52.9337791339819,22.3200040497443,13.3697419904909));
#34141=CARTESIAN_POINT('Ctrl Pts',(52.8907442400028,22.2500818439982,13.3739925606194));
#34142=CARTESIAN_POINT('Ctrl Pts',(52.8513461543074,22.1782346546382,13.3782431307479));
#34143=CARTESIAN_POINT('Ctrl Pts',(52.8122111329946,22.106867195097,13.3824653194566));
#34144=CARTESIAN_POINT('Ctrl Pts',(52.7766646506345,22.0336008296154,13.3866875081654));
#34145=CARTESIAN_POINT('Ctrl Pts',(52.7448756021483,21.9588348138308,13.3909096968741));
#34146=CARTESIAN_POINT('Ctrl Pts',(52.7127660261858,21.8833149358359,13.3951744577125));
#34147=CARTESIAN_POINT('Ctrl Pts',(52.6844902500044,21.8062654515716,13.3994392185508));
#34148=CARTESIAN_POINT('Ctrl Pts',(52.6601708012614,21.7281137072808,13.4037039793891));
#34149=CARTESIAN_POINT('Ctrl Pts',(52.6358513525184,21.6499619629899,13.4079687402275));
#34150=CARTESIAN_POINT('Ctrl Pts',(52.6154882888828,21.5707084413021,13.4122335010658));
#34151=CARTESIAN_POINT('Ctrl Pts',(52.5991509624684,21.4907893122141,13.4164982619042));
#34152=CARTESIAN_POINT('Ctrl Pts',(52.5760578947605,21.3778223669276,13.4225265683907));
#34153=CARTESIAN_POINT('Ctrl Pts',(52.5609317705013,21.263175741453,13.4285548748773));
#34154=CARTESIAN_POINT('Ctrl Pts',(52.5539600038609,21.1477788458736,13.4345831813639));
#34155=CARTESIAN_POINT('Ctrl Pts',(52.5510343073978,21.0993526281496,13.4371129555053));
#34156=CARTESIAN_POINT('Ctrl Pts',(52.5495441175164,21.0507945698908,13.4396427296466));
#34157=CARTESIAN_POINT('Ctrl Pts',(52.5495009651831,21.0021749394239,13.4421725037879));
#34158=CARTESIAN_POINT('',(52.5499009846874,21.000004473486,14.2421725034846));
#34159=CARTESIAN_POINT('Ctrl Pts',(52.5487175127731,21.0021682154797,13.4421728897047));
#34160=CARTESIAN_POINT('Ctrl Pts',(52.5547032669598,20.3526186542018,13.4759591120076));
#34161=CARTESIAN_POINT('Ctrl Pts',(53.1534784602604,18.8792388521044,13.55208976588));
#34162=CARTESIAN_POINT('Ctrl Pts',(55.640566724473,18.1751855530352,13.6705648513222));
#34163=CARTESIAN_POINT('Ctrl Pts',(57.720838282277,20.0065507411148,13.7975981460311));
#34164=CARTESIAN_POINT('Ctrl Pts',(57.3100291386536,22.7474746827509,13.92463144074));
#34165=CARTESIAN_POINT('Ctrl Pts',(54.7842582038357,23.8884871240272,14.0516647354491));
#34166=CARTESIAN_POINT('Ctrl Pts',(52.844309899764,22.6356866765821,14.1575117554562));
#34167=CARTESIAN_POINT('Ctrl Pts',(52.5534943172644,21.4087914667217,14.2210143438937));
#34168=CARTESIAN_POINT('Ctrl Pts',(52.5535009435967,21.0000045195322,14.2421725007616));
#34169=CARTESIAN_POINT('',(52.5495009672036,20.9978227852975,15.042172503748));
#34170=CARTESIAN_POINT('Ctrl Pts',(52.5495000000041,21.0000044683571,14.2421725037879));
#34171=CARTESIAN_POINT('Ctrl Pts',(52.5494998442032,20.9145614302854,14.2465876779589));
#34172=CARTESIAN_POINT('Ctrl Pts',(52.5539727787239,20.8292041264636,14.2510028521299));
#34173=CARTESIAN_POINT('Ctrl Pts',(52.5628662413919,20.7444040441387,14.2554180263009));
#34174=CARTESIAN_POINT('Ctrl Pts',(52.5717838644767,20.6593735897509,14.2598451949506));
#34175=CARTESIAN_POINT('Ctrl Pts',(52.5851459765392,20.5749037787846,14.2642723636003));
#34176=CARTESIAN_POINT('Ctrl Pts',(52.6028484141931,20.4914584336917,14.26869953225));
#34177=CARTESIAN_POINT('Ctrl Pts',(52.6205754493165,20.4078971416102,14.2731328524336));
#34178=CARTESIAN_POINT('Ctrl Pts',(52.6426547332348,20.3253635372867,14.2775661726172));
#34179=CARTESIAN_POINT('Ctrl Pts',(52.6689322213934,20.244306105925,14.2819994928009));
#34180=CARTESIAN_POINT('Ctrl Pts',(52.6952815016257,20.1630272195658,14.2864449251486));
#34181=CARTESIAN_POINT('Ctrl Pts',(52.7258517765444,20.0832329417358,14.2908903574964));
#34182=CARTESIAN_POINT('Ctrl Pts',(52.7604405008871,20.0053525750633,14.2953357898441));
#34183=CARTESIAN_POINT('Ctrl Pts',(52.7874021300513,19.9446454629827,14.2988009681851));
#34184=CARTESIAN_POINT('Ctrl Pts',(52.8168044190187,19.8851008470814,14.302266146526));
#34185=CARTESIAN_POINT('Ctrl Pts',(52.8485328046591,19.8269104222729,14.305731324867));
#34186=CARTESIAN_POINT('Ctrl Pts',(52.8872753386224,19.7558559244161,14.3099625451719));
#34187=CARTESIAN_POINT('Ctrl Pts',(52.9296142697847,19.6865895385243,14.3141937654769));
#34188=CARTESIAN_POINT('Ctrl Pts',(52.975360155001,19.6194987330529,14.3184249857818));
#34189=CARTESIAN_POINT('Ctrl Pts',(53.0210404438198,19.5525041311008,14.322650138813));
#34190=CARTESIAN_POINT('Ctrl Pts',(53.0701177243472,19.4876792946342,14.3268752918441));
#34191=CARTESIAN_POINT('Ctrl Pts',(53.1223568248339,19.425386918398,14.3311004448753));
#34192=CARTESIAN_POINT('Ctrl Pts',(53.1747301254667,19.3629345155549,14.3353364521545));
#34193=CARTESIAN_POINT('Ctrl Pts',(53.2302812804322,19.3030280125131,14.3395724594337));
#34194=CARTESIAN_POINT('Ctrl Pts',(53.2887296739244,19.2460033862367,14.3438084667129));
#34195=CARTESIAN_POINT('Ctrl Pts',(53.3469234215458,19.1892272028129,14.348026018707));
#34196=CARTESIAN_POINT('Ctrl Pts',(53.4079888859932,19.1353081697927,14.3522435707012));
#34197=CARTESIAN_POINT('Ctrl Pts',(53.4716102092135,19.0845431622144,14.3564611226953));
#34198=CARTESIAN_POINT('Ctrl Pts',(53.5352105261203,19.0337949160866,14.3606772821498));
#34199=CARTESIAN_POINT('Ctrl Pts',(53.6013646628347,18.9861989170979,14.3648934416042));
#34200=CARTESIAN_POINT('Ctrl Pts',(53.6697232007087,18.9420121751411,14.3691096010587));
#34201=CARTESIAN_POINT('Ctrl Pts',(53.7380801097372,18.8978264860649,14.3733256600506));
#34202=CARTESIAN_POINT('Ctrl Pts',(53.8086409244351,18.8570501439591,14.3775417190424));
#34203=CARTESIAN_POINT('Ctrl Pts',(53.8810279426985,18.8198963820546,14.3817577780343));
#34204=CARTESIAN_POINT('Ctrl Pts',(53.9540074949562,18.7824384928706,14.3860083481628));
#34205=CARTESIAN_POINT('Ctrl Pts',(54.0288428666092,18.7486629972304,14.3902589182913));
#34206=CARTESIAN_POINT('Ctrl Pts',(54.1051241738747,18.7187399302542,14.3945094884198));
#34207=CARTESIAN_POINT('Ctrl Pts',(54.1808961443376,18.6890166621515,14.3987316771285));
#34208=CARTESIAN_POINT('Ctrl Pts',(54.2580943351833,18.6630946242449,14.4029538658373));
#34209=CARTESIAN_POINT('Ctrl Pts',(54.3363012259363,18.6410904664853,14.4071760545461));
#34210=CARTESIAN_POINT('Ctrl Pts',(54.4152966730796,18.618864441841,14.4114408153844));
#34211=CARTESIAN_POINT('Ctrl Pts',(54.4953208023052,18.600635857537,14.4157055762227));
#34212=CARTESIAN_POINT('Ctrl Pts',(54.5759341390416,18.5864717951576,14.4199703370611));
#34213=CARTESIAN_POINT('Ctrl Pts',(54.656547475778,18.5723077327782,14.4242350978994));
#34214=CARTESIAN_POINT('Ctrl Pts',(54.7377495339812,18.5622081880313,14.4284998587377));
#34215=CARTESIAN_POINT('Ctrl Pts',(54.819098862249,18.5561863760998,14.4327646195761));
#34216=CARTESIAN_POINT('Ctrl Pts',(54.8998084125864,18.5502119231625,14.436995839881));
#34217=CARTESIAN_POINT('Ctrl Pts',(54.9809655730983,18.5482288437161,14.4412270601859));
#34218=CARTESIAN_POINT('Ctrl Pts',(55.0621420588733,18.5502880547871,14.4454582804909));
#34219=CARTESIAN_POINT('Ctrl Pts',(55.1432021432495,18.5523443130934,14.449683433522));
#34220=CARTESIAN_POINT('Ctrl Pts',(55.2242810370014,18.5584313382175,14.4539085865532));
#34221=CARTESIAN_POINT('Ctrl Pts',(55.3049464759174,18.5685481915478,14.4581337395843));
#34222=CARTESIAN_POINT('Ctrl Pts',(55.3858191410986,18.578691034667,14.4623697468635));
#34223=CARTESIAN_POINT('Ctrl Pts',(55.4662757532284,18.5928844658689,14.4666057541427));
#34224=CARTESIAN_POINT('Ctrl Pts',(55.5458818565599,18.6110748758744,14.4708417614219));
#34225=CARTESIAN_POINT('Ctrl Pts',(55.625141134867,18.6291860345519,14.4750593134161));
#34226=CARTESIAN_POINT('Ctrl Pts',(55.703556841916,18.6512593206239,14.4792768654102));
#34227=CARTESIAN_POINT('Ctrl Pts',(55.7807082676652,18.6771903111104,14.4834944174044));
#34228=CARTESIAN_POINT('Ctrl Pts',(55.8578342197686,18.7031127397738,14.4877105768588));
#34229=CARTESIAN_POINT('Ctrl Pts',(55.9336962791937,18.7328901954063,14.4919267363133));
#34230=CARTESIAN_POINT('Ctrl Pts',(56.0078890347163,18.7663684404767,14.4961428957677));
#34231=CARTESIAN_POINT('Ctrl Pts',(56.0820800223759,18.7998458878283,14.5003589547596));
#34232=CARTESIAN_POINT('Ctrl Pts',(56.1546013618978,18.8370237570559,14.5045750137515));
#34233=CARTESIAN_POINT('Ctrl Pts',(56.2250690888506,18.8777003092064,14.5087910727434));
#34234=CARTESIAN_POINT('Ctrl Pts',(56.2961136391718,18.9187098249253,14.5130416428718));
#34235=CARTESIAN_POINT('Ctrl Pts',(56.3650703779875,18.9632753399351,14.5172922130003));
#34236=CARTESIAN_POINT('Ctrl Pts',(56.4315741878375,19.0111446521385,14.5215427831288));
#34237=CARTESIAN_POINT('Ctrl Pts',(56.4976339460701,19.0586943368565,14.5257649718375));
#34238=CARTESIAN_POINT('Ctrl Pts',(56.5612731040727,19.1095034924075,14.5299871605463));
#34239=CARTESIAN_POINT('Ctrl Pts',(56.6221672597112,19.1632845534702,14.534209349255));
#34240=CARTESIAN_POINT('Ctrl Pts',(56.6836754082485,19.2176078864346,14.5384741100934));
#34241=CARTESIAN_POINT('Ctrl Pts',(56.7423825399049,19.2749630539153,14.5427388709317));
#34242=CARTESIAN_POINT('Ctrl Pts',(56.7979939976509,19.335017166932,14.54700363177));
#34243=CARTESIAN_POINT('Ctrl Pts',(56.853605455397,19.3950712799487,14.5512683926084));
#34244=CARTESIAN_POINT('Ctrl Pts',(56.9061209792954,19.457823927783,14.5555331534467));
#34245=CARTESIAN_POINT('Ctrl Pts',(56.9552901008918,19.5229113529125,14.559797914285));
#34246=CARTESIAN_POINT('Ctrl Pts',(57.0040725282214,19.5874868930761,14.56402913459));
#34247=CARTESIAN_POINT('Ctrl Pts',(57.0497439663743,19.6546027410072,14.5682603548949));
#34248=CARTESIAN_POINT('Ctrl Pts',(57.0920294076324,19.723926644898,14.5724915751998));
#34249=CARTESIAN_POINT('Ctrl Pts',(57.1342542145273,19.7931511431626,14.576716728231));
#34250=CARTESIAN_POINT('Ctrl Pts',(57.1731024274221,19.8645770155185,14.5809418812621));
#34251=CARTESIAN_POINT('Ctrl Pts',(57.2083404518764,19.9378405493494,14.5851670342933));
#34252=CARTESIAN_POINT('Ctrl Pts',(57.2436690013968,20.0112922942491,14.5894030415725));
#34253=CARTESIAN_POINT('Ctrl Pts',(57.275368510485,20.0865907739699,14.5936390488517));
#34254=CARTESIAN_POINT('Ctrl Pts',(57.3032484521605,20.1633418753037,14.5978750561309));
#34255=CARTESIAN_POINT('Ctrl Pts',(57.331006927503,20.2397585901838,14.602092608125));
#34256=CARTESIAN_POINT('Ctrl Pts',(57.3549788805052,20.3176148586486,14.6063101601192));
#34257=CARTESIAN_POINT('Ctrl Pts',(57.3750239328768,20.39650056482,14.6105277121133));
#34258=CARTESIAN_POINT('Ctrl Pts',(57.395062366828,20.4753602247257,14.6147438715678));
#34259=CARTESIAN_POINT('Ctrl Pts',(57.4111763605519,20.5552481971022,14.6189600310222));
#34260=CARTESIAN_POINT('Ctrl Pts',(57.4232756870592,20.6357402101413,14.6231761904766));
#34261=CARTESIAN_POINT('Ctrl Pts',(57.435374725264,20.7162303052188,14.6273922494685));
#34262=CARTESIAN_POINT('Ctrl Pts',(57.4434592184389,20.7973239524205,14.6316083084604));
#34263=CARTESIAN_POINT('Ctrl Pts',(57.4474904808888,20.8785891439837,14.6358243674523));
#34264=CARTESIAN_POINT('Ctrl Pts',(57.4515547417975,20.9605195430618,14.6400749375808));
#34265=CARTESIAN_POINT('Ctrl Pts',(57.4514990693311,21.0426238295319,14.6443255077092));
#34266=CARTESIAN_POINT('Ctrl Pts',(57.4473373979528,21.1244584693046,14.6485760778377));
#34267=CARTESIAN_POINT('Ctrl Pts',(57.4432035144096,21.2057466921993,14.6527982665465));
#34268=CARTESIAN_POINT('Ctrl Pts',(57.4350184058769,21.2867683974232,14.6570204552552));
#34269=CARTESIAN_POINT('Ctrl Pts',(57.4228477969882,21.367095086632,14.661242643964));
#34270=CARTESIAN_POINT('Ctrl Pts',(57.4105544724242,21.4482317060588,14.6655074048023));
#34271=CARTESIAN_POINT('Ctrl Pts',(57.3941949207406,21.5286587389069,14.6697721656406));
#34272=CARTESIAN_POINT('Ctrl Pts',(57.3738890775575,21.6079481042435,14.674036926479));
#34273=CARTESIAN_POINT('Ctrl Pts',(57.3535832343744,21.6872374695801,14.6783016873173));
#34274=CARTESIAN_POINT('Ctrl Pts',(57.3293313038483,21.7653887262961,14.6825664481556));
#34275=CARTESIAN_POINT('Ctrl Pts',(57.3013031184507,21.8419941846647,14.686831208994));
#34276=CARTESIAN_POINT('Ctrl Pts',(57.273495362832,21.9179971736258,14.6910624292989));
#34277=CARTESIAN_POINT('Ctrl Pts',(57.2418663045063,21.9927636097845,14.6952936496038));
#34278=CARTESIAN_POINT('Ctrl Pts',(57.2065459980047,22.0658822677432,14.6995248699087));
#34279=CARTESIAN_POINT('Ctrl Pts',(57.1712763383506,22.138896078664,14.7037500229399));
#34280=CARTESIAN_POINT('Ctrl Pts',(57.1323261433176,22.2102663889744,14.7079751759711));
#34281=CARTESIAN_POINT('Ctrl Pts',(57.0898743571043,22.2795997114401,14.7122003290022));
#34282=CARTESIAN_POINT('Ctrl Pts',(57.0473135139614,22.34911114842,14.7164363362814));
#34283=CARTESIAN_POINT('Ctrl Pts',(57.0012332339305,22.4165746772112,14.7206723435606));
#34284=CARTESIAN_POINT('Ctrl Pts',(56.9518613569798,22.4816165135179,14.7249083508398));
#34285=CARTESIAN_POINT('Ctrl Pts',(56.9027045816571,22.5463749778781,14.729125902834));
#34286=CARTESIAN_POINT('Ctrl Pts',(56.8502851073941,22.6087324296222,14.7333434548281));
#34287=CARTESIAN_POINT('Ctrl Pts',(56.7948714118838,22.6683485441605,14.7375610068223));
#34288=CARTESIAN_POINT('Ctrl Pts',(56.7394760127151,22.7279449748139,14.7417771662767));
#34289=CARTESIAN_POINT('Ctrl Pts',(56.6810886718463,22.7848015254518,14.7459933257312));
#34290=CARTESIAN_POINT('Ctrl Pts',(56.6200169544138,22.8386123347274,14.7502094851856));
#34291=CARTESIAN_POINT('Ctrl Pts',(56.5589466921968,22.8924218618003,14.7544255441775));
#34292=CARTESIAN_POINT('Ctrl Pts',(56.4951925301558,22.9431854852801,14.7586416031694));
#34293=CARTESIAN_POINT('Ctrl Pts',(56.4290964802649,22.9906364560347,14.7628576621613));
#34294=CARTESIAN_POINT('Ctrl Pts',(56.3624593919755,23.0384758433024,14.7671082322898));
#34295=CARTESIAN_POINT('Ctrl Pts',(56.2934422795059,23.0829478023613,14.7713588024182));
#34296=CARTESIAN_POINT('Ctrl Pts',(56.2224253714566,23.1238235475715,14.7756093725467));
#34297=CARTESIAN_POINT('Ctrl Pts',(56.1518826493667,23.1644263619404,14.7798315612555));
#34298=CARTESIAN_POINT('Ctrl Pts',(56.079367202195,23.2014806820742,14.7840537499642));
#34299=CARTESIAN_POINT('Ctrl Pts',(56.0052747067387,23.2348093909753,14.788275938673));
#34300=CARTESIAN_POINT('Ctrl Pts',(55.9304351401459,23.2684741516761,14.7925406995113));
#34301=CARTESIAN_POINT('Ctrl Pts',(55.8539869961572,23.2983375711843,14.7968054603496));
#34302=CARTESIAN_POINT('Ctrl Pts',(55.7763549952266,23.3242683088204,14.801070221188));
#34303=CARTESIAN_POINT('Ctrl Pts',(55.6987229942959,23.3501990464565,14.8053349820263));
#34304=CARTESIAN_POINT('Ctrl Pts',(55.6199076177568,23.3721970345811,14.8095997428646));
#34305=CARTESIAN_POINT('Ctrl Pts',(55.540343507813,23.3901839141715,14.813864503703));
#34306=CARTESIAN_POINT('Ctrl Pts',(55.4614051358154,23.4080293345902,14.8180957240079));
#34307=CARTESIAN_POINT('Ctrl Pts',(55.3814337654475,23.4219934753772,14.8223269443128));
#34308=CARTESIAN_POINT('Ctrl Pts',(55.300845441241,23.4319626375593,14.8265581646177));
#34309=CARTESIAN_POINT('Ctrl Pts',(55.2203726750507,23.4419175046607,14.8307833176489));
#34310=CARTESIAN_POINT('Ctrl Pts',(55.1392851695522,23.4478887138307,14.8350084706801));
#34311=CARTESIAN_POINT('Ctrl Pts',(55.0580105740899,23.4498132629435,14.8392336237112));
#34312=CARTESIAN_POINT('Ctrl Pts',(54.976527187464,23.4517427561454,14.8434696309904));
#34313=CARTESIAN_POINT('Ctrl Pts',(54.8948562102012,23.4496046734464,14.8477056382696));
#34314=CARTESIAN_POINT('Ctrl Pts',(54.8134352488942,23.4433877800392,14.8519416455488));
#34315=CARTESIAN_POINT('Ctrl Pts',(54.73236901952,23.4371979721709,14.856159197543));
#34316=CARTESIAN_POINT('Ctrl Pts',(54.6515510992603,23.4269648477751,14.8603767495371));
#34317=CARTESIAN_POINT('Ctrl Pts',(54.5714130153411,23.4127294598817,14.8645943015313));
#34318=CARTESIAN_POINT('Ctrl Pts',(54.491301391194,23.3984987721895,14.8688104609857));
#34319=CARTESIAN_POINT('Ctrl Pts',(54.4118696150248,23.3802685264764,14.8730266204402));
#34320=CARTESIAN_POINT('Ctrl Pts',(54.3335414508891,23.3581313051476,14.8772427798946));
#34321=CARTESIAN_POINT('Ctrl Pts',(54.2552151531549,23.3359946113039,14.8814588388865));
#34322=CARTESIAN_POINT('Ctrl Pts',(54.1779928622648,23.309951254453,14.8856748978784));
#34323=CARTESIAN_POINT('Ctrl Pts',(54.1022841566359,23.2801439679488,14.8898909568703));
#34324=CARTESIAN_POINT('Ctrl Pts',(54.0259557268796,23.25009268976,14.8941415269988));
#34325=CARTESIAN_POINT('Ctrl Pts',(53.9511662283322,23.2162157379607,14.8983920971272));
#34326=CARTESIAN_POINT('Ctrl Pts',(53.8783140630311,23.1787085415002,14.9026426672557));
#34327=CARTESIAN_POINT('Ctrl Pts',(53.8059483378588,23.1414517837935,14.9068648559645));
#34328=CARTESIAN_POINT('Ctrl Pts',(53.7354945284408,23.1006134016322,14.9110870446732));
#34329=CARTESIAN_POINT('Ctrl Pts',(53.6673159993428,23.0564298199531,14.915309233382));
#34330=CARTESIAN_POINT('Ctrl Pts',(53.5984500293521,23.0118007373042,14.9195739942203));
#34331=CARTESIAN_POINT('Ctrl Pts',(53.5319058748999,22.963758900825,14.9238387550586));
#34332=CARTESIAN_POINT('Ctrl Pts',(53.4680241857756,22.9125899598794,14.928103515897));
#34333=CARTESIAN_POINT('Ctrl Pts',(53.4041424966514,22.8614210189338,14.9323682767353));
#34334=CARTESIAN_POINT('Ctrl Pts',(53.3429235906776,22.8071253412798,14.9366330375736));
#34335=CARTESIAN_POINT('Ctrl Pts',(53.284668980371,22.7500256406975,14.940897798412));
#34336=CARTESIAN_POINT('Ctrl Pts',(53.227028795328,22.6935281842705,14.945117577801));
#34337=CARTESIAN_POINT('Ctrl Pts',(53.1720584083385,22.6340576330772,14.94933735719));
#34338=CARTESIAN_POINT('Ctrl Pts',(53.1200859364908,22.5719011940387,14.953557136579));
#34339=CARTESIAN_POINT('Ctrl Pts',(53.0688039783508,22.5105705743552,14.9577208513744));
#34340=CARTESIAN_POINT('Ctrl Pts',(53.0204411034233,22.4466253580654,14.9618845661698));
#34341=CARTESIAN_POINT('Ctrl Pts',(52.9752778230292,22.3803805113383,14.9660482809652));
#34342=CARTESIAN_POINT('Ctrl Pts',(52.9301575445797,22.3141987392418,14.9702080313048));
#34343=CARTESIAN_POINT('Ctrl Pts',(52.8882310864795,22.2457220735526,14.9743677816443));
#34344=CARTESIAN_POINT('Ctrl Pts',(52.84973859012,22.1752983107198,14.9785275319838));
#34345=CARTESIAN_POINT('Ctrl Pts',(52.8112701534318,22.1049185661438,14.9826846822783));
#34346=CARTESIAN_POINT('Ctrl Pts',(52.7762316482358,22.0325945592949,14.9868418325727));
#34347=CARTESIAN_POINT('Ctrl Pts',(52.7448188932777,21.9587014268702,14.9909989828672));
#34348=CARTESIAN_POINT('Ctrl Pts',(52.712595271367,21.8829008686501,14.9952634429406));
#34349=CARTESIAN_POINT('Ctrl Pts',(52.6841874401857,21.8054495065769,14.999527903014));
#34350=CARTESIAN_POINT('Ctrl Pts',(52.6597549449292,21.7267759848928,15.0037923630874));
#34351=CARTESIAN_POINT('Ctrl Pts',(52.6359347509933,21.6500740956888,15.0079499517788));
#34352=CARTESIAN_POINT('Ctrl Pts',(52.6158930621347,21.5722110794703,15.0121075404701));
#34353=CARTESIAN_POINT('Ctrl Pts',(52.5997270895804,21.4935992357224,15.0162651291615));
#34354=CARTESIAN_POINT('Ctrl Pts',(52.5829377942457,21.4119562997928,15.0205830249259));
#34355=CARTESIAN_POINT('Ctrl Pts',(52.5703292912183,21.3295061650706,15.0249009206903));
#34356=CARTESIAN_POINT('Ctrl Pts',(52.5619516542964,21.2467195047255,15.0292188164548));
#34357=CARTESIAN_POINT('Ctrl Pts',(52.5535740173746,21.1639328443803,15.0335367122192));
#34358=CARTESIAN_POINT('Ctrl Pts',(52.5494272346723,21.0808102355086,15.0378546079836));
#34359=CARTESIAN_POINT('Ctrl Pts',(52.5495009672036,20.9978227852975,15.042172503748));
#34360=CARTESIAN_POINT('',(52.5495003595367,21.0013274370615,15.8421725038163));
#34361=CARTESIAN_POINT('Ctrl Pts',(52.5495009672043,20.9978227845304,15.0421725037879));
#34362=CARTESIAN_POINT('Ctrl Pts',(52.5496037390909,20.8821509953396,15.0481909888401));
#34363=CARTESIAN_POINT('Ctrl Pts',(52.5579001031268,20.7668303186539,15.0542094738923));
#34364=CARTESIAN_POINT('Ctrl Pts',(52.5742215619191,20.6527980136261,15.0602279589445));
#34365=CARTESIAN_POINT('Ctrl Pts',(52.5811849082287,20.6041475565505,15.0627956703366));
#34366=CARTESIAN_POINT('Ctrl Pts',(52.5896084284055,20.5557312073288,15.0653633817288));
#34367=CARTESIAN_POINT('Ctrl Pts',(52.5994766191758,20.5076203211785,15.0679310931209));
#34368=CARTESIAN_POINT('Ctrl Pts',(52.6157379830066,20.4283404772714,15.0721623134258));
#34369=CARTESIAN_POINT('Ctrl Pts',(52.6359615079926,20.3497184298317,15.0763935337307));
#34370=CARTESIAN_POINT('Ctrl Pts',(52.6600793886806,20.2721801165656,15.0806247540357));
#34371=CARTESIAN_POINT('Ctrl Pts',(52.6841626860156,20.1947529878137,15.0848499070668));
#34372=CARTESIAN_POINT('Ctrl Pts',(52.7121291114251,20.1184069470735,15.089075060098));
#34373=CARTESIAN_POINT('Ctrl Pts',(52.7438598840222,20.0435576195735,15.0933002131291));
#34374=CARTESIAN_POINT('Ctrl Pts',(52.7756721716968,19.9685160071644,15.0975362204083));
#34375=CARTESIAN_POINT('Ctrl Pts',(52.8112680710964,19.8949792689268,15.1017722276875));
#34376=CARTESIAN_POINT('Ctrl Pts',(52.8504775292819,19.8233507753465,15.1060082349667));
#34377=CARTESIAN_POINT('Ctrl Pts',(52.889516161102,19.7520343502256,15.1102257869609));
#34378=CARTESIAN_POINT('Ctrl Pts',(52.9321367130421,19.6826099912273,15.114443338955));
#34379=CARTESIAN_POINT('Ctrl Pts',(52.9781239927611,19.6154539872754,15.1186608909492));
#34380=CARTESIAN_POINT('Ctrl Pts',(53.0240960885265,19.5483201567083,15.1228770504036));
#34381=CARTESIAN_POINT('Ctrl Pts',(53.0734324420786,19.4834535771597,15.1270932098581));
#34382=CARTESIAN_POINT('Ctrl Pts',(53.1258741064872,19.4212022342096,15.1313093693125));
#34383=CARTESIAN_POINT('Ctrl Pts',(53.1783145213172,19.3589523745828,15.1355254283044));
#34384=CARTESIAN_POINT('Ctrl Pts',(53.2338597995003,19.2993179825095,15.1397414872963));
#34385=CARTESIAN_POINT('Ctrl Pts',(53.2922111415219,19.2426134560496,15.1439575462882));
#34386=CARTESIAN_POINT('Ctrl Pts',(53.3510401265597,19.185444766811,15.1482081164167));
#34387=CARTESIAN_POINT('Ctrl Pts',(53.4127209934834,19.1312544760597,15.1524586865452));
#34388=CARTESIAN_POINT('Ctrl Pts',(53.4769115317551,19.0803250879643,15.1567092566737));
#34389=CARTESIAN_POINT('Ctrl Pts',(53.5406734643213,19.0297357597422,15.1609314453824));
#34390=CARTESIAN_POINT('Ctrl Pts',(53.6069112378669,18.9823641429786,15.1651536340912));
#34391=CARTESIAN_POINT('Ctrl Pts',(53.6752597219263,18.9384439261448,15.1693758228));
#34392=CARTESIAN_POINT('Ctrl Pts',(53.7442973605264,18.8940808638365,15.1736405836383));
#34393=CARTESIAN_POINT('Ctrl Pts',(53.8154880922254,18.8532394355534,15.1779053444766));
#34394=CARTESIAN_POINT('Ctrl Pts',(53.8884312921365,18.8161123523178,15.182170105315));
#34395=CARTESIAN_POINT('Ctrl Pts',(53.9613744920476,18.7789852690823,15.1864348661533));
#34396=CARTESIAN_POINT('Ctrl Pts',(54.0360696941342,18.7455726689773,15.1906996269916));
#34397=CARTESIAN_POINT('Ctrl Pts',(54.1120986250629,18.7160163314102,15.19496438783));
#34398=CARTESIAN_POINT('Ctrl Pts',(54.1875296207276,18.6866924418901,15.1991956081349));
#34399=CARTESIAN_POINT('Ctrl Pts',(54.2645562828332,18.6610543719289,15.2034268284398));
#34400=CARTESIAN_POINT('Ctrl Pts',(54.3427839578555,18.639276101712,15.2076580487448));
#34401=CARTESIAN_POINT('Ctrl Pts',(54.4208994598669,18.6175290600104,15.2118832017759));
#34402=CARTESIAN_POINT('Ctrl Pts',(54.5002121103291,18.5996309493965,15.2161083548071));
#34403=CARTESIAN_POINT('Ctrl Pts',(54.580308280633,18.5857073270428,15.2203335078382));
#34404=CARTESIAN_POINT('Ctrl Pts',(54.660610214774,18.5717479354638,15.2245695151174));
#34405=CARTESIAN_POINT('Ctrl Pts',(54.7416992573065,18.5617836439258,15.2288055223966));
#34406=CARTESIAN_POINT('Ctrl Pts',(54.8231442756635,18.5558902842202,15.2330415296758));
#34407=CARTESIAN_POINT('Ctrl Pts',(54.9042344572768,18.5500226004934,15.2372590816699));
#34408=CARTESIAN_POINT('Ctrl Pts',(54.9856770533162,18.5481904923178,15.2414766336641));
#34409=CARTESIAN_POINT('Ctrl Pts',(55.0670392105314,18.5504171795485,15.2456941856582));
#34410=CARTESIAN_POINT('Ctrl Pts',(55.1483745038132,18.5526431315777,15.2499103451127));
#34411=CARTESIAN_POINT('Ctrl Pts',(55.2296289466304,18.5589252050102,15.2541265045671));
#34412=CARTESIAN_POINT('Ctrl Pts',(55.3103697425097,18.5692345088564,15.2583426640215));
#34413=CARTESIAN_POINT('Ctrl Pts',(55.3911086144995,18.5795435670528,15.2625587230134));
#34414=CARTESIAN_POINT('Ctrl Pts',(55.4713334028487,18.5938796048835,15.2667747820053));
#34415=CARTESIAN_POINT('Ctrl Pts',(55.5506179235651,18.6121620339209,15.2709908409972));
#34416=CARTESIAN_POINT('Ctrl Pts',(55.6305514387403,18.6305941163211,15.2752414111256));
#34417=CARTESIAN_POINT('Ctrl Pts',(55.7095287507911,18.6530374034561,15.2794919812541));
#34418=CARTESIAN_POINT('Ctrl Pts',(55.7871269356959,18.6793575378568,15.2837425513826));
#34419=CARTESIAN_POINT('Ctrl Pts',(55.8642069908936,18.7055019304726,15.2879647400913));
#34420=CARTESIAN_POINT('Ctrl Pts',(55.9399258661526,18.7354713256712,15.2921869288001));
#34421=CARTESIAN_POINT('Ctrl Pts',(56.0138892264417,18.7690856389127,15.2964091175088));
#34422=CARTESIAN_POINT('Ctrl Pts',(56.0885983558037,18.803038883689,15.3006738783472));
#34423=CARTESIAN_POINT('Ctrl Pts',(56.1615159377876,18.8407107403156,15.3049386391855));
#34424=CARTESIAN_POINT('Ctrl Pts',(56.2322628222139,18.8818690817163,15.3092034000238));
#34425=CARTESIAN_POINT('Ctrl Pts',(56.3030097066402,18.9230274231169,15.3134681608622));
#34426=CARTESIAN_POINT('Ctrl Pts',(56.3715855247913,18.9676719325829,15.3177329217005));
#34427=CARTESIAN_POINT('Ctrl Pts',(56.4376443516593,19.0155280379551,15.3219976825388));
#34428=CARTESIAN_POINT('Ctrl Pts',(56.5031836538988,19.0630077753757,15.3262289028438));
#34429=CARTESIAN_POINT('Ctrl Pts',(56.5664912053607,19.113826780033,15.3304601231487));
#34430=CARTESIAN_POINT('Ctrl Pts',(56.6272068319805,19.1677477859323,15.3346913434536));
#34431=CARTESIAN_POINT('Ctrl Pts',(56.6878353966413,19.2215914728832,15.3389164964848));
#34432=CARTESIAN_POINT('Ctrl Pts',(56.7458790732919,19.278528020792,15.3431416495159));
#34433=CARTESIAN_POINT('Ctrl Pts',(56.8010080858906,19.3382779641117,15.3473668025471));
#34434=CARTESIAN_POINT('Ctrl Pts',(56.8562787227033,19.3981814026304,15.3516028098263));
#34435=CARTESIAN_POINT('Ctrl Pts',(56.9086193225069,19.460912427944,15.3558388171055));
#34436=CARTESIAN_POINT('Ctrl Pts',(56.9577323992554,19.5261499048731,15.3600748243847));
#34437=CARTESIAN_POINT('Ctrl Pts',(57.0066315019075,19.5911031574955,15.3642923763788));
#34438=CARTESIAN_POINT('Ctrl Pts',(57.0523308580345,19.6585406983729,15.368509928373));
#34439=CARTESIAN_POINT('Ctrl Pts',(57.0945762550086,19.728111419206,15.3727274803671));
#34440=CARTESIAN_POINT('Ctrl Pts',(57.1368077035136,19.7976591693698,15.3769436398216));
#34441=CARTESIAN_POINT('Ctrl Pts',(57.1755872164572,19.8693383037118,15.381159799276));
#34442=CARTESIAN_POINT('Ctrl Pts',(57.2107043973718,19.9427695060011,15.3853759587305));
#34443=CARTESIAN_POINT('Ctrl Pts',(57.2458207415151,20.0161989585736,15.3895920177224));
#34444=CARTESIAN_POINT('Ctrl Pts',(57.2772747275535,20.0913799761822,15.3938080767143));
#34445=CARTESIAN_POINT('Ctrl Pts',(57.3049029824672,20.1679107671566,15.3980241357062));
#34446=CARTESIAN_POINT('Ctrl Pts',(57.3327573922996,20.2450680115523,15.4022747058346));
#34447=CARTESIAN_POINT('Ctrl Pts',(57.3567229718169,20.3235967830605,15.4065252759631));
#34448=CARTESIAN_POINT('Ctrl Pts',(57.3766832942771,20.403068874405,15.4107758460916));
#34449=CARTESIAN_POINT('Ctrl Pts',(57.3965103399598,20.4820103238091,15.4149980348003));
#34450=CARTESIAN_POINT('Ctrl Pts',(57.4123854216895,20.5618820616089,15.4192202235091));
#34451=CARTESIAN_POINT('Ctrl Pts',(57.4242460358015,20.6422551077925,15.4234424122179));
#34452=CARTESIAN_POINT('Ctrl Pts',(57.4362262399262,20.7234385516095,15.4277071730562));
#34453=CARTESIAN_POINT('Ctrl Pts',(57.444110518731,20.8051329864981,15.4319719338945));
#34454=CARTESIAN_POINT('Ctrl Pts',(57.4478883300894,20.8868939726969,15.4362366947329));
#34455=CARTESIAN_POINT('Ctrl Pts',(57.4516661414477,20.9686549588957,15.4405014555712));
#34456=CARTESIAN_POINT('Ctrl Pts',(57.4513375515427,21.0504820148687,15.4447662164095));
#34457=CARTESIAN_POINT('Ctrl Pts',(57.446945697521,21.1319356031678,15.4490309772479));
#34458=CARTESIAN_POINT('Ctrl Pts',(57.4425883835667,21.2127485935758,15.4532621975528));
#34459=CARTESIAN_POINT('Ctrl Pts',(57.4342151951589,21.2934970116553,15.4574934178577));
#34460=CARTESIAN_POINT('Ctrl Pts',(57.421830197336,21.3737495756141,15.4617246381627));
#34461=CARTESIAN_POINT('Ctrl Pts',(57.4094629587331,21.4538870630131,15.4659497911938));
#34462=CARTESIAN_POINT('Ctrl Pts',(57.3930954062288,21.5335296528248,15.470174944225));
#34463=CARTESIAN_POINT('Ctrl Pts',(57.37278354489,21.612248723232,15.4744000972561));
#34464=CARTESIAN_POINT('Ctrl Pts',(57.3524195031971,21.691170019762,15.4786361045353));
#34465=CARTESIAN_POINT('Ctrl Pts',(57.3280908930137,21.7691625748633,15.4828721118145));
#34466=CARTESIAN_POINT('Ctrl Pts',(57.2999062400462,21.8458023037308,15.4871081190937));
#34467=CARTESIAN_POINT('Ctrl Pts',(57.271844380967,21.9221081313682,15.4913256710879));
#34468=CARTESIAN_POINT('Ctrl Pts',(57.2399601625843,21.9970724541366,15.495543223082));
#34469=CARTESIAN_POINT('Ctrl Pts',(57.2044107588722,22.0702912950073,15.4997607750762));
#34470=CARTESIAN_POINT('Ctrl Pts',(57.1688730927645,22.1434859606825,15.5039769345306));
#34471=CARTESIAN_POINT('Ctrl Pts',(57.1296728474387,22.2149358710432,15.5081930939851));
#34472=CARTESIAN_POINT('Ctrl Pts',(57.08701465625,22.284258569992,15.5124092534395));
#34473=CARTESIAN_POINT('Ctrl Pts',(57.0443574815196,22.3535796171212,15.5166253124314));
#34474=CARTESIAN_POINT('Ctrl Pts',(56.998242769351,22.4207731582393,15.5208413714233));
#34475=CARTESIAN_POINT('Ctrl Pts',(56.9489195348987,22.4854840613384,15.5250574304152));
#34476=CARTESIAN_POINT('Ctrl Pts',(56.8991925582587,22.5507246645245,15.5293080005437));
#34477=CARTESIAN_POINT('Ctrl Pts',(56.8462045673086,22.6134414068766,15.5335585706721));
#34478=CARTESIAN_POINT('Ctrl Pts',(56.7902522278264,22.6733042791921,15.5378091408006));
#34479=CARTESIAN_POINT('Ctrl Pts',(56.7346734868929,22.7327674419971,15.5420313295094));
#34480=CARTESIAN_POINT('Ctrl Pts',(56.6761702435895,22.7894144475848,15.5462535182181));
#34481=CARTESIAN_POINT('Ctrl Pts',(56.6150690512437,22.8429601758353,15.5504757069269));
#34482=CARTESIAN_POINT('Ctrl Pts',(56.5533517784577,22.8970458031379,15.5547404677652));
#34483=CARTESIAN_POINT('Ctrl Pts',(56.4889842527477,22.9479669596254,15.5590052286035));
#34484=CARTESIAN_POINT('Ctrl Pts',(56.4223341919505,22.9954738024861,15.5632699894419));
#34485=CARTESIAN_POINT('Ctrl Pts',(56.3556841311534,23.0429806453468,15.5675347502802));
#34486=CARTESIAN_POINT('Ctrl Pts',(56.2867519757585,23.087072969091,15.5717995111185));
#34487=CARTESIAN_POINT('Ctrl Pts',(56.2159304305799,23.1275486922724,15.5760642719569));
#34488=CARTESIAN_POINT('Ctrl Pts',(56.145665866787,23.1677060910748,15.5802954922618));
#34489=CARTESIAN_POINT('Ctrl Pts',(56.0732780641252,23.2044541975874,15.5845267125667));
#34490=CARTESIAN_POINT('Ctrl Pts',(55.999131604964,23.2375625769936,15.5887579328716));
#34491=CARTESIAN_POINT('Ctrl Pts',(55.9250914666357,23.2706234813009,15.5929830859028));
#34492=CARTESIAN_POINT('Ctrl Pts',(55.8492981012134,23.3000548360924,15.597208238934));
#34493=CARTESIAN_POINT('Ctrl Pts',(55.7721420190791,23.325671290697,15.6014333919651));
#34494=CARTESIAN_POINT('Ctrl Pts',(55.6947877260761,23.3513535529422,15.6056693992443));
#34495=CARTESIAN_POINT('Ctrl Pts',(55.6160641188624,23.3732010606255,15.6099054065235));
#34496=CARTESIAN_POINT('Ctrl Pts',(55.5363863735001,23.391075052842,15.6141414138027));
#34497=CARTESIAN_POINT('Ctrl Pts',(55.4570557652895,23.4088711722884,15.6183589657969));
#34498=CARTESIAN_POINT('Ctrl Pts',(55.3767797702377,23.4227282170112,15.622576517791));
#34499=CARTESIAN_POINT('Ctrl Pts',(55.2959830472944,23.4325592049762,15.6267940697852));
#34500=CARTESIAN_POINT('Ctrl Pts',(55.215213001591,23.4423869469725,15.6310102292396));
#34501=CARTESIAN_POINT('Ctrl Pts',(55.1339230305855,23.4481912159273,15.6352263886941));
#34502=CARTESIAN_POINT('Ctrl Pts',(55.0525454440931,23.449936575976,15.6394425481485));
#34503=CARTESIAN_POINT('Ctrl Pts',(54.9711697966636,23.4516818944363,15.6436586071404));
#34504=CARTESIAN_POINT('Ctrl Pts',(54.8897070027367,23.4493684874252,15.6478746661323));
#34505=CARTESIAN_POINT('Ctrl Pts',(54.8085904782411,23.4430130259538,15.6520907251242));
#34506=CARTESIAN_POINT('Ctrl Pts',(54.7268099631656,23.4366055409697,15.6563412952527));
#34507=CARTESIAN_POINT('Ctrl Pts',(54.6453818920659,23.4260895439576,15.6605918653811));
#34508=CARTESIAN_POINT('Ctrl Pts',(54.5647444090101,23.4115353658016,15.6648424355096));
#34509=CARTESIAN_POINT('Ctrl Pts',(54.4846453493145,23.397078367136,15.6690646242184));
#34510=CARTESIAN_POINT('Ctrl Pts',(54.4053267954773,23.3786371161955,15.6732868129271));
#34511=CARTESIAN_POINT('Ctrl Pts',(54.3272053798535,23.3563313962815,15.6775090016359));
#34512=CARTESIAN_POINT('Ctrl Pts',(54.2482962696811,23.3338007688459,15.6817737624742));
#34513=CARTESIAN_POINT('Ctrl Pts',(54.1706090348107,23.3073274599816,15.6860385233125));
#34514=CARTESIAN_POINT('Ctrl Pts',(54.0945529866508,23.2770849689937,15.6903032841509));
#34515=CARTESIAN_POINT('Ctrl Pts',(54.018496938491,23.2468424780058,15.6945680449892));
#34516=CARTESIAN_POINT('Ctrl Pts',(53.9440724885446,23.212831063588,15.6988328058275));
#34517=CARTESIAN_POINT('Ctrl Pts',(53.8716623659161,23.1752711172426,15.7030975666659));
#34518=CARTESIAN_POINT('Ctrl Pts',(53.7998217181607,23.1380065639293,15.7073287869708));
#34519=CARTESIAN_POINT('Ctrl Pts',(53.7296944118989,23.0971093974879,15.7115600072757));
#34520=CARTESIAN_POINT('Ctrl Pts',(53.6616717511369,23.0527610061317,15.7157912275807));
#34521=CARTESIAN_POINT('Ctrl Pts',(53.5937466301093,23.0084762072647,15.7200163806118));
#34522=CARTESIAN_POINT('Ctrl Pts',(53.527920546952,22.9607502639732,15.724241533643));
#34523=CARTESIAN_POINT('Ctrl Pts',(53.4645609831116,22.9098107957116,15.7284666866741));
#34524=CARTESIAN_POINT('Ctrl Pts',(53.4010386511023,22.8587404660069,15.7327026939533));
#34525=CARTESIAN_POINT('Ctrl Pts',(53.3399959434504,22.8044403024048,15.7369387012325));
#34526=CARTESIAN_POINT('Ctrl Pts',(53.281774569503,22.7471839113251,15.7411747085117));
#34527=CARTESIAN_POINT('Ctrl Pts',(53.2238068523557,22.6901769728428,15.7453922605059));
#34528=CARTESIAN_POINT('Ctrl Pts',(53.1686362757324,22.630239834564,15.7496098125));
#34529=CARTESIAN_POINT('Ctrl Pts',(53.1165661843707,22.5676821464009,15.7538273644942));
#34530=CARTESIAN_POINT('Ctrl Pts',(53.0645132853686,22.5051451133632,15.7580435239486));
#34531=CARTESIAN_POINT('Ctrl Pts',(53.0155591358799,22.4399896057526,15.7622596834031));
#34532=CARTESIAN_POINT('Ctrl Pts',(52.9699679181935,22.3725596514674,15.7664758428575));
#34533=CARTESIAN_POINT('Ctrl Pts',(52.9243777868535,22.3051313039015,15.7706919018494));
#34534=CARTESIAN_POINT('Ctrl Pts',(52.8821506874837,22.235429003185,15.7749079608413));
#34535=CARTESIAN_POINT('Ctrl Pts',(52.843507620092,22.1638259600982,15.7791240198332));
#34536=CARTESIAN_POINT('Ctrl Pts',(52.8045482345037,22.0916368003549,15.7833745899616));
#34537=CARTESIAN_POINT('Ctrl Pts',(52.7692320688656,22.0175160515675,15.7876251600901));
#34538=CARTESIAN_POINT('Ctrl Pts',(52.7377375999625,21.9418699928209,15.7918757302186));
#34539=CARTESIAN_POINT('Ctrl Pts',(52.7064534223177,21.8667290292682,15.7960979189273));
#34540=CARTESIAN_POINT('Ctrl Pts',(52.6789401616835,21.7900835257579,15.8003201076361));
#34541=CARTESIAN_POINT('Ctrl Pts',(52.6553230790539,21.7123485006532,15.8045422963448));
#34542=CARTESIAN_POINT('Ctrl Pts',(52.6314678664943,21.6338296769573,15.8088070571832));
#34543=CARTESIAN_POINT('Ctrl Pts',(52.6115879618003,21.5541997081427,15.8130718180215));
#34544=CARTESIAN_POINT('Ctrl Pts',(52.5957595223028,21.4738965872448,15.8173365788598));
#34545=CARTESIAN_POINT('Ctrl Pts',(52.5799310828053,21.3935934663469,15.8216013396982));
#34546=CARTESIAN_POINT('Ctrl Pts',(52.5681541142666,21.3126176793944,15.8258661005365));
#34547=CARTESIAN_POINT('Ctrl Pts',(52.5604509600289,21.2314103100038,15.8301308613749));
#34548=CARTESIAN_POINT('Ctrl Pts',(52.5532009537332,21.1549800684201,15.8341447421792));
#34549=CARTESIAN_POINT('Ctrl Pts',(52.549542003553,21.0782038541672,15.8381586229836));
#34550=CARTESIAN_POINT('Ctrl Pts',(52.549500359537,21.0013274376061,15.8421725037879));
#34551=CARTESIAN_POINT('',(52.5495245738618,21.0013531866909,16.6421724750583));
#34552=CARTESIAN_POINT('Ctrl Pts',(52.5495003595367,21.0013274370615,15.8421725038163));
#34553=CARTESIAN_POINT('Ctrl Pts',(52.549457014999,20.921311761013,15.8463502920186));
#34554=CARTESIAN_POINT('Ctrl Pts',(52.5533370002312,20.8411382049865,15.8505280802208));
#34555=CARTESIAN_POINT('Ctrl Pts',(52.5611603672117,20.7612291987261,15.854705868423));
#34556=CARTESIAN_POINT('Ctrl Pts',(52.569154716791,20.6795737513753,15.8589749637422));
#34557=CARTESIAN_POINT('Ctrl Pts',(52.5812669392635,20.5981950523709,15.8632440590614));
#34558=CARTESIAN_POINT('Ctrl Pts',(52.5974621330943,20.5175458072683,15.8675131543806));
#34559=CARTESIAN_POINT('Ctrl Pts',(52.6132746688864,20.4388021325641,15.8716813800431));
#34560=CARTESIAN_POINT('Ctrl Pts',(52.6329792633433,20.3607543185169,15.8758496057055));
#34561=CARTESIAN_POINT('Ctrl Pts',(52.6564910916385,20.2838182867246,15.880017831368));
#34562=CARTESIAN_POINT('Ctrl Pts',(52.6799915393678,20.2069194947233,15.8841840394602));
#34563=CARTESIAN_POINT('Ctrl Pts',(52.707295425388,20.1311318729757,15.8883502475524));
#34564=CARTESIAN_POINT('Ctrl Pts',(52.7382674978157,20.056858261679,15.8925164556445));
#34565=CARTESIAN_POINT('Ctrl Pts',(52.7692346193451,19.9825965230491,15.8966819977667));
#34566=CARTESIAN_POINT('Ctrl Pts',(52.8038685787417,19.909848754533,15.9008475398888));
#34567=CARTESIAN_POINT('Ctrl Pts',(52.8419857912841,19.8389983096565,15.9050130820109));
#34568=CARTESIAN_POINT('Ctrl Pts',(52.8817535957394,19.7650798237683,15.9093590048503));
#34569=CARTESIAN_POINT('Ctrl Pts',(52.9253129412092,19.6932272251965,15.9137049276897));
#34570=CARTESIAN_POINT('Ctrl Pts',(52.9724028570058,19.6238459113451,15.9180508505291));
#34571=CARTESIAN_POINT('Ctrl Pts',(53.0175954337311,19.5572600978753,15.9222216681668));
#34572=CARTESIAN_POINT('Ctrl Pts',(53.0660391913371,19.4929506050044,15.9263924858045));
#34573=CARTESIAN_POINT('Ctrl Pts',(53.1174612432284,19.4312431420858,15.9305633034422));
#34574=CARTESIAN_POINT('Ctrl Pts',(53.1689180539389,19.3694939679078,15.9347369403509));
#34575=CARTESIAN_POINT('Ctrl Pts',(53.2233568382817,19.3103506702542,15.9389105772595));
#34576=CARTESIAN_POINT('Ctrl Pts',(53.28046768838,19.2541022712384,15.9430842141681));
#34577=CARTESIAN_POINT('Ctrl Pts',(53.3376669344287,19.1977668111707,15.9472643110157));
#34578=CARTESIAN_POINT('Ctrl Pts',(53.3975461352792,19.1443354966691,15.9514444078632));
#34579=CARTESIAN_POINT('Ctrl Pts',(53.4597629127033,19.0940566732151,15.9556245047107));
#34580=CARTESIAN_POINT('Ctrl Pts',(53.4674016628953,19.0878836216973,15.9561377218351));
#34581=CARTESIAN_POINT('Ctrl Pts',(53.4750756158463,19.0817580361128,15.9566509389594));
#34582=CARTESIAN_POINT('Ctrl Pts',(53.4827841103334,19.0756803295338,15.9571641560838));
#34583=CARTESIAN_POINT('Ctrl Pts',(53.5463368190137,19.0255726572375,15.9613953763887));
#34584=CARTESIAN_POINT('Ctrl Pts',(53.6124936397374,18.978522764802,15.9656265966936));
#34585=CARTESIAN_POINT('Ctrl Pts',(53.6809280800406,18.934812473412,15.9698578169986));
#34586=CARTESIAN_POINT('Ctrl Pts',(53.7492643901463,18.8911648595205,15.9740829700297));
#34587=CARTESIAN_POINT('Ctrl Pts',(53.8198714449031,18.8508475839993,15.9783081230609));
#34588=CARTESIAN_POINT('Ctrl Pts',(53.8923904411771,18.8141017143508,15.982533276092));
#34589=CARTESIAN_POINT('Ctrl Pts',(53.9650957358331,18.7772614460425,15.9867692833712));
#34590=CARTESIAN_POINT('Ctrl Pts',(54.0397224333459,18.7440112438922,15.9910052906504));
#34591=CARTESIAN_POINT('Ctrl Pts',(54.1158804456856,18.7145497459627,15.9952412979296));
#34592=CARTESIAN_POINT('Ctrl Pts',(54.1917066555205,18.6852166048339,15.9994588499238));
#34593=CARTESIAN_POINT('Ctrl Pts',(54.269050431445,18.6596394002223,16.0036764019179));
#34594=CARTESIAN_POINT('Ctrl Pts',(54.3475046489063,18.6379669632283,16.0078939539121));
#34595=CARTESIAN_POINT('Ctrl Pts',(54.4259329625698,18.6163016819799,16.0121101133665));
#34596=CARTESIAN_POINT('Ctrl Pts',(54.505470541884,18.5985387317467,16.0163262728209));
#34597=CARTESIAN_POINT('Ctrl Pts',(54.5856950720646,18.5847770958588,16.0205424322754));
#34598=CARTESIAN_POINT('Ctrl Pts',(54.6659176906573,18.5710157878827,16.0247584912673));
#34599=CARTESIAN_POINT('Ctrl Pts',(54.746826769155,18.5612556821962,16.0289745502592));
#34600=CARTESIAN_POINT('Ctrl Pts',(54.8279911923932,18.5555443918726,16.033190609251));
#34601=CARTESIAN_POINT('Ctrl Pts',(54.9098199982933,18.5497863509885,16.0374411793795));
#34602=CARTESIAN_POINT('Ctrl Pts',(54.9919078711413,18.5481437653839,16.041691749508));
#34603=CARTESIAN_POINT('Ctrl Pts',(55.0738110835159,18.5506118776416,16.0459423196365));
#34604=CARTESIAN_POINT('Ctrl Pts',(55.1551674211474,18.5530635101031,16.0501645083452));
#34605=CARTESIAN_POINT('Ctrl Pts',(55.2363410937179,18.5595710135019,16.054386697054));
#34606=CARTESIAN_POINT('Ctrl Pts',(55.3169023351057,18.5700775403308,16.0586088857627));
#34607=CARTESIAN_POINT('Ctrl Pts',(55.3982758716903,18.5806900039742,16.0628736466011));
#34608=CARTESIAN_POINT('Ctrl Pts',(55.4790240793993,18.5953825019187,16.0671384074394));
#34609=CARTESIAN_POINT('Ctrl Pts',(55.5587164881322,18.6140439786347,16.0714031682777));
#34610=CARTESIAN_POINT('Ctrl Pts',(55.6384088968652,18.6327054553507,16.0756679291161));
#34611=CARTESIAN_POINT('Ctrl Pts',(55.7170450613846,18.6553357158492,16.0799326899544));
#34612=CARTESIAN_POINT('Ctrl Pts',(55.7942138663665,18.6817733966518,16.0841974507928));
#34613=CARTESIAN_POINT('Ctrl Pts',(55.870775771459,18.708003156319,16.0884286710977));
#34614=CARTESIAN_POINT('Ctrl Pts',(55.9461804281699,18.7380789780496,16.0926598914026));
#34615=CARTESIAN_POINT('Ctrl Pts',(56.0200140090283,18.7718793409274,16.0968911117075));
#34616=CARTESIAN_POINT('Ctrl Pts',(56.0937417176992,18.8056312364505,16.1011162647387));
#34617=CARTESIAN_POINT('Ctrl Pts',(56.1659024056086,18.8430968741381,16.1053414177699));
#34618=CARTESIAN_POINT('Ctrl Pts',(56.2360989684194,18.8841054869695,16.109566570801));
#34619=CARTESIAN_POINT('Ctrl Pts',(56.3064758633741,18.9252194492764,16.1138025780802));
#34620=CARTESIAN_POINT('Ctrl Pts',(56.3748780843435,18.9698944544936,16.1180385853594));
#34621=CARTESIAN_POINT('Ctrl Pts',(56.4409272143529,19.0179104427556,16.1222745926386));
#34622=CARTESIAN_POINT('Ctrl Pts',(56.5066885838746,19.065717236677,16.1264921446328));
#34623=CARTESIAN_POINT('Ctrl Pts',(56.5701169401544,19.1168356941034,16.1307096966269));
#34624=CARTESIAN_POINT('Ctrl Pts',(56.6308664782144,19.1710044340577,16.1349272486211));
#34625=CARTESIAN_POINT('Ctrl Pts',(56.6915959581589,19.2251552887263,16.1391434080755));
#34626=CARTESIAN_POINT('Ctrl Pts',(56.749648029612,19.2823541167226,16.1433595675299));
#34627=CARTESIAN_POINT('Ctrl Pts',(56.8047105349806,19.3422997451499,16.1475757269844));
#34628=CARTESIAN_POINT('Ctrl Pts',(56.8597717283214,19.4022439451945,16.1517917859763));
#34629=CARTESIAN_POINT('Ctrl Pts',(56.9118431835207,19.4649344723882,16.1560078449682));
#34630=CARTESIAN_POINT('Ctrl Pts',(56.9606511343337,19.5300349053682,16.1602239039601));
#34631=CARTESIAN_POINT('Ctrl Pts',(57.0098586094086,19.5956682269862,16.1644744740885));
#34632=CARTESIAN_POINT('Ctrl Pts',(57.0557486051443,19.663750715539,16.168725044217));
#34633=CARTESIAN_POINT('Ctrl Pts',(57.0980845201935,19.7339069559766,16.1729756143455));
#34634=CARTESIAN_POINT('Ctrl Pts',(57.1401377547226,19.8035947572058,16.1771978030542));
#34635=CARTESIAN_POINT('Ctrl Pts',(57.1786840580431,19.8753282585799,16.181419991763));
#34636=CARTESIAN_POINT('Ctrl Pts',(57.2135381668652,19.9487155314421,16.1856421804717));
#34637=CARTESIAN_POINT('Ctrl Pts',(57.2487437080225,20.0228427647149,16.1899069413101));
#34638=CARTESIAN_POINT('Ctrl Pts',(57.2801819930715,20.0986568582413,16.1941717021484));
#34639=CARTESIAN_POINT('Ctrl Pts',(57.3077129245077,20.1757358990832,16.1984364629868));
#34640=CARTESIAN_POINT('Ctrl Pts',(57.3352438559439,20.2528149399252,16.2027012238251));
#34641=CARTESIAN_POINT('Ctrl Pts',(57.3588673561866,20.3311584482512,16.2069659846634));
#34642=CARTESIAN_POINT('Ctrl Pts',(57.3784960928316,20.4103334956227,16.2112307455018));
#34643=CARTESIAN_POINT('Ctrl Pts',(57.3979704577963,20.48888586486,16.2154619658067));
#34644=CARTESIAN_POINT('Ctrl Pts',(57.413585740031,20.5685512919107,16.2196931861116));
#34645=CARTESIAN_POINT('Ctrl Pts',(57.4252196594165,20.6489161730017,16.2239244064165));
#34646=CARTESIAN_POINT('Ctrl Pts',(57.4368368965758,20.7291658164779,16.2281495594477));
#34647=CARTESIAN_POINT('Ctrl Pts',(57.444484043332,20.8101124657808,16.2323747124788));
#34648=CARTESIAN_POINT('Ctrl Pts',(57.4480892655331,20.8913298661928,16.23659986551));
#34649=CARTESIAN_POINT('Ctrl Pts',(57.4517037494048,20.9727559108369,16.2408358727892));
#34650=CARTESIAN_POINT('Ctrl Pts',(57.4512554077082,21.0544536397797,16.2450718800684));
#34651=CARTESIAN_POINT('Ctrl Pts',(57.4467239565788,21.1359857724297,16.2493078873476));
#34652=CARTESIAN_POINT('Ctrl Pts',(57.4422122479137,21.2171626887996,16.2535254393418));
#34653=CARTESIAN_POINT('Ctrl Pts',(57.4336529517075,21.2981749811907,16.2577429913359));
#34654=CARTESIAN_POINT('Ctrl Pts',(57.4210781864923,21.3785903655553,16.2619605433301));
#34655=CARTESIAN_POINT('Ctrl Pts',(57.4085075731784,21.4589791985895,16.2661767027845));
#34656=CARTESIAN_POINT('Ctrl Pts',(57.3919241955128,21.5387710560022,16.2703928622389));
#34657=CARTESIAN_POINT('Ctrl Pts',(57.3714118509523,21.6175403494209,16.2746090216934));
#34658=CARTESIAN_POINT('Ctrl Pts',(57.3508999951595,21.6963077659269,16.2788250806853));
#34659=CARTESIAN_POINT('Ctrl Pts',(57.3264594768472,21.7740522172467,16.2830411396772));
#34660=CARTESIAN_POINT('Ctrl Pts',(57.2982245271079,21.8503612602887,16.2872571986691));
#34661=CARTESIAN_POINT('Ctrl Pts',(57.2697584562651,21.9272949416033,16.2915077687976));
#34662=CARTESIAN_POINT('Ctrl Pts',(57.2374356989915,22.0027691512276,16.295758338926));
#34663=CARTESIAN_POINT('Ctrl Pts',(57.201443401874,22.0763815301023,16.3000089090545));
#34664=CARTESIAN_POINT('Ctrl Pts',(57.1656914283979,22.1495023928372,16.3042310977633));
#34665=CARTESIAN_POINT('Ctrl Pts',(57.1263190506184,22.2207858312159,16.308453286472));
#34666=CARTESIAN_POINT('Ctrl Pts',(57.0835551270548,22.2898636681928,16.3126754751808));
#34667=CARTESIAN_POINT('Ctrl Pts',(57.0403600168672,22.3596380137413,16.3169402360191));
#34668=CARTESIAN_POINT('Ctrl Pts',(56.9937048585003,22.4271616299197,16.3212049968574));
#34669=CARTESIAN_POINT('Ctrl Pts',(56.9438681942022,22.4920880314409,16.3254697576958));
#34670=CARTESIAN_POINT('Ctrl Pts',(56.8940315299041,22.557014432962,16.3297345185341));
#34671=CARTESIAN_POINT('Ctrl Pts',(56.8410137207801,22.6193432944647,16.3339992793724));
#34672=CARTESIAN_POINT('Ctrl Pts',(56.7851311750811,22.6787664929208,16.3382640402108));
#34673=CARTESIAN_POINT('Ctrl Pts',(56.7296881218793,22.7377223531489,16.3424952605157));
#34674=CARTESIAN_POINT('Ctrl Pts',(56.6712173592052,22.7940391998182,16.3467264808206));
#34675=CARTESIAN_POINT('Ctrl Pts',(56.6100001086279,22.8473900238494,16.3509577011256));
#34676=CARTESIAN_POINT('Ctrl Pts',(56.5488706393034,22.9006643465329,16.3551828541567));
#34677=CARTESIAN_POINT('Ctrl Pts',(56.4850028513178,22.9509807906114,16.3594080071879));
#34678=CARTESIAN_POINT('Ctrl Pts',(56.4187159489162,22.9980478738736,16.363633160219));
#34679=CARTESIAN_POINT('Ctrl Pts',(56.3522587581308,23.0452358705779,16.3678691674982));
#34680=CARTESIAN_POINT('Ctrl Pts',(56.2833703358447,23.089157450691,16.3721051747774));
#34681=CARTESIAN_POINT('Ctrl Pts',(56.2124071023241,23.1295584679069,16.3763411820566));
#34682=CARTESIAN_POINT('Ctrl Pts',(56.1417530388818,23.1697834674157,16.3805587340508));
#34683=CARTESIAN_POINT('Ctrl Pts',(56.0690426079775,23.2065182779872,16.3847762860449));
#34684=CARTESIAN_POINT('Ctrl Pts',(55.9946564453281,23.2395554928975,16.3889938380391));
#34685=CARTESIAN_POINT('Ctrl Pts',(55.9202948432973,23.272581799671,16.3932099974935));
#34686=CARTESIAN_POINT('Ctrl Pts',(55.8442590328413,23.3019127466807,16.397426156948));
#34687=CARTESIAN_POINT('Ctrl Pts',(55.7669520451756,23.3273879802046,16.4016423164024));
#34688=CARTESIAN_POINT('Ctrl Pts',(55.689646899579,23.3528626067053,16.4058583753943));
#34689=CARTESIAN_POINT('Ctrl Pts',(55.6110710789075,23.3744815579321,16.4100744343862));
#34690=CARTESIAN_POINT('Ctrl Pts',(55.5316439154648,23.392133983946,16.4142904933781));
#34691=CARTESIAN_POINT('Ctrl Pts',(55.4515665899416,23.4099309063453,16.4185410635065));
#34692=CARTESIAN_POINT('Ctrl Pts',(55.370624384555,23.4236959469679,16.422791633635));
#34693=CARTESIAN_POINT('Ctrl Pts',(55.2892568505849,23.4333681851273,16.4270422037635));
#34694=CARTESIAN_POINT('Ctrl Pts',(55.2084326145874,23.4429758409265,16.4312643924722));
#34695=CARTESIAN_POINT('Ctrl Pts',(55.1271891852546,23.4485452133612,16.435486581181));
#34696=CARTESIAN_POINT('Ctrl Pts',(55.0459600100496,23.4500689638205,16.4397087698897));
#34697=CARTESIAN_POINT('Ctrl Pts',(54.9639118049027,23.4516080781837,16.4439735307281));
#34698=CARTESIAN_POINT('Ctrl Pts',(54.8818786285043,23.4490195430659,16.4482382915664));
#34699=CARTESIAN_POINT('Ctrl Pts',(54.8003026417379,23.4423495276277,16.4525030524048));
#34700=CARTESIAN_POINT('Ctrl Pts',(54.7187266549715,23.4356795121894,16.4567678132431));
#34701=CARTESIAN_POINT('Ctrl Pts',(54.6376083270162,23.4249281434262,16.4610325740814));
#34702=CARTESIAN_POINT('Ctrl Pts',(54.5573781172022,23.4101942077079,16.4652973349198));
#34703=CARTESIAN_POINT('Ctrl Pts',(54.477778883927,23.3955761481387,16.4695285552247));
#34704=CARTESIAN_POINT('Ctrl Pts',(54.3987553529978,23.3769831691967,16.4737597755296));
#34705=CARTESIAN_POINT('Ctrl Pts',(54.3207347734857,23.3544742517277,16.4779909958345));
#34706=CARTESIAN_POINT('Ctrl Pts',(54.2428260700237,23.3319976104708,16.4822161488657));
#34707=CARTESIAN_POINT('Ctrl Pts',(54.1659179046154,23.3056163106458,16.4864413018969));
#34708=CARTESIAN_POINT('Ctrl Pts',(54.0904282704373,23.2754405109298,16.490666454928));
#34709=CARTESIAN_POINT('Ctrl Pts',(54.0147447064282,23.2451871907992,16.4949024622072));
#34710=CARTESIAN_POINT('Ctrl Pts',(53.9404874343666,23.211119941561,16.4991384694864));
#34711=CARTESIAN_POINT('Ctrl Pts',(53.8680632558197,23.1734004364531,16.5033744767656));
#34712=CARTESIAN_POINT('Ctrl Pts',(53.7959546123441,23.1358452663362,16.5075920287598));
#34713=CARTESIAN_POINT('Ctrl Pts',(53.7256635417241,23.094669806884,16.5118095807539));
#34714=CARTESIAN_POINT('Ctrl Pts',(53.6575707034229,23.0500814212347,16.5160271327481));
#34715=CARTESIAN_POINT('Ctrl Pts',(53.5895003478277,23.0055077576558,16.5202432922025));
#34716=CARTESIAN_POINT('Ctrl Pts',(53.5236271718488,22.9575236601793,16.524459451657));
#34717=CARTESIAN_POINT('Ctrl Pts',(53.460304442681,22.9063808225987,16.5286756111114));
#34718=CARTESIAN_POINT('Ctrl Pts',(53.3969832223658,22.8552392036485,16.5328916701033));
#34719=CARTESIAN_POINT('Ctrl Pts',(53.3362126890234,22.8009392872248,16.5371077290952));
#34720=CARTESIAN_POINT('Ctrl Pts',(53.2783133538254,22.7437733059042,16.5413237880871));
#34721=CARTESIAN_POINT('Ctrl Pts',(53.2199400755756,22.6861393845018,16.5455743582156));
#34722=CARTESIAN_POINT('Ctrl Pts',(53.1644855702601,22.6255925861026,16.549824928344));
#34723=CARTESIAN_POINT('Ctrl Pts',(53.1122393598967,22.5624692047131,16.5540754984725));
#34724=CARTESIAN_POINT('Ctrl Pts',(53.0603420019414,22.4997673035314,16.5582976871813));
#34725=CARTESIAN_POINT('Ctrl Pts',(53.0116104567288,22.4345235358576,16.56251987589));
#34726=CARTESIAN_POINT('Ctrl Pts',(52.9662859150989,22.367098120427,16.5667420645988));
#34727=CARTESIAN_POINT('Ctrl Pts',(52.9205043682539,22.2989928577131,16.5710068254371));
#34728=CARTESIAN_POINT('Ctrl Pts',(52.8781991674195,22.2286621210014,16.5752715862754));
#34729=CARTESIAN_POINT('Ctrl Pts',(52.8395712689205,22.1565024634328,16.5795363471138));
#34730=CARTESIAN_POINT('Ctrl Pts',(52.8009433704215,22.0843428058643,16.5838011079521));
#34731=CARTESIAN_POINT('Ctrl Pts',(52.765992921951,22.0103546905198,16.5880658687904));
#34732=CARTESIAN_POINT('Ctrl Pts',(52.7348703241554,21.9349533686812,16.5923306296288));
#34733=CARTESIAN_POINT('Ctrl Pts',(52.700383049492,21.8514003788787,16.5970564555181));
#34734=CARTESIAN_POINT('Ctrl Pts',(52.6704856308601,21.7658477178848,16.6017822814074));
#34735=CARTESIAN_POINT('Ctrl Pts',(52.6453875193758,21.6787859132958,16.6065081072968));
#34736=CARTESIAN_POINT('Ctrl Pts',(52.620372265052,21.5920115284962,16.6112183316731));
#34737=CARTESIAN_POINT('Ctrl Pts',(52.6001248278688,21.5037381827685,16.6159285560493));
#34738=CARTESIAN_POINT('Ctrl Pts',(52.5848061128296,21.4144740490969,16.6206387804256));
#34739=CARTESIAN_POINT('Ctrl Pts',(52.5695741644158,21.3257155157731,16.6253223256533));
#34740=CARTESIAN_POINT('Ctrl Pts',(52.5592153803563,21.2359776385129,16.630005870881));
#34741=CARTESIAN_POINT('Ctrl Pts',(52.553839980721,21.1457786338287,16.6346894161087));
#34742=CARTESIAN_POINT('Ctrl Pts',(52.5509771614083,21.0977406329148,16.63718376902));
#34743=CARTESIAN_POINT('Ctrl Pts',(52.5495270008763,21.049572131945,16.6396781219313));
#34744=CARTESIAN_POINT('Ctrl Pts',(52.5495003736302,21.001353204219,16.6421724748426));
#34745=CARTESIAN_POINT('',(52.5495008534978,20.9979547636087,17.4421725287708));
#34746=CARTESIAN_POINT('Ctrl Pts',(52.5527477474802,21.0013508521608,16.6421725037879));
#34747=CARTESIAN_POINT('Ctrl Pts',(52.5552350469976,20.504606588975,16.6679029773045));
#34748=CARTESIAN_POINT('Ctrl Pts',(52.9435499391095,19.1868004307352,16.7359778823908));
#34749=CARTESIAN_POINT('Ctrl Pts',(55.0960917460929,18.1050615266267,16.8463972190466));
#34750=CARTESIAN_POINT('Ctrl Pts',(57.4845327466849,19.5110408269755,16.9734305137557));
#34751=CARTESIAN_POINT('Ctrl Pts',(57.5982440738356,22.2802461173785,17.1004638084647));
#34752=CARTESIAN_POINT('Ctrl Pts',(55.3331166026311,23.8773139761478,17.2274971031737));
#34753=CARTESIAN_POINT('Ctrl Pts',(53.0286539046507,22.9472535002863,17.3414000016147));
#34754=CARTESIAN_POINT('Ctrl Pts',(52.5557259094851,21.5611067451181,17.4129584684862));
#34755=CARTESIAN_POINT('Ctrl Pts',(52.5512853518551,20.9979567345713,17.4421725037879));
#34756=CARTESIAN_POINT('',(52.5495000073192,20.9998106024674,18.2421725037368));
#34757=CARTESIAN_POINT('Ctrl Pts',(52.5495008534978,20.9979547636087,17.4421725287708));
#34758=CARTESIAN_POINT('Ctrl Pts',(52.5495817226398,20.9010614341234,17.44719535461));
#34759=CARTESIAN_POINT('Ctrl Pts',(52.5554132275324,20.8044154643906,17.4522181804492));
#34760=CARTESIAN_POINT('Ctrl Pts',(52.5668846255356,20.7086242553934,17.4572410062884));
#34761=CARTESIAN_POINT('Ctrl Pts',(52.5785010996755,20.6116215969704,17.4623273546527));
#34762=CARTESIAN_POINT('Ctrl Pts',(52.5959009390986,20.5154955018815,17.467413703017));
#34763=CARTESIAN_POINT('Ctrl Pts',(52.6189200695926,20.4208552728281,17.4725000513813));
#34764=CARTESIAN_POINT('Ctrl Pts',(52.6325930837622,20.3646404130529,17.4755212651181));
#34765=CARTESIAN_POINT('Ctrl Pts',(52.6482477619896,20.308949382765,17.4785424788548));
#34766=CARTESIAN_POINT('Ctrl Pts',(52.6658418210588,20.2539062755377,17.4815636925916));
#34767=CARTESIAN_POINT('Ctrl Pts',(52.6904823617375,20.1768182131765,17.4857949128965));
#34768=CARTESIAN_POINT('Ctrl Pts',(52.7189920782052,20.1008075996192,17.4900261332014));
#34769=CARTESIAN_POINT('Ctrl Pts',(52.7512580351567,20.0262906873441,17.4942573535064));
#34770=CARTESIAN_POINT('Ctrl Pts',(52.7834777249843,19.9518806271057,17.4984825065375));
#34771=CARTESIAN_POINT('Ctrl Pts',(52.8194427747475,19.8789604372923,17.5027076595687));
#34772=CARTESIAN_POINT('Ctrl Pts',(52.8589906676706,19.807930669433,17.5069328125998));
#34773=CARTESIAN_POINT('Ctrl Pts',(52.8986401575386,19.7367184289595,17.511168819879));
#34774=CARTESIAN_POINT('Ctrl Pts',(52.9418907726608,19.6674067833562,17.5154048271582));
#34775=CARTESIAN_POINT('Ctrl Pts',(52.9885303274327,19.6003786203612,17.5196408344374));
#34776=CARTESIAN_POINT('Ctrl Pts',(53.03496668466,19.5336424832702,17.5238583864316));
#34777=CARTESIAN_POINT('Ctrl Pts',(53.0847622529817,19.4691703618106,17.5280759384257));
#34778=CARTESIAN_POINT('Ctrl Pts',(53.1376628599747,19.4073133933876,17.5322934904199));
#34779=CARTESIAN_POINT('Ctrl Pts',(53.1905460003907,19.3454768487285,17.5365096498743));
#34780=CARTESIAN_POINT('Ctrl Pts',(53.2465318416129,19.2862540954425,17.5407258093287));
#34781=CARTESIAN_POINT('Ctrl Pts',(53.3053257318486,19.2299634538051,17.5449419687831));
#34782=CARTESIAN_POINT('Ctrl Pts',(53.364118221145,19.1736741534597,17.549158027775));
#34783=CARTESIAN_POINT('Ctrl Pts',(53.4257182898329,19.1203171465723,17.5533740867669));
#34784=CARTESIAN_POINT('Ctrl Pts',(53.4897952511075,19.0701730993629,17.5575901457588));
#34785=CARTESIAN_POINT('Ctrl Pts',(53.5543967232505,19.0196185910888,17.5618407158872));
#34786=CARTESIAN_POINT('Ctrl Pts',(53.6215154571478,18.9723301938202,17.5660912860157));
#34787=CARTESIAN_POINT('Ctrl Pts',(53.69078101193,18.9285522233769,17.5703418561442));
#34788=CARTESIAN_POINT('Ctrl Pts',(53.7595840746877,18.8850665621807,17.574564044853));
#34789=CARTESIAN_POINT('Ctrl Pts',(53.8305049373513,18.8450447686413,17.5787862335617));
#34790=CARTESIAN_POINT('Ctrl Pts',(53.9031555871003,18.8086801730713,17.5830084222704));
#34791=CARTESIAN_POINT('Ctrl Pts',(53.9765387699242,18.7719489149993,17.5872731831088));
#34792=CARTESIAN_POINT('Ctrl Pts',(54.0516863740956,18.7389492160398,17.5915379439471));
#34793=CARTESIAN_POINT('Ctrl Pts',(54.1281794747178,18.709829870578,17.5958027047855));
#34794=CARTESIAN_POINT('Ctrl Pts',(54.20467257534,18.6807105251162,17.6000674656238));
#34795=CARTESIAN_POINT('Ctrl Pts',(54.2825106942889,18.6554716206412,17.6043322264622));
#34796=CARTESIAN_POINT('Ctrl Pts',(54.36126280213,18.634209425571,17.6085969873006));
#34797=CARTESIAN_POINT('Ctrl Pts',(54.4393955580764,18.6131144486383,17.6128282076055));
#34798=CARTESIAN_POINT('Ctrl Pts',(54.5187209550309,18.5958547063319,17.6170594279104));
#34799=CARTESIAN_POINT('Ctrl Pts',(54.5988280069488,18.5825610075968,17.6212906482153));
#34800=CARTESIAN_POINT('Ctrl Pts',(54.6788201909611,18.5692863710953,17.6255158012465));
#34801=CARTESIAN_POINT('Ctrl Pts',(54.7595913490877,18.5599665587695,17.6297409542777));
#34802=CARTESIAN_POINT('Ctrl Pts',(54.8407168036213,18.5546822060617,17.6339661073088));
#34803=CARTESIAN_POINT('Ctrl Pts',(54.9220506661816,18.5493842780645,17.638202114588));
#34804=CARTESIAN_POINT('Ctrl Pts',(55.0037401904558,18.548142686925,17.6424381218672));
#34805=CARTESIAN_POINT('Ctrl Pts',(55.0853486089544,18.5509867568856,17.6466741291464));
#34806=CARTESIAN_POINT('Ctrl Pts',(55.1666014788135,18.5538184359039,17.6508916811406));
#34807=CARTESIAN_POINT('Ctrl Pts',(55.247773480268,18.5607002416188,17.6551092331347));
#34808=CARTESIAN_POINT('Ctrl Pts',(55.3284317574115,18.5716090037386,17.6593267851289));
#34809=CARTESIAN_POINT('Ctrl Pts',(55.4090634030268,18.5825141640333,17.6635429445833));
#34810=CARTESIAN_POINT('Ctrl Pts',(55.4891812008074,18.5974435780524,17.6677591040378));
#34811=CARTESIAN_POINT('Ctrl Pts',(55.5683579201622,18.6163222691419,17.6719752634922));
#34812=CARTESIAN_POINT('Ctrl Pts',(55.6475327528962,18.6352005103904,17.6761913224841));
#34813=CARTESIAN_POINT('Ctrl Pts',(55.7257660998022,18.6580277326974,17.680407381476));
#34814=CARTESIAN_POINT('Ctrl Pts',(55.802642829588,18.6846782646658,17.6846234404679));
#34815=CARTESIAN_POINT('Ctrl Pts',(55.8801488445251,18.7115469482659,17.6888740105964));
#34816=CARTESIAN_POINT('Ctrl Pts',(55.9562754717608,18.7423016809405,17.6931245807249));
#34817=CARTESIAN_POINT('Ctrl Pts',(56.0306165673728,18.7767636785405,17.6973751508533));
#34818=CARTESIAN_POINT('Ctrl Pts',(56.1044612811412,18.8109955704397,17.7015973395621));
#34819=CARTESIAN_POINT('Ctrl Pts',(56.1765438481376,18.8488850974135,17.7058195282708));
#34820=CARTESIAN_POINT('Ctrl Pts',(56.2464914363706,18.8902110652829,17.7100417169796));
#34821=CARTESIAN_POINT('Ctrl Pts',(56.3171443028361,18.9319537209368,17.7143064778179));
#34822=CARTESIAN_POINT('Ctrl Pts',(56.3856184891288,18.9772022386538,17.7185712386563));
#34823=CARTESIAN_POINT('Ctrl Pts',(56.4515618227161,19.0256853024826,17.7228359994946));
#34824=CARTESIAN_POINT('Ctrl Pts',(56.5175051563034,19.0741683663115,17.7271007603329));
#34825=CARTESIAN_POINT('Ctrl Pts',(56.5809173044246,19.1258856219538,17.7313655211712));
#34826=CARTESIAN_POINT('Ctrl Pts',(56.6414836653779,19.1805271020711,17.7356302820096));
#34827=CARTESIAN_POINT('Ctrl Pts',(56.7015736976156,19.2347388501453,17.7398615023145));
#34828=CARTESIAN_POINT('Ctrl Pts',(56.7590879060606,19.2920322453441,17.7440927226194));
#34829=CARTESIAN_POINT('Ctrl Pts',(56.8136935348023,19.3521328901224,17.7483239429244));
#34830=CARTESIAN_POINT('Ctrl Pts',(56.8682208628942,19.4121473547825,17.7525490959555));
#34831=CARTESIAN_POINT('Ctrl Pts',(56.919847584601,19.4749607330765,17.7567742489867));
#34832=CARTESIAN_POINT('Ctrl Pts',(56.9682756776452,19.5402599180709,17.7609994020178));
#34833=CARTESIAN_POINT('Ctrl Pts',(57.0168281805107,19.6057268540427,17.765235409297));
#34834=CARTESIAN_POINT('Ctrl Pts',(57.0621652532177,19.6736920639891,17.7694714165762));
#34835=CARTESIAN_POINT('Ctrl Pts',(57.1040254316298,19.7438044606611,17.7737074238554));
#34836=CARTESIAN_POINT('Ctrl Pts',(57.1457032351135,19.8136113941503,17.7779249758496));
#34837=CARTESIAN_POINT('Ctrl Pts',(57.1839341302728,19.885546446283,17.7821425278437));
#34838=CARTESIAN_POINT('Ctrl Pts',(57.2185028816817,19.9592333527778,17.7863600798379));
#34839=CARTESIAN_POINT('Ctrl Pts',(57.2530602192752,20.0328959295324,17.7905762392923));
#34840=CARTESIAN_POINT('Ctrl Pts',(57.2839576170289,20.1083087914076,17.7947923987468));
#34841=CARTESIAN_POINT('Ctrl Pts',(57.3110264192234,20.18507231017,17.7990085582012));
#34842=CARTESIAN_POINT('Ctrl Pts',(57.3380945764232,20.2618339998133,17.8032246171931));
#34843=CARTESIAN_POINT('Ctrl Pts',(57.3613341658813,20.339945843526,17.807440676185));
#34844=CARTESIAN_POINT('Ctrl Pts',(57.3806256878986,20.4189908915367,17.8116567351769));
#34845=CARTESIAN_POINT('Ctrl Pts',(57.4000751233494,20.4986829737688,17.8159073053054));
#34846=CARTESIAN_POINT('Ctrl Pts',(57.4155114287791,20.5793231463309,17.8201578754338));
#34847=CARTESIAN_POINT('Ctrl Pts',(57.42686460485,20.660473212064,17.8244084455623));
#34848=CARTESIAN_POINT('Ctrl Pts',(57.4381419747948,20.7410814318785,17.8286306342711));
#34849=CARTESIAN_POINT('Ctrl Pts',(57.4453905959142,20.8221922832546,17.8328528229798));
#34850=CARTESIAN_POINT('Ctrl Pts',(57.4485941657342,20.9033725632514,17.8370750116886));
#34851=CARTESIAN_POINT('Ctrl Pts',(57.4518300369975,20.985371380182,17.8413397725269));
#34852=CARTESIAN_POINT('Ctrl Pts',(57.4509388309823,21.0674405479362,17.8456045333652));
#34853=CARTESIAN_POINT('Ctrl Pts',(57.4459575613102,21.149137045262,17.8498692942036));
#34854=CARTESIAN_POINT('Ctrl Pts',(57.4409762916381,21.2308335425878,17.8541340550419));
#34855=CARTESIAN_POINT('Ctrl Pts',(57.4319050755729,21.3121568977794,17.8583988158802));
#34856=CARTESIAN_POINT('Ctrl Pts',(57.4188337747238,21.3926747002994,17.8626635767186));
#34857=CARTESIAN_POINT('Ctrl Pts',(57.4058652741066,21.4725592644862,17.8668947970235));
#34858=CARTESIAN_POINT('Ctrl Pts',(57.3889107966641,21.5519504667765,17.8711260173284));
#34859=CARTESIAN_POINT('Ctrl Pts',(57.3680204733985,21.6304199295433,17.8753572376333));
#34860=CARTESIAN_POINT('Ctrl Pts',(57.3471601053945,21.7087768725925,17.8795823906645));
#34861=CARTESIAN_POINT('Ctrl Pts',(57.322375219031,21.7862142556502,17.8838075436957));
#34862=CARTESIAN_POINT('Ctrl Pts',(57.2937673036419,21.8623118964409,17.8880326967268));
#34863=CARTESIAN_POINT('Ctrl Pts',(57.2650858956698,21.9386050290072,17.892268704006));
#34864=CARTESIAN_POINT('Ctrl Pts',(57.2325618730893,22.0135510621235,17.8965047112852));
#34865=CARTESIAN_POINT('Ctrl Pts',(57.1963484602612,22.0867399372012,17.9007407185644));
#34866=CARTESIAN_POINT('Ctrl Pts',(57.1602928207353,22.159609945605,17.9049582705586));
#34867=CARTESIAN_POINT('Ctrl Pts',(57.1205800716868,22.2307376521125,17.9091758225527));
#34868=CARTESIAN_POINT('Ctrl Pts',(57.077409658326,22.2997381895959,17.9133933745469));
#34869=CARTESIAN_POINT('Ctrl Pts',(57.0342534988536,22.3687159446714,17.9176095340013));
#34870=CARTESIAN_POINT('Ctrl Pts',(56.9876421886092,22.4355675316493,17.9218256934557));
#34871=CARTESIAN_POINT('Ctrl Pts',(56.9378200605565,22.4999345528739,17.9260418529102));
#34872=CARTESIAN_POINT('Ctrl Pts',(56.8879991196641,22.5643000403627,17.9302579119021));
#34873=CARTESIAN_POINT('Ctrl Pts',(56.8349677985317,22.6261807128325,17.934473970894));
#34874=CARTESIAN_POINT('Ctrl Pts',(56.779011637759,22.6852500831384,17.9386900298859));
#34875=CARTESIAN_POINT('Ctrl Pts',(56.7225974400589,22.7448029739809,17.9429406000143));
#34876=CARTESIAN_POINT('Ctrl Pts',(56.6632106165959,22.8014979663097,17.9471911701428));
#34877=CARTESIAN_POINT('Ctrl Pts',(56.6011814009535,22.8550386441367,17.9514417402713));
#34878=CARTESIAN_POINT('Ctrl Pts',(56.5395663596809,22.9082218262858,17.95566392898));
#34879=CARTESIAN_POINT('Ctrl Pts',(56.4753445140025,22.9582924489776,17.9598861176888));
#34880=CARTESIAN_POINT('Ctrl Pts',(56.4088710167949,23.0050019222024,17.9641083063975));
#34881=CARTESIAN_POINT('Ctrl Pts',(56.3417272704506,23.0521823648424,17.9683730672359));
#34882=CARTESIAN_POINT('Ctrl Pts',(56.2722866214324,23.095933236925,17.9726378280742));
#34883=CARTESIAN_POINT('Ctrl Pts',(56.2009413814607,23.1360454228072,17.9769025889125));
#34884=CARTESIAN_POINT('Ctrl Pts',(56.1295961414889,23.1761576086893,17.9811673497509));
#34885=CARTESIAN_POINT('Ctrl Pts',(56.0563467704904,23.212630951131,17.9854321105892));
#34886=CARTESIAN_POINT('Ctrl Pts',(55.9816053200206,23.245306492599,17.9896968714275));
#34887=CARTESIAN_POINT('Ctrl Pts',(55.9074516793276,23.2777250548056,17.9939280917325));
#34888=CARTESIAN_POINT('Ctrl Pts',(55.8315512950746,23.3065269466999,17.9981593120374));
#34889=CARTESIAN_POINT('Ctrl Pts',(55.7542912874203,23.3315220144193,18.0023905323423));
#34890=CARTESIAN_POINT('Ctrl Pts',(55.6771420652096,23.356481240961,18.0066156853735));
#34891=CARTESIAN_POINT('Ctrl Pts',(55.5986375302757,23.3776443428533,18.0108408384046));
#34892=CARTESIAN_POINT('Ctrl Pts',(55.5191857643622,23.3948687630189,18.0150659914358));
#34893=CARTESIAN_POINT('Ctrl Pts',(55.4395298900606,23.4121374320265,18.019301998715));
#34894=CARTESIAN_POINT('Ctrl Pts',(55.358922346814,23.4254469735827,18.0235380059942));
#34895=CARTESIAN_POINT('Ctrl Pts',(55.2777907619473,23.4347037894941,18.0277740132734));
#34896=CARTESIAN_POINT('Ctrl Pts',(55.1970126482685,23.4439202756409,18.0319915652675));
#34897=CARTESIAN_POINT('Ctrl Pts',(55.1157155136274,23.4491192148747,18.0362091172617));
#34898=CARTESIAN_POINT('Ctrl Pts',(55.0343308805465,23.4502595047547,18.0404266692558));
#34899=CARTESIAN_POINT('Ctrl Pts',(54.9529731188199,23.4513994181369,18.0446428287102));
#34900=CARTESIAN_POINT('Ctrl Pts',(54.871528380536,23.4484833368552,18.0488589881647));
#34901=CARTESIAN_POINT('Ctrl Pts',(54.7904302867506,23.4415222270724,18.0530751476191));
#34902=CARTESIAN_POINT('Ctrl Pts',(54.7093341253685,23.4345612831588,18.057291206611));
#34903=CARTESIAN_POINT('Ctrl Pts',(54.6285850551857,23.4235555432474,18.0615072656029));
#34904=CARTESIAN_POINT('Ctrl Pts',(54.5486122285985,23.4085679001907,18.0657233245948));
#34905=CARTESIAN_POINT('Ctrl Pts',(54.4679847733293,23.3934575736997,18.0699738947233));
#34906=CARTESIAN_POINT('Ctrl Pts',(54.3881468028777,23.3742999269146,18.0742244648517));
#34907=CARTESIAN_POINT('Ctrl Pts',(54.3095264363016,23.3512117105513,18.0784750349802));
#34908=CARTESIAN_POINT('Ctrl Pts',(54.231431024627,23.3282776561803,18.082697223689));
#34909=CARTESIAN_POINT('Ctrl Pts',(54.1545374292306,23.3014655748344,18.0869194123977));
#34910=CARTESIAN_POINT('Ctrl Pts',(54.0792470958768,23.270939087591,18.0911416011065));
#34911=CARTESIAN_POINT('Ctrl Pts',(54.0031976136433,23.2401048032167,18.0954063619448));
#34912=CARTESIAN_POINT('Ctrl Pts',(53.928784347114,23.2054809919233,18.0996711227831));
#34913=CARTESIAN_POINT('Ctrl Pts',(53.8563957226305,23.1672839008266,18.1039358836215));
#34914=CARTESIAN_POINT('Ctrl Pts',(53.784007098147,23.1290868097299,18.1082006444598));
#34915=CARTESIAN_POINT('Ctrl Pts',(53.7136434972102,23.0873167400179,18.1124654052981));
#34916=CARTESIAN_POINT('Ctrl Pts',(53.6456619049135,23.0422337217365,18.1167301661365));
#34917=CARTESIAN_POINT('Ctrl Pts',(53.5783618985047,22.9976027074167,18.1209521683294));
#34918=CARTESIAN_POINT('Ctrl Pts',(53.5131415056379,22.94955588298,18.1251741705222));
#34919=CARTESIAN_POINT('Ctrl Pts',(53.4503694764712,22.8983138545951,18.1293961727151));
#34920=CARTESIAN_POINT('Ctrl Pts',(53.387687550532,22.8471453792275,18.1336121146288));
#34921=CARTESIAN_POINT('Ctrl Pts',(53.3274473680911,22.7927911007097,18.1378280565424));
#34922=CARTESIAN_POINT('Ctrl Pts',(53.269989142396,22.7355151058324,18.1420439984561));
#34923=CARTESIAN_POINT('Ctrl Pts',(53.2125973181063,22.6783053017659,18.1462550682307));
#34924=CARTESIAN_POINT('Ctrl Pts',(53.1579813909364,22.6181808191965,18.1504661380052));
#34925=CARTESIAN_POINT('Ctrl Pts',(53.1064477106784,22.5554452666696,18.1546772077798));
#34926=CARTESIAN_POINT('Ctrl Pts',(53.0549465744822,22.4927493323049,18.1588856182194));
#34927=CARTESIAN_POINT('Ctrl Pts',(53.0065241175869,22.4274459608158,18.1630940286591));
#34928=CARTESIAN_POINT('Ctrl Pts',(52.9614482602216,22.3598739111574,18.1673024390988));
#34929=CARTESIAN_POINT('Ctrl Pts',(52.9163868968525,22.2923235890729,18.1715094963376));
#34930=CARTESIAN_POINT('Ctrl Pts',(52.8746702553024,22.222506425746,18.1757165535765));
#34931=CARTESIAN_POINT('Ctrl Pts',(52.8365236665253,22.1507912080368,18.1799236108154));
#34932=CARTESIAN_POINT('Ctrl Pts',(52.7983775197472,22.0790768212816,18.1841306193077));
#34933=CARTESIAN_POINT('Ctrl Pts',(52.7638015616878,22.0054648370139,18.1883376278001));
#34934=CARTESIAN_POINT('Ctrl Pts',(52.732975074571,21.9303484494982,18.1925446362924));
#34935=CARTESIAN_POINT('Ctrl Pts',(52.7021181160096,21.8551578107442,18.1967558033392));
#34936=CARTESIAN_POINT('Ctrl Pts',(52.6750182095149,21.7784602315354,18.200966970386));
#34937=CARTESIAN_POINT('Ctrl Pts',(52.65180614198,21.7006681490955,18.2051781374328));
#34938=CARTESIAN_POINT('Ctrl Pts',(52.6285829340402,21.6228387311064,18.2093913255881));
#34939=CARTESIAN_POINT('Ctrl Pts',(52.6092513929158,21.5439142179396,18.2136045137433));
#34940=CARTESIAN_POINT('Ctrl Pts',(52.5938914951548,21.4643189775484,18.2178177018986));
#34941=CARTESIAN_POINT('Ctrl Pts',(52.5785040199944,21.3845808306238,18.2220384544774));
#34942=CARTESIAN_POINT('Ctrl Pts',(52.567102501311,21.3041700140185,18.2262592070563));
#34943=CARTESIAN_POINT('Ctrl Pts',(52.5597151524206,21.2235175891835,18.2304799596351));
#34944=CARTESIAN_POINT('Ctrl Pts',(52.5528935488415,21.1490417686845,18.2343774743357));
#34945=CARTESIAN_POINT('Ctrl Pts',(52.5494942454254,21.0743602572356,18.2382749890363));
#34946=CARTESIAN_POINT('Ctrl Pts',(52.5495000073192,20.9998106024675,18.2421725037368));
#34947=CARTESIAN_POINT('',(52.5495009535749,21.0021618208968,19.0421725037529));
#34948=CARTESIAN_POINT('Ctrl Pts',(52.5495000073193,20.9998106014887,18.242172503788));
#34949=CARTESIAN_POINT('Ctrl Pts',(52.5495007913209,20.9896669322961,18.2427028228071));
#34950=CARTESIAN_POINT('Ctrl Pts',(52.5495645584554,20.97952354572,18.2432331418263));
#34951=CARTESIAN_POINT('Ctrl Pts',(52.5496913003384,20.9693809477182,18.2437634608455));
#34952=CARTESIAN_POINT('Ctrl Pts',(52.5507025271837,20.8884568905792,18.2479946811504));
#34953=CARTESIAN_POINT('Ctrl Pts',(52.5557288629305,20.8074312572561,18.2522259014553));
#34954=CARTESIAN_POINT('Ctrl Pts',(52.5647840834785,20.7267351286385,18.2564571217602));
#34955=CARTESIAN_POINT('Ctrl Pts',(52.573826319474,20.6461547126213,18.2606822747914));
#34956=CARTESIAN_POINT('Ctrl Pts',(52.5868859150317,20.5659033210397,18.2649074278226));
#34957=CARTESIAN_POINT('Ctrl Pts',(52.6039246404514,20.4864115252813,18.2691325808537));
#34958=CARTESIAN_POINT('Ctrl Pts',(52.6210071376707,20.4067155182998,18.2733685881329));
#34959=CARTESIAN_POINT('Ctrl Pts',(52.6420892230513,20.3277834867746,18.2776045954121));
#34960=CARTESIAN_POINT('Ctrl Pts',(52.6670800035458,20.2500436411736,18.2818406026913));
#34961=CARTESIAN_POINT('Ctrl Pts',(52.6919619051015,20.1726424897521,18.2860581546855));
#34962=CARTESIAN_POINT('Ctrl Pts',(52.7207183788695,20.0964236056981,18.2902757066796));
#34963=CARTESIAN_POINT('Ctrl Pts',(52.7532090935203,20.021797120961,18.2944932586738));
#34964=CARTESIAN_POINT('Ctrl Pts',(52.7856890804763,19.9471952761915,18.2987094181282));
#34965=CARTESIAN_POINT('Ctrl Pts',(52.8219006743826,19.8741852125637,18.3029255775827));
#34966=CARTESIAN_POINT('Ctrl Pts',(52.8616552350494,19.8031575223913,18.3071417370371));
#34967=CARTESIAN_POINT('Ctrl Pts',(52.9014088484456,19.7321315246649,18.311357796029));
#34968=CARTESIAN_POINT('Ctrl Pts',(52.9447050327113,19.6630882116331,18.3155738550209));
#34969=CARTESIAN_POINT('Ctrl Pts',(52.9913096737311,19.5963927104942,18.3197899140128));
#34970=CARTESIAN_POINT('Ctrl Pts',(53.0382958035143,19.5291512640654,18.3240404841413));
#34971=CARTESIAN_POINT('Ctrl Pts',(53.0886445421045,19.4642966460451,18.3282910542697));
#34972=CARTESIAN_POINT('Ctrl Pts',(53.1420731264766,19.4021708531136,18.3325416243982));
#34973=CARTESIAN_POINT('Ctrl Pts',(53.1951449636285,19.3404598794067,18.336763813107));
#34974=CARTESIAN_POINT('Ctrl Pts',(53.2512552747237,19.2814416982429,18.3409860018157));
#34975=CARTESIAN_POINT('Ctrl Pts',(53.3100895781855,19.225414691754,18.3452081905245));
#34976=CARTESIAN_POINT('Ctrl Pts',(53.3695171051537,19.1688227676015,18.3494729513628));
#34977=CARTESIAN_POINT('Ctrl Pts',(53.4317234972464,19.1152829942843,18.3537377122011));
#34978=CARTESIAN_POINT('Ctrl Pts',(53.4963516845599,19.0650602093414,18.3580024730395));
#34979=CARTESIAN_POINT('Ctrl Pts',(53.5609798718733,19.0148374243984,18.3622672338778));
#34980=CARTESIAN_POINT('Ctrl Pts',(53.6280294227939,18.967931851362,18.3665319947161));
#34981=CARTESIAN_POINT('Ctrl Pts',(53.6971163264504,18.9245616407135,18.3707967555545));
#34982=CARTESIAN_POINT('Ctrl Pts',(53.7656598909403,18.8815325183591,18.3750279758594));
#34983=CARTESIAN_POINT('Ctrl Pts',(53.8364658830572,18.8418219556989,18.3792591961643));
#34984=CARTESIAN_POINT('Ctrl Pts',(53.9091795629834,18.8056752692031,18.3834904164693));
#34985=CARTESIAN_POINT('Ctrl Pts',(53.9817889765818,18.7695804145258,18.3877155695004));
#34986=CARTESIAN_POINT('Ctrl Pts',(54.0563002322929,18.7370394916865,18.3919407225316));
#34987=CARTESIAN_POINT('Ctrl Pts',(54.1323308198289,18.7082538439476,18.3961658755627));
#34988=CARTESIAN_POINT('Ctrl Pts',(54.2085567268834,18.6793942470384,18.4004018828419));
#34989=CARTESIAN_POINT('Ctrl Pts',(54.2863093787766,18.654309489749,18.4046378901211));
#34990=CARTESIAN_POINT('Ctrl Pts',(54.3651796937318,18.6331553855926,18.4088738974003));
#34991=CARTESIAN_POINT('Ctrl Pts',(54.443706389319,18.6120934448807,18.4130914493945));
#34992=CARTESIAN_POINT('Ctrl Pts',(54.523340579708,18.5949281079748,18.4173090013886));
#34993=CARTESIAN_POINT('Ctrl Pts',(54.6036615668166,18.5817638460271,18.4215265533828));
#34994=CARTESIAN_POINT('Ctrl Pts',(54.6839560337625,18.5686039306192,18.4257427128372));
#34995=CARTESIAN_POINT('Ctrl Pts',(54.764936388665,18.5594425418583,18.4299588722916));
#34996=CARTESIAN_POINT('Ctrl Pts',(54.846172157216,18.554332965266,18.4341750317461));
#34997=CARTESIAN_POINT('Ctrl Pts',(54.9274059900832,18.5492235104246,18.438391090738));
#34998=CARTESIAN_POINT('Ctrl Pts',(55.008894760424,18.5481657038711,18.4426071497299));
#34999=CARTESIAN_POINT('Ctrl Pts',(55.0902047336656,18.5511608145849,18.4468232087217));
#35000=CARTESIAN_POINT('Ctrl Pts',(55.1721802809889,18.5541804421936,18.4510737788502));
#35001=CARTESIAN_POINT('Ctrl Pts',(55.2539736105822,18.5613196431465,18.4553243489787));
#35002=CARTESIAN_POINT('Ctrl Pts',(55.3351440444507,18.5725262680166,18.4595749191072));
#35003=CARTESIAN_POINT('Ctrl Pts',(55.4157724964008,18.5836580652956,18.4637971078159));
#35004=CARTESIAN_POINT('Ctrl Pts',(55.4957858957313,18.5988029867764,18.4680192965247));
#35005=CARTESIAN_POINT('Ctrl Pts',(55.5747630124426,18.6178585832223,18.4722414852334));
#35006=CARTESIAN_POINT('Ctrl Pts',(55.6545364516964,18.6371063163482,18.4765062460718));
#35007=CARTESIAN_POINT('Ctrl Pts',(55.7332521272118,18.660343893077,18.4807710069101));
#35008=CARTESIAN_POINT('Ctrl Pts',(55.8104939020217,18.6874148913422,18.4850357677484));
#35009=CARTESIAN_POINT('Ctrl Pts',(55.8877356768317,18.7144858896075,18.4893005285868));
#35010=CARTESIAN_POINT('Ctrl Pts',(55.9635031290862,18.7453900679564,18.4935652894251));
#35011=CARTESIAN_POINT('Ctrl Pts',(56.0374047419543,18.7799230528266,18.4978300502635));
#35012=CARTESIAN_POINT('Ctrl Pts',(56.1107251500119,18.8141844504317,18.5020612705684));
#35013=CARTESIAN_POINT('Ctrl Pts',(56.182483924496,18.852146215288,18.5062924908733));
#35014=CARTESIAN_POINT('Ctrl Pts',(56.2522825941555,18.8936432984,18.5105237111783));
#35015=CARTESIAN_POINT('Ctrl Pts',(56.3219811774079,18.9350808775992,18.5147488642094));
#35016=CARTESIAN_POINT('Ctrl Pts',(56.3897248417463,18.9800434712623,18.5189740172406));
#35017=CARTESIAN_POINT('Ctrl Pts',(56.4551370060087,19.0283188534289,18.5231991702717));
#35018=CARTESIAN_POINT('Ctrl Pts',(56.5207172114877,19.0767182531087,18.5274351775509));
#35019=CARTESIAN_POINT('Ctrl Pts',(56.5839534975876,19.1284472782783,18.5316711848301));
#35020=CARTESIAN_POINT('Ctrl Pts',(56.6444931312107,19.1832466894482,18.5359071921093));
#35021=CARTESIAN_POINT('Ctrl Pts',(56.7047690079228,19.2378073525031,18.5401247441035));
#35022=CARTESIAN_POINT('Ctrl Pts',(56.7623713281544,19.2954113955379,18.5443422960976));
#35023=CARTESIAN_POINT('Ctrl Pts',(56.8169841998611,19.3557619796832,18.5485598480918));
#35024=CARTESIAN_POINT('Ctrl Pts',(56.87157903964,19.4160926374386,18.5527760075462));
#35025=CARTESIAN_POINT('Ctrl Pts',(56.923186079324,19.4791676909798,18.5569921670007));
#35026=CARTESIAN_POINT('Ctrl Pts',(56.9715271339629,19.5446543331401,18.5612083264551));
#35027=CARTESIAN_POINT('Ctrl Pts',(57.0198670367325,19.6101394148864,18.565424385447));
#35028=CARTESIAN_POINT('Ctrl Pts',(57.0649408339631,19.678035596293,18.5696404444389));
#35029=CARTESIAN_POINT('Ctrl Pts',(57.1065122790564,19.7479791262983,18.5738565034308));
#35030=CARTESIAN_POINT('Ctrl Pts',(57.1484240129886,19.8184951887851,18.5781070735593));
#35031=CARTESIAN_POINT('Ctrl Pts',(57.1867755332491,19.891091868116,18.5823576436877));
#35032=CARTESIAN_POINT('Ctrl Pts',(57.2213717123995,19.9653706144946,18.5866082138162));
#35033=CARTESIAN_POINT('Ctrl Pts',(57.2557368899074,20.0391533953407,18.590830402525));
#35034=CARTESIAN_POINT('Ctrl Pts',(57.2863966035495,20.1145953907973,18.5950525912337));
#35035=CARTESIAN_POINT('Ctrl Pts',(57.3132085346942,20.1912871183059,18.5992747799425));
#35036=CARTESIAN_POINT('Ctrl Pts',(57.3402908092758,20.2687521248852,18.6035395407808));
#35037=CARTESIAN_POINT('Ctrl Pts',(57.3634471335384,20.3474917412843,18.6078043016191));
#35038=CARTESIAN_POINT('Ctrl Pts',(57.3825833002841,20.4270714990442,18.6120690624575));
#35039=CARTESIAN_POINT('Ctrl Pts',(57.4017194670298,20.5066512568041,18.6163338232958));
#35040=CARTESIAN_POINT('Ctrl Pts',(57.4168354503997,20.5870706705503,18.6205985841341));
#35041=CARTESIAN_POINT('Ctrl Pts',(57.4278906833145,20.6678899581848,18.6248633449724));
#35042=CARTESIAN_POINT('Ctrl Pts',(57.4388589715159,20.7480736364335,18.6290945652774));
#35043=CARTESIAN_POINT('Ctrl Pts',(57.4458713284404,20.8289515948451,18.6333257855823));
#35044=CARTESIAN_POINT('Ctrl Pts',(57.4488503742784,20.9100995306101,18.6375570058872));
#35045=CARTESIAN_POINT('Ctrl Pts',(57.4518251483731,20.9911311059149,18.6417821589184));
#35046=CARTESIAN_POINT('Ctrl Pts',(57.4507780809056,21.0724314290177,18.6460073119495));
#35047=CARTESIAN_POINT('Ctrl Pts',(57.445683301105,21.1535690095559,18.6502324649807));
#35048=CARTESIAN_POINT('Ctrl Pts',(57.4405754330203,21.2349150292721,18.6544684722599));
#35049=CARTESIAN_POINT('Ctrl Pts',(57.4313989715538,21.3160970006676,18.6587044795391));
#35050=CARTESIAN_POINT('Ctrl Pts',(57.418180479306,21.3966779796048,18.6629404868183));
#35051=CARTESIAN_POINT('Ctrl Pts',(57.4050195769126,21.4769078862144,18.6671580388124));
#35052=CARTESIAN_POINT('Ctrl Pts',(57.387851858305,21.5565415631848,18.6713755908066));
#35053=CARTESIAN_POINT('Ctrl Pts',(57.3667554544363,21.6351526343296,18.6755931428007));
#35054=CARTESIAN_POINT('Ctrl Pts',(57.3456660161203,21.7137377498871,18.6798093022552));
#35055=CARTESIAN_POINT('Ctrl Pts',(57.3206505889357,21.7913004814464,18.6840254617096));
#35056=CARTESIAN_POINT('Ctrl Pts',(57.2918379712813,21.8674266328592,18.688241621164));
#35057=CARTESIAN_POINT('Ctrl Pts',(57.2630260401731,21.9435509703401,18.6924576801559));
#35058=CARTESIAN_POINT('Ctrl Pts',(57.230417264101,22.018238361307,18.6966737391478));
#35059=CARTESIAN_POINT('Ctrl Pts',(57.1941891815087,22.091093069243,18.7008897981397));
#35060=CARTESIAN_POINT('Ctrl Pts',(57.1576645489136,22.1645441395118,18.7051403682682));
#35061=CARTESIAN_POINT('Ctrl Pts',(57.1174612828544,22.236131948211,18.7093909383966));
#35062=CARTESIAN_POINT('Ctrl Pts',(57.0738084566093,22.305476439962,18.7136415085251));
#35063=CARTESIAN_POINT('Ctrl Pts',(57.0304471040127,22.3743579126199,18.7178636972338));
#35064=CARTESIAN_POINT('Ctrl Pts',(56.9836824371873,22.441025585864,18.7220858859426));
#35065=CARTESIAN_POINT('Ctrl Pts',(56.9337813495928,22.5051378481611,18.7263080746513));
#35066=CARTESIAN_POINT('Ctrl Pts',(56.8833771116861,22.5698965513746,18.7305728354897));
#35067=CARTESIAN_POINT('Ctrl Pts',(56.8297731655299,22.6320476535413,18.734837596328));
#35068=CARTESIAN_POINT('Ctrl Pts',(56.7732834856916,22.6912764201554,18.7391023571663));
#35069=CARTESIAN_POINT('Ctrl Pts',(56.7167938058533,22.7505051867694,18.7433671180047));
#35070=CARTESIAN_POINT('Ctrl Pts',(56.6574187861403,22.8068113329226,18.747631878843));
#35071=CARTESIAN_POINT('Ctrl Pts',(56.595505950671,22.8599223132629,18.7518966396814));
#35072=CARTESIAN_POINT('Ctrl Pts',(56.5340800333679,22.9126155982909,18.7561278599863));
#35073=CARTESIAN_POINT('Ctrl Pts',(56.4699257649903,22.9623614237981,18.7603590802912));
#35074=CARTESIAN_POINT('Ctrl Pts',(56.4033577027442,23.0088647062828,18.7645903005961));
#35075=CARTESIAN_POINT('Ctrl Pts',(56.3368850944403,23.0553013063151,18.7688154536273));
#35076=CARTESIAN_POINT('Ctrl Pts',(56.2680059444106,23.098504333733,18.7730406066584));
#35077=CARTESIAN_POINT('Ctrl Pts',(56.1970687784232,23.1382180875029,18.7772657596896));
#35078=CARTESIAN_POINT('Ctrl Pts',(56.1259493777121,23.1780338643074,18.7815017669688));
#35079=CARTESIAN_POINT('Ctrl Pts',(56.0527617360255,23.2143421144585,18.785737774248));
#35080=CARTESIAN_POINT('Ctrl Pts',(55.9778873921048,23.2469282361398,18.7899737815272));
#35081=CARTESIAN_POINT('Ctrl Pts',(55.9033392580483,23.2793723877715,18.7941913335214));
#35082=CARTESIAN_POINT('Ctrl Pts',(55.8271195139761,23.3081265819627,18.7984088855155));
#35083=CARTESIAN_POINT('Ctrl Pts',(55.7496287805504,23.3330252766249,18.8026264375097));
#35084=CARTESIAN_POINT('Ctrl Pts',(55.672163632802,23.3579157503045,18.8068425969641));
#35085=CARTESIAN_POINT('Ctrl Pts',(55.5934287713559,23.3789531103391,18.8110587564185));
#35086=CARTESIAN_POINT('Ctrl Pts',(55.5138420557708,23.3960209915026,18.815274915873));
#35087=CARTESIAN_POINT('Ctrl Pts',(55.4342572365759,23.4130884659731,18.8194909748649));
#35088=CARTESIAN_POINT('Ctrl Pts',(55.3538210584178,23.4261865532265,18.8237070338568));
#35089=CARTESIAN_POINT('Ctrl Pts',(55.2729622983371,23.4352498503617,18.8279230928487));
#35090=CARTESIAN_POINT('Ctrl Pts',(55.1914416576428,23.4443873363747,18.8321736629772));
#35091=CARTESIAN_POINT('Ctrl Pts',(55.1094919598312,23.4494236033213,18.8364242331056));
#35092=CARTESIAN_POINT('Ctrl Pts',(55.0275567494081,23.4503450523471,18.8406748032341));
#35093=CARTESIAN_POINT('Ctrl Pts',(54.9461686273817,23.4512603487791,18.8448969919429));
#35094=CARTESIAN_POINT('Ctrl Pts',(54.8647952666353,23.4481156898308,18.8491191806516));
#35095=CARTESIAN_POINT('Ctrl Pts',(54.7838684167242,23.4409500995946,18.8533413693604));
#35096=CARTESIAN_POINT('Ctrl Pts',(54.7021255852031,23.43371225905,18.8576061301987));
#35097=CARTESIAN_POINT('Ctrl Pts',(54.6208388006313,23.4223720122261,18.861870891037));
#35098=CARTESIAN_POINT('Ctrl Pts',(54.54044275794,23.4070225157381,18.8661356518754));
#35099=CARTESIAN_POINT('Ctrl Pts',(54.4600467152487,23.3916730192501,18.8704004127137));
#35100=CARTESIAN_POINT('Ctrl Pts',(54.3805418673589,23.3723144495057,18.874665173552));
#35101=CARTESIAN_POINT('Ctrl Pts',(54.3023456516815,23.3490910285198,18.8789299343904));
#35102=CARTESIAN_POINT('Ctrl Pts',(54.2247644160425,23.3260502498806,18.8831611546953));
#35103=CARTESIAN_POINT('Ctrl Pts',(54.1481803686174,23.299118837247,18.8873923750002));
#35104=CARTESIAN_POINT('Ctrl Pts',(54.0730120087879,23.2684010919916,18.8916235953052));
#35105=CARTESIAN_POINT('Ctrl Pts',(53.9979514351253,23.2377273938328,18.8958487483363));
#35106=CARTESIAN_POINT('Ctrl Pts',(53.9243029440742,23.20327832051,18.9000739013675));
#35107=CARTESIAN_POINT('Ctrl Pts',(53.85247036297,23.1652080690173,18.9042990543986));
#35108=CARTESIAN_POINT('Ctrl Pts',(53.7804532468567,23.1270400165812,18.9085350616778));
#35109=CARTESIAN_POINT('Ctrl Pts',(53.7102618332828,23.0852322973752,18.912771068957));
#35110=CARTESIAN_POINT('Ctrl Pts',(53.6422833169227,23.0399891319548,18.9170070762362));
#35111=CARTESIAN_POINT('Ctrl Pts',(53.5746009669319,22.9949430803396,18.9212246282304));
#35112=CARTESIAN_POINT('Ctrl Pts',(53.5091126662484,22.9464917073601,18.9254421802245));
#35113=CARTESIAN_POINT('Ctrl Pts',(53.4461747344618,22.8948818681319,18.9296597322187));
#35114=CARTESIAN_POINT('Ctrl Pts',(53.3832575833485,22.8432890692985,18.9338758916731));
#35115=CARTESIAN_POINT('Ctrl Pts',(53.3228894881164,22.7885401697459,18.9380920511276));
#35116=CARTESIAN_POINT('Ctrl Pts',(53.2653947955222,22.730923174089,18.942308210582));
#35117=CARTESIAN_POINT('Ctrl Pts',(53.2079014729099,22.6733075513284,18.9465242695739));
#35118=CARTESIAN_POINT('Ctrl Pts',(53.1532817444197,22.6128242982245,18.9507403285658));
#35119=CARTESIAN_POINT('Ctrl Pts',(53.1018230561569,22.5497982255322,18.9549563875577));
#35120=CARTESIAN_POINT('Ctrl Pts',(53.0499431456527,22.4862562441662,18.9592069576862));
#35121=CARTESIAN_POINT('Ctrl Pts',(53.0012765803358,22.4201299832977,18.9634575278146));
#35122=CARTESIAN_POINT('Ctrl Pts',(52.9560752859617,22.3517847511137,18.9677080979431));
#35123=CARTESIAN_POINT('Ctrl Pts',(52.9111758044901,22.2838958658812,18.9719302866519));
#35124=CARTESIAN_POINT('Ctrl Pts',(52.8696956450238,22.2138179871338,18.9761524753606));
#35125=CARTESIAN_POINT('Ctrl Pts',(52.8318361221775,22.1419350458348,18.9803746640694));
#35126=CARTESIAN_POINT('Ctrl Pts',(52.7935948635482,22.0693273122295,18.9846394249077));
#35127=CARTESIAN_POINT('Ctrl Pts',(52.7590478703977,21.9948783511333,18.988904185746));
#35128=CARTESIAN_POINT('Ctrl Pts',(52.7283525703267,21.9190039201541,18.9931689465844));
#35129=CARTESIAN_POINT('Ctrl Pts',(52.6976572702557,21.843129489175,18.9974337074227));
#35130=CARTESIAN_POINT('Ctrl Pts',(52.6708137606241,21.7658300645252,19.001698468261));
#35131=CARTESIAN_POINT('Ctrl Pts',(52.6479272046732,21.6875345922088,19.0059632290994));
#35132=CARTESIAN_POINT('Ctrl Pts',(52.6197371321448,21.5910956588898,19.0112162657558));
#35133=CARTESIAN_POINT('Ctrl Pts',(52.5974627565319,21.4928545750512,19.0164693024122));
#35134=CARTESIAN_POINT('Ctrl Pts',(52.5812939432754,21.3934606221259,19.0217223390686));
#35135=CARTESIAN_POINT('Ctrl Pts',(52.5653763691369,21.2956111022191,19.0268937514106));
#35136=CARTESIAN_POINT('Ctrl Pts',(52.5553761126385,21.1966441865217,19.0320651637527));
#35137=CARTESIAN_POINT('Ctrl Pts',(52.5514285146056,21.0972004676609,19.0372365760948));
#35138=CARTESIAN_POINT('Ctrl Pts',(52.5501725676789,21.065561979637,19.0388818853142));
#35139=CARTESIAN_POINT('Ctrl Pts',(52.549528931169,21.0338753951898,19.0405271945335));
#35140=CARTESIAN_POINT('Ctrl Pts',(52.5495009535749,21.0021618208968,19.0421725037529));
#35141=CARTESIAN_POINT('',(52.5495002327295,20.9989320078278,19.8421725038355));
#35142=CARTESIAN_POINT('Ctrl Pts',(52.5495009535743,21.0021618202204,19.042172503788));
#35143=CARTESIAN_POINT('Ctrl Pts',(52.5494297852942,20.9214900785257,19.0463577766029));
#35144=CARTESIAN_POINT('Ctrl Pts',(52.5533465260389,20.8407379080871,19.0505430494178));
#35145=CARTESIAN_POINT('Ctrl Pts',(52.561248273611,20.7603330080405,19.0547283222326));
#35146=CARTESIAN_POINT('Ctrl Pts',(52.5691465090023,20.6799638464871,19.0589117347711));
#35147=CARTESIAN_POINT('Ctrl Pts',(52.5810261897998,20.5999421189795,19.0630951473095));
#35148=CARTESIAN_POINT('Ctrl Pts',(52.5968324058427,20.5206924115017,19.0672785598479));
#35149=CARTESIAN_POINT('Ctrl Pts',(52.6126366275038,20.4414527035183,19.0714614445356));
#35150=CARTESIAN_POINT('Ctrl Pts',(52.632366307305,20.3629852857009,19.0756443292234));
#35151=CARTESIAN_POINT('Ctrl Pts',(52.655915337234,20.2857050022677,19.0798272139111));
#35152=CARTESIAN_POINT('Ctrl Pts',(52.6794688917087,20.2084098707424,19.084010902269));
#35153=CARTESIAN_POINT('Ctrl Pts',(52.7068431129201,20.132302777971,19.0881945906269));
#35154=CARTESIAN_POINT('Ctrl Pts',(52.7378823698768,20.0577823619324,19.0923782789848));
#35155=CARTESIAN_POINT('Ctrl Pts',(52.7689564606817,19.9831783152558,19.0965666624926));
#35156=CARTESIAN_POINT('Ctrl Pts',(52.8037036093297,19.9101649341082,19.1007550460004));
#35157=CARTESIAN_POINT('Ctrl Pts',(52.8419207859546,19.8391191465508,19.1049434295082));
#35158=CARTESIAN_POINT('Ctrl Pts',(52.880163830866,19.7680252698106,19.109134648032));
#35159=CARTESIAN_POINT('Ctrl Pts',(52.9218813306025,19.6989020392003,19.1133258665557));
#35160=CARTESIAN_POINT('Ctrl Pts',(52.9668265530173,19.6320979623948,19.1175170850795));
#35161=CARTESIAN_POINT('Ctrl Pts',(53.0118440847632,19.5651864090246,19.1217150465715));
#35162=CARTESIAN_POINT('Ctrl Pts',(53.0600994125051,19.5006018271536,19.1259130080635));
#35163=CARTESIAN_POINT('Ctrl Pts',(53.1113056482137,19.4386595837132,19.1301109695555));
#35164=CARTESIAN_POINT('Ctrl Pts',(53.1230381975715,19.4244671632308,19.1310728209731));
#35165=CARTESIAN_POINT('Ctrl Pts',(53.1349255128873,19.4104133028115,19.1320346723907));
#35166=CARTESIAN_POINT('Ctrl Pts',(53.1469638846957,19.3965015106406,19.1329965238083));
#35167=CARTESIAN_POINT('Ctrl Pts',(53.1999211318349,19.3353030173666,19.1372277441133));
#35168=CARTESIAN_POINT('Ctrl Pts',(53.2560126451939,19.2766160559906,19.1414589644182));
#35169=CARTESIAN_POINT('Ctrl Pts',(53.3149709686592,19.2207789868769,19.1456901847231));
#35170=CARTESIAN_POINT('Ctrl Pts',(53.3738447500152,19.1650219842123,19.1499153377543));
#35171=CARTESIAN_POINT('Ctrl Pts',(53.4355768423949,19.1121070746184,19.1541404907854));
#35172=CARTESIAN_POINT('Ctrl Pts',(53.4998603701468,19.0623386929229,19.1583656438166));
#35173=CARTESIAN_POINT('Ctrl Pts',(53.5643090396935,19.0124424582583,19.1626016510958));
#35174=CARTESIAN_POINT('Ctrl Pts',(53.6313219567419,18.9657092915203,19.166837658375));
#35175=CARTESIAN_POINT('Ctrl Pts',(53.700553517281,18.9224078628014,19.1710736656542));
#35176=CARTESIAN_POINT('Ctrl Pts',(53.7694834522328,18.8792950881989,19.1752912176483));
#35177=CARTESIAN_POINT('Ctrl Pts',(53.8406123464424,18.8395844664646,19.1795087696425));
#35178=CARTESIAN_POINT('Ctrl Pts',(53.9135684680578,18.8034989696334,19.1837263216366));
#35179=CARTESIAN_POINT('Ctrl Pts',(53.9865005012216,18.7674253874122,19.1879424810911));
#35180=CARTESIAN_POINT('Ctrl Pts',(54.0612581473,18.7349747591132,19.1921586405455));
#35181=CARTESIAN_POINT('Ctrl Pts',(54.1374453520316,18.7063239702896,19.1963748));
#35182=CARTESIAN_POINT('Ctrl Pts',(54.2136307413766,18.6776738641562,19.2005908589919));
#35183=CARTESIAN_POINT('Ctrl Pts',(54.2912451860894,18.6528235800871,19.2048069179838));
#35184=CARTESIAN_POINT('Ctrl Pts',(54.3698742973329,18.6319012164104,19.2090229769757));
#35185=CARTESIAN_POINT('Ctrl Pts',(54.4491470380896,18.6108075898194,19.2132735471042));
#35186=CARTESIAN_POINT('Ctrl Pts',(54.5294506739798,18.593706624379,19.2175241172326));
#35187=CARTESIAN_POINT('Ctrl Pts',(54.6103485494582,18.5806773681275,19.2217746873611));
#35188=CARTESIAN_POINT('Ctrl Pts',(54.6907062629137,18.5677351093325,19.2259968760699));
#35189=CARTESIAN_POINT('Ctrl Pts',(54.771649831094,18.5588103410262,19.2302190647786));
#35190=CARTESIAN_POINT('Ctrl Pts',(54.8527464809369,18.5539283225703,19.2344412534874));
#35191=CARTESIAN_POINT('Ctrl Pts',(54.9346608244747,18.5489970789527,19.2387060143257));
#35192=CARTESIAN_POINT('Ctrl Pts',(55.0167308683073,18.5481905745412,19.242970775164));
#35193=CARTESIAN_POINT('Ctrl Pts',(55.0985129203709,18.5514809670905,19.2472355360024));
#35194=CARTESIAN_POINT('Ctrl Pts',(55.1802949724344,18.5547713596398,19.2515002968407));
#35195=CARTESIAN_POINT('Ctrl Pts',(55.2617885586987,18.5621585416679,19.255765057679));
#35196=CARTESIAN_POINT('Ctrl Pts',(55.3425595024362,18.5735616147755,19.2600298185174));
#35197=CARTESIAN_POINT('Ctrl Pts',(55.4226952169922,18.5848750075544,19.2642610388223));
#35198=CARTESIAN_POINT('Ctrl Pts',(55.5024201211983,18.6001837291142,19.2684922591272));
#35199=CARTESIAN_POINT('Ctrl Pts',(55.5813048921626,18.6194465197463,19.2727234794322));
#35200=CARTESIAN_POINT('Ctrl Pts',(55.6600765478865,18.6386816888849,19.2769486324633));
#35201=CARTESIAN_POINT('Ctrl Pts',(55.7380100151372,18.661859556974,19.2811737854945));
#35202=CARTESIAN_POINT('Ctrl Pts',(55.8146831023249,18.6888873474479,19.2853989385256));
#35203=CARTESIAN_POINT('Ctrl Pts',(55.891553159587,18.7159845712276,19.2896349458048));
#35204=CARTESIAN_POINT('Ctrl Pts',(55.9671558862857,18.746951450961,19.293870953084));
#35205=CARTESIAN_POINT('Ctrl Pts',(56.0410781422642,18.7816432767249,19.2981069603632));
#35206=CARTESIAN_POINT('Ctrl Pts',(56.1146783364012,18.8161839583829,19.3023245123574));
#35207=CARTESIAN_POINT('Ctrl Pts',(56.1866122450872,18.8544170049677,19.3065420643515));
#35208=CARTESIAN_POINT('Ctrl Pts',(56.2564909582044,18.8961509745348,19.3107596163457));
#35209=CARTESIAN_POINT('Ctrl Pts',(56.3263465989601,18.9378711644946,19.3149757758001));
#35210=CARTESIAN_POINT('Ctrl Pts',(56.3941479928693,18.9830897437309,19.3191919352545));
#35211=CARTESIAN_POINT('Ctrl Pts',(56.4595317651643,19.0315698446538,19.323408094709));
#35212=CARTESIAN_POINT('Ctrl Pts',(56.5249139794966,19.0800487903942,19.3276241537009));
#35213=CARTESIAN_POINT('Ctrl Pts',(56.5878783139519,19.1317888255023,19.3318402126928));
#35214=CARTESIAN_POINT('Ctrl Pts',(56.6480924451072,19.1865112235305,19.3360562716847));
#35215=CARTESIAN_POINT('Ctrl Pts',(56.708799467398,19.2416815593499,19.3403068418131));
#35216=CARTESIAN_POINT('Ctrl Pts',(56.7667106884168,19.2998829977883,19.3445574119416));
#35217=CARTESIAN_POINT('Ctrl Pts',(56.8215229250338,19.3607915069839,19.3488079820701));
#35218=CARTESIAN_POINT('Ctrl Pts',(56.8759691756664,19.4212933248623,19.3530301707788));
#35219=CARTESIAN_POINT('Ctrl Pts',(56.9273574519107,19.4844657696759,19.3572523594876));
#35220=CARTESIAN_POINT('Ctrl Pts',(56.9754318709531,19.5499589063675,19.3614745481964));
#35221=CARTESIAN_POINT('Ctrl Pts',(57.0239910220948,19.6161124072669,19.3657393090347));
#35222=CARTESIAN_POINT('Ctrl Pts',(57.0691688455571,19.6846332567307,19.370004069873));
#35223=CARTESIAN_POINT('Ctrl Pts',(57.1107481558536,19.7551335523196,19.3742688307113));
#35224=CARTESIAN_POINT('Ctrl Pts',(57.1523274661502,19.8256338479085,19.3785335915497));
#35225=CARTESIAN_POINT('Ctrl Pts',(57.1903080965616,19.8981131330463,19.382798352388));
#35226=CARTESIAN_POINT('Ctrl Pts',(57.2245226006815,19.9721627322104,19.3870631132263));
#35227=CARTESIAN_POINT('Ctrl Pts',(57.2584680222521,20.0456299627146,19.3912943335313));
#35228=CARTESIAN_POINT('Ctrl Pts',(57.2888336769176,20.1209183703428,19.3955255538362));
#35229=CARTESIAN_POINT('Ctrl Pts',(57.3154214442977,20.1976448509006,19.3997567741411));
#35230=CARTESIAN_POINT('Ctrl Pts',(57.3419710866803,20.2742613110556,19.4039819271723));
#35231=CARTESIAN_POINT('Ctrl Pts',(57.3647534498519,20.3523113130751,19.4082070802034));
#35232=CARTESIAN_POINT('Ctrl Pts',(57.3836175664651,20.431389811172,19.4124322332346));
#35233=CARTESIAN_POINT('Ctrl Pts',(57.4025301442344,20.5106714587467,19.4166682405138));
#35234=CARTESIAN_POINT('Ctrl Pts',(57.4175041258897,20.5909864623144,19.420904247793));
#35235=CARTESIAN_POINT('Ctrl Pts',(57.4284370882124,20.6719092220216,19.4251402550722));
#35236=CARTESIAN_POINT('Ctrl Pts',(57.4393224181958,20.7524794203431,19.4293578070663));
#35237=CARTESIAN_POINT('Ctrl Pts',(57.4462017962051,20.8336516275832,19.4335753590605));
#35238=CARTESIAN_POINT('Ctrl Pts',(57.449025202975,20.9149952637015,19.4377929110547));
#35239=CARTESIAN_POINT('Ctrl Pts',(57.4518476775203,20.9963120420016,19.4420090705091));
#35240=CARTESIAN_POINT('Ctrl Pts',(57.4506168241535,21.0777996724995,19.4462252299635));
#35241=CARTESIAN_POINT('Ctrl Pts',(57.4453346376679,21.1590244000826,19.4504413894179));
#35242=CARTESIAN_POINT('Ctrl Pts',(57.4400525770461,21.2402471922451,19.4546574484098));
#35243=CARTESIAN_POINT('Ctrl Pts',(57.4307194065195,21.3212066300785,19.4588735074017));
#35244=CARTESIAN_POINT('Ctrl Pts',(57.4173891288913,21.4014723521216,19.4630895663936));
#35245=CARTESIAN_POINT('Ctrl Pts',(57.4039497344238,21.4823951003831,19.4673401365221));
#35246=CARTESIAN_POINT('Ctrl Pts',(57.3864475558196,21.5626122475542,19.4715907066506));
#35247=CARTESIAN_POINT('Ctrl Pts',(57.364990463597,21.6416933512942,19.475841276779));
#35248=CARTESIAN_POINT('Ctrl Pts',(57.3436766422115,21.7202464237515,19.4800634654878));
#35249=CARTESIAN_POINT('Ctrl Pts',(57.3184607651209,21.7976781502054,19.4842856541965));
#35250=CARTESIAN_POINT('Ctrl Pts',(57.2894981148884,21.8735837864353,19.4885078429053));
#35251=CARTESIAN_POINT('Ctrl Pts',(57.2602434356198,21.9502547756146,19.4927726037436));
#35252=CARTESIAN_POINT('Ctrl Pts',(57.227166196645,22.0253682817625,19.4970373645819));
#35253=CARTESIAN_POINT('Ctrl Pts',(57.1904745646009,22.0985314887779,19.5013021254203));
#35254=CARTESIAN_POINT('Ctrl Pts',(57.1537829325567,22.1716946957933,19.5055668862586));
#35255=CARTESIAN_POINT('Ctrl Pts',(57.1134772006757,22.2429072160272,19.5098316470969));
#35256=CARTESIAN_POINT('Ctrl Pts',(57.0698099594893,22.3118067622935,19.5140964079353));
#35257=CARTESIAN_POINT('Ctrl Pts',(57.026486142616,22.3801644428795,19.5183276282402));
#35258=CARTESIAN_POINT('Ctrl Pts',(56.9796910805182,22.4465017586957,19.5225588485451));
#35259=CARTESIAN_POINT('Ctrl Pts',(56.9296392456943,22.5104445145308,19.52679006885));
#35260=CARTESIAN_POINT('Ctrl Pts',(56.8796591816983,22.5742955809296,19.5310152218812));
#35261=CARTESIAN_POINT('Ctrl Pts',(56.8264319040669,22.6357585437843,19.5352403749124));
#35262=CARTESIAN_POINT('Ctrl Pts',(56.7702158888053,22.6944869303188,19.5394655279435));
#35263=CARTESIAN_POINT('Ctrl Pts',(56.7138554568637,22.7533661877139,19.5437015352227));
#35264=CARTESIAN_POINT('Ctrl Pts',(56.6544911698454,22.8094964055248,19.5479375425019));
#35265=CARTESIAN_POINT('Ctrl Pts',(56.5924250956956,22.8625607546061,19.5521735497811));
#35266=CARTESIAN_POINT('Ctrl Pts',(56.5306294287983,22.9153939148288,19.5563911017753));
#35267=CARTESIAN_POINT('Ctrl Pts',(56.4661558180753,22.965187554888,19.5606086537694));
#35268=CARTESIAN_POINT('Ctrl Pts',(56.3993389305689,23.0116661769276,19.5648262057636));
#35269=CARTESIAN_POINT('Ctrl Pts',(56.3325441044787,23.0581294527835,19.569042365218));
#35270=CARTESIAN_POINT('Ctrl Pts',(56.2634079194224,23.1012796189479,19.5732585246725));
#35271=CARTESIAN_POINT('Ctrl Pts',(56.1922959134083,23.1408831600229,19.5774746841269));
#35272=CARTESIAN_POINT('Ctrl Pts',(56.1211856018494,23.1804857574258,19.5816907431188));
#35273=CARTESIAN_POINT('Ctrl Pts',(56.0480999696586,23.2165416725246,19.5859068021107));
#35274=CARTESIAN_POINT('Ctrl Pts',(55.9734299032573,23.2488629290031,19.5901228611026));
#35275=CARTESIAN_POINT('Ctrl Pts',(55.8981486146541,23.2814487556167,19.594373431231));
#35276=CARTESIAN_POINT('Ctrl Pts',(55.8212572667672,23.3102382949725,19.5986240013595));
#35277=CARTESIAN_POINT('Ctrl Pts',(55.7431760222275,23.3350887884588,19.602874571488));
#35278=CARTESIAN_POINT('Ctrl Pts',(55.6656161328252,23.3597733530781,19.6070967601967));
#35279=CARTESIAN_POINT('Ctrl Pts',(55.5868826581863,23.3805712541825,19.6113189489055));
#35280=CARTESIAN_POINT('Ctrl Pts',(55.5073998763178,23.3973935045196,19.6155411376142));
#35281=CARTESIAN_POINT('Ctrl Pts',(55.4271156733091,23.4143853728132,19.6198058984526));
#35282=CARTESIAN_POINT('Ctrl Pts',(55.3460674472878,23.4273208899218,19.6240706592909));
#35283=CARTESIAN_POINT('Ctrl Pts',(55.2646981287331,23.4361619713486,19.6283354201293));
#35284=CARTESIAN_POINT('Ctrl Pts',(55.1833288101783,23.4450030527755,19.6326001809676));
#35285=CARTESIAN_POINT('Ctrl Pts',(55.1016388838035,23.4497497347133,19.6368649418059));
#35286=CARTESIAN_POINT('Ctrl Pts',(55.0200697162189,23.4504178126374,19.6411297026443));
#35287=CARTESIAN_POINT('Ctrl Pts',(54.9391420555075,23.4510806364124,19.6453609229492));
#35288=CARTESIAN_POINT('Ctrl Pts',(54.8580297917767,23.4477313112697,19.6495921432541));
#35289=CARTESIAN_POINT('Ctrl Pts',(54.777163628751,23.440347147774,19.6538233635591));
#35290=CARTESIAN_POINT('Ctrl Pts',(54.6964134221429,23.4329735726519,19.6580485165902));
#35291=CARTESIAN_POINT('Ctrl Pts',(54.6159090744608,23.4215766918839,19.6622736696214));
#35292=CARTESIAN_POINT('Ctrl Pts',(54.5360818557209,23.4061858210472,19.6664988226526));
#35293=CARTESIAN_POINT('Ctrl Pts',(54.45604956407,23.390755411683,19.6707348299318));
#35294=CARTESIAN_POINT('Ctrl Pts',(54.3766983568976,23.3713104677392,19.674970837211));
#35295=CARTESIAN_POINT('Ctrl Pts',(54.2984582330946,23.3479330057068,19.6792068444902));
#35296=CARTESIAN_POINT('Ctrl Pts',(54.2205589830653,23.324657393765,19.6834243964843));
#35297=CARTESIAN_POINT('Ctrl Pts',(54.1437616057692,23.2974835844915,19.6876419484785));
#35298=CARTESIAN_POINT('Ctrl Pts',(54.0684790480282,23.266543396019,19.6918595004726));
#35299=CARTESIAN_POINT('Ctrl Pts',(53.9932213468753,23.235613423293,19.6960756599271));
#35300=CARTESIAN_POINT('Ctrl Pts',(53.9194779017149,23.2009197175233,19.7002918193815));
#35301=CARTESIAN_POINT('Ctrl Pts',(53.8476431231349,23.162642799526,19.7045079788359));
#35302=CARTESIAN_POINT('Ctrl Pts',(53.775810056232,23.1243667935901,19.7087240378278));
#35303=CARTESIAN_POINT('Ctrl Pts',(53.7058859752706,23.0825079647952,19.7129400968197));
#35304=CARTESIAN_POINT('Ctrl Pts',(53.6382407717543,23.0372928248751,19.7171561558116));
#35305=CARTESIAN_POINT('Ctrl Pts',(53.5700418490274,22.991707570146,19.7214067259401));
#35306=CARTESIAN_POINT('Ctrl Pts',(53.5041596918322,22.9427110568059,19.7256572960685));
#35307=CARTESIAN_POINT('Ctrl Pts',(53.4409420723575,22.8905789135223,19.729907866197));
#35308=CARTESIAN_POINT('Ctrl Pts',(53.3781465623265,22.8387948610112,19.7341300549058));
#35309=CARTESIAN_POINT('Ctrl Pts',(53.3179804209147,22.7839172868419,19.7383522436145));
#35310=CARTESIAN_POINT('Ctrl Pts',(53.2607484711599,22.7262544335721,19.7425744323233));
#35311=CARTESIAN_POINT('Ctrl Pts',(53.2029394543555,22.6680101684728,19.7468391931616));
#35312=CARTESIAN_POINT('Ctrl Pts',(53.1481244573347,22.6069245020227,19.7511039539999));
#35313=CARTESIAN_POINT('Ctrl Pts',(53.0965756466165,22.5433489498317,19.7553687148383));
#35314=CARTESIAN_POINT('Ctrl Pts',(53.0450268358984,22.4797733976408,19.7596334756766));
#35315=CARTESIAN_POINT('Ctrl Pts',(52.9967444438948,22.4137083866067,19.7638982365149));
#35316=CARTESIAN_POINT('Ctrl Pts',(52.9519545173027,22.345533333219,19.7681629973533));
#35317=CARTESIAN_POINT('Ctrl Pts',(52.9066393874759,22.276558864398,19.7724777664492));
#35318=CARTESIAN_POINT('Ctrl Pts',(52.8647339880631,22.2051736964748,19.7767925355452));
#35319=CARTESIAN_POINT('Ctrl Pts',(52.8264977671134,22.1317412662075,19.7811073046411));
#35320=CARTESIAN_POINT('Ctrl Pts',(52.7883228181496,22.0584265084174,19.7854151594954));
#35321=CARTESIAN_POINT('Ctrl Pts',(52.7538055636304,21.983071395981,19.7897230143497));
#35322=CARTESIAN_POINT('Ctrl Pts',(52.7231620146361,21.9060678994446,19.794030869204));
#35323=CARTESIAN_POINT('Ctrl Pts',(52.6925687719447,21.8291908165042,19.7983316520233));
#35324=CARTESIAN_POINT('Ctrl Pts',(52.6658367414319,21.7506711416486,19.8026324348426));
#35325=CARTESIAN_POINT('Ctrl Pts',(52.6431351825498,21.6709236038963,19.8069332176618));
#35326=CARTESIAN_POINT('Ctrl Pts',(52.6204555946949,21.5912532474222,19.8112298380966));
#35327=CARTESIAN_POINT('Ctrl Pts',(52.6017988463954,21.5103578116504,19.8155264585314));
#35328=CARTESIAN_POINT('Ctrl Pts',(52.587285206786,21.4286695424289,19.8198230789662));
#35329=CARTESIAN_POINT('Ctrl Pts',(52.5727825748233,21.3470432284185,19.8241164406953));
#35330=CARTESIAN_POINT('Ctrl Pts',(52.5624168795559,21.2646257096145,19.8284098024244));
#35331=CARTESIAN_POINT('Ctrl Pts',(52.5562575955193,21.1818606899327,19.8327031641535));
#35332=CARTESIAN_POINT('Ctrl Pts',(52.5517293372353,21.1210124835883,19.8358596106983));
#35333=CARTESIAN_POINT('Ctrl Pts',(52.5494736278551,21.0599767387354,19.8390160572431));
#35334=CARTESIAN_POINT('Ctrl Pts',(52.5495002327291,20.9989320087486,19.8421725037879));
#35335=CARTESIAN_POINT('',(52.5495005252726,20.9983955185562,20.6421725037879));
#35336=CARTESIAN_POINT('Ctrl Pts',(52.5495002327295,20.9989320078278,19.8421725038355));
#35337=CARTESIAN_POINT('Ctrl Pts',(52.5495391024497,20.9097457359996,19.8467840681691));
#35338=CARTESIAN_POINT('Ctrl Pts',(52.5544510791458,20.8207169626876,19.8513956325027));
#35339=CARTESIAN_POINT('Ctrl Pts',(52.5641597639198,20.7323573384293,19.8560071968362));
#35340=CARTESIAN_POINT('Ctrl Pts',(52.5738970811663,20.6437371274313,19.8606323614145));
#35341=CARTESIAN_POINT('Ctrl Pts',(52.5884593140069,20.5557903160324,19.8652575259928));
#35342=CARTESIAN_POINT('Ctrl Pts',(52.6077191292299,20.4690174340456,19.8698826905711));
#35343=CARTESIAN_POINT('Ctrl Pts',(52.6270652852011,20.38185555375,19.8745285895212));
#35344=CARTESIAN_POINT('Ctrl Pts',(52.6511511000742,20.2958784425238,19.8791744884714));
#35345=CARTESIAN_POINT('Ctrl Pts',(52.6797988482953,20.2115731704032,19.8838203874215));
#35346=CARTESIAN_POINT('Ctrl Pts',(52.7031810509242,20.1427634705903,19.8876123556351));
#35347=CARTESIAN_POINT('Ctrl Pts',(52.7296013596882,20.0750671950961,19.8914043238486));
#35348=CARTESIAN_POINT('Ctrl Pts',(52.7589403160553,20.0087372986955,19.8951962920622));
#35349=CARTESIAN_POINT('Ctrl Pts',(52.7916778235747,19.934723913386,19.8994275123671));
#35350=CARTESIAN_POINT('Ctrl Pts',(52.8281472075493,19.8621952891128,19.9036587326721));
#35351=CARTESIAN_POINT('Ctrl Pts',(52.8681916962783,19.7915532257549,19.907889952977));
#35352=CARTESIAN_POINT('Ctrl Pts',(52.9081787640133,19.7210124581716,19.9121151060081));
#35353=CARTESIAN_POINT('Ctrl Pts',(52.9517305276497,19.6523532798264,19.9163402590393));
#35354=CARTESIAN_POINT('Ctrl Pts',(52.9986425958401,19.585956581001,19.9205654120705));
#35355=CARTESIAN_POINT('Ctrl Pts',(53.0456751792452,19.5193893117292,19.9248014193497));
#35356=CARTESIAN_POINT('Ctrl Pts',(53.0960851574693,19.4550965903672,19.9290374266289));
#35357=CARTESIAN_POINT('Ctrl Pts',(53.1496206424203,19.3934364366628,19.9332734339081));
#35358=CARTESIAN_POINT('Ctrl Pts',(53.2029228858847,19.3320449217112,19.9374909859022));
#35359=CARTESIAN_POINT('Ctrl Pts',(53.2593231581153,19.2732634419551,19.9417085378964));
#35360=CARTESIAN_POINT('Ctrl Pts',(53.3185312176626,19.2174139616768,19.9459260898905));
#35361=CARTESIAN_POINT('Ctrl Pts',(53.3777197280557,19.1615829216263,19.950142249345));
#35362=CARTESIAN_POINT('Ctrl Pts',(53.4397138468037,19.1086822773503,19.9543584087994));
#35363=CARTESIAN_POINT('Ctrl Pts',(53.5041865919209,19.0589970380727,19.9585745682538));
#35364=CARTESIAN_POINT('Ctrl Pts',(53.5686578007832,19.0093129826936,19.9627906272457));
#35365=CARTESIAN_POINT('Ctrl Pts',(53.6356071496528,18.9628444628948,19.9670066862376));
#35366=CARTESIAN_POINT('Ctrl Pts',(53.704675851816,18.9198351985645,19.9712227452295));
#35367=CARTESIAN_POINT('Ctrl Pts',(53.7743099254359,18.876473875926,19.975473315358));
#35368=CARTESIAN_POINT('Ctrl Pts',(53.8460978102861,18.8366289697907,19.9797238854865));
#35369=CARTESIAN_POINT('Ctrl Pts',(53.9196450778532,18.8005038094616,19.983974455615));
#35370=CARTESIAN_POINT('Ctrl Pts',(53.9927012640342,18.7646198599128,19.9881966443237));
#35371=CARTESIAN_POINT('Ctrl Pts',(54.0674929537223,18.7324062622766,19.9924188330325));
#35372=CARTESIAN_POINT('Ctrl Pts',(54.143613695683,18.7040137744798,19.9966410217412));
#35373=CARTESIAN_POINT('Ctrl Pts',(54.2205019594944,18.6753350065679,20.0009057825796));
#35374=CARTESIAN_POINT('Ctrl Pts',(54.2987457648483,18.6505549850221,20.0051705434179));
#35375=CARTESIAN_POINT('Ctrl Pts',(54.3779126848174,18.6297768834371,20.0094353042563));
#35376=CARTESIAN_POINT('Ctrl Pts',(54.4570796047866,18.6089987818522,20.0137000650946));
#35377=CARTESIAN_POINT('Ctrl Pts',(54.5371691546353,18.5922226361211,20.0179648259329));
#35378=CARTESIAN_POINT('Ctrl Pts',(54.6177424854411,18.5794981011031,20.0222295867713));
#35379=CARTESIAN_POINT('Ctrl Pts',(54.6976821412072,18.566873639151,20.0264608070762));
#35380=CARTESIAN_POINT('Ctrl Pts',(54.7783977531393,18.5581899016551,20.0306920273812));
#35381=CARTESIAN_POINT('Ctrl Pts',(54.8594667097273,18.5535330281557,20.0349232476861));
#35382=CARTESIAN_POINT('Ctrl Pts',(54.9404194191055,18.548882832287,20.0391484007172));
#35383=CARTESIAN_POINT('Ctrl Pts',(55.0217240066113,18.5482480587764,20.0433735537484));
#35384=CARTESIAN_POINT('Ctrl Pts',(55.1029496093053,18.5516634978125,20.0475987067796));
#35385=CARTESIAN_POINT('Ctrl Pts',(55.1843838773027,18.5550877109739,20.0518347140588));
#35386=CARTESIAN_POINT('Ctrl Pts',(55.2657382869153,18.5625830402717,20.056070721338));
#35387=CARTESIAN_POINT('Ctrl Pts',(55.346575438063,18.5741319665465,20.0603067286171));
#35388=CARTESIAN_POINT('Ctrl Pts',(55.4270604008013,18.5856305768723,20.0645242806113));
#35389=CARTESIAN_POINT('Ctrl Pts',(55.5070321384962,18.6011474786276,20.0687418326055));
#35390=CARTESIAN_POINT('Ctrl Pts',(55.5860627501174,18.620613376745,20.0729593845996));
#35391=CARTESIAN_POINT('Ctrl Pts',(55.6650672676286,18.6400728476657,20.0771755440541));
#35392=CARTESIAN_POINT('Ctrl Pts',(55.7431308250737,18.6634786145446,20.0813917035085));
#35393=CARTESIAN_POINT('Ctrl Pts',(55.8198366508486,18.6907104737765,20.0856078629629));
#35394=CARTESIAN_POINT('Ctrl Pts',(55.8965406488791,18.7179416841284,20.0898239219548));
#35395=CARTESIAN_POINT('Ctrl Pts',(55.9718865418039,18.7489986489792,20.0940399809467));
#35396=CARTESIAN_POINT('Ctrl Pts',(56.0454750055611,18.7837120532866,20.0982560399386));
#35397=CARTESIAN_POINT('Ctrl Pts',(56.1196658379113,18.8187096089873,20.1025066100671));
#35398=CARTESIAN_POINT('Ctrl Pts',(56.1920698962164,18.8574235508832,20.1067571801956));
#35399=CARTESIAN_POINT('Ctrl Pts',(56.2623024682511,18.8996327157739,20.111007750324));
#35400=CARTESIAN_POINT('Ctrl Pts',(56.3320660914049,18.9415600464663,20.1152299390328));
#35401=CARTESIAN_POINT('Ctrl Pts',(56.3996867829558,18.9869357535491,20.1194521277415));
#35402=CARTESIAN_POINT('Ctrl Pts',(56.464817484026,19.0355000665585,20.1236743164503));
#35403=CARTESIAN_POINT('Ctrl Pts',(56.5306048948826,19.0845540512449,20.1279390772886));
#35404=CARTESIAN_POINT('Ctrl Pts',(56.5938514453632,19.1368609952995,20.1322038381269));
#35405=CARTESIAN_POINT('Ctrl Pts',(56.6542359740413,19.1921135012984,20.1364685989653));
#35406=CARTESIAN_POINT('Ctrl Pts',(56.7146205027195,19.2473660072973,20.1407333598036));
#35407=CARTESIAN_POINT('Ctrl Pts',(56.7721427166022,19.3055636874104,20.1449981206419));
#35408=CARTESIAN_POINT('Ctrl Pts',(56.8265229404517,19.3663647291994,20.1492628814802));
#35409=CARTESIAN_POINT('Ctrl Pts',(56.8804754869275,19.4266875966076,20.1534941017852));
#35410=CARTESIAN_POINT('Ctrl Pts',(56.9315376377036,19.4897991966869,20.1577253220901));
#35411=CARTESIAN_POINT('Ctrl Pts',(56.979407866102,19.5553911430379,20.161956542395));
#35412=CARTESIAN_POINT('Ctrl Pts',(57.0272094519435,19.6208890351287,20.1661816954262));
#35413=CARTESIAN_POINT('Ctrl Pts',(57.0718279338929,19.688859837356,20.1704068484573));
#35414=CARTESIAN_POINT('Ctrl Pts',(57.1130004567089,19.758960387438,20.1746320014885));
#35415=CARTESIAN_POINT('Ctrl Pts',(57.1542787500784,19.8292410230109,20.1788680087677));
#35416=CARTESIAN_POINT('Ctrl Pts',(57.1920930467087,19.9016620068143,20.1831040160469));
#35417=CARTESIAN_POINT('Ctrl Pts',(57.2262208989421,19.9758463205586,20.1873400233261));
#35418=CARTESIAN_POINT('Ctrl Pts',(57.2602000641693,20.0497074307376,20.1915575753202));
#35419=CARTESIAN_POINT('Ctrl Pts',(57.2905246369787,20.1253161164419,20.1957751273144));
#35420=CARTESIAN_POINT('Ctrl Pts',(57.3170208242543,20.2022752667919,20.1999926793085));
#35421=CARTESIAN_POINT('Ctrl Pts',(57.3435082630916,20.2792090069812,20.2042088387629));
#35422=CARTESIAN_POINT('Ctrl Pts',(57.3661696753829,20.3574918870836,20.2084249982174));
#35423=CARTESIAN_POINT('Ctrl Pts',(57.3848800777843,20.4367085438358,20.2126411576718));
#35424=CARTESIAN_POINT('Ctrl Pts',(57.4035900343547,20.5159233130157,20.2168572166637));
#35425=CARTESIAN_POINT('Ctrl Pts',(57.4183490624273,20.5960713618798,20.2210732756556));
#35426=CARTESIAN_POINT('Ctrl Pts',(57.4290829042632,20.6767253579134,20.2252893346475));
#35427=CARTESIAN_POINT('Ctrl Pts',(57.4399046094526,20.7580395584361,20.229539904776));
#35428=CARTESIAN_POINT('Ctrl Pts',(57.4466348476017,20.8398675539549,20.2337904749044));
#35429=CARTESIAN_POINT('Ctrl Pts',(57.4492508484847,20.9217661761336,20.2380410450329));
#35430=CARTESIAN_POINT('Ctrl Pts',(57.4518493821065,21.0031179542183,20.2422632337417));
#35431=CARTESIAN_POINT('Ctrl Pts',(57.4503885236005,21.0845389503526,20.2464854224504));
#35432=CARTESIAN_POINT('Ctrl Pts',(57.4448983583969,21.1655967001733,20.2507076111592));
#35433=CARTESIAN_POINT('Ctrl Pts',(57.4393528361164,21.2474717514617,20.2549723719975));
#35434=CARTESIAN_POINT('Ctrl Pts',(57.4296963523323,21.3289757075925,20.2592371328358));
#35435=CARTESIAN_POINT('Ctrl Pts',(57.4160130524944,21.4096720397793,20.2635018936742));
#35436=CARTESIAN_POINT('Ctrl Pts',(57.4023297526564,21.490368371966,20.2677666545125));
#35437=CARTESIAN_POINT('Ctrl Pts',(57.3846198037662,21.5702566237358,20.2720314153508));
#35438=CARTESIAN_POINT('Ctrl Pts',(57.3630187627035,21.648916463893,20.2762961761892));
#35439=CARTESIAN_POINT('Ctrl Pts',(57.3415876046581,21.726957677802,20.2805273964941));
#35440=CARTESIAN_POINT('Ctrl Pts',(57.3162460191148,21.8040823907584,20.284758616799));
#35441=CARTESIAN_POINT('Ctrl Pts',(57.2870896288855,21.8798700355419,20.2889898371039));
#35442=CARTESIAN_POINT('Ctrl Pts',(57.2579750468791,21.9555490061471,20.2932149901351));
#35443=CARTESIAN_POINT('Ctrl Pts',(57.2250566898657,22.0298942861481,20.2974401431662));
#35444=CARTESIAN_POINT('Ctrl Pts',(57.1884803690812,22.1024989451906,20.3016652961974));
#35445=CARTESIAN_POINT('Ctrl Pts',(57.1518100852009,22.1752901226793,20.3059013034766));
#35446=CARTESIAN_POINT('Ctrl Pts',(57.1114631503549,22.2463312711302,20.3101373107558));
#35447=CARTESIAN_POINT('Ctrl Pts',(57.0676357326681,22.3152310546037,20.314373318035));
#35448=CARTESIAN_POINT('Ctrl Pts',(57.0239992607075,22.3838306579643,20.3185908700291));
#35449=CARTESIAN_POINT('Ctrl Pts',(56.9769128141619,22.4503071171187,20.3228084220233));
#35450=CARTESIAN_POINT('Ctrl Pts',(56.9266158252163,22.5142990827529,20.3270259740174));
#35451=CARTESIAN_POINT('Ctrl Pts',(56.8763354431922,22.5782699196958,20.3312421334719));
#35452=CARTESIAN_POINT('Ctrl Pts',(56.8228469109498,22.6397575269245,20.3354582929263));
#35453=CARTESIAN_POINT('Ctrl Pts',(56.7664314626968,22.6984316699811,20.3396744523807));
#35454=CARTESIAN_POINT('Ctrl Pts',(56.7100173587095,22.7571044149518,20.3438905113726));
#35455=CARTESIAN_POINT('Ctrl Pts',(56.6506768004122,22.8129634946732,20.3481065703645));
#35456=CARTESIAN_POINT('Ctrl Pts',(56.5887285835314,22.8657148061454,20.3523226293564));
#35457=CARTESIAN_POINT('Ctrl Pts',(56.5262732809154,22.918897920806,20.3565731994849));
#35458=CARTESIAN_POINT('Ctrl Pts',(56.4611677867953,22.9689218310047,20.3608237696134));
#35459=CARTESIAN_POINT('Ctrl Pts',(56.3937721203693,23.0155271088431,20.3650743397419));
#35460=CARTESIAN_POINT('Ctrl Pts',(56.3268264605633,23.0618211992614,20.3692965284506));
#35461=CARTESIAN_POINT('Ctrl Pts',(56.2576215502471,23.1047419763653,20.3735187171594));
#35462=CARTESIAN_POINT('Ctrl Pts',(56.1865370742528,23.1440802273757,20.3777409058681));
#35463=CARTESIAN_POINT('Ctrl Pts',(56.1147358568401,23.1838151241156,20.3820056667065));
#35464=CARTESIAN_POINT('Ctrl Pts',(56.0410173936067,23.2198946296911,20.3862704275448));
#35465=CARTESIAN_POINT('Ctrl Pts',(55.96579409698,23.2521527506452,20.3905351883831));
#35466=CARTESIAN_POINT('Ctrl Pts',(55.8905708003533,23.2844108715993,20.3947999492215));
#35467=CARTESIAN_POINT('Ctrl Pts',(55.8138431444299,23.312847500743,20.3990647100598));
#35468=CARTESIAN_POINT('Ctrl Pts',(55.7360378082485,23.3373486250084,20.4033294708982));
#35469=CARTESIAN_POINT('Ctrl Pts',(55.6588443780043,23.3616570583334,20.4075606912031));
#35470=CARTESIAN_POINT('Ctrl Pts',(55.5803007050971,23.3821828653269,20.411791911508));
#35471=CARTESIAN_POINT('Ctrl Pts',(55.5008120137583,23.3987783509269,20.416023131813));
#35472=CARTESIAN_POINT('Ctrl Pts',(55.4214373036394,23.415350039762,20.4202482848441));
#35473=CARTESIAN_POINT('Ctrl Pts',(55.341120717669,23.4280025061218,20.4244734378753));
#35474=CARTESIAN_POINT('Ctrl Pts',(55.2602832351607,23.4366376192397,20.4286985909065));
#35475=CARTESIAN_POINT('Ctrl Pts',(55.1792380844143,23.4452949156156,20.4329345981857));
#35476=CARTESIAN_POINT('Ctrl Pts',(55.097669809526,23.4499140558417,20.4371706054649));
#35477=CARTESIAN_POINT('Ctrl Pts',(55.0160135914354,23.4504476764235,20.4414066127441));
#35478=CARTESIAN_POINT('Ctrl Pts',(54.9347131302358,23.4509789721462,20.4456241647382));
#35479=CARTESIAN_POINT('Ctrl Pts',(54.8533259583399,23.4474602620402,20.4498417167324));
#35480=CARTESIAN_POINT('Ctrl Pts',(54.772285519582,23.4398967940075,20.4540592687265));
#35481=CARTESIAN_POINT('Ctrl Pts',(54.6912718385334,23.4323358232598,20.458275428181));
#35482=CARTESIAN_POINT('Ctrl Pts',(54.6106051258215,23.4207327898445,20.4624915876354));
#35483=CARTESIAN_POINT('Ctrl Pts',(54.5307153474474,23.4051449363559,20.4667077470899));
#35484=CARTESIAN_POINT('Ctrl Pts',(54.4508274726848,23.3895574542943,20.4709238060818));
#35485=CARTESIAN_POINT('Ctrl Pts',(54.3717169515563,23.3699854310681,20.4751398650737));
#35486=CARTESIAN_POINT('Ctrl Pts',(54.2938037578098,23.3465372610544,20.4793559240656));
#35487=CARTESIAN_POINT('Ctrl Pts',(54.2152527947924,23.3228971527876,20.483606494194));
#35488=CARTESIAN_POINT('Ctrl Pts',(54.1379193154039,23.2953172702312,20.4878570643225));
#35489=CARTESIAN_POINT('Ctrl Pts',(54.0622165104119,23.2639594467781,20.492107634451));
#35490=CARTESIAN_POINT('Ctrl Pts',(53.9870191795132,23.23281100219,20.4963298231597));
#35491=CARTESIAN_POINT('Ctrl Pts',(53.9134312108186,23.197935171268,20.5005520118685));
#35492=CARTESIAN_POINT('Ctrl Pts',(53.8418342657123,23.1595375389008,20.5047742005772));
#35493=CARTESIAN_POINT('Ctrl Pts',(53.769515411986,23.1207527450179,20.5090389614156));
#35494=CARTESIAN_POINT('Ctrl Pts',(53.6992283746618,23.0783749804686,20.5133037222539));
#35495=CARTESIAN_POINT('Ctrl Pts',(53.6313362463376,23.0326607634848,20.5175684830922));
#35496=CARTESIAN_POINT('Ctrl Pts',(53.5634441180134,22.9869465465011,20.5218332439305));
#35497=CARTESIAN_POINT('Ctrl Pts',(53.4979472458188,22.9378962173154,20.5260980047689));
#35498=CARTESIAN_POINT('Ctrl Pts',(53.4351727822584,22.8858064663732,20.5303627656072));
#35499=CARTESIAN_POINT('Ctrl Pts',(53.3737435940809,22.8348330142518,20.5345361313551));
#35500=CARTESIAN_POINT('Ctrl Pts',(53.3146772603322,22.7807463896056,20.5387094971031));
#35501=CARTESIAN_POINT('Ctrl Pts',(53.2583127972822,22.723796953788,20.542882862851));
#35502=CARTESIAN_POINT('Ctrl Pts',(53.2020418709362,22.6669420254356,20.5470493029076));
#35503=CARTESIAN_POINT('Ctrl Pts',(53.1484642415818,22.6072340609324,20.5512157429641));
#35504=CARTESIAN_POINT('Ctrl Pts',(53.0978860992566,22.5449637402214,20.5553821830207));
#35505=CARTESIAN_POINT('Ctrl Pts',(53.0473552090205,22.4827515948921,20.5595447306251));
#35506=CARTESIAN_POINT('Ctrl Pts',(52.9998185486412,22.4179822101817,20.5637072782296));
#35507=CARTESIAN_POINT('Ctrl Pts',(52.9555448532792,22.3509823844324,20.567869825834));
#35508=CARTESIAN_POINT('Ctrl Pts',(52.9112980752924,22.2840232930162,20.5720298427065));
#35509=CARTESIAN_POINT('Ctrl Pts',(52.8703105898291,22.2148368494016,20.576189859579));
#35510=CARTESIAN_POINT('Ctrl Pts',(52.8328092765498,22.1437808436022,20.5803498764515));
#35511=CARTESIAN_POINT('Ctrl Pts',(52.7953185310003,22.0727448611197,20.5845087210468));
#35512=CARTESIAN_POINT('Ctrl Pts',(52.7613122300788,21.999840785893,20.5886675656421));
#35513=CARTESIAN_POINT('Ctrl Pts',(52.7309717177786,21.9254517299565,20.5928264102373));
#35514=CARTESIAN_POINT('Ctrl Pts',(52.7006122507968,21.8510162008142,20.5969878529949));
#35515=CARTESIAN_POINT('Ctrl Pts',(52.6739233341779,21.7750942796353,20.6011492957525));
#35516=CARTESIAN_POINT('Ctrl Pts',(52.6510381008611,21.6980889960411,20.6053107385101));
#35517=CARTESIAN_POINT('Ctrl Pts',(52.6281465986378,21.6210626185426,20.6094733212034));
#35518=CARTESIAN_POINT('Ctrl Pts',(52.6090609727083,21.5429527524677,20.6136359038967));
#35519=CARTESIAN_POINT('Ctrl Pts',(52.5938637359314,21.4641751056811,20.6177984865901));
#35520=CARTESIAN_POINT('Ctrl Pts',(52.5786432827025,21.3852771121837,20.6219674283606));
#35521=CARTESIAN_POINT('Ctrl Pts',(52.5673231569836,21.3057097746646,20.6261363701311));
#35522=CARTESIAN_POINT('Ctrl Pts',(52.5599341697403,21.2258959804843,20.6303053119016));
#35523=CARTESIAN_POINT('Ctrl Pts',(52.5529230756155,21.1501640831302,20.6342610425303));
#35524=CARTESIAN_POINT('Ctrl Pts',(52.5494508847733,21.0742106786019,20.6382167731591));
#35525=CARTESIAN_POINT('Ctrl Pts',(52.5495005252726,20.9983955185562,20.6421725037879));
#35526=CARTESIAN_POINT('',(52.5495008698404,21.0020647244182,21.442172503788));
#35527=CARTESIAN_POINT('Ctrl Pts',(52.5468288761996,20.9983937692755,20.6421725037879));
#35528=CARTESIAN_POINT('Ctrl Pts',(52.5460903334207,20.9010294596174,20.6472470226307));
#35529=CARTESIAN_POINT('Ctrl Pts',(52.5955624235799,19.9919636142317,20.6946659730428));
#35530=CARTESIAN_POINT('Ctrl Pts',(53.7309516898259,18.396268298246,20.7844293550254));
#35531=CARTESIAN_POINT('Ctrl Pts',(56.4996417677023,18.5219005353188,20.9114626497339));
#35532=CARTESIAN_POINT('Ctrl Pts',(57.8953253383877,20.9163724138012,21.0384959444432));
#35533=CARTESIAN_POINT('Ctrl Pts',(56.6401754796155,23.3874100578551,21.165529239152));
#35534=CARTESIAN_POINT('Ctrl Pts',(53.8833525846904,23.6726393206288,21.2925625338611));
#35535=CARTESIAN_POINT('Ctrl Pts',(52.6242883163623,22.1034286881138,21.3847769554064));
#35536=CARTESIAN_POINT('Ctrl Pts',(52.5468214014796,21.1466563462855,21.434646945382));
#35537=CARTESIAN_POINT('Ctrl Pts',(52.5481225970323,21.0020658857137,21.442172503788));
#35538=CARTESIAN_POINT('',(52.5495000224195,21.0003314787029,22.2421725037548));
#35539=CARTESIAN_POINT('Ctrl Pts',(52.5495008698404,21.0020647244182,21.442172503788));
#35540=CARTESIAN_POINT('Ctrl Pts',(52.5494304515662,20.918489445297,21.4465248629335));
#35541=CARTESIAN_POINT('Ctrl Pts',(52.5536406367923,20.8347652266227,21.4508772220789));
#35542=CARTESIAN_POINT('Ctrl Pts',(52.5621453286912,20.7513740729974,21.4552295812244));
#35543=CARTESIAN_POINT('Ctrl Pts',(52.5702688987333,20.671719937914,21.4593868975371));
#35544=CARTESIAN_POINT('Ctrl Pts',(52.5823103019167,20.59237020044,21.4635442138498));
#35545=CARTESIAN_POINT('Ctrl Pts',(52.5982284637294,20.5137451927636,21.4677015301625));
#35546=CARTESIAN_POINT('Ctrl Pts',(52.6141376778356,20.4351643807365,21.4718565096196));
#35547=CARTESIAN_POINT('Ctrl Pts',(52.6339192331866,20.3573079598964,21.4760114890767));
#35548=CARTESIAN_POINT('Ctrl Pts',(52.6574805417972,20.2805885475327,21.4801664685337));
#35549=CARTESIAN_POINT('Ctrl Pts',(52.6810363253825,20.2038871255404,21.484320473666));
#35550=CARTESIAN_POINT('Ctrl Pts',(52.7083699617319,20.1283226413996,21.4884744787983));
#35551=CARTESIAN_POINT('Ctrl Pts',(52.7393387648728,20.0542933700172,21.4926284839306));
#35552=CARTESIAN_POINT('Ctrl Pts',(52.770310451467,19.980257205894,21.4967828758354));
#35553=CARTESIAN_POINT('Ctrl Pts',(52.8049177886942,19.9077569799207,21.5009372677401));
#35554=CARTESIAN_POINT('Ctrl Pts',(52.8429702805564,19.8371702448609,21.5050916596448));
#35555=CARTESIAN_POINT('Ctrl Pts',(52.8810619410912,19.7665108525694,21.5092503278008));
#35556=CARTESIAN_POINT('Ctrl Pts',(52.9226056021255,19.6977693032916,21.5134089959568));
#35557=CARTESIAN_POINT('Ctrl Pts',(52.9673656338089,19.6312970434097,21.5175676641128));
#35558=CARTESIAN_POINT('Ctrl Pts',(53.0121527784242,19.5647845186356,21.5217288513396));
#35559=CARTESIAN_POINT('Ctrl Pts',(53.0601598798022,19.5005443998092,21.5258900385663));
#35560=CARTESIAN_POINT('Ctrl Pts',(53.1111105325369,19.4388956377913,21.5300512257931));
#35561=CARTESIAN_POINT('Ctrl Pts',(53.1621424293653,19.3771485728562,21.5342190483005));
#35562=CARTESIAN_POINT('Ctrl Pts',(53.2161269149132,19.3180014579987,21.538386870808));
#35563=CARTESIAN_POINT('Ctrl Pts',(53.2727508194675,19.2617363495862,21.5425546933155));
#35564=CARTESIAN_POINT('Ctrl Pts',(53.2912025116041,19.2434015761962,21.5439128366367));
#35565=CARTESIAN_POINT('Ctrl Pts',(53.3099342199554,19.2253725119082,21.5452709799578));
#35566=CARTESIAN_POINT('Ctrl Pts',(53.3289343994194,19.2076579543636,21.546629123279));
#35567=CARTESIAN_POINT('Ctrl Pts',(53.3881284063353,19.1524692313414,21.5508603435839));
#35568=CARTESIAN_POINT('Ctrl Pts',(53.4501703342923,19.1001126034721,21.5550915638888));
#35569=CARTESIAN_POINT('Ctrl Pts',(53.5147580996481,19.0508959115945,21.5593227841938));
#35570=CARTESIAN_POINT('Ctrl Pts',(53.5792532506689,19.0017497930083,21.5635479372249));
#35571=CARTESIAN_POINT('Ctrl Pts',(53.6462866221427,18.9557349476237,21.5677730902561));
#35572=CARTESIAN_POINT('Ctrl Pts',(53.7155205621037,18.913121272421,21.5719982432872));
#35573=CARTESIAN_POINT('Ctrl Pts',(53.7849323612694,18.8703981244022,21.5762342505664));
#35574=CARTESIAN_POINT('Ctrl Pts',(53.8565557001205,18.8310939610539,21.5804702578456));
#35575=CARTESIAN_POINT('Ctrl Pts',(53.9300182421362,18.7954389806951,21.5847062651248));
#35576=CARTESIAN_POINT('Ctrl Pts',(54.0031607251758,18.7599393406797,21.588923817119));
#35577=CARTESIAN_POINT('Ctrl Pts',(54.078126001508,18.7280573643538,21.5931413691131));
#35578=CARTESIAN_POINT('Ctrl Pts',(54.154520639949,18.6999750214992,21.5973589211073));
#35579=CARTESIAN_POINT('Ctrl Pts',(54.2308900546184,18.6719019507953,21.6015750805617));
#35580=CARTESIAN_POINT('Ctrl Pts',(54.3086874581541,18.6476261824804,21.6057912400162));
#35581=CARTESIAN_POINT('Ctrl Pts',(54.3875001613117,18.6272812645392,21.6100073994706));
#35582=CARTESIAN_POINT('Ctrl Pts',(54.4663109865222,18.6069368313761,21.6142234584625));
#35583=CARTESIAN_POINT('Ctrl Pts',(54.5461366128117,18.5905231774913,21.6184395174544));
#35584=CARTESIAN_POINT('Ctrl Pts',(54.6265513350359,18.5781233836885,21.6226555764463));
#35585=CARTESIAN_POINT('Ctrl Pts',(54.7076243031402,18.5656220896509,21.6269061465748));
#35586=CARTESIAN_POINT('Ctrl Pts',(54.7892955842799,18.5572007599945,21.6311567167032));
#35587=CARTESIAN_POINT('Ctrl Pts',(54.8711225759084,18.5528913265734,21.6354072868317));
#35588=CARTESIAN_POINT('Ctrl Pts',(54.9524032017264,18.5486106676073,21.6396294755405));
#35589=CARTESIAN_POINT('Ctrl Pts',(55.0338369953068,18.5483871006073,21.6438516642492));
#35590=CARTESIAN_POINT('Ctrl Pts',(55.1149909625191,18.5521994916785,21.648073852958));
#35591=CARTESIAN_POINT('Ctrl Pts',(55.1969632013544,18.556050322909,21.6523386137963));
#35592=CARTESIAN_POINT('Ctrl Pts',(55.2786494556059,18.5640189118933,21.6566033746346));
#35593=CARTESIAN_POINT('Ctrl Pts',(55.3596115494113,18.5760301603506,21.660868135473));
#35594=CARTESIAN_POINT('Ctrl Pts',(55.4405736432166,18.5880414088078,21.6651328963113));
#35595=CARTESIAN_POINT('Ctrl Pts',(55.5208111167463,18.604095159214,21.6693976571496));
#35596=CARTESIAN_POINT('Ctrl Pts',(55.5999009248688,18.6240645778259,21.673662417988));
#35597=CARTESIAN_POINT('Ctrl Pts',(55.6783687252279,18.6438769454385,21.6778936382929));
#35598=CARTESIAN_POINT('Ctrl Pts',(55.7560011040426,18.6676178608814,21.6821248585978));
#35599=CARTESIAN_POINT('Ctrl Pts',(55.832375606204,18.6952004208182,21.6863560789028));
#35600=CARTESIAN_POINT('Ctrl Pts',(55.9086405926748,18.7227434292946,21.6905812319339));
#35601=CARTESIAN_POINT('Ctrl Pts',(55.9836508512003,18.7541169850837,21.6948063849651));
#35602=CARTESIAN_POINT('Ctrl Pts',(56.0569965225224,18.7891837250971,21.6990315379963));
#35603=CARTESIAN_POINT('Ctrl Pts',(56.1305306159211,18.8243405501538,21.7032675452755));
#35604=CARTESIAN_POINT('Ctrl Pts',(56.2023911025759,18.8632094372283,21.7075035525547));
#35605=CARTESIAN_POINT('Ctrl Pts',(56.2721826727244,18.9056023545611,21.7117395598339));
#35606=CARTESIAN_POINT('Ctrl Pts',(56.3416701774559,18.9478105759477,21.715957111828));
#35607=CARTESIAN_POINT('Ctrl Pts',(56.409106351521,18.993511948985,21.7201746638222));
#35608=CARTESIAN_POINT('Ctrl Pts',(56.4741249704932,19.0424745668655,21.7243922158164));
#35609=CARTESIAN_POINT('Ctrl Pts',(56.5391221217966,19.0914210184035,21.7286083752708));
#35610=CARTESIAN_POINT('Ctrl Pts',(56.6017029320628,19.143626296974,21.7328245347253));
#35611=CARTESIAN_POINT('Ctrl Pts',(56.6615314204312,19.19881605911,21.7370406941797));
#35612=CARTESIAN_POINT('Ctrl Pts',(56.7213584832078,19.2540045061857,21.7412567531716));
#35613=CARTESIAN_POINT('Ctrl Pts',(56.7784330135025,19.3121769793841,21.7454728121635));
#35614=CARTESIAN_POINT('Ctrl Pts',(56.83245437726,19.373020834411,21.7496888711554));
#35615=CARTESIAN_POINT('Ctrl Pts',(56.8869179403951,19.4343627352656,21.7539394412839));
#35616=CARTESIAN_POINT('Ctrl Pts',(56.9382777915358,19.4984196056773,21.7581900114123));
#35617=CARTESIAN_POINT('Ctrl Pts',(56.9862671116431,19.5648368694797,21.7624405815408));
#35618=CARTESIAN_POINT('Ctrl Pts',(57.0339360029623,19.6308106595403,21.7666627702496));
#35619=CARTESIAN_POINT('Ctrl Pts',(57.0782790330116,19.6991129904314,21.7708849589583));
#35620=CARTESIAN_POINT('Ctrl Pts',(57.1190791803643,19.7693685859095,21.7751071476671));
#35621=CARTESIAN_POINT('Ctrl Pts',(57.1602907136779,19.8403325652422,21.7793719085054));
#35622=CARTESIAN_POINT('Ctrl Pts',(57.1978872941892,19.9132889883853,21.7836366693437));
#35623=CARTESIAN_POINT('Ctrl Pts',(57.231694433609,19.9878289645527,21.787901430182));
#35624=CARTESIAN_POINT('Ctrl Pts',(57.2655015730289,20.0623689407201,21.7921661910204));
#35625=CARTESIAN_POINT('Ctrl Pts',(57.2955191543851,20.1384919981338,21.7964309518587));
#35626=CARTESIAN_POINT('Ctrl Pts',(57.3216243635664,20.2157739072852,21.800695712697));
#35627=CARTESIAN_POINT('Ctrl Pts',(57.3475242663604,20.292448027031,21.8049269330019));
#35628=CARTESIAN_POINT('Ctrl Pts',(57.3696702805044,20.3705503404663,21.8091581533068));
#35629=CARTESIAN_POINT('Ctrl Pts',(57.3879063608704,20.4496787649792,21.8133893736117));
#35630=CARTESIAN_POINT('Ctrl Pts',(57.4061162919734,20.5286937248694,21.8176145266429));
#35631=CARTESIAN_POINT('Ctrl Pts',(57.4204273208408,20.6087314243591,21.821839679674));
#35632=CARTESIAN_POINT('Ctrl Pts',(57.4307326301583,20.6893730039358,21.8260648327052));
#35633=CARTESIAN_POINT('Ctrl Pts',(57.4410644134005,20.7702217484844,21.8303008399844));
#35634=CARTESIAN_POINT('Ctrl Pts',(57.4473697247112,20.8516770305352,21.8345368472636));
#35635=CARTESIAN_POINT('Ctrl Pts',(57.44959220944,20.933304741917,21.8387728545428));
#35636=CARTESIAN_POINT('Ctrl Pts',(57.4518050113268,21.0145768206044,21.8429904065369));
#35637=CARTESIAN_POINT('Ctrl Pts',(57.4499704673567,21.0960193618123,21.847207958531));
#35638=CARTESIAN_POINT('Ctrl Pts',(57.4440848589507,21.1771989058883,21.8514255105252));
#35639=CARTESIAN_POINT('Ctrl Pts',(57.4382011938387,21.2583516463257,21.8556416699796));
#35640=CARTESIAN_POINT('Ctrl Pts',(57.4282691541085,21.3392410987342,21.8598578294341));
#35641=CARTESIAN_POINT('Ctrl Pts',(57.4143370766855,21.4194362050917,21.8640739888885));
#35642=CARTESIAN_POINT('Ctrl Pts',(57.4004053312357,21.4996294005622,21.8682900478804));
#35643=CARTESIAN_POINT('Ctrl Pts',(57.3824738182696,21.5791278250063,21.8725061068723));
#35644=CARTESIAN_POINT('Ctrl Pts',(57.3606422222319,21.6575093524931,21.8767221658641));
#35645=CARTESIAN_POINT('Ctrl Pts',(57.3386319206319,21.7365324828623,21.8809727359926));
#35646=CARTESIAN_POINT('Ctrl Pts',(57.3126575051584,21.8144198804118,21.8852233061211));
#35647=CARTESIAN_POINT('Ctrl Pts',(57.2828722281388,21.8907550954065,21.8894738762496));
#35648=CARTESIAN_POINT('Ctrl Pts',(57.2532858299575,21.9665806136517,21.8936960649583));
#35649=CARTESIAN_POINT('Ctrl Pts',(57.2199395547992,22.040874211304,21.8979182536671));
#35650=CARTESIAN_POINT('Ctrl Pts',(57.1830310492812,22.11325005631,21.9021404423758));
#35651=CARTESIAN_POINT('Ctrl Pts',(57.1457503970427,22.1863556635477,21.9064052032142));
#35652=CARTESIAN_POINT('Ctrl Pts',(57.1048355166899,22.2575042061177,21.9106699640525));
#35653=CARTESIAN_POINT('Ctrl Pts',(57.0605353613637,22.3263273632742,21.9149347248909));
#35654=CARTESIAN_POINT('Ctrl Pts',(57.0162352060374,22.3951505204308,21.9191994857292));
#35655=CARTESIAN_POINT('Ctrl Pts',(56.9685501087175,22.4616479380812,21.9234642465676));
#35656=CARTESIAN_POINT('Ctrl Pts',(56.9177699295494,22.525486396962,21.927729007406));
#35657=CARTESIAN_POINT('Ctrl Pts',(56.8673891149322,22.5888227934657,21.9319602277109));
#35658=CARTESIAN_POINT('Ctrl Pts',(56.81377284106,22.649779437751,21.9361914480158));
#35659=CARTESIAN_POINT('Ctrl Pts',(56.7571743408898,22.7080071972092,21.9404226683207));
#35660=CARTESIAN_POINT('Ctrl Pts',(56.7006569990074,22.7661514621358,21.9446478213519));
#35661=CARTESIAN_POINT('Ctrl Pts',(56.6411662452053,22.8215742832384,21.9488729743831));
#35662=CARTESIAN_POINT('Ctrl Pts',(56.578996101381,22.873958794057,21.9530981274142));
#35663=CARTESIAN_POINT('Ctrl Pts',(56.5166662449602,22.9264778785749,21.9573341346934));
#35664=CARTESIAN_POINT('Ctrl Pts',(56.4516435132685,22.9759426568323,21.9615701419726));
#35665=CARTESIAN_POINT('Ctrl Pts',(56.3842621026245,23.0220703947285,21.9658061492518));
#35666=CARTESIAN_POINT('Ctrl Pts',(56.3171742569011,23.0679971649457,21.970023701246));
#35667=CARTESIAN_POINT('Ctrl Pts',(56.2477486232329,23.1106156405142,21.9742412532401));
#35668=CARTESIAN_POINT('Ctrl Pts',(56.1763473934574,23.1496876656635,21.9784588052343));
#35669=CARTESIAN_POINT('Ctrl Pts',(56.1049697387436,23.1887467901191,21.9826749646887));
#35670=CARTESIAN_POINT('Ctrl Pts',(56.0316181908223,23.2242615665046,21.9868911241431));
#35671=CARTESIAN_POINT('Ctrl Pts',(55.9566811492274,23.2560388801421,21.9911072835976));
#35672=CARTESIAN_POINT('Ctrl Pts',(55.8817458932301,23.2878154365908,21.9953233425895));
#35673=CARTESIAN_POINT('Ctrl Pts',(55.8052256471341,23.3158545268721,21.9995394015814));
#35674=CARTESIAN_POINT('Ctrl Pts',(55.7275291471605,23.3400110234851,22.0037554605733));
#35675=CARTESIAN_POINT('Ctrl Pts',(55.6491966516928,23.3643652564569,22.0080060307018));
#35676=CARTESIAN_POINT('Ctrl Pts',(55.5696690100063,23.3847728815998,22.0122566008302));
#35677=CARTESIAN_POINT('Ctrl Pts',(55.4893792346574,23.4011368587996,22.0165071709587));
#35678=CARTESIAN_POINT('Ctrl Pts',(55.4096255609947,23.4173915723263,22.0207293596675));
#35679=CARTESIAN_POINT('Ctrl Pts',(55.3291203737993,23.4296564634265,22.0249515483762));
#35680=CARTESIAN_POINT('Ctrl Pts',(55.2482950311215,23.4378883952143,22.0291737370849));
#35681=CARTESIAN_POINT('Ctrl Pts',(55.1666547303261,23.4462033291819,22.0334384979233));
#35682=CARTESIAN_POINT('Ctrl Pts',(55.0846882666446,23.4504034929406,22.0377032587616));
#35683=CARTESIAN_POINT('Ctrl Pts',(55.0028401040249,23.4504983541739,22.0419680196));
#35684=CARTESIAN_POINT('Ctrl Pts',(54.9209919414053,23.4505932154072,22.0462327804383));
#35685=CARTESIAN_POINT('Ctrl Pts',(54.8392625579176,23.4465828618997,22.0504975412766));
#35686=CARTESIAN_POINT('Ctrl Pts',(54.7580891046741,23.4385301656372,22.054762302115));
#35687=CARTESIAN_POINT('Ctrl Pts',(54.6775540461783,23.4305408004121,22.0589935224199));
#35688=CARTESIAN_POINT('Ctrl Pts',(54.5972642030111,23.4185425342583,22.0632247427249));
#35689=CARTESIAN_POINT('Ctrl Pts',(54.5176502371787,23.4025588351394,22.0674559630298));
#35690=CARTESIAN_POINT('Ctrl Pts',(54.4381504322012,23.3865980555262,22.071681116061));
#35691=CARTESIAN_POINT('Ctrl Pts',(54.3593250317129,23.3666632837747,22.0759062690921));
#35692=CARTESIAN_POINT('Ctrl Pts',(54.2815997032149,23.3428297555689,22.0801314221233));
#35693=CARTESIAN_POINT('Ctrl Pts',(54.2036747014774,23.3189349999888,22.0843674294025));
#35694=CARTESIAN_POINT('Ctrl Pts',(54.1268559001192,23.2911214838037,22.0886034366817));
#35695=CARTESIAN_POINT('Ctrl Pts',(54.0515620708741,23.2595167059784,22.0928394439609));
#35696=CARTESIAN_POINT('Ctrl Pts',(53.9765962790917,23.2280496227188,22.097056995955));
#35697=CARTESIAN_POINT('Ctrl Pts',(53.9031426338185,23.1928244177353,22.1012745479492));
#35698=CARTESIAN_POINT('Ctrl Pts',(53.8315976302803,23.1540162841616,22.1054920999434));
#35699=CARTESIAN_POINT('Ctrl Pts',(53.7600762492746,23.1152209641508,22.1097082593978));
#35700=CARTESIAN_POINT('Ctrl Pts',(53.6904626668853,23.072845286326,22.1139244188523));
#35701=CARTESIAN_POINT('Ctrl Pts',(53.6231297436042,23.0271108867184,22.1181405783067));
#35702=CARTESIAN_POINT('Ctrl Pts',(53.5557984247301,22.981377576869,22.1223566372986));
#35703=CARTESIAN_POINT('Ctrl Pts',(53.4907480408866,22.9322859665042,22.1265726962905));
#35704=CARTESIAN_POINT('Ctrl Pts',(53.428322159038,22.8801007989544,22.1307887552824));
#35705=CARTESIAN_POINT('Ctrl Pts',(53.3653852814616,22.8274884624663,22.1350393254109));
#35706=CARTESIAN_POINT('Ctrl Pts',(53.3051164490023,22.7717319849042,22.1392898955393));
#35707=CARTESIAN_POINT('Ctrl Pts',(53.2478319870599,22.7131425814653,22.1435404656678));
#35708=CARTESIAN_POINT('Ctrl Pts',(53.1909300183614,22.654944384476,22.1477626543766));
#35709=CARTESIAN_POINT('Ctrl Pts',(53.1369729525433,22.5939513703889,22.1519848430853));
#35710=CARTESIAN_POINT('Ctrl Pts',(53.0862309264975,22.5305025917343,22.1562070317941));
#35711=CARTESIAN_POINT('Ctrl Pts',(53.0349772709971,22.466414062038,22.1604717926324));
#35712=CARTESIAN_POINT('Ctrl Pts',(52.9870041383326,22.3998203604865,22.1647365534707));
#35713=CARTESIAN_POINT('Ctrl Pts',(52.9425445714796,22.331100074995,22.169001314309));
#35714=CARTESIAN_POINT('Ctrl Pts',(52.8980850046265,22.2623797895035,22.1732660751474));
#35715=CARTESIAN_POINT('Ctrl Pts',(52.8571391890453,22.191533369362,22.1775308359857));
#35716=CARTESIAN_POINT('Ctrl Pts',(52.8198913303488,22.1189622149616,22.181795596824));
#35717=CARTESIAN_POINT('Ctrl Pts',(52.7805832678882,22.0423771018883,22.1862962444123));
#35718=CARTESIAN_POINT('Ctrl Pts',(52.7452605276227,21.9636134198769,22.1907968920006));
#35719=CARTESIAN_POINT('Ctrl Pts',(52.7141540642048,21.8830960354393,22.1952975395889));
#35720=CARTESIAN_POINT('Ctrl Pts',(52.68314566471,21.8028324841196,22.1997839987704));
#35721=CARTESIAN_POINT('Ctrl Pts',(52.6563271933403,21.7208265945311,22.2042704579518));
#35722=CARTESIAN_POINT('Ctrl Pts',(52.6338824286974,21.6375248142409,22.2087569171332));
#35723=CARTESIAN_POINT('Ctrl Pts',(52.6114813847721,21.5543852995692,22.2132346370288));
#35724=CARTESIAN_POINT('Ctrl Pts',(52.593437190479,21.4699552777701,22.2177123569243));
#35725=CARTESIAN_POINT('Ctrl Pts',(52.5798849594671,21.3846991559471,22.2221900768198));
#35726=CARTESIAN_POINT('Ctrl Pts',(52.5663684050419,21.2996674729948,22.2266560090059));
#35727=CARTESIAN_POINT('Ctrl Pts',(52.5573203157249,21.2138143915247,22.2311219411919));
#35728=CARTESIAN_POINT('Ctrl Pts',(52.5528252148071,21.127615910904,22.235587873378));
#35729=CARTESIAN_POINT('Ctrl Pts',(52.5506160024248,21.0852518451807,22.2377827501703));
#35730=CARTESIAN_POINT('Ctrl Pts',(52.5495057677445,21.0428045501252,22.2399776269625));
#35731=CARTESIAN_POINT('Ctrl Pts',(52.5495000224195,21.000331478703,22.2421725037548));
#35732=CARTESIAN_POINT('',(52.5495010182643,20.9977660545166,23.042172503788));
#35733=CARTESIAN_POINT('Ctrl Pts',(52.5495000224194,21.0003314780632,22.2421725037879));
#35734=CARTESIAN_POINT('Ctrl Pts',(52.5494885746931,20.9157024895623,22.2465458678182));
#35735=CARTESIAN_POINT('Ctrl Pts',(52.5538654945652,20.8311384562012,22.2509192318486));
#35736=CARTESIAN_POINT('Ctrl Pts',(52.5625847018229,20.7471029572889,22.2552925958789));
#35737=CARTESIAN_POINT('Ctrl Pts',(52.5714793432319,20.6613766284642,22.25975395385));
#35738=CARTESIAN_POINT('Ctrl Pts',(52.5848928388564,20.5762007824509,22.2642153118212));
#35739=CARTESIAN_POINT('Ctrl Pts',(52.6027216171688,20.4920564940763,22.2686766697924));
#35740=CARTESIAN_POINT('Ctrl Pts',(52.6202583231078,20.4092906636968,22.2730649414652));
#35741=CARTESIAN_POINT('Ctrl Pts',(52.6420665382094,20.3275232218687,22.277453213138));
#35742=CARTESIAN_POINT('Ctrl Pts',(52.6679975407064,20.2471953906567,22.2818414848108));
#35743=CARTESIAN_POINT('Ctrl Pts',(52.6945763612259,20.1648607794609,22.2863393859312));
#35744=CARTESIAN_POINT('Ctrl Pts',(52.7254865272691,20.0840391011955,22.2908372870515));
#35745=CARTESIAN_POINT('Ctrl Pts',(52.760516573242,20.0051813073348,22.2953351881719));
#35746=CARTESIAN_POINT('Ctrl Pts',(52.7955466192149,19.9263235134742,22.2998330892922));
#35747=CARTESIAN_POINT('Ctrl Pts',(52.8346962709619,19.8494299791551,22.3043309904125));
#35748=CARTESIAN_POINT('Ctrl Pts',(52.8777058399428,19.7749213297967,22.3088288915329));
#35749=CARTESIAN_POINT('Ctrl Pts',(52.918165369112,19.7048303025322,22.3130601118378));
#35750=CARTESIAN_POINT('Ctrl Pts',(52.9621767339345,19.6366143434541,22.3172913321427));
#35751=CARTESIAN_POINT('Ctrl Pts',(53.0095411218324,19.5706561979973,22.3215225524477));
#35752=CARTESIAN_POINT('Ctrl Pts',(53.0568375925131,19.5047926319045,22.3257477054788));
#35753=CARTESIAN_POINT('Ctrl Pts',(53.107477268325,19.4411808238766,22.32997285851));
#35754=CARTESIAN_POINT('Ctrl Pts',(53.1612162242584,19.3801776405823,22.3341980115412));
#35755=CARTESIAN_POINT('Ctrl Pts',(53.215093233406,19.3190177425662,22.3384340188204));
#35756=CARTESIAN_POINT('Ctrl Pts',(53.2720852253751,19.2604802949272,22.3426700260996));
#35757=CARTESIAN_POINT('Ctrl Pts',(53.3319034944793,19.2048943489952,22.3469060333788));
#35758=CARTESIAN_POINT('Ctrl Pts',(53.3914611494878,19.1495505779246,22.3511235853729));
#35759=CARTESIAN_POINT('Ctrl Pts',(53.4538201689723,19.0971329686796,22.3553411373671));
#35760=CARTESIAN_POINT('Ctrl Pts',(53.5186575666153,19.0479306249382,22.3595586893613));
#35761=CARTESIAN_POINT('Ctrl Pts',(53.5834735564246,18.9987445266915,22.3637748488157));
#35762=CARTESIAN_POINT('Ctrl Pts',(53.6507659292892,18.9527718665722,22.3679910082701));
#35763=CARTESIAN_POINT('Ctrl Pts',(53.7201791179804,18.9102610785204,22.3722071677246));
#35764=CARTESIAN_POINT('Ctrl Pts',(53.7895906526959,18.8677513034147,22.3764232267165));
#35765=CARTESIAN_POINT('Ctrl Pts',(53.8611225057065,18.8287034782351,22.3806392857084));
#35766=CARTESIAN_POINT('Ctrl Pts',(53.9343918996012,18.7933215851954,22.3848553447003));
#35767=CARTESIAN_POINT('Ctrl Pts',(54.0082610502981,18.7576500687551,22.3891059148288));
#35768=CARTESIAN_POINT('Ctrl Pts',(54.0838958939356,18.7257050005271,22.3933564849572));
#35769=CARTESIAN_POINT('Ctrl Pts',(54.1608825317766,18.6976463945514,22.3976070550857));
#35770=CARTESIAN_POINT('Ctrl Pts',(54.2373551232628,18.6697751382836,22.4018292437944));
#35771=CARTESIAN_POINT('Ctrl Pts',(54.3151610450022,18.6457386813615,22.4060514325032));
#35772=CARTESIAN_POINT('Ctrl Pts',(54.3938800624636,18.625643482684,22.410273621212));
#35773=CARTESIAN_POINT('Ctrl Pts',(54.4733928000644,18.6053456650663,22.4145383820503));
#35774=CARTESIAN_POINT('Ctrl Pts',(54.5538366742813,18.5890691284264,22.4188031428886));
#35775=CARTESIAN_POINT('Ctrl Pts',(54.6347707087752,18.5768702439136,22.4230679037269));
#35776=CARTESIAN_POINT('Ctrl Pts',(54.7157047432691,18.5646713594007,22.4273326645652));
#35777=CARTESIAN_POINT('Ctrl Pts',(54.7971284522444,18.5565501109006,22.4315974254036));
#35778=CARTESIAN_POINT('Ctrl Pts',(54.8786001934614,18.5525089710129,22.4358621862419));
#35779=CARTESIAN_POINT('Ctrl Pts',(54.9594311940223,18.5484996129747,22.4400934065468));
#35780=CARTESIAN_POINT('Ctrl Pts',(55.0406125788216,18.5484913358027,22.4443246268517));
#35781=CARTESIAN_POINT('Ctrl Pts',(55.1217149510855,18.5525246230693,22.4485558471566));
#35782=CARTESIAN_POINT('Ctrl Pts',(55.202701028224,18.5565521268842,22.4527810001878));
#35783=CARTESIAN_POINT('Ctrl Pts',(55.283607857416,18.5646096622987,22.4570061532189));
#35784=CARTESIAN_POINT('Ctrl Pts',(55.3640033251966,18.5766857757926,22.4612313062501));
#35785=CARTESIAN_POINT('Ctrl Pts',(55.4446053256976,18.5887929123359,22.4654673135293));
#35786=CARTESIAN_POINT('Ctrl Pts',(55.5246928623394,18.6049393174882,22.4697033208085));
#35787=CARTESIAN_POINT('Ctrl Pts',(55.6038329120281,18.6250608293365,22.4739393280877));
#35788=CARTESIAN_POINT('Ctrl Pts',(55.6826281671781,18.6450946765015,22.4781568800818));
#35789=CARTESIAN_POINT('Ctrl Pts',(55.7604837186519,18.6690689580281,22.482374432076));
#35790=CARTESIAN_POINT('Ctrl Pts',(55.8369815210786,18.6968690477151,22.4865919840701));
#35791=CARTESIAN_POINT('Ctrl Pts',(55.9134540656711,18.7246599584448,22.4908081435246));
#35792=CARTESIAN_POINT('Ctrl Pts',(55.9885693148541,18.7562740101354,22.495024302979));
#35793=CARTESIAN_POINT('Ctrl Pts',(56.0619257293278,18.7915471489317,22.4992404624334));
#35794=CARTESIAN_POINT('Ctrl Pts',(56.135280395867,18.8268194472407,22.5034565214253));
#35795=CARTESIAN_POINT('Ctrl Pts',(56.2068758925048,18.8657504568286,22.5076725804172));
#35796=CARTESIAN_POINT('Ctrl Pts',(56.2763332758992,18.9081291581858,22.5118886394091));
#35797=CARTESIAN_POINT('Ctrl Pts',(56.3463592123547,18.9508547562905,22.5161392095375));
#35798=CARTESIAN_POINT('Ctrl Pts',(56.414211452482,18.9970845136542,22.520389779666));
#35799=CARTESIAN_POINT('Ctrl Pts',(56.4795311218914,19.0465574210244,22.5246403497945));
#35800=CARTESIAN_POINT('Ctrl Pts',(56.5444146462899,19.0956999935673,22.5288625385033));
#35801=CARTESIAN_POINT('Ctrl Pts',(56.606798997415,19.1480421892964,22.533084727212));
#35802=CARTESIAN_POINT('Ctrl Pts',(56.6663668643945,19.2032886366342,22.5373069159208));
#35803=CARTESIAN_POINT('Ctrl Pts',(56.7265353513672,19.2590921312946,22.5415716767591));
#35804=CARTESIAN_POINT('Ctrl Pts',(56.7838298984299,19.3178584262345,22.5458364375975));
#35805=CARTESIAN_POINT('Ctrl Pts',(56.8379640335488,19.3792475632038,22.5501011984358));
#35806=CARTESIAN_POINT('Ctrl Pts',(56.8920981686677,19.440636700173,22.5543659592742));
#35807=CARTESIAN_POINT('Ctrl Pts',(56.9430716419734,19.5046482622515,22.5586307201125));
#35808=CARTESIAN_POINT('Ctrl Pts',(56.9906429078337,19.5709125067053,22.5628954809508));
#35809=CARTESIAN_POINT('Ctrl Pts',(57.0378400458841,19.6366556110084,22.5671267012558));
#35810=CARTESIAN_POINT('Ctrl Pts',(57.0818653202519,19.7048625939595,22.5713579215607));
#35811=CARTESIAN_POINT('Ctrl Pts',(57.1224518869003,19.7751946122778,22.5755891418656));
#35812=CARTESIAN_POINT('Ctrl Pts',(57.1629802552527,19.8454257794044,22.5798142948968));
#35813=CARTESIAN_POINT('Ctrl Pts',(57.2000794785399,19.9177755307403,22.5840394479279));
#35814=CARTESIAN_POINT('Ctrl Pts',(57.2335248790578,19.991874578919,22.5882646009591));
#35815=CARTESIAN_POINT('Ctrl Pts',(57.2670561994633,20.0661639845696,22.5925006082383));
#35816=CARTESIAN_POINT('Ctrl Pts',(57.2969146299699,20.1422112991335,22.5967366155175));
#35817=CARTESIAN_POINT('Ctrl Pts',(57.3229192871087,20.2196178913004,22.6009726227967));
#35818=CARTESIAN_POINT('Ctrl Pts',(57.3488106480872,20.2966872411944,22.6051901747908));
#35819=CARTESIAN_POINT('Ctrl Pts',(57.3708815888824,20.3751036083789,22.609407726785));
#35820=CARTESIAN_POINT('Ctrl Pts',(57.3890017491544,20.4544535835172,22.6136252787791));
#35821=CARTESIAN_POINT('Ctrl Pts',(57.4071159265617,20.5337773590989,22.6178414382336));
#35822=CARTESIAN_POINT('Ctrl Pts',(57.4212818104931,20.6140336775829,22.622057597688));
#35823=CARTESIAN_POINT('Ctrl Pts',(57.431419521424,20.6947961978637,22.6262737571424));
#35824=CARTESIAN_POINT('Ctrl Pts',(57.4415569907937,20.7755567937372,22.6304898161343));
#35825=CARTESIAN_POINT('Ctrl Pts',(57.4476664211974,20.8568231059859,22.6347058751262));
#35826=CARTESIAN_POINT('Ctrl Pts',(57.4497196473359,20.9381623136237,22.6389219341181));
#35827=CARTESIAN_POINT('Ctrl Pts',(57.4517896804423,21.0201673346456,22.6431725042466));
#35828=CARTESIAN_POINT('Ctrl Pts',(57.4497367693757,21.1022459707963,22.6474230743751));
#35829=CARTESIAN_POINT('Ctrl Pts',(57.4435856338116,21.1839551582031,22.6516736445035));
#35830=CARTESIAN_POINT('Ctrl Pts',(57.437475569905,21.2651187663879,22.6558958332123));
#35831=CARTESIAN_POINT('Ctrl Pts',(57.4273219630985,21.3459173863507,22.660118021921));
#35832=CARTESIAN_POINT('Ctrl Pts',(57.4132009421555,21.4259242453534,22.6643402106298));
#35833=CARTESIAN_POINT('Ctrl Pts',(57.3989375396244,21.5067378097416,22.6686049714681));
#35834=CARTESIAN_POINT('Ctrl Pts',(57.3806263745226,21.5867430831721,22.6728697323065));
#35835=CARTESIAN_POINT('Ctrl Pts',(57.358397760404,21.6655150289222,22.6771344931448));
#35836=CARTESIAN_POINT('Ctrl Pts',(57.3361691462854,21.7442869746723,22.6813992539832));
#35837=CARTESIAN_POINT('Ctrl Pts',(57.3100232979766,21.8218251567298,22.6856640148215));
#35838=CARTESIAN_POINT('Ctrl Pts',(57.2801399150844,21.8977261373262,22.6899287756598));
#35839=CARTESIAN_POINT('Ctrl Pts',(57.2504915523118,21.9730301889339,22.6941599959648));
#35840=CARTESIAN_POINT('Ctrl Pts',(57.2170530977956,22.0470050972885,22.6983912162697));
#35841=CARTESIAN_POINT('Ctrl Pts',(57.1799645709816,22.1192429223655,22.7026224365747));
#35842=CARTESIAN_POINT('Ctrl Pts',(57.1429292265191,22.1913771634574,22.7068475896058));
#35843=CARTESIAN_POINT('Ctrl Pts',(57.1022544153297,22.2617788581933,22.711072742637));
#35844=CARTESIAN_POINT('Ctrl Pts',(57.0581286005639,22.3300589887449,22.7152978956682));
#35845=CARTESIAN_POINT('Ctrl Pts',(57.0138894283566,22.3985145282026,22.7195339029474));
#35846=CARTESIAN_POINT('Ctrl Pts',(56.9661816777924,22.4648371522518,22.7237699102266));
#35847=CARTESIAN_POINT('Ctrl Pts',(56.9152422140318,22.5286587296027,22.7280059175058));
#35848=CARTESIAN_POINT('Ctrl Pts',(56.8645246815052,22.5922022513878,22.7322234694999));
#35849=CARTESIAN_POINT('Ctrl Pts',(56.8106038221552,22.6532661031908,22.7364410214941));
#35850=CARTESIAN_POINT('Ctrl Pts',(56.7537563129064,22.7115165920729,22.7406585734883));
#35851=CARTESIAN_POINT('Ctrl Pts',(56.696927573412,22.7697478479687,22.7448747329427));
#35852=CARTESIAN_POINT('Ctrl Pts',(56.6371744274441,22.8251672531546,22.7490908923972));
#35853=CARTESIAN_POINT('Ctrl Pts',(56.5748117894574,22.8774765185712,22.7533070518516));
#35854=CARTESIAN_POINT('Ctrl Pts',(56.5124506374458,22.9297845375639,22.7575231108435));
#35855=CARTESIAN_POINT('Ctrl Pts',(56.4474804739603,22.9789822662016,22.7617391698355));
#35856=CARTESIAN_POINT('Ctrl Pts',(56.3802496986626,23.0248113540135,22.7659552288274));
#35857=CARTESIAN_POINT('Ctrl Pts',(56.3124685965145,23.0710155821898,22.7702057989558));
#35858=CARTESIAN_POINT('Ctrl Pts',(56.2423900899683,23.1137954825678,22.7744563690843));
#35859=CARTESIAN_POINT('Ctrl Pts',(56.1703998605091,23.1529315865861,22.7787069392127));
#35860=CARTESIAN_POINT('Ctrl Pts',(56.098890315959,23.1918063754963,22.7829291279215));
#35861=CARTESIAN_POINT('Ctrl Pts',(56.025494950164,23.2270857320517,22.7871513166303));
#35862=CARTESIAN_POINT('Ctrl Pts',(55.9506136313523,23.2586022168339,22.791373505339));
#35863=CARTESIAN_POINT('Ctrl Pts',(55.8749772877364,23.2904364808451,22.7956382661773));
#35864=CARTESIAN_POINT('Ctrl Pts',(55.7978253135168,23.3184313985612,22.7999030270156));
#35865=CARTESIAN_POINT('Ctrl Pts',(55.7195854984368,23.3424659998471,22.8041677878539));
#35866=CARTESIAN_POINT('Ctrl Pts',(55.6413456833568,23.3665006011329,22.8084325486922));
#35867=CARTESIAN_POINT('Ctrl Pts',(55.5620185102528,23.386574830078,22.8126973095305));
#35868=CARTESIAN_POINT('Ctrl Pts',(55.482040398859,23.4026209238804,22.8169620703688));
#35869=CARTESIAN_POINT('Ctrl Pts',(55.4026912813566,23.4185408219674,22.8211932906737));
#35870=CARTESIAN_POINT('Ctrl Pts',(55.3224038865215,23.4305554604141,22.8254245109786));
#35871=CARTESIAN_POINT('Ctrl Pts',(55.2415969015931,23.438561294522,22.8296557312835));
#35872=CARTESIAN_POINT('Ctrl Pts',(55.1609057882251,23.4465556488241,22.8338808843147));
#35873=CARTESIAN_POINT('Ctrl Pts',(55.079697023254,23.4505525699812,22.8381060373458));
#35874=CARTESIAN_POINT('Ctrl Pts',(54.9983996620546,23.4504994774369,22.842331190377));
#35875=CARTESIAN_POINT('Ctrl Pts',(54.916893451207,23.4504462485,22.8465671976562));
#35876=CARTESIAN_POINT('Ctrl Pts',(54.8352986524015,23.446322084028,22.8508032049354));
#35877=CARTESIAN_POINT('Ctrl Pts',(54.7540530160318,23.4381263976826,22.8550392122146));
#35878=CARTESIAN_POINT('Ctrl Pts',(54.6731613477456,23.4299664180105,22.8592567642088));
#35879=CARTESIAN_POINT('Ctrl Pts',(54.5926162721334,23.4177703586222,22.8634743162029));
#35880=CARTESIAN_POINT('Ctrl Pts',(54.5128481900759,23.401589757658,22.8676918681971));
#35881=CARTESIAN_POINT('Ctrl Pts',(54.4331064456245,23.3854144991601,22.8719080276515));
#35882=CARTESIAN_POINT('Ctrl Pts',(54.3541416405487,23.3652574040454,22.8761241871059));
#35883=CARTESIAN_POINT('Ctrl Pts',(54.2763751613613,23.3412213357359,22.8803403465603));
#35884=CARTESIAN_POINT('Ctrl Pts',(54.1986105351915,23.3171858401572,22.8845564055522));
#35885=CARTESIAN_POINT('Ctrl Pts',(54.1220446219994,23.2892716935036,22.8887724645441));
#35886=CARTESIAN_POINT('Ctrl Pts',(54.0470834068934,23.2576315502274,22.892988523536));
#35887=CARTESIAN_POINT('Ctrl Pts',(53.971508586347,23.2257324121628,22.8972390936645));
#35888=CARTESIAN_POINT('Ctrl Pts',(53.8975653043072,23.1900461683508,22.901489663793));
#35889=CARTESIAN_POINT('Ctrl Pts',(53.8256470909457,23.1507778813712,22.9057402339214));
#35890=CARTESIAN_POINT('Ctrl Pts',(53.7542090816366,23.1117717920973,22.9099624226302));
#35891=CARTESIAN_POINT('Ctrl Pts',(53.6847695483082,23.0692316471731,22.9141846113389));
#35892=CARTESIAN_POINT('Ctrl Pts',(53.6176859967675,23.0234026407187,22.9184068000477));
#35893=CARTESIAN_POINT('Ctrl Pts',(53.5499260449404,22.9771115425537,22.922671560886));
#35894=CARTESIAN_POINT('Ctrl Pts',(53.4845702396638,22.9274651805442,22.9269363217244));
#35895=CARTESIAN_POINT('Ctrl Pts',(53.4219521812646,22.8747574061154,22.9312010825628));
#35896=CARTESIAN_POINT('Ctrl Pts',(53.3593341228654,22.8220496316865,22.9354658434011));
#35897=CARTESIAN_POINT('Ctrl Pts',(53.299454120126,22.7662808202186,22.9397306042395));
#35898=CARTESIAN_POINT('Ctrl Pts',(53.2426057460595,22.7077809245383,22.9439953650778));
#35899=CARTESIAN_POINT('Ctrl Pts',(53.1869656341608,22.6505243926645,22.9481694821773));
#35900=CARTESIAN_POINT('Ctrl Pts',(53.1340088995045,22.5904244190989,22.9523435992767));
#35901=CARTESIAN_POINT('Ctrl Pts',(53.0840457450709,22.527766193833,22.9565177163762));
#35902=CARTESIAN_POINT('Ctrl Pts',(53.0341473180934,22.4651891425358,22.9606864258911));
#35903=CARTESIAN_POINT('Ctrl Pts',(52.987235075695,22.4000607818049,22.964855135406));
#35904=CARTESIAN_POINT('Ctrl Pts',(52.9435826130974,22.3327031855761,22.9690238449209));
#35905=CARTESIAN_POINT('Ctrl Pts',(52.8999724782983,22.2654109029308,22.9731885122287));
#35906=CARTESIAN_POINT('Ctrl Pts',(52.8596161114748,22.1958940718837,22.9773531795364));
#35907=CARTESIAN_POINT('Ctrl Pts',(52.8227459819001,22.1245066432297,22.9815178468442));
#35908=CARTESIAN_POINT('Ctrl Pts',(52.7858995965409,22.0531651877935,22.9856798321229));
#35909=CARTESIAN_POINT('Ctrl Pts',(52.7525352111079,21.9799559496433,22.9898418174016));
#35910=CARTESIAN_POINT('Ctrl Pts',(52.7228403545881,21.9052591890214,22.9940038026803));
#35911=CARTESIAN_POINT('Ctrl Pts',(52.6931444373135,21.8305597600938,22.9981659366328));
#35912=CARTESIAN_POINT('Ctrl Pts',(52.6671185050231,21.7543731400044,23.0023280705853));
#35913=CARTESIAN_POINT('Ctrl Pts',(52.644902245445,21.6771003001696,23.0064902045377));
#35914=CARTESIAN_POINT('Ctrl Pts',(52.622686792589,21.5998302662847,23.0106521873538));
#35915=CARTESIAN_POINT('Ctrl Pts',(52.6042808618236,21.5214745534456,23.0148141701699));
#35916=CARTESIAN_POINT('Ctrl Pts',(52.5897738661255,21.4424480009992,23.018976152986));
#35917=CARTESIAN_POINT('Ctrl Pts',(52.5752530319411,21.3633460636921,23.0231421059929));
#35918=CARTESIAN_POINT('Ctrl Pts',(52.564638639425,21.2835724816293,23.0273080589998));
#35919=CARTESIAN_POINT('Ctrl Pts',(52.5579685557735,21.2035501790938,23.0314740120067));
#35920=CARTESIAN_POINT('Ctrl Pts',(52.5522587910044,21.1350490106478,23.0350401759338));
#35921=CARTESIAN_POINT('Ctrl Pts',(52.5494384806997,21.0663658657097,23.0386063398609));
#35922=CARTESIAN_POINT('Ctrl Pts',(52.5495010182643,20.9977660545166,23.042172503788));
#35923=CARTESIAN_POINT('',(52.5493390396331,21.0010204409205,23.842172503788));
#35924=CARTESIAN_POINT('Ctrl Pts',(52.5493375787181,20.9977659055204,23.042172503788));
#35925=CARTESIAN_POINT('Ctrl Pts',(52.5476321658041,20.8127232659271,23.0517912224542));
#35926=CARTESIAN_POINT('Ctrl Pts',(52.6512743420045,19.8149599677488,23.1037543726902));
#35927=CARTESIAN_POINT('Ctrl Pts',(54.016468625562,18.2755608973991,23.1980619544957));
#35928=CARTESIAN_POINT('Ctrl Pts',(56.7558779128847,18.6963517752573,23.3250952492048));
#35929=CARTESIAN_POINT('Ctrl Pts',(57.8876820693198,21.2262623582219,23.4521285439137));
#35930=CARTESIAN_POINT('Ctrl Pts',(56.3756506396827,23.5490170077549,23.5791618386227));
#35931=CARTESIAN_POINT('Ctrl Pts',(53.6041335644077,23.5380030107376,23.7061951333316));
#35932=CARTESIAN_POINT('Ctrl Pts',(52.5734000928234,21.9267438999263,23.7938653550534));
#35933=CARTESIAN_POINT('Ctrl Pts',(52.5456780645203,21.0581726905573,23.8391911452055));
#35934=CARTESIAN_POINT('Ctrl Pts',(52.5459788927558,21.0010218400661,23.842172503788));
#35935=CARTESIAN_POINT('',(52.5495005229243,21.0016008908874,24.6421725037586));
#35936=CARTESIAN_POINT('Ctrl Pts',(52.5495002124388,21.0010203738091,23.842172503788));
#35937=CARTESIAN_POINT('Ctrl Pts',(52.5494668326451,20.9208564408857,23.8463603929974));
#35938=CARTESIAN_POINT('Ctrl Pts',(52.5533713350428,20.8405326990059,23.8505482822069));
#35939=CARTESIAN_POINT('Ctrl Pts',(52.56123452562,20.7604729431319,23.8547361714163));
#35940=CARTESIAN_POINT('Ctrl Pts',(52.5694901515391,20.6764175728358,23.8591330693886));
#35941=CARTESIAN_POINT('Ctrl Pts',(52.5821100009684,20.5926537422153,23.8635299673608));
#35942=CARTESIAN_POINT('Ctrl Pts',(52.5990562459595,20.5096742512026,23.867926865333));
#35943=CARTESIAN_POINT('Ctrl Pts',(52.6151575944103,20.4308319059056,23.8721045451902));
#35944=CARTESIAN_POINT('Ctrl Pts',(52.6351641859981,20.3526981031234,23.8762822250473));
#35945=CARTESIAN_POINT('Ctrl Pts',(52.658990506447,20.2756901208084,23.8804599049045));
#35946=CARTESIAN_POINT('Ctrl Pts',(52.6828042394724,20.1987228217407,23.8846353776972));
#35947=CARTESIAN_POINT('Ctrl Pts',(52.7104335572416,20.1228806160397,23.8888108504898));
#35948=CARTESIAN_POINT('Ctrl Pts',(52.7417425205983,20.0485677077552,23.8929863232825));
#35949=CARTESIAN_POINT('Ctrl Pts',(52.7730450047718,19.9742701780362,23.8971609319887));
#35950=CARTESIAN_POINT('Ctrl Pts',(52.8080254378594,19.9015017549563,23.9013355406949));
#35951=CARTESIAN_POINT('Ctrl Pts',(52.8464995341962,19.8306471902019,23.905510149401));
#35952=CARTESIAN_POINT('Ctrl Pts',(52.8849780324974,19.7597845187132,23.9096852357397));
#35953=CARTESIAN_POINT('Ctrl Pts',(52.9269507585838,19.6908365565364,23.9138603220784));
#35954=CARTESIAN_POINT('Ctrl Pts',(52.9721879835204,19.6241625547249,23.9180354084171));
#35955=CARTESIAN_POINT('Ctrl Pts',(53.0174728968491,19.5574182661983,23.922214896068));
#35956=CARTESIAN_POINT('Ctrl Pts',(53.0660289078327,19.4929531144201,23.926394383719));
#35957=CARTESIAN_POINT('Ctrl Pts',(53.1175840045912,19.4310958377806,23.93057387137));
#35958=CARTESIAN_POINT('Ctrl Pts',(53.1691707310827,19.3692006108848,23.9347559231918));
#35959=CARTESIAN_POINT('Ctrl Pts',(53.2237598811306,19.3099167901632,23.9389379750137));
#35960=CARTESIAN_POINT('Ctrl Pts',(53.28104210512,19.253536715064,23.9431200268356));
#35961=CARTESIAN_POINT('Ctrl Pts',(53.3384170143248,19.1970654144667,23.9473088454054));
#35962=CARTESIAN_POINT('Ctrl Pts',(53.3984933359345,19.1435075469078,23.9514976639753));
#35963=CARTESIAN_POINT('Ctrl Pts',(53.4609287307505,19.0931151376733,23.9556864825451));
#35964=CARTESIAN_POINT('Ctrl Pts',(53.4836604329225,19.0747680888266,23.9572115626133));
#35965=CARTESIAN_POINT('Ctrl Pts',(53.5067045739923,19.0568402232667,23.9587366426815));
#35966=CARTESIAN_POINT('Ctrl Pts',(53.5300437569289,19.0393422293892,23.9602617227496));
#35967=CARTESIAN_POINT('Ctrl Pts',(53.5947965700661,18.9907953573373,23.9644929430516));
#35968=CARTESIAN_POINT('Ctrl Pts',(53.6620783416047,18.945368707485,23.9687241633536));
#35969=CARTESIAN_POINT('Ctrl Pts',(53.7315558201613,18.9033360754204,23.9729553836556));
#35970=CARTESIAN_POINT('Ctrl Pts',(53.8009336728765,18.8613637152083,23.9771805366839));
#35971=CARTESIAN_POINT('Ctrl Pts',(53.8725005850379,18.8227759456113,23.9814056897121));
#35972=CARTESIAN_POINT('Ctrl Pts',(53.9458919955203,18.7878050346111,23.9856308427403));
#35973=CARTESIAN_POINT('Ctrl Pts',(54.0194719456453,18.7527442847182,23.9898668500203));
#35974=CARTESIAN_POINT('Ctrl Pts',(54.0948853987074,18.7213192783467,23.9941028573002));
#35975=CARTESIAN_POINT('Ctrl Pts',(54.1717375500737,18.6937191055637,23.9983388645801));
#35976=CARTESIAN_POINT('Ctrl Pts',(54.2482548746696,18.6662391802499,24.0025564165714));
#35977=CARTESIAN_POINT('Ctrl Pts',(54.3261979500002,18.6425509960614,24.0067739685627));
#35978=CARTESIAN_POINT('Ctrl Pts',(54.4051561515476,18.6227934364136,24.010991520554));
#35979=CARTESIAN_POINT('Ctrl Pts',(54.4840882828935,18.6030424002623,24.0152076800056));
#35980=CARTESIAN_POINT('Ctrl Pts',(54.5640344241906,18.5872195241659,24.0194238394571));
#35981=CARTESIAN_POINT('Ctrl Pts',(54.6445699777732,18.5754134890048,24.0236399989087));
#35982=CARTESIAN_POINT('Ctrl Pts',(54.7251036123572,18.5636077351575,24.0278560578978));
#35983=CARTESIAN_POINT('Ctrl Pts',(54.8062261711365,18.5558186982803,24.0320721168868));
#35984=CARTESIAN_POINT('Ctrl Pts',(54.8875055082934,18.5520834901215,24.0362881758759));
#35985=CARTESIAN_POINT('Ctrl Pts',(54.969450168877,18.5483177068919,24.0405387460078));
#35986=CARTESIAN_POINT('Ctrl Pts',(55.0515537078735,18.5486724631353,24.0447893161397));
#35987=CARTESIAN_POINT('Ctrl Pts',(55.1333726448945,18.5531322088037,24.0490398862716));
#35988=CARTESIAN_POINT('Ctrl Pts',(55.214645269768,18.557562176363,24.0532620749776));
#35989=CARTESIAN_POINT('Ctrl Pts',(55.2956366211994,18.5660423711746,24.0574842636836));
#35990=CARTESIAN_POINT('Ctrl Pts',(55.3759184431055,18.5785055081349,24.0617064523897));
#35991=CARTESIAN_POINT('Ctrl Pts',(55.4570097430109,18.5910943103445,24.0659712132345));
#35992=CARTESIAN_POINT('Ctrl Pts',(55.5373766488547,18.6077467278717,24.0702359740793));
#35993=CARTESIAN_POINT('Ctrl Pts',(55.6165915194357,18.6283412665057,24.0745007349242));
#35994=CARTESIAN_POINT('Ctrl Pts',(55.6958063900168,18.6489358051396,24.078765495769));
#35995=CARTESIAN_POINT('Ctrl Pts',(55.7738687849726,18.6734722591182,24.0830302566138));
#35996=CARTESIAN_POINT('Ctrl Pts',(55.8503716359342,18.7017793119897,24.0872950174587));
#35997=CARTESIAN_POINT('Ctrl Pts',(55.9262728243055,18.7298637418538,24.0915262377619));
#35998=CARTESIAN_POINT('Ctrl Pts',(56.0009235480879,18.7617649446338,24.0957574580651));
#35999=CARTESIAN_POINT('Ctrl Pts',(56.0739130583664,18.7973513686767,24.0999886783683));
#36000=CARTESIAN_POINT('Ctrl Pts',(56.1467979067951,18.832886764278,24.1042138313977));
#36001=CARTESIAN_POINT('Ctrl Pts',(56.2180258583051,18.8720966839983,24.1084389844271));
#36002=CARTESIAN_POINT('Ctrl Pts',(56.2872040801193,18.914800751457,24.1126641374566));
#36003=CARTESIAN_POINT('Ctrl Pts',(56.356560018036,18.9576145239678,24.1169001447362));
#36004=CARTESIAN_POINT('Ctrl Pts',(56.4238552409761,19.0039402500301,24.1211361520158));
#36005=CARTESIAN_POINT('Ctrl Pts',(56.488716797084,19.0535487295902,24.1253721592954));
#36006=CARTESIAN_POINT('Ctrl Pts',(56.5532957666491,19.1029410766741,24.1295897112878));
#36007=CARTESIAN_POINT('Ctrl Pts',(56.6154618543834,19.1555873547957,24.1338072632801));
#36008=CARTESIAN_POINT('Ctrl Pts',(56.6748757159482,19.2112178483317,24.1380248152724));
#36009=CARTESIAN_POINT('Ctrl Pts',(56.7342699604073,19.266829973944,24.142240974725));
#36010=CARTESIAN_POINT('Ctrl Pts',(56.7909134441815,19.3254240407466,24.1464571341776));
#36011=CARTESIAN_POINT('Ctrl Pts',(56.8445014283317,19.3866913714721,24.1506732936302));
#36012=CARTESIAN_POINT('Ctrl Pts',(56.8980881355884,19.4479572423209,24.1548893526202));
#36013=CARTESIAN_POINT('Ctrl Pts',(56.948619182728,19.5118958997652,24.1591054116102));
#36014=CARTESIAN_POINT('Ctrl Pts',(56.9958290682475,19.5781643624039,24.1633214706002));
#36015=CARTESIAN_POINT('Ctrl Pts',(57.0434253968885,19.644975274813,24.1675720407308));
#36016=CARTESIAN_POINT('Ctrl Pts',(57.0876456498621,19.7141539289657,24.1718226108614));
#36017=CARTESIAN_POINT('Ctrl Pts',(57.128262428118,19.7853192653783,24.176073180992));
#36018=CARTESIAN_POINT('Ctrl Pts',(57.1686080046385,19.8560094246949,24.1802953696989));
#36019=CARTESIAN_POINT('Ctrl Pts',(57.2053979243557,19.9286593697791,24.1845175584057));
#36020=CARTESIAN_POINT('Ctrl Pts',(57.238456512793,20.0028727812688,24.1887397471126));
#36021=CARTESIAN_POINT('Ctrl Pts',(57.2718484294658,20.0778344831929,24.1930045079551));
#36022=CARTESIAN_POINT('Ctrl Pts',(57.3014331705383,20.154390904565,24.1972692687976));
#36023=CARTESIAN_POINT('Ctrl Pts',(57.3270809433459,20.2321168493083,24.2015340296401));
#36024=CARTESIAN_POINT('Ctrl Pts',(57.3527287161536,20.3098427940516,24.2057987904826));
#36025=CARTESIAN_POINT('Ctrl Pts',(57.3744394548109,20.3887377805894,24.2100635513251));
#36026=CARTESIAN_POINT('Ctrl Pts',(57.3921363841013,20.468366884159,24.2143283121676));
#36027=CARTESIAN_POINT('Ctrl Pts',(57.4096941346004,20.5473697388351,24.2185595324873));
#36028=CARTESIAN_POINT('Ctrl Pts',(57.423366868251,20.6273914465543,24.2227907528071));
#36029=CARTESIAN_POINT('Ctrl Pts',(57.4330424023754,20.708015551367,24.2270219731268));
#36030=CARTESIAN_POINT('Ctrl Pts',(57.4427040624612,20.7885240468576,24.2312471261729));
#36031=CARTESIAN_POINT('Ctrl Pts',(57.448379851686,20.8696327661643,24.2354722792189));
#36032=CARTESIAN_POINT('Ctrl Pts',(57.4500083261566,20.9509138332773,24.239697432265));
#36033=CARTESIAN_POINT('Ctrl Pts',(57.4516409841053,21.0324037078212,24.2439334395404));
#36034=CARTESIAN_POINT('Ctrl Pts',(57.4492054098064,21.1140663546487,24.2481694468159));
#36035=CARTESIAN_POINT('Ctrl Pts',(57.4426919626134,21.1954641291484,24.2524054540914));
#36036=CARTESIAN_POINT('Ctrl Pts',(57.4362068929457,21.2765072730917,24.2566230061005));
#36037=CARTESIAN_POINT('Ctrl Pts',(57.4256794380758,21.3572873808308,24.2608405581095));
#36038=CARTESIAN_POINT('Ctrl Pts',(57.4111522227015,21.4373730775457,24.2650581101185));
#36039=CARTESIAN_POINT('Ctrl Pts',(57.3966298038832,21.5174323317849,24.2692742695878));
#36040=CARTESIAN_POINT('Ctrl Pts',(57.3781103300617,21.596797173218,24.2734904290571));
#36041=CARTESIAN_POINT('Ctrl Pts',(57.355687926689,21.6750441778517,24.2777065885264));
#36042=CARTESIAN_POINT('Ctrl Pts',(57.3332660575971,21.7532893180169,24.2819226475331));
#36043=CARTESIAN_POINT('Ctrl Pts',(57.3069415729986,21.8304162277134,24.2861387065398));
#36044=CARTESIAN_POINT('Ctrl Pts',(57.2768586972871,21.9060158511793,24.2903547655465));
#36045=CARTESIAN_POINT('Ctrl Pts',(57.2465295742494,21.982234305282,24.2946053356573));
#36046=CARTESIAN_POINT('Ctrl Pts',(57.2123804089379,22.0568999024811,24.2988559057682));
#36047=CARTESIAN_POINT('Ctrl Pts',(57.1746080802747,22.1296149552853,24.303106475879));
#36048=CARTESIAN_POINT('Ctrl Pts',(57.1370879603909,22.2018444840201,24.3073286646023));
#36049=CARTESIAN_POINT('Ctrl Pts',(57.0959932043955,22.2721490627644,24.3115508533255));
#36050=CARTESIAN_POINT('Ctrl Pts',(57.051561559298,22.3401661905938,24.3157730420488));
#36051=CARTESIAN_POINT('Ctrl Pts',(57.0066819125277,22.4088691311359,24.3200378028534));
#36052=CARTESIAN_POINT('Ctrl Pts',(56.9583979923833,22.4752378398237,24.3243025636581));
#36053=CARTESIAN_POINT('Ctrl Pts',(56.9069966872212,22.5389327096815,24.3285673244627));
#36054=CARTESIAN_POINT('Ctrl Pts',(56.8555953820591,22.6026275795392,24.3328320852674));
#36055=CARTESIAN_POINT('Ctrl Pts',(56.8010770607924,22.6636482940861,24.337096846072));
#36056=CARTESIAN_POINT('Ctrl Pts',(56.74376553338,22.7216945183731,24.3413616068767));
#36057=CARTESIAN_POINT('Ctrl Pts',(56.686904736685,22.7792842338651,24.3455928271567));
#36058=CARTESIAN_POINT('Ctrl Pts',(56.6270813226942,22.8341620652118,24.3498240474367));
#36059=CARTESIAN_POINT('Ctrl Pts',(56.564584384522,22.8860079410517,24.3540552677167));
#36060=CARTESIAN_POINT('Ctrl Pts',(56.5021770625848,22.9377794735343,24.3582804207229));
#36061=CARTESIAN_POINT('Ctrl Pts',(56.4371041851804,22.9865273908568,24.3625055737292));
#36062=CARTESIAN_POINT('Ctrl Pts',(56.3696919526391,23.0319680619723,24.3667307267355));
#36063=CARTESIAN_POINT('Ctrl Pts',(56.3021065402889,23.0775254686779,24.3709667340209));
#36064=CARTESIAN_POINT('Ctrl Pts',(56.232170074164,23.1197582836417,24.3752027413063));
#36065=CARTESIAN_POINT('Ctrl Pts',(56.1602450513843,23.1584211059796,24.3794387485917));
#36066=CARTESIAN_POINT('Ctrl Pts',(56.0886333894946,23.1969154832347,24.3836563005613));
#36067=CARTESIAN_POINT('Ctrl Pts',(56.0150508704219,23.2318706815473,24.3878738525309));
#36068=CARTESIAN_POINT('Ctrl Pts',(55.939883062584,23.2630886148509,24.3920914045004));
#36069=CARTESIAN_POINT('Ctrl Pts',(55.8647400734435,23.2942962407042,24.3963075639304));
#36070=CARTESIAN_POINT('Ctrl Pts',(55.7880132640168,23.3217688738396,24.4005237233604));
#36071=CARTESIAN_POINT('Ctrl Pts',(55.7101094469895,23.3453560120579,24.4047398827904));
#36072=CARTESIAN_POINT('Ctrl Pts',(55.6322074862489,23.3689425882436,24.4089559417581));
#36073=CARTESIAN_POINT('Ctrl Pts',(55.5531290189643,23.3886437199271,24.4131720007257));
#36074=CARTESIAN_POINT('Ctrl Pts',(55.4732959498653,23.4043587905804,24.4173880596934));
#36075=CARTESIAN_POINT('Ctrl Pts',(55.3928093950728,23.4202024993276,24.4216386298511));
#36076=CARTESIAN_POINT('Ctrl Pts',(55.3115562952131,23.4319944804183,24.4258892000088));
#36077=CARTESIAN_POINT('Ctrl Pts',(55.2299775534543,23.4396845236438,24.4301397701664));
#36078=CARTESIAN_POINT('Ctrl Pts',(55.1489435209287,23.4473232196991,24.4343619588517));
#36079=CARTESIAN_POINT('Ctrl Pts',(55.0675886537223,23.4509146302014,24.4385841475369));
#36080=CARTESIAN_POINT('Ctrl Pts',(54.9863464495475,23.4504619626838,24.4428063362221));
#36081=CARTESIAN_POINT('Ctrl Pts',(54.904285082534,23.4500047309325,24.447071097116));
#36082=CARTESIAN_POINT('Ctrl Pts',(54.8223391483354,23.4454214366196,24.4513358580099));
#36083=CARTESIAN_POINT('Ctrl Pts',(54.7409495539087,23.4367689911807,24.4556006189038));
#36084=CARTESIAN_POINT('Ctrl Pts',(54.659559959482,23.4281165457418,24.4598653797978));
#36085=CARTESIAN_POINT('Ctrl Pts',(54.5787271707783,23.415395087548,24.4641301406917));
#36086=CARTESIAN_POINT('Ctrl Pts',(54.4988791167051,23.3987138450273,24.4683949015856));
#36087=CARTESIAN_POINT('Ctrl Pts',(54.4196590347824,23.3821637936279,24.4726261218866));
#36088=CARTESIAN_POINT('Ctrl Pts',(54.3411111780572,23.3616540035517,24.4768573421877));
#36089=CARTESIAN_POINT('Ctrl Pts',(54.2636612344112,23.337253831378,24.4810885624888));
#36090=CARTESIAN_POINT('Ctrl Pts',(54.1863223485687,23.312888647345,24.4853137155158));
#36091=CARTESIAN_POINT('Ctrl Pts',(54.1100786887618,23.2846442991288,24.4895388685429));
#36092=CARTESIAN_POINT('Ctrl Pts',(54.0353454447737,23.2526410808385,24.4937640215699));
#36093=CARTESIAN_POINT('Ctrl Pts',(53.9604202139999,23.2205556475299,24.4980000288501));
#36094=CARTESIAN_POINT('Ctrl Pts',(53.8870136301012,23.1846921094567,24.5022360361303));
#36095=CARTESIAN_POINT('Ctrl Pts',(53.8155284414307,23.1452219878,24.5064720434105));
#36096=CARTESIAN_POINT('Ctrl Pts',(53.7443546969706,23.1059238282112,24.5106895953999));
#36097=CARTESIAN_POINT('Ctrl Pts',(53.6750860540547,23.0630506645706,24.5149071473893));
#36098=CARTESIAN_POINT('Ctrl Pts',(53.6080980152219,23.0168190585104,24.5191246993788));
#36099=CARTESIAN_POINT('Ctrl Pts',(53.5411320943189,22.9706027170771,24.5233408588283));
#36100=CARTESIAN_POINT('Ctrl Pts',(53.4764456644804,22.9210303991786,24.5275570182777));
#36101=CARTESIAN_POINT('Ctrl Pts',(53.4143857657028,22.8683623176446,24.5317731777272));
#36102=CARTESIAN_POINT('Ctrl Pts',(53.3523273456901,22.8156954910869,24.535989236714));
#36103=CARTESIAN_POINT('Ctrl Pts',(53.2928956860611,22.7599333492358,24.5402052957007));
#36104=CARTESIAN_POINT('Ctrl Pts',(53.2364040943428,22.7013758348904,24.5444213546874));
#36105=CARTESIAN_POINT('Ctrl Pts',(53.1794500827098,22.6423389897284,24.5486719248214));
#36106=CARTESIAN_POINT('Ctrl Pts',(53.125484838457,22.580461131107,24.5529224949553));
#36107=CARTESIAN_POINT('Ctrl Pts',(53.0747896172992,22.5160854963824,24.5571730650892));
#36108=CARTESIAN_POINT('Ctrl Pts',(53.0244328925937,22.4521397034352,24.5613952537924));
#36109=CARTESIAN_POINT('Ctrl Pts',(52.97730287682,22.3857298072079,24.5656174424955));
#36110=CARTESIAN_POINT('Ctrl Pts',(52.933631926826,22.3172217870074,24.5698396311986));
#36111=CARTESIAN_POINT('Ctrl Pts',(52.8895206445309,22.2480230034006,24.574104392048));
#36112=CARTESIAN_POINT('Ctrl Pts',(52.8489388160609,22.1766839693441,24.5783691528973));
#36113=CARTESIAN_POINT('Ctrl Pts',(52.8120776917919,22.1036060090655,24.5826339137466));
#36114=CARTESIAN_POINT('Ctrl Pts',(52.775216567523,22.0305280487869,24.5868986745959));
#36115=CARTESIAN_POINT('Ctrl Pts',(52.7420762838396,21.9557116288227,24.5911634354452));
#36116=CARTESIAN_POINT('Ctrl Pts',(52.7127970955513,21.8795755362,24.5954281962945));
#36117=CARTESIAN_POINT('Ctrl Pts',(52.6797334709213,21.7935985903062,24.6002441922323));
#36118=CARTESIAN_POINT('Ctrl Pts',(52.6514890713543,21.7056709150828,24.6050601881701));
#36119=CARTESIAN_POINT('Ctrl Pts',(52.6282678414551,21.6163090281052,24.6098761841079));
#36120=CARTESIAN_POINT('Ctrl Pts',(52.6051398843363,21.5273060812737,24.6146728356211));
#36121=CARTESIAN_POINT('Ctrl Pts',(52.586994953676,21.4368806120397,24.6194694871343));
#36122=CARTESIAN_POINT('Ctrl Pts',(52.5739877880387,21.3455647514063,24.6242661386475));
#36123=CARTESIAN_POINT('Ctrl Pts',(52.5610695804394,21.2548734142115,24.6290299851116));
#36124=CARTESIAN_POINT('Ctrl Pts',(52.5532192128864,21.1633040306489,24.6337938315756));
#36125=CARTESIAN_POINT('Ctrl Pts',(52.5505403056274,21.0713964680082,24.6385576780397));
#36126=CARTESIAN_POINT('Ctrl Pts',(52.5498627171191,21.0481498595023,24.639762619946));
#36127=CARTESIAN_POINT('Ctrl Pts',(52.5495157320829,21.024881700089,24.6409675618523));
#36128=CARTESIAN_POINT('Ctrl Pts',(52.5495005229243,21.0016008908875,24.6421725037586));
#36129=CARTESIAN_POINT('',(52.5495007252096,20.9981147276813,25.442172503788));
#36130=CARTESIAN_POINT('Ctrl Pts',(52.5495005229239,21.0016008903187,24.642172503788));
#36131=CARTESIAN_POINT('Ctrl Pts',(52.5494469895352,20.919656774874,24.6464136750385));
#36132=CARTESIAN_POINT('Ctrl Pts',(52.5535080759981,20.8376904850347,24.6506548462889));
#36133=CARTESIAN_POINT('Ctrl Pts',(52.5616638957009,20.7561408347598,24.6548960175394));
#36134=CARTESIAN_POINT('Ctrl Pts',(52.5698203090628,20.6745852485174,24.659137497503));
#36135=CARTESIAN_POINT('Ctrl Pts',(52.5820720017549,20.5934468167741,24.6633789774667));
#36136=CARTESIAN_POINT('Ctrl Pts',(52.5983472524457,20.5131588244971,24.6676204574304));
#36137=CARTESIAN_POINT('Ctrl Pts',(52.6146284494122,20.4328414984462,24.6718634870481));
#36138=CARTESIAN_POINT('Ctrl Pts',(52.6349360333774,20.3533756766673,24.6761065166659));
#36139=CARTESIAN_POINT('Ctrl Pts',(52.6591475485383,20.2751827468349,24.6803495462836));
#36140=CARTESIAN_POINT('Ctrl Pts',(52.6833913128904,20.1968856657866,24.684598227521));
#36141=CARTESIAN_POINT('Ctrl Pts',(52.711549249218,20.1198652968742,24.6888469087583));
#36142=CARTESIAN_POINT('Ctrl Pts',(52.7434497051681,20.044525763354,24.6930955899957));
#36143=CARTESIAN_POINT('Ctrl Pts',(52.7753750807105,19.9691273770557,24.6973475901637));
#36144=CARTESIAN_POINT('Ctrl Pts',(52.8110485959233,19.8954128500759,24.7015995903318));
#36145=CARTESIAN_POINT('Ctrl Pts',(52.8502524249652,19.8237620930985,24.7058515904999));
#36146=CARTESIAN_POINT('Ctrl Pts',(52.8895250790829,19.7519855481841,24.710111055353));
#36147=CARTESIAN_POINT('Ctrl Pts',(52.9323401763454,19.6822803915989,24.7143705202061));
#36148=CARTESIAN_POINT('Ctrl Pts',(52.9784366254433,19.6149975550018,24.7186299850591));
#36149=CARTESIAN_POINT('Ctrl Pts',(52.9922583006089,19.5948233001543,24.7199071537073));
#36150=CARTESIAN_POINT('Ctrl Pts',(53.0063747167523,19.5748665941868,24.7211843223554));
#36151=CARTESIAN_POINT('Ctrl Pts',(53.0207781605817,19.5551362831154,24.7224614910035));
#36152=CARTESIAN_POINT('Ctrl Pts',(53.0684963230416,19.4897703747783,24.7266927111036));
#36153=CARTESIAN_POINT('Ctrl Pts',(53.1195456006491,19.426648366204,24.7309239312036));
#36154=CARTESIAN_POINT('Ctrl Pts',(53.173687417,19.3661295647525,24.7351551513036));
#36155=CARTESIAN_POINT('Ctrl Pts',(53.2277515977743,19.3056975430281,24.73938030413));
#36156=CARTESIAN_POINT('Ctrl Pts',(53.2848992027025,19.2478616583465,24.7436054569565));
#36157=CARTESIAN_POINT('Ctrl Pts',(53.3448495668384,19.1929506665271,24.7478306097829));
#36158=CARTESIAN_POINT('Ctrl Pts',(53.4049539446849,19.1378986072475,24.7520666171133));
#36159=CARTESIAN_POINT('Ctrl Pts',(53.4678752173697,19.0857868657356,24.7563026244437));
#36160=CARTESIAN_POINT('Ctrl Pts',(53.5332911681543,19.0369117562917,24.7605386317741));
#36161=CARTESIAN_POINT('Ctrl Pts',(53.598422113145,18.9882495871047,24.7647561835655));
#36162=CARTESIAN_POINT('Ctrl Pts',(53.6660256739054,18.9427961925174,24.7689737353569));
#36163=CARTESIAN_POINT('Ctrl Pts',(53.7357498184658,18.9008045044611,24.7731912871483));
#36164=CARTESIAN_POINT('Ctrl Pts',(53.8054509417181,18.8588266810939,24.7774074464011));
#36165=CARTESIAN_POINT('Ctrl Pts',(53.8772708603774,18.8203085341402,24.7816236056539));
#36166=CARTESIAN_POINT('Ctrl Pts',(53.9508294943397,18.7854590769073,24.7858397649068));
#36167=CARTESIAN_POINT('Ctrl Pts',(54.0243863755737,18.7506104500544,24.7900558236985));
#36168=CARTESIAN_POINT('Ctrl Pts',(54.0996814691092,18.7194305371688,24.7942718824902));
#36169=CARTESIAN_POINT('Ctrl Pts',(54.1763123908464,18.6920812465499,24.7984879412819));
#36170=CARTESIAN_POINT('Ctrl Pts',(54.2535705936829,18.6645080816424,24.8027385116512));
#36171=CARTESIAN_POINT('Ctrl Pts',(54.3321861487511,18.6408287178226,24.8069890820204));
#36172=CARTESIAN_POINT('Ctrl Pts',(54.4117304274016,18.6211580212307,24.8112396523896));
#36173=CARTESIAN_POINT('Ctrl Pts',(54.4907435739932,18.6016186695672,24.8154618409037));
#36174=CARTESIAN_POINT('Ctrl Pts',(54.5706726067556,18.5860346440911,24.8196840294178));
#36175=CARTESIAN_POINT('Ctrl Pts',(54.65108832087,18.57446688537,24.8239062179319));
#36176=CARTESIAN_POINT('Ctrl Pts',(54.7323148753122,18.5627824876888,24.8281709792287));
#36177=CARTESIAN_POINT('Ctrl Pts',(54.8140374971521,18.5551958504485,24.8324357405255));
#36178=CARTESIAN_POINT('Ctrl Pts',(54.8958117110061,18.5517158967071,24.8367005018222));
#36179=CARTESIAN_POINT('Ctrl Pts',(54.9775859248601,18.5482359429657,24.840965263119));
#36180=CARTESIAN_POINT('Ctrl Pts',(55.0594112494361,18.5488626047862,24.8452300244158));
#36181=CARTESIAN_POINT('Ctrl Pts',(55.1408483071797,18.5535511441347,24.8494947857125));
#36182=CARTESIAN_POINT('Ctrl Pts',(55.221644889089,18.5582028096541,24.853726006056));
#36183=CARTESIAN_POINT('Ctrl Pts',(55.3023622703535,18.5668700877868,24.8579572263995));
#36184=CARTESIAN_POINT('Ctrl Pts',(55.3825691868474,18.5795473424843,24.862188446743));
#36185=CARTESIAN_POINT('Ctrl Pts',(55.4626610922015,18.5922064188803,24.8664135998108));
#36186=CARTESIAN_POINT('Ctrl Pts',(55.5422435311876,18.6088639798844,24.8706387528786));
#36187=CARTESIAN_POINT('Ctrl Pts',(55.6208880888397,18.6294624594542,24.8748639059464));
#36188=CARTESIAN_POINT('Ctrl Pts',(55.6997346803356,18.6501138554638,24.8790999132162));
#36189=CARTESIAN_POINT('Ctrl Pts',(55.7776380947281,18.6747264104519,24.883335920486));
#36190=CARTESIAN_POINT('Ctrl Pts',(55.8541746453639,18.7031900546154,24.8875719277558));
#36191=CARTESIAN_POINT('Ctrl Pts',(55.9303777450363,18.7315296896684,24.8917894797817));
#36192=CARTESIAN_POINT('Ctrl Pts',(56.005225424915,18.7636867719553,24.8960070318077));
#36193=CARTESIAN_POINT('Ctrl Pts',(56.0783142831877,18.799502656972,24.9002245838336));
#36194=CARTESIAN_POINT('Ctrl Pts',(56.1513790091499,18.8353067163824,24.9044407433179));
#36195=CARTESIAN_POINT('Ctrl Pts',(56.2226856495796,18.8747669750721,24.9086569028023));
#36196=CARTESIAN_POINT('Ctrl Pts',(56.2918524963338,18.9176774078649,24.9128730622866));
#36197=CARTESIAN_POINT('Ctrl Pts',(56.361017694951,18.9605868181698,24.9170891213065));
#36198=CARTESIAN_POINT('Ctrl Pts',(56.428042806785,19.0069459930796,24.9213051803265));
#36199=CARTESIAN_POINT('Ctrl Pts',(56.4925736092709,19.0565046254472,24.9255212393464));
#36200=CARTESIAN_POINT('Ctrl Pts',(56.5576326365779,19.1064689260958,24.929771809436));
#36201=CARTESIAN_POINT('Ctrl Pts',(56.6201559408607,19.1596850256144,24.9340223795256));
#36202=CARTESIAN_POINT('Ctrl Pts',(56.6798145957848,19.2158550580773,24.9382729496151));
#36203=CARTESIAN_POINT('Ctrl Pts',(56.7390749056417,19.2716500392525,24.942495138347));
#36204=CARTESIAN_POINT('Ctrl Pts',(56.7955084237743,19.3303592449377,24.9467173270788));
#36205=CARTESIAN_POINT('Ctrl Pts',(56.8488312214888,19.39165508536,24.9509395158107));
#36206=CARTESIAN_POINT('Ctrl Pts',(56.9026916692801,19.4535689674965,24.9552042765792));
#36207=CARTESIAN_POINT('Ctrl Pts',(56.9533780132041,19.5181215575935,24.9594690373476));
#36208=CARTESIAN_POINT('Ctrl Pts',(57.0006417516066,19.5849442301702,24.9637337981161));
#36209=CARTESIAN_POINT('Ctrl Pts',(57.0479054900091,19.6517669027469,24.9679985588845));
#36210=CARTESIAN_POINT('Ctrl Pts',(57.0917464190062,19.7208592165682,24.972263319653));
#36211=CARTESIAN_POINT('Ctrl Pts',(57.1319638890079,19.7918277333235,24.9765280804214));
#36212=CARTESIAN_POINT('Ctrl Pts',(57.1718650729558,19.8622381256591,24.9807593014284));
#36213=CARTESIAN_POINT('Ctrl Pts',(57.208349251496,19.9347593240248,24.9849905224353));
#36214=CARTESIAN_POINT('Ctrl Pts',(57.2411873194301,20.009025908903,24.9892217434422));
#36215=CARTESIAN_POINT('Ctrl Pts',(57.2739782999067,20.0831860007721,24.9934468971786));
#36216=CARTESIAN_POINT('Ctrl Pts',(57.3031333670747,20.1590860868616,24.9976720509151));
#36217=CARTESIAN_POINT('Ctrl Pts',(57.3284685940376,20.2363349840535,25.0018972046515));
#36218=CARTESIAN_POINT('Ctrl Pts',(57.3538689008839,20.3137823144083,25.0061332117548));
#36219=CARTESIAN_POINT('Ctrl Pts',(57.3754294908446,20.3925849804311,25.0103692188581));
#36220=CARTESIAN_POINT('Ctrl Pts',(57.3930131164161,20.4723273034727,25.0146052259614));
#36221=CARTESIAN_POINT('Ctrl Pts',(57.410520137943,20.5517222246407,25.0188227786637));
#36222=CARTESIAN_POINT('Ctrl Pts',(57.4240846658178,20.6320481774305,25.023040331366));
#36223=CARTESIAN_POINT('Ctrl Pts',(57.4336212655173,20.7128801887332,25.0272578840683));
#36224=CARTESIAN_POINT('Ctrl Pts',(57.443154716448,20.7936855111397,25.0314740442304));
#36225=CARTESIAN_POINT('Ctrl Pts',(57.4486628258277,20.874996098887,25.0356902043925));
#36226=CARTESIAN_POINT('Ctrl Pts',(57.4501117328319,20.9563795158251,25.0399063645546));
#36227=CARTESIAN_POINT('Ctrl Pts',(57.451560605311,21.0377609935332,25.0441224242527));
#36228=CARTESIAN_POINT('Ctrl Pts',(57.4489504605594,21.1192148321139,25.0483384839508));
#36229=CARTESIAN_POINT('Ctrl Pts',(57.4422995483118,21.2003076791242,25.0525545436489));
#36230=CARTESIAN_POINT('Ctrl Pts',(57.4355941965437,21.2820642930798,25.0568051129391));
#36231=CARTESIAN_POINT('Ctrl Pts',(57.4247816456242,21.3634534991379,25.0610556822292));
#36232=CARTESIAN_POINT('Ctrl Pts',(57.4099338219404,21.4440374126894,25.0653062515193));
#36233=CARTESIAN_POINT('Ctrl Pts',(57.395185133105,21.5240832895412,25.0695284409236));
#36234=CARTESIAN_POINT('Ctrl Pts',(57.3764550603819,21.6033341518738,25.0737506303278));
#36235=CARTESIAN_POINT('Ctrl Pts',(57.353864903956,21.6813738063093,25.077972819732));
#36236=CARTESIAN_POINT('Ctrl Pts',(57.3310469843956,21.7602002882448,25.0822375789651));
#36237=CARTESIAN_POINT('Ctrl Pts',(57.3042908635483,21.8377905417839,25.0865023381982));
#36238=CARTESIAN_POINT('Ctrl Pts',(57.2737715302839,21.9137358907641,25.0907670974313));
#36239=CARTESIAN_POINT('Ctrl Pts',(57.2432521970195,21.9896812397442,25.0950318566643));
#36240=CARTESIAN_POINT('Ctrl Pts',(57.2089699115283,22.0639812736087,25.0992966158974));
#36241=CARTESIAN_POINT('Ctrl Pts',(57.1711464576412,22.1362540690674,25.1035613751305));
#36242=CARTESIAN_POINT('Ctrl Pts',(57.1336204695482,22.2079584689332,25.1077925937992));
#36243=CARTESIAN_POINT('Ctrl Pts',(57.0924681360465,22.2779363079199,25.1120238124678));
#36244=CARTESIAN_POINT('Ctrl Pts',(57.0478722692984,22.3457969455451,25.1162550311365));
#36245=CARTESIAN_POINT('Ctrl Pts',(57.0033403499239,22.4135602757322,25.1204801825316));
#36246=CARTESIAN_POINT('Ctrl Pts',(56.9553749572966,22.4792120488663,25.1247053339268));
#36247=CARTESIAN_POINT('Ctrl Pts',(56.9042050477441,22.5423856152551,25.1289304853219));
#36248=CARTESIAN_POINT('Ctrl Pts',(56.8529036599361,22.6057215026325,25.1331664930102));
#36249=CARTESIAN_POINT('Ctrl Pts',(56.7983814910119,22.6665660165,25.1374025006984));
#36250=CARTESIAN_POINT('Ctrl Pts',(56.7409133904935,22.7245784461138,25.1416385083866));
#36251=CARTESIAN_POINT('Ctrl Pts',(56.6836956924912,22.782338101437,25.1458560587572));
#36252=CARTESIAN_POINT('Ctrl Pts',(56.6235580050994,22.8372899630489,25.1500736091279));
#36253=CARTESIAN_POINT('Ctrl Pts',(56.5608110809614,22.8891318163506,25.1542911594985));
#36254=CARTESIAN_POINT('Ctrl Pts',(56.4980848743157,22.9409565527464,25.1585073173376));
#36255=CARTESIAN_POINT('Ctrl Pts',(56.4327514998883,22.9896730241156,25.1627234751768));
#36256=CARTESIAN_POINT('Ctrl Pts',(56.3651559454247,23.0350183032768,25.1669396330159));
#36257=CARTESIAN_POINT('Ctrl Pts',(56.2975620014607,23.0803625020629,25.1711556904029));
#36258=CARTESIAN_POINT('Ctrl Pts',(56.2277063713352,23.1223354102548,25.1753717477898));
#36259=CARTESIAN_POINT('Ctrl Pts',(56.1559630681782,23.1607173889725,25.1795878051768));
#36260=CARTESIAN_POINT('Ctrl Pts',(56.0836324399257,23.1994135809802,25.183838377232));
#36261=CARTESIAN_POINT('Ctrl Pts',(56.009383504594,23.2344595375161,25.1880889492872));
#36262=CARTESIAN_POINT('Ctrl Pts',(55.9336231895077,23.2656782626872,25.1923395213425));
#36263=CARTESIAN_POINT('Ctrl Pts',(55.8583687944921,23.2966885122253,25.1965617084878));
#36264=CARTESIAN_POINT('Ctrl Pts',(55.7816236070862,23.3239223917217,25.2007838956332));
#36265=CARTESIAN_POINT('Ctrl Pts',(55.7038030989693,23.3472561530181,25.2050060827786));
#36266=CARTESIAN_POINT('Ctrl Pts',(55.6251978335577,23.3708252165482,25.2092708472887));
#36267=CARTESIAN_POINT('Ctrl Pts',(55.5454959096208,23.3904149440204,25.2135356117989));
#36268=CARTESIAN_POINT('Ctrl Pts',(55.4651355960718,23.4059507740739,25.217800376309));
#36269=CARTESIAN_POINT('Ctrl Pts',(55.3847752825228,23.4214866041274,25.2220651408191));
#36270=CARTESIAN_POINT('Ctrl Pts',(55.3037570654115,23.432968532771,25.2263299053293));
#36271=CARTESIAN_POINT('Ctrl Pts',(55.222522108151,23.4403758237993,25.2305946698394));
#36272=CARTESIAN_POINT('Ctrl Pts',(55.1419260837726,23.4477248546651,25.2348258909297));
#36273=CARTESIAN_POINT('Ctrl Pts',(55.0608144934773,23.451090718721,25.23905711202));
#36274=CARTESIAN_POINT('Ctrl Pts',(54.9796146923591,23.4504152075174,25.2432883331102));
#36275=CARTESIAN_POINT('Ctrl Pts',(54.8985313263053,23.4497406649515,25.2475134869135));
#36276=CARTESIAN_POINT('Ctrl Pts',(54.8173604616272,23.4450362603868,25.2517386407167));
#36277=CARTESIAN_POINT('Ctrl Pts',(54.7365343158626,23.4362955656656,25.2559637945199));
#36278=CARTESIAN_POINT('Ctrl Pts',(54.6555005495152,23.4275324184557,25.2601998016045));
#36279=CARTESIAN_POINT('Ctrl Pts',(54.574813745973,23.4147121818007,25.264435808689));
#36280=CARTESIAN_POINT('Ctrl Pts',(54.4949092113116,23.3978810531763,25.2686718157735));
#36281=CARTESIAN_POINT('Ctrl Pts',(54.4153527843546,23.381123250122,25.2728893685024));
#36282=CARTESIAN_POINT('Ctrl Pts',(54.3365722840239,23.3603895179163,25.2771069212312));
#36283=CARTESIAN_POINT('Ctrl Pts',(54.2589901389481,23.3357770946355,25.2813244739601));
#36284=CARTESIAN_POINT('Ctrl Pts',(54.1814336100137,23.3111727979064,25.2855406341336));
#36285=CARTESIAN_POINT('Ctrl Pts',(54.105075093389,23.2826924938103,25.2897567943072));
#36286=CARTESIAN_POINT('Ctrl Pts',(54.0303225700522,23.2504834884642,25.2939729544807));
#36287=CARTESIAN_POINT('Ctrl Pts',(53.9555718282075,23.2182752507187,25.2981890141753));
#36288=CARTESIAN_POINT('Ctrl Pts',(53.8824274300873,23.1823386733941,25.3024050738699));
#36289=CARTESIAN_POINT('Ctrl Pts',(53.8112767225188,23.1428689226302,25.3066211335645));
#36290=CARTESIAN_POINT('Ctrl Pts',(53.7395436277525,23.103076101607,25.3108717028131));
#36291=CARTESIAN_POINT('Ctrl Pts',(53.6698374392182,23.0596922189523,25.3151222720618));
#36292=CARTESIAN_POINT('Ctrl Pts',(53.6025275191101,23.0129632175366,25.3193728413105));
#36293=CARTESIAN_POINT('Ctrl Pts',(53.5356670088646,22.9665462128381,25.3235950306749));
#36294=CARTESIAN_POINT('Ctrl Pts',(53.4711712001428,22.9168289578344,25.3278172200393));
#36295=CARTESIAN_POINT('Ctrl Pts',(53.4093693488068,22.8640934476267,25.3320394094037));
#36296=CARTESIAN_POINT('Ctrl Pts',(53.3469443861286,22.8108262366068,25.3363041685945));
#36297=CARTESIAN_POINT('Ctrl Pts',(53.2872683629448,22.7544798988007,25.3405689277853));
#36298=CARTESIAN_POINT('Ctrl Pts',(53.2306415662832,22.6953822527781,25.3448336869761));
#36299=CARTESIAN_POINT('Ctrl Pts',(53.1740147696215,22.6362846067556,25.3490984461669));
#36300=CARTESIAN_POINT('Ctrl Pts',(53.1204374663805,22.574436058744,25.3533632053577));
#36301=CARTESIAN_POINT('Ctrl Pts',(53.0701662876029,22.5101960443915,25.3576279645485));
#36302=CARTESIAN_POINT('Ctrl Pts',(53.0203123989143,22.4464892723848,25.3618573229035));
#36303=CARTESIAN_POINT('Ctrl Pts',(52.9735195039211,22.3801872905676,25.3660866812586));
#36304=CARTESIAN_POINT('Ctrl Pts',(52.930069306222,22.3116162445455,25.3703160396137));
#36305=CARTESIAN_POINT('Ctrl Pts',(52.8866800828081,22.2431414252551,25.3745394628495));
#36306=CARTESIAN_POINT('Ctrl Pts',(52.8466244911782,22.1724042513461,25.3787628860854));
#36307=CARTESIAN_POINT('Ctrl Pts',(52.8101436289925,22.0997633037877,25.3829863093213));
#36308=CARTESIAN_POINT('Ctrl Pts',(52.7737027894316,22.0272020495592,25.3872050991007));
#36309=CARTESIAN_POINT('Ctrl Pts',(52.7408290987219,21.9527415820618,25.3914238888802));
#36310=CARTESIAN_POINT('Ctrl Pts',(52.7117192342973,21.8767675788458,25.3956426786597));
#36311=CARTESIAN_POINT('Ctrl Pts',(52.6826311694021,21.8008504703471,25.3998583091105));
#36312=CARTESIAN_POINT('Ctrl Pts',(52.6573014986653,21.7234225098316,25.4040739395612));
#36313=CARTESIAN_POINT('Ctrl Pts',(52.6358794043523,21.6448907343375,25.408289570012));
#36314=CARTESIAN_POINT('Ctrl Pts',(52.6144670306404,21.5663945938309,25.4125032875563));
#36315=CARTESIAN_POINT('Ctrl Pts',(52.5969588308594,21.4867960817994,25.4167170051006));
#36316=CARTESIAN_POINT('Ctrl Pts',(52.5834541557757,21.4065174445975,25.4209307226449));
#36317=CARTESIAN_POINT('Ctrl Pts',(52.5699475313697,21.3262272196357,25.4251450484152));
#36318=CARTESIAN_POINT('Ctrl Pts',(52.5604456702665,21.2452571306903,25.4293593741854));
#36319=CARTESIAN_POINT('Ctrl Pts',(52.554996609532,21.1640386253292,25.4335736999556));
#36320=CARTESIAN_POINT('Ctrl Pts',(52.5512905675788,21.1087998965082,25.4364399678998));
#36321=CARTESIAN_POINT('Ctrl Pts',(52.5494581561907,21.053446442291,25.4393062358439));
#36322=CARTESIAN_POINT('Ctrl Pts',(52.5495007252096,20.9981147276813,25.442172503788));
#36323=CARTESIAN_POINT('',(52.5491673979362,20.9994536141197,26.2421724504355));
#36324=CARTESIAN_POINT('Ctrl Pts',(52.5517830077512,20.9980990070289,25.4421734099415));
#36325=CARTESIAN_POINT('Ctrl Pts',(52.5498278305076,20.7249505487043,25.4563360263802));
#36326=CARTESIAN_POINT('Ctrl Pts',(52.7180374006172,19.6374647203878,25.5128430743885));
#36327=CARTESIAN_POINT('Ctrl Pts',(54.3132510197648,18.1860561181197,25.6116945539665));
#36328=CARTESIAN_POINT('Ctrl Pts',(56.9920019014522,18.8971880273581,25.7387278486753));
#36329=CARTESIAN_POINT('Ctrl Pts',(57.8469697728126,21.5335586496174,25.8657611433844));
#36330=CARTESIAN_POINT('Ctrl Pts',(56.0953629013814,23.681434275856,25.9927944380933));
#36331=CARTESIAN_POINT('Ctrl Pts',(53.3748075180771,23.3780693189303,26.1182646831502));
#36332=CARTESIAN_POINT('Ctrl Pts',(52.5479892655699,21.7809080491335,26.2013904966373));
#36333=CARTESIAN_POINT('Ctrl Pts',(52.5456016115373,20.9994637759287,26.2421718785549));
#36334=CARTESIAN_POINT('',(52.682543123578,21.7964570772642,26.9999757050611));
#36335=CARTESIAN_POINT('Ctrl Pts',(52.5495000611252,20.9994526660932,26.242172503788));
#36336=CARTESIAN_POINT('Ctrl Pts',(52.5495067393017,20.9695534198073,26.2437353450291));
#36337=CARTESIAN_POINT('Ctrl Pts',(52.5500606104301,20.9396609804658,26.2452981862702));
#36338=CARTESIAN_POINT('Ctrl Pts',(52.5511610538356,20.9097887714958,26.2468610275113));
#36339=CARTESIAN_POINT('Ctrl Pts',(52.5541398745223,20.8289268629256,26.2510915256869));
#36340=CARTESIAN_POINT('Ctrl Pts',(52.5611337487646,20.7480607455217,26.2553220238625));
#36341=CARTESIAN_POINT('Ctrl Pts',(52.5721460426103,20.6676215837523,26.259552522038));
#36342=CARTESIAN_POINT('Ctrl Pts',(52.5831425394922,20.587297810706,26.26377695163));
#36343=CARTESIAN_POINT('Ctrl Pts',(52.598145945089,20.5074002338127,26.2680013812219));
#36344=CARTESIAN_POINT('Ctrl Pts',(52.6171076473889,20.4283582539146,26.2722258108139));
#36345=CARTESIAN_POINT('Ctrl Pts',(52.6361221281665,20.3490962665874,26.2764619987891));
#36346=CARTESIAN_POINT('Ctrl Pts',(52.6591169495656,20.2706951180793,26.2806981867644));
#36347=CARTESIAN_POINT('Ctrl Pts',(52.6859908382534,20.1935808476031,26.2849343747396));
#36348=CARTESIAN_POINT('Ctrl Pts',(52.712741926051,20.1168189526675,26.2891512053505));
#36349=CARTESIAN_POINT('Ctrl Pts',(52.7433365599026,20.0413326450863,26.2933680359615));
#36350=CARTESIAN_POINT('Ctrl Pts',(52.7776245398402,19.9675284197231,26.2975848665724));
#36351=CARTESIAN_POINT('Ctrl Pts',(52.8119012158823,19.8937485257802,26.301800306999));
#36352=CARTESIAN_POINT('Ctrl Pts',(52.8498686242415,19.8216500342973,26.3060157474256));
#36353=CARTESIAN_POINT('Ctrl Pts',(52.8913287446482,19.7516187333778,26.3102311878523));
#36354=CARTESIAN_POINT('Ctrl Pts',(52.9327879095229,19.6815890464709,26.3144465311256));
#36355=CARTESIAN_POINT('Ctrl Pts',(52.9777393885013,19.6136268550547,26.3186618743989));
#36356=CARTESIAN_POINT('Ctrl Pts',(53.0259403201985,19.5480913835292,26.3228772176722));
#36357=CARTESIAN_POINT('Ctrl Pts',(53.0745538377756,19.4819949475321,26.3271286430512));
#36358=CARTESIAN_POINT('Ctrl Pts',(53.1264724334857,19.418367372663,26.3313800684302));
#36359=CARTESIAN_POINT('Ctrl Pts',(53.1814048467678,19.3575439370746,26.3356314938092));
#36360=CARTESIAN_POINT('Ctrl Pts',(53.2359504452579,19.2971487987915,26.3398529821415));
#36361=CARTESIAN_POINT('Ctrl Pts',(53.2934671764026,19.239518722849,26.3440744704738));
#36362=CARTESIAN_POINT('Ctrl Pts',(53.3536334496469,19.184944234499,26.3482959588061));
#36363=CARTESIAN_POINT('Ctrl Pts',(53.4144397343252,19.1297892166487,26.3525623527085));
#36364=CARTESIAN_POINT('Ctrl Pts',(53.4779518868354,19.0777554876658,26.3568287466109));
#36365=CARTESIAN_POINT('Ctrl Pts',(53.543805961697,19.0290994005757,26.3610951405133));
#36366=CARTESIAN_POINT('Ctrl Pts',(53.6096600365586,18.9804433134857,26.3653615344157));
#36367=CARTESIAN_POINT('Ctrl Pts',(53.677855595404,18.93516508174,26.3696279283181));
#36368=CARTESIAN_POINT('Ctrl Pts',(53.7480028554,18.8934736175605,26.3738943222205));
#36369=CARTESIAN_POINT('Ctrl Pts',(53.8175864726838,18.8521171499291,26.3781264350714));
#36370=CARTESIAN_POINT('Ctrl Pts',(53.889351692782,18.8141347455355,26.3823585479223));
#36371=CARTESIAN_POINT('Ctrl Pts',(53.9629377574519,18.7797630407812,26.3865906607732));
#36372=CARTESIAN_POINT('Ctrl Pts',(54.0364182646889,18.7454406414074,26.3908167027604));
#36373=CARTESIAN_POINT('Ctrl Pts',(54.1117140113946,18.7147188497728,26.3950427447476));
#36374=CARTESIAN_POINT('Ctrl Pts',(54.1884375540172,18.6877896621911,26.3992687867348));
#36375=CARTESIAN_POINT('Ctrl Pts',(54.2653379730445,18.66079839278,26.4035045713262));
#36376=CARTESIAN_POINT('Ctrl Pts',(54.3436723692843,18.6376174674684,26.4077403559176));
#36377=CARTESIAN_POINT('Ctrl Pts',(54.4230281736965,18.6183926096747,26.4119761405091));
#36378=CARTESIAN_POINT('Ctrl Pts',(54.5020587700292,18.5992465372846,26.4161945664286));
#36379=CARTESIAN_POINT('Ctrl Pts',(54.5821019674695,18.5840242911116,26.4204129923482));
#36380=CARTESIAN_POINT('Ctrl Pts',(54.6627345151479,18.5728201049927,26.4246314182677));
#36381=CARTESIAN_POINT('Ctrl Pts',(54.7433403011021,18.5616196375129,26.4288484441031));
#36382=CARTESIAN_POINT('Ctrl Pts',(54.82453458892,18.5544346456498,26.4330654699385));
#36383=CARTESIAN_POINT('Ctrl Pts',(54.9058855980812,18.5513079553869,26.4372824957739));
#36384=CARTESIAN_POINT('Ctrl Pts',(54.9872345019779,18.5481813460389,26.4414994124778));
#36385=CARTESIAN_POINT('Ctrl Pts',(55.068739654742,18.5491128462283,26.4457163291817));
#36386=CARTESIAN_POINT('Ctrl Pts',(55.1499672776044,18.5540932017659,26.4499332458857));
#36387=CARTESIAN_POINT('Ctrl Pts',(55.2318231261238,18.5591120760612,26.454182776806));
#36388=CARTESIAN_POINT('Ctrl Pts',(55.3133966543977,18.568242694247,26.4584323077262));
#36389=CARTESIAN_POINT('Ctrl Pts',(55.3942490159461,18.5814223263609,26.4626818386465));
#36390=CARTESIAN_POINT('Ctrl Pts',(55.4745969115593,18.5945197261774,26.4669048552691));
#36391=CARTESIAN_POINT('Ctrl Pts',(55.5542321679018,18.611615600415,26.4711278718916));
#36392=CARTESIAN_POINT('Ctrl Pts',(55.6327360089674,18.6325973318939,26.4753508885141));
#36393=CARTESIAN_POINT('Ctrl Pts',(55.7119791820332,18.6537766647294,26.4796136765833));
#36394=CARTESIAN_POINT('Ctrl Pts',(55.7900690561176,18.6789152840031,26.4838764646525));
#36395=CARTESIAN_POINT('Ctrl Pts',(55.8665940424694,18.7078470784966,26.4881392527216));
#36396=CARTESIAN_POINT('Ctrl Pts',(55.9431190288212,18.7367788729901,26.4924020407908));
#36397=CARTESIAN_POINT('Ctrl Pts',(56.0180787129721,18.7695035922549,26.49666482886));
#36398=CARTESIAN_POINT('Ctrl Pts',(56.0910871936131,18.8058078967571,26.5009276169292));
#36399=CARTESIAN_POINT('Ctrl Pts',(56.1635699506814,18.8418507791821,26.5051597092743));
#36400=CARTESIAN_POINT('Ctrl Pts',(56.2344001739273,18.8815564034035,26.5093918016195));
#36401=CARTESIAN_POINT('Ctrl Pts',(56.3031834376743,18.9247498517597,26.5136238939646));
#36402=CARTESIAN_POINT('Ctrl Pts',(56.3718682972822,18.9678815058091,26.5178499317061));
#36403=CARTESIAN_POINT('Ctrl Pts',(56.4385116233919,19.0144908286332,26.5220759694475));
#36404=CARTESIAN_POINT('Ctrl Pts',(56.5027420427641,19.0643562820319,26.526302007189));
#36405=CARTESIAN_POINT('Ctrl Pts',(56.5671206489311,19.1143367806349,26.5305377948744));
#36406=CARTESIAN_POINT('Ctrl Pts',(56.6290747840083,19.1675882338332,26.5347735825597));
#36407=CARTESIAN_POINT('Ctrl Pts',(56.6882583461772,19.2238429105051,26.5390093702451));
#36408=CARTESIAN_POINT('Ctrl Pts',(56.7471998111796,19.2798674709534,26.5432278309539));
#36409=CARTESIAN_POINT('Ctrl Pts',(56.8033929800567,19.3388704181465,26.5474462916627));
#36410=CARTESIAN_POINT('Ctrl Pts',(56.8565292291881,19.4005471338079,26.5516647523715));
#36411=CARTESIAN_POINT('Ctrl Pts',(56.9096480251894,19.4622035911379,26.5558818274849));
#36412=CARTESIAN_POINT('Ctrl Pts',(56.95971159236,19.5265317210938,26.5600989025982));
#36413=CARTESIAN_POINT('Ctrl Pts',(57.0064498866016,19.5931918742925,26.5643159777116));
#36414=CARTESIAN_POINT('Ctrl Pts',(57.0531871300737,19.659850528839,26.5685329580168));
#36415=CARTESIAN_POINT('Ctrl Pts',(57.0965989834007,19.7288407212579,26.572749938322));
#36416=CARTESIAN_POINT('Ctrl Pts',(57.1364580866657,19.7997928954048,26.5769669186271));
#36417=CARTESIAN_POINT('Ctrl Pts',(57.1766245621654,19.8712922150352,26.5812164180447));
#36418=CARTESIAN_POINT('Ctrl Pts',(57.2131830074292,19.9447834979307,26.5854659174623));
#36419=CARTESIAN_POINT('Ctrl Pts',(57.2459482686662,20.0198639765444,26.5897154168799));
#36420=CARTESIAN_POINT('Ctrl Pts',(57.2785100903249,20.0944782803032,26.5939385311464));
#36421=CARTESIAN_POINT('Ctrl Pts',(57.3073255883373,20.1706616411086,26.5981616454129));
#36422=CARTESIAN_POINT('Ctrl Pts',(57.3322623959351,20.2480010860999,26.6023847596794));
#36423=CARTESIAN_POINT('Ctrl Pts',(57.3574329036161,20.3260653325581,26.6066474516726));
#36424=CARTESIAN_POINT('Ctrl Pts',(57.3786515154079,20.4053069781661,26.6109101436657));
#36425=CARTESIAN_POINT('Ctrl Pts',(57.3958347250919,20.4852901593674,26.6151728356589));
#36426=CARTESIAN_POINT('Ctrl Pts',(57.4130179347758,20.5652733405687,26.619435527652));
#36427=CARTESIAN_POINT('Ctrl Pts',(57.4261657282633,20.6459975734496,26.6236982196452));
#36428=CARTESIAN_POINT('Ctrl Pts',(57.4352482010145,20.727022987313,26.6279609116383));
#36429=CARTESIAN_POINT('Ctrl Pts',(57.4442524333069,20.8073504122328,26.6321868829072));
#36430=CARTESIAN_POINT('Ctrl Pts',(57.4492950829039,20.8882766980863,26.6364128541761));
#36431=CARTESIAN_POINT('Ctrl Pts',(57.4503086474803,20.9693767721592,26.640638825445));
#36432=CARTESIAN_POINT('Ctrl Pts',(57.4513207538296,21.0503601666194,26.6448587167602));
#36433=CARTESIAN_POINT('Ctrl Pts',(57.4483152812012,21.1315163906118,26.6490786080755));
#36434=CARTESIAN_POINT('Ctrl Pts',(57.4412763855329,21.2124143578939,26.6532984993907));
#36435=CARTESIAN_POINT('Ctrl Pts',(57.4342084164619,21.2936464655432,26.6575358205139));
#36436=CARTESIAN_POINT('Ctrl Pts',(57.4230735756371,21.3746177053289,26.6617731416371));
#36437=CARTESIAN_POINT('Ctrl Pts',(57.4079087777954,21.4548907207405,26.6660104627603));
#36438=CARTESIAN_POINT('Ctrl Pts',(57.3928335373729,21.5346896748314,26.670222759907));
#36439=CARTESIAN_POINT('Ctrl Pts',(57.3737758937374,21.6137981655812,26.6744350570538));
#36440=CARTESIAN_POINT('Ctrl Pts',(57.3508239366155,21.6917926488737,26.6786473542005));
#36441=CARTESIAN_POINT('Ctrl Pts',(57.3278794911986,21.7697616061708,26.6828582727487));
#36442=CARTESIAN_POINT('Ctrl Pts',(57.3010433946186,21.8466168330897,26.687069191297));
#36443=CARTESIAN_POINT('Ctrl Pts',(57.2704540986355,21.9219481742427,26.6912801098452));
#36444=CARTESIAN_POINT('Ctrl Pts',(57.2398653813777,21.997278090186,26.6954909487262));
#36445=CARTESIAN_POINT('Ctrl Pts',(57.2055237823416,22.0710837461625,26.6997017876071));
#36446=CARTESIAN_POINT('Ctrl Pts',(57.1676160316486,22.1429746232266,26.7039126264881));
#36447=CARTESIAN_POINT('Ctrl Pts',(57.1292945346533,22.21565015736,26.7081694248097));
#36448=CARTESIAN_POINT('Ctrl Pts',(57.0873287762015,22.286368421148,26.7124262231313));
#36449=CARTESIAN_POINT('Ctrl Pts',(57.0419586006651,22.3547528642412,26.7166830214529));
#36450=CARTESIAN_POINT('Ctrl Pts',(56.997011838929,22.4224991145881,26.7209000935197));
#36451=CARTESIAN_POINT('Ctrl Pts',(56.9487242697108,22.4879545818773,26.7251171655865));
#36452=CARTESIAN_POINT('Ctrl Pts',(56.897370724117,22.5507851512262,26.7293342376532));
#36453=CARTESIAN_POINT('Ctrl Pts',(56.8452915266946,22.6145035486114,26.7336108991022));
#36454=CARTESIAN_POINT('Ctrl Pts',(56.7900593633578,22.6755219190545,26.7378875605512));
#36455=CARTESIAN_POINT('Ctrl Pts',(56.7319993586573,22.7335306376325,26.7421642220002));
#36456=CARTESIAN_POINT('Ctrl Pts',(56.6739393539568,22.7915393562106,26.7464408834492));
#36457=CARTESIAN_POINT('Ctrl Pts',(56.6130519184716,22.8465381425506,26.7507175448982));
#36458=CARTESIAN_POINT('Ctrl Pts',(56.5496951052037,22.8982611334871,26.7549942063472));
#36459=CARTESIAN_POINT('Ctrl Pts',(56.4868952408543,22.9495294446129,26.7592332730713));
#36460=CARTESIAN_POINT('Ctrl Pts',(56.4214326579385,22.9977725913542,26.7634723397953));
#36461=CARTESIAN_POINT('Ctrl Pts',(56.3536303884841,23.0427028715338,26.7677114065194));
#36462=CARTESIAN_POINT('Ctrl Pts',(56.2859254991731,23.0875686211724,26.771944384938));
#36463=CARTESIAN_POINT('Ctrl Pts',(56.2158879807024,23.1291307013787,26.7761773633566));
#36464=CARTESIAN_POINT('Ctrl Pts',(56.1438738006428,23.1671416608526,26.7804103417752));
#36465=CARTESIAN_POINT('Ctrl Pts',(56.0718414190082,23.2051622275918,26.7846443900786));
#36466=CARTESIAN_POINT('Ctrl Pts',(55.9978317530468,23.2396296051631,26.788878438382));
#36467=CARTESIAN_POINT('Ctrl Pts',(55.9222300314476,23.2703396263767,26.7931124866853));
#36468=CARTESIAN_POINT('Ctrl Pts',(55.846785064203,23.3009859727233,26.7973377560152));
#36469=CARTESIAN_POINT('Ctrl Pts',(55.7697550562113,23.327890330548,26.8015630253451));
#36470=CARTESIAN_POINT('Ctrl Pts',(55.6915457231059,23.3508965870182,26.805788294675));
#36471=CARTESIAN_POINT('Ctrl Pts',(55.6133632373863,23.3738949459932,26.8100121135714));
#36472=CARTESIAN_POINT('Ctrl Pts',(55.5340026744714,23.3929977306962,26.8142359324678));
#36473=CARTESIAN_POINT('Ctrl Pts',(55.453885790929,23.408098407207,26.8184597513642));
#36474=CARTESIAN_POINT('Ctrl Pts',(55.3737721059884,23.4231984808355,26.8226834016281));
#36475=CARTESIAN_POINT('Ctrl Pts',(55.2929026156913,23.4342966792029,26.8269070518919));
#36476=CARTESIAN_POINT('Ctrl Pts',(55.2117087794886,23.4413376748593,26.8311307021558));
#36477=CARTESIAN_POINT('Ctrl Pts',(55.1301737309127,23.4484082598903,26.8353721020641));
#36478=CARTESIAN_POINT('Ctrl Pts',(55.0483120716804,23.4513874126894,26.8396135019725));
#36479=CARTESIAN_POINT('Ctrl Pts',(54.9665636225421,23.4502718744381,26.8438549018809));
#36480=CARTESIAN_POINT('Ctrl Pts',(54.8850438303021,23.4491594564358,26.8480844382572));
#36481=CARTESIAN_POINT('Ctrl Pts',(54.803637078279,23.4439752929518,26.8523139746335));
#36482=CARTESIAN_POINT('Ctrl Pts',(54.7227753986737,23.4347683196599,26.8565435110098));
#36483=CARTESIAN_POINT('Ctrl Pts',(54.6415735026559,23.4255226090645,26.8607908426842));
#36484=CARTESIAN_POINT('Ctrl Pts',(54.560921738975,23.4122202445618,26.8650381743587));
#36485=CARTESIAN_POINT('Ctrl Pts',(54.4812464891015,23.3949624307973,26.8692855060331));
#36486=CARTESIAN_POINT('Ctrl Pts',(54.401571239228,23.3777046170328,26.8735328377075));
#36487=CARTESIAN_POINT('Ctrl Pts',(54.3228729380817,23.3564915329934,26.8777801693819));
#36488=CARTESIAN_POINT('Ctrl Pts',(54.2455601136359,23.3314739346308,26.8820275010563));
#36489=CARTESIAN_POINT('Ctrl Pts',(54.169285408542,23.3067922605238,26.8862178016076));
#36490=CARTESIAN_POINT('Ctrl Pts',(54.0940686995614,23.2783134695851,26.890408102159));
#36491=CARTESIAN_POINT('Ctrl Pts',(54.0203200073828,23.2461472262667,26.8945984027103));
#36492=CARTESIAN_POINT('Ctrl Pts',(53.9430439450967,23.2124424845451,26.8989891236416));
#36493=CARTESIAN_POINT('Ctrl Pts',(53.867380360135,23.1746887917181,26.9033798445729));
#36494=CARTESIAN_POINT('Ctrl Pts',(53.7937845128205,23.1330715994753,26.9077705655042));
#36495=CARTESIAN_POINT('Ctrl Pts',(53.7237284891418,23.0934561169232,26.9119501009094));
#36496=CARTESIAN_POINT('Ctrl Pts',(53.655546373461,23.0503404512337,26.9161296363146));
#36497=CARTESIAN_POINT('Ctrl Pts',(53.5896096017808,23.0039334256934,26.9203091717198));
#36498=CARTESIAN_POINT('Ctrl Pts',(53.5237109517532,22.9575532305916,26.9244862907071));
#36499=CARTESIAN_POINT('Ctrl Pts',(53.4600554572414,22.9078857240475,26.9286634096944));
#36500=CARTESIAN_POINT('Ctrl Pts',(53.3989867597946,22.8551837792216,26.9328405286817));
#36501=CARTESIAN_POINT('Ctrl Pts',(53.3379337749728,22.8024953943033,26.9370165729203));
#36502=CARTESIAN_POINT('Ctrl Pts',(53.2794666247867,22.7467744315117,26.9411926171589));
#36503=CARTESIAN_POINT('Ctrl Pts',(53.2238957157063,22.688313898928,26.9453686613975));
#36504=CARTESIAN_POINT('Ctrl Pts',(53.1683212744554,22.629849650505,26.9495449710717));
#36505=CARTESIAN_POINT('Ctrl Pts',(53.1156437649222,22.5686458324901,26.9537212807459));
#36506=CARTESIAN_POINT('Ctrl Pts',(53.0661354820089,22.5050309884036,26.9578975904202));
#36507=CARTESIAN_POINT('Ctrl Pts',(53.0165789796522,22.4413541855458,26.962077967683));
#36508=CARTESIAN_POINT('Ctrl Pts',(52.9701981548031,22.3752620463761,26.9662583449458));
#36509=CARTESIAN_POINT('Ctrl Pts',(52.9272233588278,22.3071140905869,26.9704387222087));
#36510=CARTESIAN_POINT('Ctrl Pts',(52.8842240998105,22.2389273421457,26.9746214791162));
#36511=CARTESIAN_POINT('Ctrl Pts',(52.8446349593748,22.1686828624283,26.9788042360237));
#36512=CARTESIAN_POINT('Ctrl Pts',(52.8086402700108,22.0967646893393,26.9829869929312));
#36513=CARTESIAN_POINT('Ctrl Pts',(52.7725900071155,22.0247354791248,26.9871762077517));
#36514=CARTESIAN_POINT('Ctrl Pts',(52.7401454567778,21.9510278541624,26.9913654225722));
#36515=CARTESIAN_POINT('Ctrl Pts',(52.7114425093182,21.8760450113118,26.9955546373927));
#36516=CARTESIAN_POINT('Ctrl Pts',(52.7013453369014,21.8496674173858,26.9970283266155));
#36517=CARTESIAN_POINT('Ctrl Pts',(52.6917107340805,21.8231321393686,26.9985020158383));
#36518=CARTESIAN_POINT('Ctrl Pts',(52.682543123578,21.7964570772642,26.9999757050611));
#36519=CARTESIAN_POINT('',(54.2031000556071,23.3173046257725,27.));
#36520=CARTESIAN_POINT('Origin',(55.,21.,27.));
#36521=CARTESIAN_POINT('',(52.5485180219995,20.9992126141703,26.3578274962121));
#36522=CARTESIAN_POINT('Ctrl Pts',(54.203100055607,23.3173046257725,27.));
#36523=CARTESIAN_POINT('Ctrl Pts',(54.9737715883742,23.5823315431561,26.9576555684304));
#36524=CARTESIAN_POINT('Ctrl Pts',(56.7871288453655,23.2781442292576,26.872966705291));
#36525=CARTESIAN_POINT('Ctrl Pts',(57.8856565523512,20.7291287202087,26.745933410582));
#36526=CARTESIAN_POINT('Ctrl Pts',(56.3358056379254,18.430681285051,26.618900115873));
#36527=CARTESIAN_POINT('Ctrl Pts',(53.5661178804319,18.4833632214424,26.4918668211641));
#36528=CARTESIAN_POINT('Ctrl Pts',(52.5669730182605,20.0983171962907,26.4048426146105));
#36529=CARTESIAN_POINT('Ctrl Pts',(52.5455281581047,20.9544531196991,26.3601628396264));
#36530=CARTESIAN_POINT('Ctrl Pts',(52.5457196275622,20.9992117153605,26.3578274962121));
#36531=CARTESIAN_POINT('',(52.5495006168754,20.9982612343869,25.557827496241));
#36532=CARTESIAN_POINT('Ctrl Pts',(52.5495001263987,20.9992129296102,26.3578274962121));
#36533=CARTESIAN_POINT('Ctrl Pts',(52.5494743355874,21.0795111858266,26.3536313506362));
#36534=CARTESIAN_POINT('Ctrl Pts',(52.5533996345101,21.1599691050755,26.3494352050602));
#36535=CARTESIAN_POINT('Ctrl Pts',(52.5612969373346,21.2401616583602,26.3452390594843));
#36536=CARTESIAN_POINT('Ctrl Pts',(52.5691832420487,21.3202425321801,26.3410487576341));
#36537=CARTESIAN_POINT('Ctrl Pts',(52.581030522992,21.4000583066965,26.3368584557839));
#36538=CARTESIAN_POINT('Ctrl Pts',(52.596807678344,21.4791835923042,26.3326681539338));
#36539=CARTESIAN_POINT('Ctrl Pts',(52.6125678008879,21.5582234553005,26.328482375878));
#36540=CARTESIAN_POINT('Ctrl Pts',(52.6322492777825,21.6365738483382,26.3242965978223));
#36541=CARTESIAN_POINT('Ctrl Pts',(52.6557693381687,21.7138157003947,26.3201108197666));
#36542=CARTESIAN_POINT('Ctrl Pts',(52.679275888901,21.7910131856141,26.3159274459739));
#36543=CARTESIAN_POINT('Ctrl Pts',(52.7066165106108,21.8671029415645,26.3117440721813));
#36544=CARTESIAN_POINT('Ctrl Pts',(52.7376579070066,21.9416785567647,26.3075606983886));
#36545=CARTESIAN_POINT('Ctrl Pts',(52.768691371173,22.0162351151259,26.3033783936033));
#36546=CARTESIAN_POINT('Ctrl Pts',(52.8034235504787,22.0892778642556,26.299196088818));
#36547=CARTESIAN_POINT('Ctrl Pts',(52.8416726362047,22.1604194244723,26.2950137840327));
#36548=CARTESIAN_POINT('Ctrl Pts',(52.8799241435921,22.2315654888688,26.2908312144534));
#36549=CARTESIAN_POINT('Ctrl Pts',(52.9216927733975,22.3008097095626,26.2866486448742));
#36550=CARTESIAN_POINT('Ctrl Pts',(52.9667510390727,22.3677897911916,26.282466075295));
#36551=CARTESIAN_POINT('Ctrl Pts',(53.0118554409332,22.434838455253,26.2782792230874));
#36552=CARTESIAN_POINT('Ctrl Pts',(53.0602559369734,22.499617959663,26.2740923708799));
#36553=CARTESIAN_POINT('Ctrl Pts',(53.1116824370535,22.5617960915138,26.2699055186723));
#36554=CARTESIAN_POINT('Ctrl Pts',(53.1631379050008,22.6240092474837,26.2657163080663));
#36555=CARTESIAN_POINT('Ctrl Pts',(53.2176224490737,22.6836177662396,26.2615270974603));
#36556=CARTESIAN_POINT('Ctrl Pts',(53.2748282562834,22.7403254594132,26.2573378868542));
#36557=CARTESIAN_POINT('Ctrl Pts',(53.3321296921619,22.7971279485783,26.2531416733117));
#36558=CARTESIAN_POINT('Ctrl Pts',(53.3921611187412,22.8510196177861,26.2489454597692));
#36559=CARTESIAN_POINT('Ctrl Pts',(53.4545811722834,22.9017441723163,26.2447492462267));
#36560=CARTESIAN_POINT('Ctrl Pts',(53.4890374625839,22.9297444683282,26.2424329080665));
#36561=CARTESIAN_POINT('Ctrl Pts',(53.5242210620795,22.9567804653042,26.2401165699063));
#36562=CARTESIAN_POINT('Ctrl Pts',(53.5600710532226,22.9828148875355,26.2378002317461));
#36563=CARTESIAN_POINT('Ctrl Pts',(53.6255700198798,23.0303805270042,26.2335682151936));
#36564=CARTESIAN_POINT('Ctrl Pts',(53.6935506530067,23.0747859913906,26.2293361986411));
#36565=CARTESIAN_POINT('Ctrl Pts',(53.7636753302762,23.1157626428861,26.2251041820886));
#36566=CARTESIAN_POINT('Ctrl Pts',(53.8336997560659,23.1566807134353,26.2208782157019));
#36567=CARTESIAN_POINT('Ctrl Pts',(53.9058617403943,23.1941794742577,26.2166522493152));
#36568=CARTESIAN_POINT('Ctrl Pts',(53.979793008219,23.2280323031593,26.2124262829285));
#36569=CARTESIAN_POINT('Ctrl Pts',(54.0538964167674,23.2619639546028,26.2081904768497));
#36570=CARTESIAN_POINT('Ctrl Pts',(54.1297769710899,23.2922324063916,26.2039546707709));
#36571=CARTESIAN_POINT('Ctrl Pts',(54.207037125881,23.3186548105031,26.1997188646921));
#36572=CARTESIAN_POINT('Ctrl Pts',(54.2839798177425,23.3449686446299,26.1955004635927));
#36573=CARTESIAN_POINT('Ctrl Pts',(54.3622903557061,23.367467815414,26.1912820624934));
#36574=CARTESIAN_POINT('Ctrl Pts',(54.4415558711848,23.3860197830261,26.187063661394));
#36575=CARTESIAN_POINT('Ctrl Pts',(54.5207954381148,23.4045656774217,26.1828466412406));
#36576=CARTESIAN_POINT('Ctrl Pts',(54.6009889095858,23.4191668289195,26.1786296210871));
#36577=CARTESIAN_POINT('Ctrl Pts',(54.6817102262335,23.4297411117063,26.1744126009336));
#36578=CARTESIAN_POINT('Ctrl Pts',(54.7624298199797,23.4403151687975,26.1701956707875));
#36579=CARTESIAN_POINT('Ctrl Pts',(54.8436767755754,23.4468624688256,26.1659787406413));
#36580=CARTESIAN_POINT('Ctrl Pts',(54.9250182856289,23.4493525659876,26.1617618104952));
#36581=CARTESIAN_POINT('Ctrl Pts',(55.0069894484636,23.451861938629,26.157512237707));
#36582=CARTESIAN_POINT('Ctrl Pts',(55.0890561580517,23.4502509915335,26.1532626649189));
#36583=CARTESIAN_POINT('Ctrl Pts',(55.1707756721488,23.4445420675051,26.1490130921307));
#36584=CARTESIAN_POINT('Ctrl Pts',(55.251985666481,23.4388687385198,26.1447900153558));
#36585=CARTESIAN_POINT('Ctrl Pts',(55.3328523239207,23.4291485044898,26.1405669385809));
#36586=CARTESIAN_POINT('Ctrl Pts',(55.4129483312974,23.4154552212117,26.1363438618059));
#36587=CARTESIAN_POINT('Ctrl Pts',(55.4937981344202,23.4016330683553,26.1320810410111));
#36588=CARTESIAN_POINT('Ctrl Pts',(55.5738622334867,23.3837627967394,26.1278182202163));
#36589=CARTESIAN_POINT('Ctrl Pts',(55.6527155994374,23.3619721836319,26.1235553994216));
#36590=CARTESIAN_POINT('Ctrl Pts',(55.7315689653882,23.3401815705244,26.1192925786268));
#36591=CARTESIAN_POINT('Ctrl Pts',(55.8092111626853,23.3144708275666,26.115029757832));
#36592=CARTESIAN_POINT('Ctrl Pts',(55.8852384319867,23.2850171046479,26.1107669370372));
#36593=CARTESIAN_POINT('Ctrl Pts',(55.9606899593003,23.2557864299216,26.1065363978821));
#36594=CARTESIAN_POINT('Ctrl Pts',(56.0348340446258,23.2227596316656,26.1023058587271));
#36595=CARTESIAN_POINT('Ctrl Pts',(56.10726206758,23.1860743271212,26.098075319572));
#36596=CARTESIAN_POINT('Ctrl Pts',(56.1795860444293,23.149441722663,26.0938508577763));
#36597=CARTESIAN_POINT('Ctrl Pts',(56.2501984435353,23.1091612582058,26.0896263959806));
#36598=CARTESIAN_POINT('Ctrl Pts',(56.3187092839997,23.0654191037881,26.0854019341848));
#36599=CARTESIAN_POINT('Ctrl Pts',(56.3874101471757,23.0215556254641,26.0811657553575));
#36600=CARTESIAN_POINT('Ctrl Pts',(56.4539973385911,22.9742114027611,26.0769295765301));
#36601=CARTESIAN_POINT('Ctrl Pts',(56.5181012589417,22.9236212770708,26.0726933977028));
#36602=CARTESIAN_POINT('Ctrl Pts',(56.5819125540839,22.8732620880533,26.0684765564246));
#36603=CARTESIAN_POINT('Ctrl Pts',(56.6432628283119,22.8196868501988,26.0642597151464));
#36604=CARTESIAN_POINT('Ctrl Pts',(56.7018169237209,22.7631702720206,26.0600428738682));
#36605=CARTESIAN_POINT('Ctrl Pts',(56.7603516026685,22.7066724346657,26.0558274308891));
#36606=CARTESIAN_POINT('Ctrl Pts',(56.8160916097042,22.6472355166042,26.05161198791));
#36607=CARTESIAN_POINT('Ctrl Pts',(56.8687369733639,22.5851726639021,26.0473965449308));
#36608=CARTESIAN_POINT('Ctrl Pts',(56.9213810224365,22.5231113609478,26.0431812072139));
#36609=CARTESIAN_POINT('Ctrl Pts',(56.9709302817531,22.4584246091144,26.038965869497));
#36610=CARTESIAN_POINT('Ctrl Pts',(57.017124529458,22.3914592637439,26.0347505317801));
#36611=CARTESIAN_POINT('Ctrl Pts',(57.0637140513964,22.3239209103288,26.0304991243257));
#36612=CARTESIAN_POINT('Ctrl Pts',(57.1068905822333,22.2540651667685,26.0262477168714));
#36613=CARTESIAN_POINT('Ctrl Pts',(57.1464323385103,22.1822768145392,26.0219963094171));
#36614=CARTESIAN_POINT('Ctrl Pts',(57.185695585155,22.1109940986164,26.0177748464579));
#36615=CARTESIAN_POINT('Ctrl Pts',(57.2213749463101,22.0378063609927,26.0135533834986));
#36616=CARTESIAN_POINT('Ctrl Pts',(57.2533008416306,21.9631124374166,26.0093319205394));
#36617=CARTESIAN_POINT('Ctrl Pts',(57.2855664313269,21.887623763827,26.0050655408375));
#36618=CARTESIAN_POINT('Ctrl Pts',(57.313998038042,21.8105971193485,26.0007991611357));
#36619=CARTESIAN_POINT('Ctrl Pts',(57.3384722095208,21.7324602209669,25.9965327814338));
#36620=CARTESIAN_POINT('Ctrl Pts',(57.3629463809996,21.6543233225853,25.9922664017319));
#36621=CARTESIAN_POINT('Ctrl Pts',(57.383463058575,21.5750766543416,25.98800002203));
#36622=CARTESIAN_POINT('Ctrl Pts',(57.3999520678217,21.4951568662136,25.9837336423281));
#36623=CARTESIAN_POINT('Ctrl Pts',(57.4163058464752,21.4158925207623,25.9795022523002));
#36624=CARTESIAN_POINT('Ctrl Pts',(57.4287591978242,21.335668594493,25.9752708622723));
#36625=CARTESIAN_POINT('Ctrl Pts',(57.4372063082182,21.25490323886,25.9710394722444));
#36626=CARTESIAN_POINT('Ctrl Pts',(57.4456413088147,21.174253668633,25.9668141483473));
#36627=CARTESIAN_POINT('Ctrl Pts',(57.4500814272728,21.0930646690861,25.9625888244503));
#36628=CARTESIAN_POINT('Ctrl Pts',(57.450471757429,21.0117650347583,25.9583635005532));
#36629=CARTESIAN_POINT('Ctrl Pts',(57.4508630705698,20.930260660188,25.9541275358476));
#36630=CARTESIAN_POINT('Ctrl Pts',(57.4471840837195,20.8486455564067,25.949891571142));
#36631=CARTESIAN_POINT('Ctrl Pts',(57.4394318362206,20.7673574277278,25.9456556064364));
#36632=CARTESIAN_POINT('Ctrl Pts',(57.4317129704213,20.6864193312027,25.94143788208));
#36633=CARTESIAN_POINT('Ctrl Pts',(57.4199558870623,20.6058058660911,25.9372201577235));
#36634=CARTESIAN_POINT('Ctrl Pts',(57.4042097873049,20.525947736397,25.9330024333671));
#36635=CARTESIAN_POINT('Ctrl Pts',(57.3884688856889,20.4461159696657,25.9287861013763));
#36636=CARTESIAN_POINT('Ctrl Pts',(57.3687416726496,20.367039498909,25.9245697693854));
#36637=CARTESIAN_POINT('Ctrl Pts',(57.3451287228792,20.2891402929362,25.9203534373945));
#36638=CARTESIAN_POINT('Ctrl Pts',(57.3215163360887,20.2112429442359,25.9161372059294));
#36639=CARTESIAN_POINT('Ctrl Pts',(57.2940185326838,20.1345232490794,25.9119209744644));
#36640=CARTESIAN_POINT('Ctrl Pts',(57.2627857615478,20.0593880463568,25.9077047429993));
#36641=CARTESIAN_POINT('Ctrl Pts',(57.2313001283659,19.9836445453505,25.9034543767176));
#36642=CARTESIAN_POINT('Ctrl Pts',(57.1960189436645,19.9095117590793,25.8992040104359));
#36643=CARTESIAN_POINT('Ctrl Pts',(57.1571450758474,19.8373842544729,25.8949536441542));
#36644=CARTESIAN_POINT('Ctrl Pts',(57.118527360474,19.7657320212406,25.8907312849058));
#36645=CARTESIAN_POINT('Ctrl Pts',(57.0763644619894,19.6960590920095,25.8865089256575));
#36646=CARTESIAN_POINT('Ctrl Pts',(57.0308996285668,19.6287243352676,25.8822865664091));
#36647=CARTESIAN_POINT('Ctrl Pts',(56.9849824407749,19.5607196283879,25.8780221966108));
#36648=CARTESIAN_POINT('Ctrl Pts',(56.935697539068,19.4951002681144,25.8737578268124));
#36649=CARTESIAN_POINT('Ctrl Pts',(56.8833368420662,19.4322013556212,25.8694934570141));
#36650=CARTESIAN_POINT('Ctrl Pts',(56.8309761450644,19.369302443128,25.8652290872158));
#36651=CARTESIAN_POINT('Ctrl Pts',(56.7755400261528,19.3091242890382,25.8609647174175));
#36652=CARTESIAN_POINT('Ctrl Pts',(56.7173567069577,19.2519621883187,25.8567003476191));
#36653=CARTESIAN_POINT('Ctrl Pts',(56.6596245349327,19.1952433163516,25.8524690432835));
#36654=CARTESIAN_POINT('Ctrl Pts',(56.5989712868893,19.1412812952135,25.8482377389478));
#36655=CARTESIAN_POINT('Ctrl Pts',(56.5356909213767,19.0903917564063,25.8440064346121));
#36656=CARTESIAN_POINT('Ctrl Pts',(56.4725012636275,19.039575164021,25.8397811955408));
#36657=CARTESIAN_POINT('Ctrl Pts',(56.4066923267724,18.9918225958151,25.8355559564696));
#36658=CARTESIAN_POINT('Ctrl Pts',(56.3385946155272,18.9474126802297,25.8313307173984));
#36659=CARTESIAN_POINT('Ctrl Pts',(56.2703236968907,18.9028898074615,25.827094731378));
#36660=CARTESIAN_POINT('Ctrl Pts',(56.1997526873778,18.8617269389932,25.8228587453577));
#36661=CARTESIAN_POINT('Ctrl Pts',(56.1272477717193,18.8241639052645,25.8186227593374));
#36662=CARTESIAN_POINT('Ctrl Pts',(56.0550568347439,18.7867635362566,25.8144051170293));
#36663=CARTESIAN_POINT('Ctrl Pts',(55.9809491178069,18.7529321114306,25.8101874747213));
#36664=CARTESIAN_POINT('Ctrl Pts',(55.9053131801079,18.7228618188782,25.8059698324132));
#36665=CARTESIAN_POINT('Ctrl Pts',(55.82970218982,18.6928014445732,25.801753581233));
#36666=CARTESIAN_POINT('Ctrl Pts',(55.7525644114385,18.6664999105888,25.7975373300528));
#36667=CARTESIAN_POINT('Ctrl Pts',(55.6743089198722,18.6441015024877,25.7933210788725));
#36668=CARTESIAN_POINT('Ctrl Pts',(55.5960552689602,18.6217036212215,25.7891049268631));
#36669=CARTESIAN_POINT('Ctrl Pts',(55.5166844043928,18.603208810164,25.7848887748537));
#36670=CARTESIAN_POINT('Ctrl Pts',(55.4366197304326,18.5887112447911,25.7806726228443));
#36671=CARTESIAN_POINT('Ctrl Pts',(55.3559034691396,18.5740956944257,25.7764221586831));
#36672=CARTESIAN_POINT('Ctrl Pts',(55.2744825229026,18.5635428507918,25.7721716945219));
#36673=CARTESIAN_POINT('Ctrl Pts',(55.1927984612472,18.5570961944152,25.7679212303608));
#36674=CARTESIAN_POINT('Ctrl Pts',(55.1116559575289,18.5506922787871,25.7636989463923));
#36675=CARTESIAN_POINT('Ctrl Pts',(55.0302542877551,18.5483402197066,25.7594766624239));
#36676=CARTESIAN_POINT('Ctrl Pts',(54.9490268651635,18.5500302064056,25.7552543784555));
#36677=CARTESIAN_POINT('Ctrl Pts',(54.8669862555232,18.5517371119635,25.750989824198));
#36678=CARTESIAN_POINT('Ctrl Pts',(54.7851238857998,18.5575674128837,25.7467252699404));
#36679=CARTESIAN_POINT('Ctrl Pts',(54.7038796664837,18.5674575033356,25.7424607156829));
#36680=CARTESIAN_POINT('Ctrl Pts',(54.6226354471676,18.5773475937875,25.7381961614254));
#36681=CARTESIAN_POINT('Ctrl Pts',(54.5420098418629,18.5912973283797,25.7339316071678));
#36682=CARTESIAN_POINT('Ctrl Pts',(54.4624289921549,18.6091910027097,25.7296670529103));
#36683=CARTESIAN_POINT('Ctrl Pts',(54.3834718846294,18.6269444292348,25.7254359235582));
#36684=CARTESIAN_POINT('Ctrl Pts',(54.3052470881391,18.6486467291004,25.7212047942062));
#36685=CARTESIAN_POINT('Ctrl Pts',(54.2281791718382,18.6742220958966,25.7169736648541));
#36686=CARTESIAN_POINT('Ctrl Pts',(54.1512217936304,18.6997607800834,25.7127486041879));
#36687=CARTESIAN_POINT('Ctrl Pts',(54.0754184376643,18.7291613531296,25.7085235435216));
#36688=CARTESIAN_POINT('Ctrl Pts',(54.0011824034266,18.7622972362766,25.7042984828554));
#36689=CARTESIAN_POINT('Ctrl Pts',(53.9267536301263,18.7955191501379,25.7000624526614));
#36690=CARTESIAN_POINT('Ctrl Pts',(53.8539007868142,18.8324956855936,25.6958264224675));
#36691=CARTESIAN_POINT('Ctrl Pts',(53.7830239881532,18.8730492162277,25.6915903922736));
#36692=CARTESIAN_POINT('Ctrl Pts',(53.7124579563411,18.9134249356011,25.6873729354038));
#36693=CARTESIAN_POINT('Ctrl Pts',(53.6438510873143,18.9573461231155,25.683155478534));
#36694=CARTESIAN_POINT('Ctrl Pts',(53.5775755357257,19.0045905449172,25.6789380216642));
#36695=CARTESIAN_POINT('Ctrl Pts',(53.5113218803221,19.0518193580581,25.6747219581622));
#36696=CARTESIAN_POINT('Ctrl Pts',(53.4473983911052,19.1023689554765,25.6705058946601));
#36697=CARTESIAN_POINT('Ctrl Pts',(53.3861481003195,19.1559738895836,25.6662898311581));
#36698=CARTESIAN_POINT('Ctrl Pts',(53.324899279199,19.2095775374713,25.662073868818));
#36699=CARTESIAN_POINT('Ctrl Pts',(53.2663238781257,19.2662360692495,25.657857906478));
#36700=CARTESIAN_POINT('Ctrl Pts',(53.2107305969442,19.32564482463,25.653641944138));
#36701=CARTESIAN_POINT('Ctrl Pts',(53.1546794870073,19.3855428304371,25.6493912619766));
#36702=CARTESIAN_POINT('Ctrl Pts',(53.1016601821046,19.4482362287982,25.6451405798152));
#36703=CARTESIAN_POINT('Ctrl Pts',(53.0519487152839,19.5133775051762,25.6408898976538));
#36704=CARTESIAN_POINT('Ctrl Pts',(53.0025716166071,19.5780806297744,25.6366678063346));
#36705=CARTESIAN_POINT('Ctrl Pts',(52.9564582090912,19.6451983815589,25.6324457150154));
#36706=CARTESIAN_POINT('Ctrl Pts',(52.9138352448007,19.7143613010786,25.6282236236962));
#36707=CARTESIAN_POINT('Ctrl Pts',(52.8707793340077,19.7842267490267,25.6239586461137));
#36708=CARTESIAN_POINT('Ctrl Pts',(52.8312854112849,19.8561787221728,25.6196936685312));
#36709=CARTESIAN_POINT('Ctrl Pts',(52.7955386279351,19.9298129560334,25.6154286909487));
#36710=CARTESIAN_POINT('Ctrl Pts',(52.7597918445854,20.0034471898942,25.6111637133662));
#36711=CARTESIAN_POINT('Ctrl Pts',(52.727792329923,20.078763215713,25.6068987357837));
#36712=CARTESIAN_POINT('Ctrl Pts',(52.6996739643788,20.1553400803617,25.6026337582012));
#36713=CARTESIAN_POINT('Ctrl Pts',(52.667503705164,20.2429517725044,25.5977541917072));
#36714=CARTESIAN_POINT('Ctrl Pts',(52.6403127382136,20.3324844781953,25.5928746252133));
#36715=CARTESIAN_POINT('Ctrl Pts',(52.6183017873507,20.423403196451,25.5879950587193));
#36716=CARTESIAN_POINT('Ctrl Pts',(52.595621605406,20.5170862492664,25.5829671316396));
#36717=CARTESIAN_POINT('Ctrl Pts',(52.5784416541832,20.6122408387639,25.5779392045599));
#36718=CARTESIAN_POINT('Ctrl Pts',(52.5669285807952,20.7082574438846,25.5729112774802));
#36719=CARTESIAN_POINT('Ctrl Pts',(52.5554155074072,20.8042740490054,25.5678833504004));
#36720=CARTESIAN_POINT('Ctrl Pts',(52.5495695209335,20.9011524863519,25.5628554233207));
#36721=CARTESIAN_POINT('Ctrl Pts',(52.5495006168754,20.9982612343868,25.557827496241));
#36722=CARTESIAN_POINT('',(52.5495006353634,21.0017646290239,24.7578274961833));
#36723=CARTESIAN_POINT('Ctrl Pts',(52.549500616875,20.9982612349457,25.5578274962121));
#36724=CARTESIAN_POINT('Ctrl Pts',(52.5494426726785,21.0799239169191,25.5535993085524));
#36725=CARTESIAN_POINT('Ctrl Pts',(52.5534711553422,21.161620251567,25.5493711208926));
#36726=CARTESIAN_POINT('Ctrl Pts',(52.5615695457031,21.242913913882,25.5451429332329));
#36727=CARTESIAN_POINT('Ctrl Pts',(52.5696676334938,21.3242045389216,25.5409149035457));
#36728=CARTESIAN_POINT('Ctrl Pts',(52.581835280649,21.4050920630522,25.5366868738586));
#36729=CARTESIAN_POINT('Ctrl Pts',(52.5980040885974,21.4851452273341,25.5324588441714));
#36730=CARTESIAN_POINT('Ctrl Pts',(52.6141771330571,21.5652193669495,25.5282297066663));
#36731=CARTESIAN_POINT('Ctrl Pts',(52.6343533283592,21.644458261135,25.5240005691613));
#36732=CARTESIAN_POINT('Ctrl Pts',(52.6584134445613,21.7224421453576,25.5197714316562));
#36733=CARTESIAN_POINT('Ctrl Pts',(52.6825035509126,21.8005232339455,25.5155370226692));
#36734=CARTESIAN_POINT('Ctrl Pts',(52.7104871040229,21.8773457495278,25.5113026136823));
#36735=CARTESIAN_POINT('Ctrl Pts',(52.7421955433444,21.9525068427607,25.5070682046954));
#36736=CARTESIAN_POINT('Ctrl Pts',(52.773926246832,22.0277207105576,25.5028308225068));
#36737=CARTESIAN_POINT('Ctrl Pts',(52.8093868421525,22.1012704194946,25.4985934403183));
#36738=CARTESIAN_POINT('Ctrl Pts',(52.8483624271334,22.1727770483041,25.4943560581297));
#36739=CARTESIAN_POINT('Ctrl Pts',(52.8874072856409,22.2444107699167,25.4901111446005));
#36740=CARTESIAN_POINT('Ctrl Pts',(52.9299793642756,22.3139937704215,25.4858662310712));
#36741=CARTESIAN_POINT('Ctrl Pts',(52.9758202471203,22.3811757954843,25.481621317542));
#36742=CARTESIAN_POINT('Ctrl Pts',(52.9974933438922,22.4129387642616,25.4796143661921));
#36743=CARTESIAN_POINT('Ctrl Pts',(53.0198965302943,22.4441655212112,25.4776074148422));
#36744=CARTESIAN_POINT('Ctrl Pts',(53.0429994982016,22.4748217810844,25.4756004634922));
#36745=CARTESIAN_POINT('Ctrl Pts',(53.0917071719663,22.5394539578134,25.4713692351926));
#36746=CARTESIAN_POINT('Ctrl Pts',(53.1437114313465,22.6017917748592,25.467138006893));
#36747=CARTESIAN_POINT('Ctrl Pts',(53.1987682558081,22.6614795977428,25.4629067785934));
#36748=CARTESIAN_POINT('Ctrl Pts',(53.2537461357293,22.7210818358184,25.4586816173414));
#36749=CARTESIAN_POINT('Ctrl Pts',(53.3117675751297,22.7780412874812,25.4544564560894));
#36750=CARTESIAN_POINT('Ctrl Pts',(53.3725469350141,22.8320335071357,25.4502312948374));
#36751=CARTESIAN_POINT('Ctrl Pts',(53.4334822869078,22.8861642994052,25.4459952895851));
#36752=CARTESIAN_POINT('Ctrl Pts',(53.497189444735,22.9373122361443,25.4417592843329));
#36753=CARTESIAN_POINT('Ctrl Pts',(53.5633417190128,22.9851859443566,25.4375232790806));
#36754=CARTESIAN_POINT('Ctrl Pts',(53.6292059510151,23.0328511993902,25.4333057183733));
#36755=CARTESIAN_POINT('Ctrl Pts',(53.6974936764225,23.0772703990278,25.4290881576659));
#36756=CARTESIAN_POINT('Ctrl Pts',(53.7678490520451,23.1181959993008,25.4248705969585));
#36757=CARTESIAN_POINT('Ctrl Pts',(53.8381812007487,23.1591080885151,25.4206544286244));
#36758=CARTESIAN_POINT('Ctrl Pts',(53.9105792425456,23.1965286352039,25.4164382602902));
#36759=CARTESIAN_POINT('Ctrl Pts',(53.9846599580242,23.2302544359693,25.4122220919561));
#36760=CARTESIAN_POINT('Ctrl Pts',(54.0587389110369,23.2639794343589,25.4080060239294));
#36761=CARTESIAN_POINT('Ctrl Pts',(54.1345000345426,23.294009669972,25.4037899559028));
#36762=CARTESIAN_POINT('Ctrl Pts',(54.211538524869,23.320189378528,25.3995738878762));
#36763=CARTESIAN_POINT('Ctrl Pts',(54.2892072715661,23.3465832648026,25.3953233279517));
#36764=CARTESIAN_POINT('Ctrl Pts',(54.3681739328913,23.369063161065,25.3910727680273));
#36765=CARTESIAN_POINT('Ctrl Pts',(54.4480081858695,23.3875207406707,25.3868222081029));
#36766=CARTESIAN_POINT('Ctrl Pts',(54.5273097442534,23.4058551619514,25.3826000100684));
#36767=CARTESIAN_POINT('Ctrl Pts',(54.6074668784613,23.4202207590966,25.378377812034));
#36768=CARTESIAN_POINT('Ctrl Pts',(54.6880495043284,23.4305631319203,25.3741556139995));
#36769=CARTESIAN_POINT('Ctrl Pts',(54.7694440801131,23.4410097144129,25.3698908731301));
#36770=CARTESIAN_POINT('Ctrl Pts',(54.8512722859611,23.4473515030673,25.3656261322607));
#36771=CARTESIAN_POINT('Ctrl Pts',(54.9330895701137,23.4495863414814,25.3613613913914));
#36772=CARTESIAN_POINT('Ctrl Pts',(55.0149068542662,23.4518211798956,25.357096650522));
#36773=CARTESIAN_POINT('Ctrl Pts',(55.0967127365403,23.449949143322,25.3528319096526));
#36774=CARTESIAN_POINT('Ctrl Pts',(55.1780685790446,23.4440216511228,25.3485671687832));
#36775=CARTESIAN_POINT('Ctrl Pts',(55.2587847438053,23.4381407651011,25.3443359603528));
#36776=CARTESIAN_POINT('Ctrl Pts',(55.3393606068678,23.4282459619067,25.3401047519223));
#36777=CARTESIAN_POINT('Ctrl Pts',(55.4193650420496,23.4143494385666,25.3358735434918));
#36778=CARTESIAN_POINT('Ctrl Pts',(55.4992547525024,23.4004728425577,25.3316484025279));
#36779=CARTESIAN_POINT('Ctrl Pts',(55.5785742082945,23.3826060021575,25.327423261564));
#36780=CARTESIAN_POINT('Ctrl Pts',(55.6568959221464,23.3608129950226,25.3231981206002));
#36781=CARTESIAN_POINT('Ctrl Pts',(55.7354191210712,23.3389639246911,25.3189621103283));
#36782=CARTESIAN_POINT('Ctrl Pts',(55.8129389677181,23.3131685020274,25.3147261000564));
#36783=CARTESIAN_POINT('Ctrl Pts',(55.8890334968853,23.2835432317817,25.3104900897844));
#36784=CARTESIAN_POINT('Ctrl Pts',(55.964796222984,23.2540471397526,25.3062725502386));
#36785=CARTESIAN_POINT('Ctrl Pts',(56.0391455966255,23.2207546919595,25.3020550106928));
#36786=CARTESIAN_POINT('Ctrl Pts',(56.1116806788173,23.183830652396,25.297837471147));
#36787=CARTESIAN_POINT('Ctrl Pts',(56.1841918095111,23.1469188053611,25.2936213242568));
#36788=CARTESIAN_POINT('Ctrl Pts',(56.2548894244571,23.1063779586927,25.2894051773666));
#36789=CARTESIAN_POINT('Ctrl Pts',(56.3233949968083,23.062419921457,25.2851890304764));
#36790=CARTESIAN_POINT('Ctrl Pts',(56.3918989351956,23.0184629326885,25.2809729841479));
#36791=CARTESIAN_POINT('Ctrl Pts',(56.4582105442443,22.9710891674222,25.2767569378193));
#36792=CARTESIAN_POINT('Ctrl Pts',(56.5219794533741,22.9205542932985,25.2725408914908));
#36793=CARTESIAN_POINT('Ctrl Pts',(56.5862707665526,22.8696054302387,25.268290306706));
#36794=CARTESIAN_POINT('Ctrl Pts',(56.6479771410842,22.8154437119307,25.2640397219213));
#36795=CARTESIAN_POINT('Ctrl Pts',(56.7067742173164,22.7583719803,25.2597891371366));
#36796=CARTESIAN_POINT('Ctrl Pts',(56.7651783223078,22.7016816885405,25.2555669612063));
#36797=CARTESIAN_POINT('Ctrl Pts',(56.8207116241952,22.6421205487075,25.251344785276));
#36798=CARTESIAN_POINT('Ctrl Pts',(56.8730952145496,22.5800204325361,25.2471226093456));
#36799=CARTESIAN_POINT('Ctrl Pts',(56.9260074983365,22.5172935566608,25.2428578201337));
#36800=CARTESIAN_POINT('Ctrl Pts',(56.9757058398398,22.4519765519319,25.2385930309218));
#36801=CARTESIAN_POINT('Ctrl Pts',(57.0219473713568,22.3844417927321,25.2343282417099));
#36802=CARTESIAN_POINT('Ctrl Pts',(57.0681889028738,22.3169070335323,25.230063452498));
#36803=CARTESIAN_POINT('Ctrl Pts',(57.1109734272501,22.2471549641736,25.2257986632861));
#36804=CARTESIAN_POINT('Ctrl Pts',(57.1501063028945,22.1755820414814,25.2215338740742));
#36805=CARTESIAN_POINT('Ctrl Pts',(57.1889311980197,22.1045724064476,25.2173026492752));
#36806=CARTESIAN_POINT('Ctrl Pts',(57.2243073473097,22.031504217792,25.2130714244762));
#36807=CARTESIAN_POINT('Ctrl Pts',(57.2560112343045,21.9567463408302,25.2088401996772));
#36808=CARTESIAN_POINT('Ctrl Pts',(57.2876696605508,21.8820956604731,25.2046150421041));
#36809=CARTESIAN_POINT('Ctrl Pts',(57.3156661026306,21.8057605282281,25.200389884531));
#36810=CARTESIAN_POINT('Ctrl Pts',(57.3398226093414,21.728134882295,25.196164726958));
#36811=CARTESIAN_POINT('Ctrl Pts',(57.3640411406536,21.6503099236132,25.1919287208083));
#36812=CARTESIAN_POINT('Ctrl Pts',(57.384399771629,21.5711882329147,25.1876927146586));
#36813=CARTESIAN_POINT('Ctrl Pts',(57.4007675983464,21.4911875290864,25.1834567085089));
#36814=CARTESIAN_POINT('Ctrl Pts',(57.4170641365159,21.4115352608879,25.1792391518903));
#36815=CARTESIAN_POINT('Ctrl Pts',(57.4294044593048,21.3310120772491,25.1750215952716));
#36816=CARTESIAN_POINT('Ctrl Pts',(57.437709610775,21.2500442031628,25.170804038653));
#36817=CARTESIAN_POINT('Ctrl Pts',(57.4460120201169,21.1691030623992,25.1665878745533));
#36818=CARTESIAN_POINT('Ctrl Pts',(57.4502818564995,21.0877179848915,25.1623717104537));
#36819=CARTESIAN_POINT('Ctrl Pts',(57.4504918453088,21.0063218727681,25.158155546354));
#36820=CARTESIAN_POINT('Ctrl Pts',(57.4507018291151,20.9249276998684,25.1539394827025));
#36821=CARTESIAN_POINT('Ctrl Pts',(57.4468521575695,20.8435229577976,25.149723419051));
#36822=CARTESIAN_POINT('Ctrl Pts',(57.4389676745274,20.7625406716709,25.1455073553994));
#36823=CARTESIAN_POINT('Ctrl Pts',(57.4310186709482,20.6808956888822,25.1412567907299));
#36824=CARTESIAN_POINT('Ctrl Pts',(57.41896854609,20.5996805870595,25.1370062260604));
#36825=CARTESIAN_POINT('Ctrl Pts',(57.4028958826981,20.5193321033057,25.1327556613909));
#36826=CARTESIAN_POINT('Ctrl Pts',(57.3869304997749,20.439519922888,25.1285334680347));
#36827=CARTESIAN_POINT('Ctrl Pts',(57.3669962883082,20.3605632669893,25.1243112746786));
#36828=CARTESIAN_POINT('Ctrl Pts',(57.343220869384,20.2828764351359,25.1200890813225));
#36829=CARTESIAN_POINT('Ctrl Pts',(57.3192058096602,20.2044065704133,25.1158243309963));
#36830=CARTESIAN_POINT('Ctrl Pts',(57.2912718383737,20.1272327285547,25.1115595806701));
#36831=CARTESIAN_POINT('Ctrl Pts',(57.2596001429528,20.0517608719486,25.1072948303439));
#36832=CARTESIAN_POINT('Ctrl Pts',(57.2279284475319,19.9762890153425,25.1030300800177));
#36833=CARTESIAN_POINT('Ctrl Pts',(57.1925192943806,19.9025195505309,25.0987653296915));
#36834=CARTESIAN_POINT('Ctrl Pts',(57.1536002527356,19.8308309782511,25.0945005793653));
#36835=CARTESIAN_POINT('Ctrl Pts',(57.1149871920646,19.7597060205477,25.0902693584479));
#36836=CARTESIAN_POINT('Ctrl Pts',(57.0727744823731,19.6903626228375,25.0860381375306));
#36837=CARTESIAN_POINT('Ctrl Pts',(57.0271508610185,19.623188598002,25.0818069166132));
#36838=CARTESIAN_POINT('Ctrl Pts',(56.9815926604765,19.556110895623,25.0775817629457));
#36839=CARTESIAN_POINT('Ctrl Pts',(56.9326335211538,19.4911967693597,25.0733566092782));
#36840=CARTESIAN_POINT('Ctrl Pts',(56.880507954045,19.428809341686,25.0691314556107));
#36841=CARTESIAN_POINT('Ctrl Pts',(56.8282484882493,19.3662616549472,25.0648954484876));
#36842=CARTESIAN_POINT('Ctrl Pts',(56.7728065370341,19.3062540761956,25.0606594413645));
#36843=CARTESIAN_POINT('Ctrl Pts',(56.7144621038584,19.2491230927237,25.0564234342414));
#36844=CARTESIAN_POINT('Ctrl Pts',(56.6563718519762,19.1922410040732,25.0522058815571));
#36845=CARTESIAN_POINT('Ctrl Pts',(56.5954046836663,19.1382108320083,25.0479883288727));
#36846=CARTESIAN_POINT('Ctrl Pts',(56.5318759159369,19.0873300263316,25.0437707761884));
#36847=CARTESIAN_POINT('Ctrl Pts',(56.4683681236747,19.0364660201099,25.039554616025));
#36848=CARTESIAN_POINT('Ctrl Pts',(56.4023007741706,18.9887496057174,25.0353384558616));
#36849=CARTESIAN_POINT('Ctrl Pts',(56.3340228175641,18.9444384289887,25.0311222956982));
#36850=CARTESIAN_POINT('Ctrl Pts',(56.2657464875926,18.9001283079172,25.0269062359794));
#36851=CARTESIAN_POINT('Ctrl Pts',(56.1952600458253,18.8592235153788,25.0226901762606));
#36852=CARTESIAN_POINT('Ctrl Pts',(56.1229408055264,18.8219379721221,25.0184741165418));
#36853=CARTESIAN_POINT('Ctrl Pts',(56.0500296124128,18.7843472364686,25.014223547218));
#36854=CARTESIAN_POINT('Ctrl Pts',(55.9752558973944,18.7504355067548,25.0099729778943));
#36855=CARTESIAN_POINT('Ctrl Pts',(55.8990292335745,18.7203735641166,25.0057224085705));
#36856=CARTESIAN_POINT('Ctrl Pts',(55.8233115136671,18.6905123365818,25.0015002190979));
#36857=CARTESIAN_POINT('Ctrl Pts',(55.7461606523289,18.6644497364852,24.9972780296254));
#36858=CARTESIAN_POINT('Ctrl Pts',(55.6679939570079,18.6423031739851,24.9930558401529));
#36859=CARTESIAN_POINT('Ctrl Pts',(55.5890391542837,18.6199333211208,24.9887910809035));
#36860=CARTESIAN_POINT('Ctrl Pts',(55.5090483916766,18.6015590251151,24.984526321654));
#36861=CARTESIAN_POINT('Ctrl Pts',(55.4284610202324,18.587248167726,24.9802615624046));
#36862=CARTESIAN_POINT('Ctrl Pts',(55.3478736487883,18.572937310337,24.9759968031552));
#36863=CARTESIAN_POINT('Ctrl Pts',(55.2666901545566,18.5626898881577,24.9717320439058));
#36864=CARTESIAN_POINT('Ctrl Pts',(55.1853519635064,18.5565199203545,24.9674672846563));
#36865=CARTESIAN_POINT('Ctrl Pts',(55.104653461615,18.550398476639,24.9632360658658));
#36866=CARTESIAN_POINT('Ctrl Pts',(55.0235000796318,18.5482675811919,24.9590048470753));
#36867=CARTESIAN_POINT('Ctrl Pts',(54.9423200086918,18.5501789313089,24.9547736282848));
#36868=CARTESIAN_POINT('Ctrl Pts',(54.8612563448273,18.552087540671,24.9505484767939));
#36869=CARTESIAN_POINT('Ctrl Pts',(54.7801665288857,18.5580268728122,24.9463233253029));
#36870=CARTESIAN_POINT('Ctrl Pts',(54.6994828257887,18.5679967767283,24.9420981738119));
#36871=CARTESIAN_POINT('Ctrl Pts',(54.6185918127283,18.5779922974708,24.9378621661509));
#36872=CARTESIAN_POINT('Ctrl Pts',(54.5381094732769,18.5920391582366,24.9336261584899));
#36873=CARTESIAN_POINT('Ctrl Pts',(54.458470360457,18.6100845413495,24.9293901508289));
#36874=CARTESIAN_POINT('Ctrl Pts',(54.3791782535467,18.6280512965828,24.9251726004263));
#36875=CARTESIAN_POINT('Ctrl Pts',(54.3007224984419,18.6499817064567,24.9209550500238));
#36876=CARTESIAN_POINT('Ctrl Pts',(54.2235239944632,18.6757721146958,24.9167374996213));
#36877=CARTESIAN_POINT('Ctrl Pts',(54.1463509799739,18.7015540074288,24.9125213417743));
#36878=CARTESIAN_POINT('Ctrl Pts',(54.0704348328585,18.7311932203502,24.9083051839273));
#36879=CARTESIAN_POINT('Ctrl Pts',(53.9961812444017,18.7645362548435,24.9040890260804));
#36880=CARTESIAN_POINT('Ctrl Pts',(53.9219294254996,18.7978784947312,24.8998729687097));
#36881=CARTESIAN_POINT('Ctrl Pts',(53.84934051015,18.8349241892326,24.895656911339));
#36882=CARTESIAN_POINT('Ctrl Pts',(53.778798829418,18.8754722993171,24.8914408539682));
#36883=CARTESIAN_POINT('Ctrl Pts',(53.7076796612686,18.9163523553253,24.8871902819665));
#36884=CARTESIAN_POINT('Ctrl Pts',(53.638641825627,18.960792211328,24.8829397099648));
#36885=CARTESIAN_POINT('Ctrl Pts',(53.572050899435,19.0085403302613,24.878689137963));
#36886=CARTESIAN_POINT('Ctrl Pts',(53.505904661363,19.0559695916197,24.8744669508927));
#36887=CARTESIAN_POINT('Ctrl Pts',(53.4421730807613,19.1066627252754,24.8702447638223));
#36888=CARTESIAN_POINT('Ctrl Pts',(53.3811810828112,19.1603327574391,24.866022576752));
#36889=CARTESIAN_POINT('Ctrl Pts',(53.3195740290917,19.2145440091732,24.8617578122846));
#36890=CARTESIAN_POINT('Ctrl Pts',(53.2607624701863,19.2717921978405,24.8574930478171));
#36891=CARTESIAN_POINT('Ctrl Pts',(53.2050416698394,19.3317449706394,24.8532282833497));
#36892=CARTESIAN_POINT('Ctrl Pts',(53.1493208694925,19.3916977434382,24.8489635188822));
#36893=CARTESIAN_POINT('Ctrl Pts',(53.0966910883909,19.4543546901213,24.8446987544148));
#36894=CARTESIAN_POINT('Ctrl Pts',(53.0474034577743,19.5193525087691,24.8404339899473));
#36895=CARTESIAN_POINT('Ctrl Pts',(52.9983789905267,19.5840032820282,24.8361919965032));
#36896=CARTESIAN_POINT('Ctrl Pts',(52.9524752143873,19.6512149433991,24.831950003059));
#36897=CARTESIAN_POINT('Ctrl Pts',(52.9099697495301,19.7206549323499,24.8277080096149));
#36898=CARTESIAN_POINT('Ctrl Pts',(52.8675250489743,19.7899956523612,24.8234720803738));
#36899=CARTESIAN_POINT('Ctrl Pts',(52.8284692525181,19.8615579854376,24.8192361511326));
#36900=CARTESIAN_POINT('Ctrl Pts',(52.7930388342031,19.9349776233974,24.8150002218915));
#36901=CARTESIAN_POINT('Ctrl Pts',(52.7576484095447,20.0083143856833,24.8107690741434));
#36902=CARTESIAN_POINT('Ctrl Pts',(52.725875434281,20.083503875713,24.8065379263954));
#36903=CARTESIAN_POINT('Ctrl Pts',(52.6979115347011,20.1601554025072,24.8023067786473));
#36904=CARTESIAN_POINT('Ctrl Pts',(52.6699708433048,20.2367433136135,24.7980791424715));
#36905=CARTESIAN_POINT('Ctrl Pts',(52.6458331031965,20.3147904181951,24.7938515062957));
#36906=CARTESIAN_POINT('Ctrl Pts',(52.6256421094426,20.3938854418943,24.7896238701199));
#36907=CARTESIAN_POINT('Ctrl Pts',(52.6054609709417,20.4729418591987,24.7853982974593));
#36908=CARTESIAN_POINT('Ctrl Pts',(52.5892228633599,20.5530447324479,24.7811727247988));
#36909=CARTESIAN_POINT('Ctrl Pts',(52.577021547851,20.6337682831571,24.7769471521383));
#36910=CARTESIAN_POINT('Ctrl Pts',(52.5648200476823,20.7144930555703,24.7727215155262));
#36911=CARTESIAN_POINT('Ctrl Pts',(52.5566555379763,20.7958380691267,24.7684958789141));
#36912=CARTESIAN_POINT('Ctrl Pts',(52.5525703438381,20.8773691387166,24.764270242302));
#36913=CARTESIAN_POINT('Ctrl Pts',(52.5504941384457,20.9188054182667,24.7621226602721));
#36914=CARTESIAN_POINT('Ctrl Pts',(52.5494707688368,20.9602896636726,24.7599750782421));
#36915=CARTESIAN_POINT('Ctrl Pts',(52.549500635363,21.0017646284675,24.7578274962121));
#36916=CARTESIAN_POINT('',(52.5495001212409,21.0007708448949,23.9578274962553));
#36917=CARTESIAN_POINT('Ctrl Pts',(52.5495006353634,21.001764629024,24.7578274961833));
#36918=CARTESIAN_POINT('Ctrl Pts',(52.5495679528408,21.0952468472569,24.7529869680962));
#36919=CARTESIAN_POINT('Ctrl Pts',(52.5549885424231,21.1885143020218,24.7481464400091));
#36920=CARTESIAN_POINT('Ctrl Pts',(52.5656650324199,21.2810044761507,24.743305911922));
#36921=CARTESIAN_POINT('Ctrl Pts',(52.5766584178876,21.3762399080658,24.7383217091414));
#36922=CARTESIAN_POINT('Ctrl Pts',(52.5932244071865,21.4706509753609,24.7333375063608));
#36923=CARTESIAN_POINT('Ctrl Pts',(52.6152033071151,21.5636443768948,24.7283533035802));
#36924=CARTESIAN_POINT('Ctrl Pts',(52.6371822070437,21.6566377784288,24.7233691007996));
#36925=CARTESIAN_POINT('Ctrl Pts',(52.6645738460604,21.7482133664511,24.718384898019));
#36926=CARTESIAN_POINT('Ctrl Pts',(52.6971671152198,21.8378012620991,24.7134006952384));
#36927=CARTESIAN_POINT('Ctrl Pts',(52.7248363953362,21.9138547738718,24.7091694749144));
#36928=CARTESIAN_POINT('Ctrl Pts',(52.7563292240878,21.9886786948271,24.7049382545903));
#36929=CARTESIAN_POINT('Ctrl Pts',(52.7915162961357,22.0618615633714,24.7007070342663));
#36930=CARTESIAN_POINT('Ctrl Pts',(52.8266529124041,22.1349394928442,24.6964818812138));
#36931=CARTESIAN_POINT('Ctrl Pts',(52.8654730514026,22.2063806279751,24.6922567281613));
#36932=CARTESIAN_POINT('Ctrl Pts',(52.9077984858989,22.2757911562607,24.6880315751087));
#36933=CARTESIAN_POINT('Ctrl Pts',(52.9502326524672,22.3453799969641,24.6837955678346));
#36934=CARTESIAN_POINT('Ctrl Pts',(52.9961899800574,22.4129273430252,24.6795595605604));
#36935=CARTESIAN_POINT('Ctrl Pts',(53.0454433098682,22.4780589957985,24.6753235532863));
#36936=CARTESIAN_POINT('Ctrl Pts',(53.0944820549032,22.5429068858058,24.6711060012653));
#36937=CARTESIAN_POINT('Ctrl Pts',(53.1467878666111,22.6053597096896,24.6668884492444));
#36938=CARTESIAN_POINT('Ctrl Pts',(53.2020928875876,22.6650766544327,24.6626708972234));
#36939=CARTESIAN_POINT('Ctrl Pts',(53.2573796481305,22.7247738820275,24.6584547377402));
#36940=CARTESIAN_POINT('Ctrl Pts',(53.3156633357472,22.781736683515,24.6542385782569));
#36941=CARTESIAN_POINT('Ctrl Pts',(53.3766369428855,22.8356586378725,24.6500224187737));
#36942=CARTESIAN_POINT('Ctrl Pts',(53.4376090971747,22.8895793074042,24.645806359751));
#36943=CARTESIAN_POINT('Ctrl Pts',(53.5012706945447,22.9404589667043,24.6415903007283));
#36944=CARTESIAN_POINT('Ctrl Pts',(53.5672802094262,22.9880302441608,24.6373742417057));
#36945=CARTESIAN_POINT('Ctrl Pts',(53.6338300533993,23.0359909222239,24.6331236716076));
#36946=CARTESIAN_POINT('Ctrl Pts',(53.7027660508481,23.0805885126075,24.6288731015096));
#36947=CARTESIAN_POINT('Ctrl Pts',(53.7737083905136,23.1215935375333,24.6246225314116));
#36948=CARTESIAN_POINT('Ctrl Pts',(53.8441770432134,23.1623247690387,24.6204003426675));
#36949=CARTESIAN_POINT('Ctrl Pts',(53.9166248808244,23.1995111052045,24.6161781539234));
#36950=CARTESIAN_POINT('Ctrl Pts',(53.9906565497935,23.2329747086622,24.6119559651793));
#36951=CARTESIAN_POINT('Ctrl Pts',(54.0654346748524,23.2667757232703,24.6076912044043));
#36952=CARTESIAN_POINT('Ctrl Pts',(54.1418282981851,23.2967783329379,24.6034264436293));
#36953=CARTESIAN_POINT('Ctrl Pts',(54.2194129392859,23.3228504236489,24.5991616828543));
#36954=CARTESIAN_POINT('Ctrl Pts',(54.2969975803868,23.3489225143599,24.5948969220793));
#36955=CARTESIAN_POINT('Ctrl Pts',(54.3757727580464,23.3710640175984,24.5906321613043));
#36956=CARTESIAN_POINT('Ctrl Pts',(54.4553039735296,23.3891957828415,24.5863674005293));
#36957=CARTESIAN_POINT('Ctrl Pts',(54.5342097074288,23.4071849489154,24.5821361804126));
#36958=CARTESIAN_POINT('Ctrl Pts',(54.6141555072841,23.421294723698,24.577904960296));
#36959=CARTESIAN_POINT('Ctrl Pts',(54.6947255363877,23.4314106506031,24.5736737401793));
#36960=CARTESIAN_POINT('Ctrl Pts',(54.7751800336395,23.4415120719684,24.5694485873398));
#36961=CARTESIAN_POINT('Ctrl Pts',(54.8562565249924,23.447630962083,24.5652234345002));
#36962=CARTESIAN_POINT('Ctrl Pts',(54.937527476602,23.4497035399861,24.5609982816607));
#36963=CARTESIAN_POINT('Ctrl Pts',(55.0190072146233,23.4517814423759,24.556762274334));
#36964=CARTESIAN_POINT('Ctrl Pts',(55.1006819516917,23.4497921171981,24.5525262670073));
#36965=CARTESIAN_POINT('Ctrl Pts',(55.1821141023636,23.4437235325872,24.5482902596807));
#36966=CARTESIAN_POINT('Ctrl Pts',(55.2631914676302,23.4376813877207,24.5440727078849));
#36967=CARTESIAN_POINT('Ctrl Pts',(55.3440278887176,23.4275954811244,24.5398551560892));
#36968=CARTESIAN_POINT('Ctrl Pts',(55.4241917643742,23.4135060797597,24.5356376042934));
#36969=CARTESIAN_POINT('Ctrl Pts',(55.5043291717013,23.3994213304021,24.5314214450395));
#36970=CARTESIAN_POINT('Ctrl Pts',(55.5837940170331,23.381335791731,24.5272052857856));
#36971=CARTESIAN_POINT('Ctrl Pts',(55.6621623684179,23.359341274138,24.5229891265317));
#36972=CARTESIAN_POINT('Ctrl Pts',(55.7405288524091,23.3373472806395,24.5187730677422));
#36973=CARTESIAN_POINT('Ctrl Pts',(55.8177984470749,23.3114446201112,24.5145570089527));
#36974=CARTESIAN_POINT('Ctrl Pts',(55.8935613147325,23.2817752796482,24.5103409501632));
#36975=CARTESIAN_POINT('Ctrl Pts',(55.9699443577297,23.2518630735985,24.5060903798013));
#36976=CARTESIAN_POINT('Ctrl Pts',(56.0447954399595,23.2181223968107,24.5018398094394));
#36977=CARTESIAN_POINT('Ctrl Pts',(56.1177158039986,23.1807479523071,24.4975892390775));
#36978=CARTESIAN_POINT('Ctrl Pts',(56.1901492650474,23.1436230640013,24.4933670505736));
#36979=CARTESIAN_POINT('Ctrl Pts',(56.2606773371968,23.1029130751492,24.4891448620697));
#36980=CARTESIAN_POINT('Ctrl Pts',(56.328936225891,23.0588537484519,24.4849226735659));
#36981=CARTESIAN_POINT('Ctrl Pts',(56.3978833764026,23.0143501667596,24.480657912275));
#36982=CARTESIAN_POINT('Ctrl Pts',(56.464514930647,22.9664296072111,24.476393150984));
#36983=CARTESIAN_POINT('Ctrl Pts',(56.5284897189965,22.91537709836,24.4721283896931));
#36984=CARTESIAN_POINT('Ctrl Pts',(56.592464507346,22.8643245895089,24.4678636284022));
#36985=CARTESIAN_POINT('Ctrl Pts',(56.6537822113085,22.810140498534,24.4635988671113));
#36986=CARTESIAN_POINT('Ctrl Pts',(56.712140730981,22.7531469896491,24.4593341058204));
#36987=CARTESIAN_POINT('Ctrl Pts',(56.7700402808879,22.6966017151877,24.4551028854161));
#36988=CARTESIAN_POINT('Ctrl Pts',(56.825244174904,22.6370790495558,24.4508716650117));
#36989=CARTESIAN_POINT('Ctrl Pts',(56.8774307668126,22.5748663326852,24.4466404446074));
#36990=CARTESIAN_POINT('Ctrl Pts',(56.9295425268185,22.5127428244755,24.4424152914756));
#36991=CARTESIAN_POINT('Ctrl Pts',(56.9786452813961,22.4479372791931,24.4381901383438));
#36992=CARTESIAN_POINT('Ctrl Pts',(57.0244536213447,22.3807743425427,24.433964985212));
#36993=CARTESIAN_POINT('Ctrl Pts',(57.0703796397092,22.3134388690136,24.4297289779578));
#36994=CARTESIAN_POINT('Ctrl Pts',(57.112993962336,22.2437342110515,24.4254929707036));
#36995=CARTESIAN_POINT('Ctrl Pts',(57.1520492113159,22.1720215194588,24.4212569634494));
#36996=CARTESIAN_POINT('Ctrl Pts',(57.1909343069628,22.1006212609913,24.4170394113523));
#36997=CARTESIAN_POINT('Ctrl Pts',(57.2262910452087,22.0272308363188,24.4128218592551));
#36998=CARTESIAN_POINT('Ctrl Pts',(57.2579192361645,21.952234725768,24.4086043071579));
#36999=CARTESIAN_POINT('Ctrl Pts',(57.2895369842162,21.8772633772145,24.4043881475999));
#37000=CARTESIAN_POINT('Ctrl Pts',(57.3174284492104,21.8006878236554,24.4001719880418));
#37001=CARTESIAN_POINT('Ctrl Pts',(57.341440908335,21.7229140493692,24.3959558284837));
#37002=CARTESIAN_POINT('Ctrl Pts',(57.3654527952943,21.6451421282649,24.3917397693876));
#37003=CARTESIAN_POINT('Ctrl Pts',(57.3855857240596,21.5661724877579,24.3875237102915));
#37004=CARTESIAN_POINT('Ctrl Pts',(57.4017367742816,21.486426476524,24.3833076511955));
#37005=CARTESIAN_POINT('Ctrl Pts',(57.4180200303012,21.4060276975208,24.3790570811885));
#37006=CARTESIAN_POINT('Ctrl Pts',(57.4302558079205,21.3248402460121,24.3748065111815));
#37007=CARTESIAN_POINT('Ctrl Pts',(57.4383914885568,21.2433047441661,24.3705559411745));
#37008=CARTESIAN_POINT('Ctrl Pts',(57.4464728469894,21.1623136575121,24.3663337523614));
#37009=CARTESIAN_POINT('Ctrl Pts',(57.4505087331316,21.0809796262463,24.3621115635482));
#37010=CARTESIAN_POINT('Ctrl Pts',(57.4504999857964,20.9997361591577,24.3578893747351));
#37011=CARTESIAN_POINT('Ctrl Pts',(57.4504911502629,20.9176735245613,24.3536246141312));
#37012=CARTESIAN_POINT('Ctrl Pts',(57.4463556836074,20.8357037758953,24.3493598535272));
#37013=CARTESIAN_POINT('Ctrl Pts',(57.4381480872401,20.754268124397,24.3450950929233));
#37014=CARTESIAN_POINT('Ctrl Pts',(57.4299404908729,20.6728324728988,24.3408303323193));
#37015=CARTESIAN_POINT('Ctrl Pts',(57.417660900617,20.5919313852684,24.3365655717154));
#37016=CARTESIAN_POINT('Ctrl Pts',(57.4014162049876,20.511993380759,24.3323008111114));
#37017=CARTESIAN_POINT('Ctrl Pts',(57.3852992661294,20.4326840504696,24.3280695908124));
#37018=CARTESIAN_POINT('Ctrl Pts',(57.3652189746059,20.3540252989922,24.3238383705134));
#37019=CARTESIAN_POINT('Ctrl Pts',(57.3412423599677,20.2764431868243,24.3196071502143));
#37020=CARTESIAN_POINT('Ctrl Pts',(57.3173001261158,20.1989723219722,24.3153819971889));
#37021=CARTESIAN_POINT('Ctrl Pts',(57.2894728015774,20.1225754707219,24.3111568441635));
#37022=CARTESIAN_POINT('Ctrl Pts',(57.2578784100349,20.0476684739556,24.306931691138));
#37023=CARTESIAN_POINT('Ctrl Pts',(57.2262028537188,19.9725690440028,24.3026956838574));
#37024=CARTESIAN_POINT('Ctrl Pts',(57.1907409510164,19.8989675943689,24.2984596765767));
#37025=CARTESIAN_POINT('Ctrl Pts',(57.1516620198987,19.827267804601,24.2942236692961));
#37026=CARTESIAN_POINT('Ctrl Pts',(57.1127533465325,19.7558803940265,24.2900061173072));
#37027=CARTESIAN_POINT('Ctrl Pts',(57.070259312843,19.6863785224298,24.2857885653183));
#37028=CARTESIAN_POINT('Ctrl Pts',(57.024394425453,19.6191388700544,24.2815710133293));
#37029=CARTESIAN_POINT('Ctrl Pts',(56.9785446816035,19.5519214186795,24.27735485388));
#37030=CARTESIAN_POINT('Ctrl Pts',(56.9293265560521,19.4869650869988,24.2731386944306));
#37031=CARTESIAN_POINT('Ctrl Pts',(56.8769983614893,19.4246183316521,24.2689225349812));
#37032=CARTESIAN_POINT('Ctrl Pts',(56.8246714137989,19.3622730618994,24.2647064759942));
#37033=CARTESIAN_POINT('Ctrl Pts',(56.7692348441787,19.3025376002505,24.2604904170071));
#37034=CARTESIAN_POINT('Ctrl Pts',(56.7109868790124,19.2457268884671,24.2562743580201));
#37035=CARTESIAN_POINT('Ctrl Pts',(56.6522621168805,19.1884511445591,24.2520237878853));
#37036=CARTESIAN_POINT('Ctrl Pts',(56.5906800528197,19.1341485998738,24.2477732177505));
#37037=CARTESIAN_POINT('Ctrl Pts',(56.5265823822585,19.0831023814042,24.2435226476157));
#37038=CARTESIAN_POINT('Ctrl Pts',(56.4629126974768,19.0323970030216,24.2393004589112));
#37039=CARTESIAN_POINT('Ctrl Pts',(56.3967613151867,18.9849048213301,24.2350782702068));
#37040=CARTESIAN_POINT('Ctrl Pts',(56.3284929396148,18.9408601894496,24.2308560815023));
#37041=CARTESIAN_POINT('Ctrl Pts',(56.2595362169737,18.8963714574566,24.2265913206523));
#37042=CARTESIAN_POINT('Ctrl Pts',(56.1884199905976,18.8554004320855,24.2223265598024));
#37043=CARTESIAN_POINT('Ctrl Pts',(56.1155445337149,18.8181405537251,24.2180617989524));
#37044=CARTESIAN_POINT('Ctrl Pts',(56.0426690768322,18.7808806753648,24.2137970381024));
#37045=CARTESIAN_POINT('Ctrl Pts',(55.9680348552272,18.7473320829471,24.2095322772524));
#37046=CARTESIAN_POINT('Ctrl Pts',(55.8920598833107,18.7176373174739,24.2052675164025));
#37047=CARTESIAN_POINT('Ctrl Pts',(55.8166824229039,18.688176088963,24.2010362961202));
#37048=CARTESIAN_POINT('Ctrl Pts',(55.7397025854611,18.6623977675449,24.196805075838));
#37049=CARTESIAN_POINT('Ctrl Pts',(55.6615147069631,18.6404770519295,24.1925738555558));
#37050=CARTESIAN_POINT('Ctrl Pts',(55.583438944419,18.6185877690884,24.1883487025478));
#37051=CARTESIAN_POINT('Ctrl Pts',(55.5041590250756,18.6005452304495,24.1841235495398));
#37052=CARTESIAN_POINT('Ctrl Pts',(55.4240883481641,18.5864757463511,24.1798983965318));
#37053=CARTESIAN_POINT('Ctrl Pts',(55.3438119723586,18.5723701182181,24.1756623892469));
#37054=CARTESIAN_POINT('Ctrl Pts',(55.2627412128886,18.5622581498905,24.1714263819619));
#37055=CARTESIAN_POINT('Ctrl Pts',(55.1813070634924,18.556216458291,24.167190374677));
#37056=CARTESIAN_POINT('Ctrl Pts',(55.1002277040579,18.5502010889598,24.1629728227069));
#37057=CARTESIAN_POINT('Ctrl Pts',(55.0187885804917,18.5482206465637,24.1587552707367));
#37058=CARTESIAN_POINT('Ctrl Pts',(54.93742250303,18.5502991393084,24.1545377187666));
#37059=CARTESIAN_POINT('Ctrl Pts',(54.8560832908016,18.5523769457821,24.1503215593365));
#37060=CARTESIAN_POINT('Ctrl Pts',(54.7748175411876,18.5585110141472,24.1461053999063));
#37061=CARTESIAN_POINT('Ctrl Pts',(54.6940581025609,18.5686732417482,24.1418892404762));
#37062=CARTESIAN_POINT('Ctrl Pts',(54.6133005882727,18.5788352272032,24.1376731815088));
#37063=CARTESIAN_POINT('Ctrl Pts',(54.5330498221303,18.5930251219099,24.1334571225415));
#37064=CARTESIAN_POINT('Ctrl Pts',(54.4537321341972,18.6111631138164,24.1292410635741));
#37065=CARTESIAN_POINT('Ctrl Pts',(54.3737651793135,18.6294495770035,24.1249904934174));
#37066=CARTESIAN_POINT('Ctrl Pts',(54.294747120078,18.6517489799349,24.1207399232607));
#37067=CARTESIAN_POINT('Ctrl Pts',(54.2171011245379,18.6779277356637,24.116489353104));
#37068=CARTESIAN_POINT('Ctrl Pts',(54.139973578908,18.7039316932787,24.1122671644201));
#37069=CARTESIAN_POINT('Ctrl Pts',(54.0642002441902,18.7337631263087,24.1080449757363));
#37070=CARTESIAN_POINT('Ctrl Pts',(53.9901757827592,18.7672426687448,24.1038227870524));
#37071=CARTESIAN_POINT('Ctrl Pts',(53.9154049347732,18.8010597844621,24.0995580261592));
#37072=CARTESIAN_POINT('Ctrl Pts',(53.8424188582653,18.8385987690382,24.0952932652661));
#37073=CARTESIAN_POINT('Ctrl Pts',(53.7715971255929,18.8796281863436,24.0910285043729));
#37074=CARTESIAN_POINT('Ctrl Pts',(53.7007753929206,18.920657603649,24.0867637434798));
#37075=CARTESIAN_POINT('Ctrl Pts',(53.6321183733777,18.9651771376472,24.0824989825866));
#37076=CARTESIAN_POINT('Ctrl Pts',(53.5659724915114,19.0129128466778,24.0782342216934));
#37077=CARTESIAN_POINT('Ctrl Pts',(53.5008642707206,19.0598997035385,24.0740363640791));
#37078=CARTESIAN_POINT('Ctrl Pts',(53.4379362932099,19.1101850001007,24.0698385064647));
#37079=CARTESIAN_POINT('Ctrl Pts',(53.3775460234526,19.1635378185256,24.0656406488503));
#37080=CARTESIAN_POINT('Ctrl Pts',(53.3172425789925,19.2168139296543,24.0614488266492));
#37081=CARTESIAN_POINT('Ctrl Pts',(53.2594699503941,19.2731484967592,24.0572570044481));
#37082=CARTESIAN_POINT('Ctrl Pts',(53.2045555862405,19.3322681249374,24.053065182247));
#37083=CARTESIAN_POINT('Ctrl Pts',(53.1497042104883,19.3913199411519,24.04887816819));
#37084=CARTESIAN_POINT('Ctrl Pts',(53.0977049060763,19.453150127131,24.044691154133));
#37085=CARTESIAN_POINT('Ctrl Pts',(53.0488498620535,19.5174470029064,24.0405041400761));
#37086=CARTESIAN_POINT('Ctrl Pts',(53.0000249526541,19.5817042192734,24.0363197086407));
#37087=CARTESIAN_POINT('Ctrl Pts',(52.9543407407577,19.6484247306994,24.0321352772054));
#37088=CARTESIAN_POINT('Ctrl Pts',(52.912049694455,19.7172631713503,24.02795084577));
#37089=CARTESIAN_POINT('Ctrl Pts',(52.8697712616863,19.7860810805625,24.0237676623641));
#37090=CARTESIAN_POINT('Ctrl Pts',(52.8308842326171,19.8570152619749,24.0195844789581));
#37091=CARTESIAN_POINT('Ctrl Pts',(52.7955973479013,19.9296920081489,24.0154012955521));
#37092=CARTESIAN_POINT('Ctrl Pts',(52.7603097468149,20.0023702297574,24.011218027222));
#37093=CARTESIAN_POINT('Ctrl Pts',(52.7286226398433,20.0767906598515,24.0070347588918));
#37094=CARTESIAN_POINT('Ctrl Pts',(52.7006977712595,20.1525570751319,24.0028514905617));
#37095=CARTESIAN_POINT('Ctrl Pts',(52.6727459280927,20.2283966784902,23.9986641813202));
#37096=CARTESIAN_POINT('Ctrl Pts',(52.6485637418823,20.3055844177771,23.9944768720787));
#37097=CARTESIAN_POINT('Ctrl Pts',(52.6282636822496,20.3837069779204,23.9902895628372));
#37098=CARTESIAN_POINT('Ctrl Pts',(52.6079529533278,20.4618705976567,23.986100052833));
#37099=CARTESIAN_POINT('Ctrl Pts',(52.591528507675,20.5409695528187,23.9819105428288));
#37100=CARTESIAN_POINT('Ctrl Pts',(52.5790515600889,20.6205808369471,23.9777210328247));
#37101=CARTESIAN_POINT('Ctrl Pts',(52.5665542265355,20.7003221972033,23.9735246776195));
#37102=CARTESIAN_POINT('Ctrl Pts',(52.5580173158697,20.7805770872105,23.9693283224144));
#37103=CARTESIAN_POINT('Ctrl Pts',(52.5534500674818,20.8609184494799,23.9651319672093));
#37104=CARTESIAN_POINT('Ctrl Pts',(52.5508000429122,20.9075343910461,23.962697143558));
#37105=CARTESIAN_POINT('Ctrl Pts',(52.5494854651526,20.9541794450299,23.9602623199067));
#37106=CARTESIAN_POINT('Ctrl Pts',(52.5495001212409,21.0007708448949,23.9578274962553));
#37107=CARTESIAN_POINT('',(52.5495010260079,20.9977575763378,23.1578275052968));
#37108=CARTESIAN_POINT('Ctrl Pts',(52.5495001212412,21.0007708457221,23.9578274962121));
#37109=CARTESIAN_POINT('Ctrl Pts',(52.5495134171649,21.0430382650271,23.9556186398029));
#37110=CARTESIAN_POINT('Ctrl Pts',(52.5506202182564,21.0852870907162,23.9534097833937));
#37111=CARTESIAN_POINT('Ctrl Pts',(52.5528180575916,21.1274785893789,23.9512009269845));
#37112=CARTESIAN_POINT('Ctrl Pts',(52.5570281739119,21.2082993819897,23.9469697066815));
#37113=CARTESIAN_POINT('Ctrl Pts',(52.5652542756311,21.2890629167757,23.9427384863785));
#37114=CARTESIAN_POINT('Ctrl Pts',(52.5774930832419,21.3693379052562,23.9385072660755));
#37115=CARTESIAN_POINT('Ctrl Pts',(52.5897143412591,21.4494977850218,23.9342821130463));
#37116=CARTESIAN_POINT('Ctrl Pts',(52.6059368079309,21.5291700540761,23.930056960017));
#37117=CARTESIAN_POINT('Ctrl Pts',(52.6261052589627,21.6079259893073,23.9258318069878));
#37118=CARTESIAN_POINT('Ctrl Pts',(52.6463255219447,21.6868842454103,23.9215957997081));
#37119=CARTESIAN_POINT('Ctrl Pts',(52.6705120384248,21.7649209825741,23.9173597924284));
#37120=CARTESIAN_POINT('Ctrl Pts',(52.6985570552922,21.8416119190308,23.9131237851488));
#37121=CARTESIAN_POINT('Ctrl Pts',(52.7264798866173,21.9179687311151,23.9089062331565));
#37122=CARTESIAN_POINT('Ctrl Pts',(52.75822751428,21.99299100249,23.9046886811642));
#37123=CARTESIAN_POINT('Ctrl Pts',(52.7936435003593,22.0662744705249,23.900471129172));
#37124=CARTESIAN_POINT('Ctrl Pts',(52.8290477928857,22.139533742026,23.8962549697194));
#37125=CARTESIAN_POINT('Ctrl Pts',(52.8681178363983,22.2110549320226,23.8920388102668));
#37126=CARTESIAN_POINT('Ctrl Pts',(52.9106496944755,22.2804552123385,23.8878226508143));
#37127=CARTESIAN_POINT('Ctrl Pts',(52.953180539105,22.3498538389867,23.8836065918242));
#37128=CARTESIAN_POINT('Ctrl Pts',(52.9991727904118,22.4171312606115,23.8793905328341));
#37129=CARTESIAN_POINT('Ctrl Pts',(53.0483780804816,22.4819318922459,23.8751744738441));
#37130=CARTESIAN_POINT('Ctrl Pts',(53.097986147337,22.5472629585158,23.8709239037134));
#37131=CARTESIAN_POINT('Ctrl Pts',(53.1508598199829,22.610076107651,23.8666733335826));
#37132=CARTESIAN_POINT('Ctrl Pts',(53.206703034202,22.6700407906574,23.8624227634519));
#37133=CARTESIAN_POINT('Ctrl Pts',(53.2621733784582,22.729605084298,23.858200574745));
#37134=CARTESIAN_POINT('Ctrl Pts',(53.3205733494969,22.7863585519973,23.853978386038));
#37135=CARTESIAN_POINT('Ctrl Pts',(53.3815769138414,22.8400154793341,23.849756197331));
#37136=CARTESIAN_POINT('Ctrl Pts',(53.4431955743353,22.8942134270152,23.8454914364884));
#37137=CARTESIAN_POINT('Ctrl Pts',(53.5074702470363,22.9452517362166,23.8412266756458));
#37138=CARTESIAN_POINT('Ctrl Pts',(53.5740336697725,22.9928798947898,23.8369619148032));
#37139=CARTESIAN_POINT('Ctrl Pts',(53.6405970925086,23.040508053363,23.8326971539606));
#37140=CARTESIAN_POINT('Ctrl Pts',(53.7094488251654,23.0847258550163,23.828432393118));
#37141=CARTESIAN_POINT('Ctrl Pts',(53.780196531644,23.1253305033775,23.8241676322754));
#37142=CARTESIAN_POINT('Ctrl Pts',(53.8503878373329,23.1656158133524,23.8199364119731));
#37143=CARTESIAN_POINT('Ctrl Pts',(53.9227085879526,23.2024957039034,23.8157051916708));
#37144=CARTESIAN_POINT('Ctrl Pts',(53.9967946214461,23.2357390765562,23.8114739713685));
#37145=CARTESIAN_POINT('Ctrl Pts',(54.0707744207519,23.268934780539,23.8072488183401));
#37146=CARTESIAN_POINT('Ctrl Pts',(54.1465140549981,23.2985041343083,23.8030236653116));
#37147=CARTESIAN_POINT('Ctrl Pts',(54.2236233520432,23.3242610762364,23.7987985122832));
#37148=CARTESIAN_POINT('Ctrl Pts',(54.3009307398298,23.3500841867319,23.7945625050033));
#37149=CARTESIAN_POINT('Ctrl Pts',(54.3796144240673,23.3720750430543,23.7903264977234));
#37150=CARTESIAN_POINT('Ctrl Pts',(54.4592594821174,23.3900941283389,23.7860904904436));
#37151=CARTESIAN_POINT('Ctrl Pts',(54.5385575453611,23.4080347087023,23.7818729384522));
#37152=CARTESIAN_POINT('Ctrl Pts',(54.6188081683935,23.4220379427811,23.7776553864609));
#37153=CARTESIAN_POINT('Ctrl Pts',(54.699586851396,23.4320160752236,23.7734378344695));
#37154=CARTESIAN_POINT('Ctrl Pts',(54.7803388631143,23.4419909131136,23.7692216750179));
#37155=CARTESIAN_POINT('Ctrl Pts',(54.8616181275089,23.4479432316177,23.7650055155664));
#37156=CARTESIAN_POINT('Ctrl Pts',(54.942992400024,23.4498368075333,23.7607893561148));
#37157=CARTESIAN_POINT('Ctrl Pts',(55.0243647335545,23.4517303383288,23.7565732971258));
#37158=CARTESIAN_POINT('Ctrl Pts',(55.1058316058827,23.4495653091161,23.7523572381367));
#37159=CARTESIAN_POINT('Ctrl Pts',(55.1869595714351,23.4433576014675,23.7481411791477));
#37160=CARTESIAN_POINT('Ctrl Pts',(55.2687516213392,23.4370990797563,23.7438906090159));
#37161=CARTESIAN_POINT('Ctrl Pts',(55.350198710976,23.4267314108936,23.7396400388842));
#37162=CARTESIAN_POINT('Ctrl Pts',(55.4308625689044,23.412324127624,23.7353894687524));
#37163=CARTESIAN_POINT('Ctrl Pts',(55.5109878272474,23.3980130430362,23.7311672800466));
#37164=CARTESIAN_POINT('Ctrl Pts',(55.5903398378285,23.3797162911962,23.7269450913408));
#37165=CARTESIAN_POINT('Ctrl Pts',(55.6685017508143,23.3575528963648,23.7227229026349));
#37166=CARTESIAN_POINT('Ctrl Pts',(55.7474517668551,23.3351660290197,23.7184581417902));
#37167=CARTESIAN_POINT('Ctrl Pts',(55.8251870907016,23.308834261285,23.7141933809455));
#37168=CARTESIAN_POINT('Ctrl Pts',(55.9012980956155,23.2787303466711,23.7099286201007));
#37169=CARTESIAN_POINT('Ctrl Pts',(55.9774091005293,23.2486264320573,23.705663859256));
#37170=CARTESIAN_POINT('Ctrl Pts',(56.051895374537,23.2147506285081,23.7013990984112));
#37171=CARTESIAN_POINT('Ctrl Pts',(56.1243737877523,23.1773226300701,23.6971343375665));
#37172=CARTESIAN_POINT('Ctrl Pts',(56.1962821889435,23.1401889869885,23.6929031172596));
#37173=CARTESIAN_POINT('Ctrl Pts',(56.2664838678145,23.0994196161714,23.6886718969527));
#37174=CARTESIAN_POINT('Ctrl Pts',(56.3345871906329,23.055195192822,23.6844406766458));
#37175=CARTESIAN_POINT('Ctrl Pts',(56.4025928580535,23.0110341842,23.6802155236126));
#37176=CARTESIAN_POINT('Ctrl Pts',(56.4685057586814,22.963428213733,23.6759903705795));
#37177=CARTESIAN_POINT('Ctrl Pts',(56.5319579971,22.9126042311783,23.6717652175463));
#37178=CARTESIAN_POINT('Ctrl Pts',(56.5955732417271,22.8616496838887,23.6675292102676));
#37179=CARTESIAN_POINT('Ctrl Pts',(56.6567147488336,22.807460791746,23.6632932029889));
#37180=CARTESIAN_POINT('Ctrl Pts',(56.7150403113011,22.7503105383366,23.6590571957102));
#37181=CARTESIAN_POINT('Ctrl Pts',(56.7731117630788,22.6934092750733,23.654839643714));
#37182=CARTESIAN_POINT('Ctrl Pts',(56.8283914159485,22.6335727222424,23.6506220917178));
#37183=CARTESIAN_POINT('Ctrl Pts',(56.8805753616882,22.5711099767398,23.6464045397216));
#37184=CARTESIAN_POINT('Ctrl Pts',(56.9327420774763,22.5086678550145,23.6421883802651));
#37185=CARTESIAN_POINT('Ctrl Pts',(56.9818148181,22.4436016190868,23.6379722208086));
#37186=CARTESIAN_POINT('Ctrl Pts',(57.0275287751062,22.3762548151111,23.6337560613521));
#37187=CARTESIAN_POINT('Ctrl Pts',(57.0732416428415,22.308909615873,23.6295400023581));
#37188=CARTESIAN_POINT('Ctrl Pts',(57.1155956258926,22.2392843419275,23.6253239433641));
#37189=CARTESIAN_POINT('Ctrl Pts',(57.154369044863,22.1677518009133,23.6211078843701));
#37190=CARTESIAN_POINT('Ctrl Pts',(57.1934598489991,22.0956337204241,23.6168573142441));
#37191=CARTESIAN_POINT('Ctrl Pts',(57.2289109573716,22.0215774184445,23.612606744118));
#37192=CARTESIAN_POINT('Ctrl Pts',(57.2605431535074,21.9459888483121,23.608356173992));
#37193=CARTESIAN_POINT('Ctrl Pts',(57.2919641388019,21.870904989437,23.6041339852811));
#37194=CARTESIAN_POINT('Ctrl Pts',(57.3196169536619,21.7943097248618,23.5999117965703));
#37195=CARTESIAN_POINT('Ctrl Pts',(57.3433755813988,21.7166178441149,23.5956896078594));
#37196=CARTESIAN_POINT('Ctrl Pts',(57.3673737662201,21.6381425999246,23.5914248470258));
#37197=CARTESIAN_POINT('Ctrl Pts',(57.3873986735856,21.5585489719529,23.5871600861921));
#37198=CARTESIAN_POINT('Ctrl Pts',(57.4033733485433,21.4782748137963,23.5828953253585));
#37199=CARTESIAN_POINT('Ctrl Pts',(57.419348023501,21.3980006556397,23.5786305645248));
#37200=CARTESIAN_POINT('Ctrl Pts',(57.4312724594035,21.3170464533155,23.5743658036912));
#37201=CARTESIAN_POINT('Ctrl Pts',(57.4391235095687,21.2358532490114,23.5701010428575));
#37202=CARTESIAN_POINT('Ctrl Pts',(57.4469128145653,21.1552985947081,23.565869822553));
#37203=CARTESIAN_POINT('Ctrl Pts',(57.4507218304109,21.0742066178951,23.5616386022485));
#37204=CARTESIAN_POINT('Ctrl Pts',(57.4504900144397,20.9930043491268,23.557407381944));
#37205=CARTESIAN_POINT('Ctrl Pts',(57.4502585308765,20.9119185187286,23.5531822289132));
#37206=CARTESIAN_POINT('Ctrl Pts',(57.4459977246676,20.8307231714723,23.5489570758825));
#37207=CARTESIAN_POINT('Ctrl Pts',(57.437698806098,20.7498504832138,23.5447319228517));
#37208=CARTESIAN_POINT('Ctrl Pts',(57.4293785679397,20.6687700362652,23.5404959155724));
#37209=CARTESIAN_POINT('Ctrl Pts',(57.4169994043282,20.5880143786716,23.5362599082931));
#37210=CARTESIAN_POINT('Ctrl Pts',(57.4006051335561,20.508019062621,23.5320239010138));
#37211=CARTESIAN_POINT('Ctrl Pts',(57.3842822887586,20.4283722673126,23.5278063490201));
#37212=CARTESIAN_POINT('Ctrl Pts',(57.3639793355127,20.3494796620933,23.5235887970264));
#37213=CARTESIAN_POINT('Ctrl Pts',(57.3397912022887,20.2717642004871,23.5193712450326));
#37214=CARTESIAN_POINT('Ctrl Pts',(57.3156110554361,20.1940743987583,23.5151550855786));
#37215=CARTESIAN_POINT('Ctrl Pts',(57.2875484141183,20.1175614123755,23.5109389261246));
#37216=CARTESIAN_POINT('Ctrl Pts',(57.2557483530398,20.042634020994,23.5067227666705));
#37217=CARTESIAN_POINT('Ctrl Pts',(57.2239490496924,19.9677084149805,23.5025067076791));
#37218=CARTESIAN_POINT('Ctrl Pts',(57.188412686306,19.8943687563882,23.4982906486876));
#37219=CARTESIAN_POINT('Ctrl Pts',(57.1493323096355,19.8230034525297,23.4940745896961));
#37220=CARTESIAN_POINT('Ctrl Pts',(57.1099320351043,19.751053978047,23.4898240195671));
#37221=CARTESIAN_POINT('Ctrl Pts',(57.0669296757901,19.6811117586712,23.4855734494382));
#37222=CARTESIAN_POINT('Ctrl Pts',(57.0205691529617,19.6135474951879,23.4813228793092));
#37223=CARTESIAN_POINT('Ctrl Pts',(56.9745181833128,19.5464343640756,23.4771006906009));
#37224=CARTESIAN_POINT('Ctrl Pts',(56.9251540928421,19.4816678658699,23.4728785018925));
#37225=CARTESIAN_POINT('Ctrl Pts',(56.8727570733825,19.4195787921899,23.4686563131842));
#37226=CARTESIAN_POINT('Ctrl Pts',(56.8198317372307,19.3568636772891,23.4643915523449));
#37227=CARTESIAN_POINT('Ctrl Pts',(56.7638122976572,19.2968806385461,23.4601267915056));
#37228=CARTESIAN_POINT('Ctrl Pts',(56.7050249280874,19.2399317500163,23.4558620306664));
#37229=CARTESIAN_POINT('Ctrl Pts',(56.6462375585176,19.1829828614865,23.4515972698271));
#37230=CARTESIAN_POINT('Ctrl Pts',(56.5846826637161,19.1290683922845,23.4473325089878));
#37231=CARTESIAN_POINT('Ctrl Pts',(56.5207182722946,19.0784469337775,23.4430677481486));
#37232=CARTESIAN_POINT('Ctrl Pts',(56.457256933674,19.0282235915648,23.4388365278439));
#37233=CARTESIAN_POINT('Ctrl Pts',(56.3911859179795,18.9810532810875,23.4346053075393));
#37234=CARTESIAN_POINT('Ctrl Pts',(56.3228312038322,18.9372184177262,23.4303740872346));
#37235=CARTESIAN_POINT('Ctrl Pts',(56.2545745055609,18.8934464104911,23.4261489342038));
#37236=CARTESIAN_POINT('Ctrl Pts',(56.1840410006248,18.8530006002341,23.4219237811729));
#37237=CARTESIAN_POINT('Ctrl Pts',(56.1115890524893,18.8161227075713,23.417698628142));
#37238=CARTESIAN_POINT('Ctrl Pts',(56.0389509782095,18.7791500770836,23.4134626208628));
#37239=CARTESIAN_POINT('Ctrl Pts',(55.9643849654187,18.7457640072126,23.4092266135835));
#37240=CARTESIAN_POINT('Ctrl Pts',(55.8882807397064,18.7161638461863,23.4049906063042));
#37241=CARTESIAN_POINT('Ctrl Pts',(55.8125080821701,18.6866926460857,23.4007730543104));
#37242=CARTESIAN_POINT('Ctrl Pts',(55.7352110201091,18.6609746122216,23.3965555023165));
#37243=CARTESIAN_POINT('Ctrl Pts',(55.6567964063242,18.6391593169721,23.3923379503227));
#37244=CARTESIAN_POINT('Ctrl Pts',(55.578407683261,18.6173512246369,23.3881217908686));
#37245=CARTESIAN_POINT('Ctrl Pts',(55.4989025887961,18.5994434364596,23.3839056314144));
#37246=CARTESIAN_POINT('Ctrl Pts',(55.4187032567279,18.585535704798,23.3796894719603));
#37247=CARTESIAN_POINT('Ctrl Pts',(55.3385058356473,18.5716283045294,23.3754734129687));
#37248=CARTESIAN_POINT('Ctrl Pts',(55.2576146681281,18.5617208496152,23.3712573539772));
#37249=CARTESIAN_POINT('Ctrl Pts',(55.1764607818987,18.5558617382702,23.3670412949856));
#37250=CARTESIAN_POINT('Ctrl Pts',(55.0946425992463,18.5499546663543,23.3627907248567));
#37251=CARTESIAN_POINT('Ctrl Pts',(55.0125578543063,18.5481625710354,23.3585401547279));
#37252=CARTESIAN_POINT('Ctrl Pts',(54.9306502824293,18.5504815030964,23.3542895845991));
#37253=CARTESIAN_POINT('Ctrl Pts',(54.8492896144173,18.5527849514497,23.3500673958906));
#37254=CARTESIAN_POINT('Ctrl Pts',(54.7681042239192,18.5591445967131,23.3458452071822));
#37255=CARTESIAN_POINT('Ctrl Pts',(54.6875239798841,18.5695043742371,23.3416230184738));
#37256=CARTESIAN_POINT('Ctrl Pts',(54.6061312490298,18.5799686089118,23.3373582576347));
#37257=CARTESIAN_POINT('Ctrl Pts',(54.5253564147595,18.5945140100771,23.3330934967957));
#37258=CARTESIAN_POINT('Ctrl Pts',(54.4456301487333,18.6130303064332,23.3288287359566));
#37259=CARTESIAN_POINT('Ctrl Pts',(54.3659038827071,18.6315466027892,23.3245639751176));
#37260=CARTESIAN_POINT('Ctrl Pts',(54.2872266305167,18.6540336001583,23.3202992142786));
#37261=CARTESIAN_POINT('Ctrl Pts',(54.2100098007072,18.680330684123,23.3160344534395));
#37262=CARTESIAN_POINT('Ctrl Pts',(54.13340024849,18.7064209526839,23.3118032331343));
#37263=CARTESIAN_POINT('Ctrl Pts',(54.0579409376308,18.7363593847075,23.3075720128291));
#37264=CARTESIAN_POINT('Ctrl Pts',(53.984045916249,18.7700252132121,23.3033407925239));
#37265=CARTESIAN_POINT('Ctrl Pts',(53.9102568551558,18.803642767275,23.2991156394925));
#37266=CARTESIAN_POINT('Ctrl Pts',(53.8380280481248,18.8409769114683,23.2948904864611));
#37267=CARTESIAN_POINT('Ctrl Pts',(53.7677569098642,18.8818576023287,23.2906653334296));
#37268=CARTESIAN_POINT('Ctrl Pts',(53.6973052478841,18.9228433140349,23.2864293261505));
#37269=CARTESIAN_POINT('Ctrl Pts',(53.6288217706353,18.9673936593575,23.2821933188714));
#37270=CARTESIAN_POINT('Ctrl Pts',(53.5626852952752,19.0152892680338,23.2779573115923));
#37271=CARTESIAN_POINT('Ctrl Pts',(53.4968369609406,19.0629762068387,23.2737397595978));
#37272=CARTESIAN_POINT('Ctrl Pts',(53.433315604212,19.1139790529377,23.2695222076034));
#37273=CARTESIAN_POINT('Ctrl Pts',(53.3724675055654,19.168037055626,23.2653046556089));
#37274=CARTESIAN_POINT('Ctrl Pts',(53.3116394975768,19.2220772095916,23.2610884961542));
#37275=CARTESIAN_POINT('Ctrl Pts',(53.2534833421499,19.2791702083826,23.2568723366995));
#37276=CARTESIAN_POINT('Ctrl Pts',(53.1983117449078,19.3390154481564,23.2526561772448));
#37277=CARTESIAN_POINT('Ctrl Pts',(53.1431414622932,19.3988592619394,23.2484401182526));
#37278=CARTESIAN_POINT('Ctrl Pts',(53.0909559107819,19.4614548437374,23.2442240592604));
#37279=CARTESIAN_POINT('Ctrl Pts',(53.0420294689127,19.5264662713756,23.2400080002683));
#37280=CARTESIAN_POINT('Ctrl Pts',(52.9927025328638,19.5920098590766,23.2357574301401));
#37281=CARTESIAN_POINT('Ctrl Pts',(52.9466886098102,19.6600086520088,23.231506860012));
#37282=CARTESIAN_POINT('Ctrl Pts',(52.9042249844769,19.7300876666836,23.2272562898838));
#37283=CARTESIAN_POINT('Ctrl Pts',(52.8620448923899,19.7996987578032,23.2230341011748));
#37284=CARTESIAN_POINT('Ctrl Pts',(52.8233679997169,19.8713619330961,23.2188119124658));
#37285=CARTESIAN_POINT('Ctrl Pts',(52.7883802832879,19.9446856019886,23.2145897237567));
#37286=CARTESIAN_POINT('Ctrl Pts',(52.7530397873723,20.0187485899594,23.210324962919));
#37287=CARTESIAN_POINT('Ctrl Pts',(52.7214634689174,20.0945052969547,23.2060602020813));
#37288=CARTESIAN_POINT('Ctrl Pts',(52.6937921936552,20.171534065906,23.2017954412436));
#37289=CARTESIAN_POINT('Ctrl Pts',(52.666120918393,20.2485628348572,23.197530680406));
#37290=CARTESIAN_POINT('Ctrl Pts',(52.6423547647779,20.3268631860749,23.1932659195683));
#37291=CARTESIAN_POINT('Ctrl Pts',(52.6225818535924,20.4060023509036,23.1890011587306));
#37292=CARTESIAN_POINT('Ctrl Pts',(52.596985294238,20.5084501043372,23.1834803124126));
#37293=CARTESIAN_POINT('Ctrl Pts',(52.5780003177254,20.6126109162437,23.1779594660946));
#37294=CARTESIAN_POINT('Ctrl Pts',(52.5658093151964,20.7177484100749,23.1724386197766));
#37295=CARTESIAN_POINT('Ctrl Pts',(52.5550546758219,20.8104984384828,23.1675682482834));
#37296=CARTESIAN_POINT('Ctrl Pts',(52.5495868147034,20.9040085164618,23.1626978767901));
#37297=CARTESIAN_POINT('Ctrl Pts',(52.5495010260079,20.9977575763378,23.1578275052968));
#37298=CARTESIAN_POINT('',(52.549839723371,21.0005724374191,22.3578274699494));
#37299=CARTESIAN_POINT('Ctrl Pts',(52.5497869278457,20.9977580128137,23.1578274962121));
#37300=CARTESIAN_POINT('Ctrl Pts',(52.5553781978731,21.6127545089065,23.1258742854819));
#37301=CARTESIAN_POINT('Ctrl Pts',(53.1016016749266,23.0515966978432,23.051576643182));
#37302=CARTESIAN_POINT('Ctrl Pts',(55.5179968719808,23.8498389112592,22.9349345693128));
#37303=CARTESIAN_POINT('Ctrl Pts',(57.6754046717511,22.1100055954292,22.8079012746036));
#37304=CARTESIAN_POINT('Ctrl Pts',(57.3833287996288,19.3538996347802,22.6808679798947));
#37305=CARTESIAN_POINT('Ctrl Pts',(54.9091811680088,18.1048912767784,22.5538346851856));
#37306=CARTESIAN_POINT('Ctrl Pts',(52.8824444977937,19.2929844814695,22.4461545239581));
#37307=CARTESIAN_POINT('Ctrl Pts',(52.554303994583,20.5564224075133,22.3808187943003));
#37308=CARTESIAN_POINT('Ctrl Pts',(52.5533783220755,21.0005711032702,22.3578274962121));
#37309=CARTESIAN_POINT('',(52.5495007750096,21.0019489283386,21.5578274962564));
#37310=CARTESIAN_POINT('Ctrl Pts',(52.5495000668907,21.000572565479,22.3578274674285));
#37311=CARTESIAN_POINT('Ctrl Pts',(52.5495204243597,21.0876996773897,22.3533244795148));
#37312=CARTESIAN_POINT('Ctrl Pts',(52.5541917027174,21.1747038922701,22.348821491601));
#37313=CARTESIAN_POINT('Ctrl Pts',(52.5634494157742,21.2610967263463,22.3443185036873));
#37314=CARTESIAN_POINT('Ctrl Pts',(52.5727418499892,21.3478135777309,22.3397986272661));
#37315=CARTESIAN_POINT('Ctrl Pts',(52.5866550846643,21.4339141026509,22.3352787508448));
#37316=CARTESIAN_POINT('Ctrl Pts',(52.6050731906035,21.5189179392099,22.3307588744236));
#37317=CARTESIAN_POINT('Ctrl Pts',(52.6235282272307,21.6040922194711,22.3262299350648));
#37318=CARTESIAN_POINT('Ctrl Pts',(52.6465060677051,21.6881650763028,22.3217009957059));
#37319=CARTESIAN_POINT('Ctrl Pts',(52.6738411873686,21.7706720628239,22.3171720563471));
#37320=CARTESIAN_POINT('Ctrl Pts',(52.70125775696,21.8534248938186,22.3126296221951));
#37321=CARTESIAN_POINT('Ctrl Pts',(52.7330574340931,21.9346021901369,22.3080871880432));
#37322=CARTESIAN_POINT('Ctrl Pts',(52.7690265296219,22.0137591550605,22.3035447538912));
#37323=CARTESIAN_POINT('Ctrl Pts',(52.7789949718184,22.0356966438323,22.30228586785));
#37324=CARTESIAN_POINT('Ctrl Pts',(52.7892833845875,22.0574791148083,22.3010269818088));
#37325=CARTESIAN_POINT('Ctrl Pts',(52.7998866174955,22.0790974720222,22.2997680957676));
#37326=CARTESIAN_POINT('Ctrl Pts',(52.8355249619605,22.1517585620726,22.2955368754627));
#37327=CARTESIAN_POINT('Ctrl Pts',(52.8748335582081,22.2227884963781,22.2913056551578));
#37328=CARTESIAN_POINT('Ctrl Pts',(52.9176398702462,22.2917919879035,22.2870744348529));
#37329=CARTESIAN_POINT('Ctrl Pts',(52.9603848010288,22.3606965332516,22.2828492818218));
#37330=CARTESIAN_POINT('Ctrl Pts',(53.0066172434651,22.4275800151676,22.2786241287906));
#37331=CARTESIAN_POINT('Ctrl Pts',(53.0561179059046,22.4920699227099,22.2743989757595));
#37332=CARTESIAN_POINT('Ctrl Pts',(53.1057457335535,22.5567255022287,22.2701629684803));
#37333=CARTESIAN_POINT('Ctrl Pts',(53.1586583809308,22.618974772684,22.2659269612011));
#37334=CARTESIAN_POINT('Ctrl Pts',(53.214590001068,22.6784699537715,22.2616909539219));
#37335=CARTESIAN_POINT('Ctrl Pts',(53.2702779403224,22.7377059283811,22.2574734019278));
#37336=CARTESIAN_POINT('Ctrl Pts',(53.3289582867809,22.7942114149242,22.2532558499336));
#37337=CARTESIAN_POINT('Ctrl Pts',(53.3903282957173,22.8476761768318,22.2490382979395));
#37338=CARTESIAN_POINT('Ctrl Pts',(53.4516780416729,22.9011232858912,22.2448221384851));
#37339=CARTESIAN_POINT('Ctrl Pts',(53.5157153362577,22.951531358919,22.2406059790307));
#37340=CARTESIAN_POINT('Ctrl Pts',(53.5821021841165,22.9986285382013,22.2363898195762));
#37341=CARTESIAN_POINT('Ctrl Pts',(53.6484874501112,23.0457245952533,22.2321737605844));
#37342=CARTESIAN_POINT('Ctrl Pts',(53.7172217782354,23.0895096473104,22.2279577015925));
#37343=CARTESIAN_POINT('Ctrl Pts',(53.7879370258276,23.1297543512434,22.2237416426006));
#37344=CARTESIAN_POINT('Ctrl Pts',(53.8592311229034,23.1703284837917,22.2194910724721));
#37345=CARTESIAN_POINT('Ctrl Pts',(53.9325383103316,23.2073037894376,22.2152405023437));
#37346=CARTESIAN_POINT('Ctrl Pts',(54.007456428538,23.2404926933042,22.2109899322152));
#37347=CARTESIAN_POINT('Ctrl Pts',(54.0818743120709,23.2734599920252,22.2067677435064));
#37348=CARTESIAN_POINT('Ctrl Pts',(54.1578812188451,23.3026911884024,22.2025455547977));
#37349=CARTESIAN_POINT('Ctrl Pts',(54.2350650546021,23.3280517131948,22.198323366089));
#37350=CARTESIAN_POINT('Ctrl Pts',(54.313027131335,23.3536679469626,22.1940586052506));
#37351=CARTESIAN_POINT('Ctrl Pts',(54.3921895359128,23.3753348859622,22.1897938444122));
#37352=CARTESIAN_POINT('Ctrl Pts',(54.4721161001478,23.3929665351352,22.1855290835739));
#37353=CARTESIAN_POINT('Ctrl Pts',(54.5520426643828,23.4105981843081,22.1812643227355));
#37354=CARTESIAN_POINT('Ctrl Pts',(54.632732902499,23.4241945269557,22.1769995618971));
#37355=CARTESIAN_POINT('Ctrl Pts',(54.7137463454286,23.4337232988252,22.1727348010588));
#37356=CARTESIAN_POINT('Ctrl Pts',(54.794122652023,23.4431771309493,22.1685035807538));
#37357=CARTESIAN_POINT('Ctrl Pts',(54.875118494528,23.4486626394389,22.1642723604489));
#37358=CARTESIAN_POINT('Ctrl Pts',(54.9563081860119,23.4501104618752,22.160041140144));
#37359=CARTESIAN_POINT('Ctrl Pts',(55.0373814571608,23.4515562082355,22.1558159871128));
#37360=CARTESIAN_POINT('Ctrl Pts',(55.1186475643015,23.448975759219,22.1515908340817));
#37361=CARTESIAN_POINT('Ctrl Pts',(55.1996746058428,23.44235138786,22.1473656810505));
#37362=CARTESIAN_POINT('Ctrl Pts',(55.2809098025917,23.4357099987576,22.1431296737713));
#37363=CARTESIAN_POINT('Ctrl Pts',(55.3619042343381,23.4250038346097,22.1388936664921));
#37364=CARTESIAN_POINT('Ctrl Pts',(55.4422215357371,23.4102676953671,22.1346576592129));
#37365=CARTESIAN_POINT('Ctrl Pts',(55.5221889135895,23.395595758009,22.1304401072187));
#37366=CARTESIAN_POINT('Ctrl Pts',(55.6014845873182,23.3769289640167,22.1262225552246));
#37367=CARTESIAN_POINT('Ctrl Pts',(55.6796837303828,23.3543534731754,22.1220050032304));
#37368=CARTESIAN_POINT('Ctrl Pts',(55.7578570538693,23.3317854362476,22.1177888437759));
#37369=CARTESIAN_POINT('Ctrl Pts',(55.8349341193415,23.3053113941992,22.1135726843215));
#37370=CARTESIAN_POINT('Ctrl Pts',(55.9105032338699,23.2750679354939,22.1093565248671));
#37371=CARTESIAN_POINT('Ctrl Pts',(55.9860705477393,23.244825197429,22.1051404658751));
#37372=CARTESIAN_POINT('Ctrl Pts',(56.0601295508799,23.2108133950625,22.1009244068832));
#37373=CARTESIAN_POINT('Ctrl Pts',(56.1322879260922,23.1732175000275,22.0967083478913));
#37374=CARTESIAN_POINT('Ctrl Pts',(56.2050369637089,23.1353138585709,22.0924577777629));
#37375=CARTESIAN_POINT('Ctrl Pts',(56.2758536812153,23.0937673848603,22.0882072076344));
#37376=CARTESIAN_POINT('Ctrl Pts',(56.3443624118618,23.0488142804006,22.0839566375059));
#37377=CARTESIAN_POINT('Ctrl Pts',(56.4124137038637,23.0041613316578,22.0797344487972));
#37378=CARTESIAN_POINT('Ctrl Pts',(56.4781873936258,22.9561474331056,22.0755122600884));
#37379=CARTESIAN_POINT('Ctrl Pts',(56.5413469648059,22.9050458745352,22.0712900713796));
#37380=CARTESIAN_POINT('Ctrl Pts',(56.6051433709626,22.8534290613605,22.0670253105413));
#37381=CARTESIAN_POINT('Ctrl Pts',(56.6662722839316,22.7986622964092,22.062760549703));
#37382=CARTESIAN_POINT('Ctrl Pts',(56.7244249477072,22.741065435222,22.0584957888647));
#37383=CARTESIAN_POINT('Ctrl Pts',(56.7825776114828,22.6834685740348,22.0542310280263));
#37384=CARTESIAN_POINT('Ctrl Pts',(56.8377537486358,22.6230420157234,22.049966267188));
#37385=CARTESIAN_POINT('Ctrl Pts',(56.8896874176529,22.5601383635962,22.0457015063497));
#37386=CARTESIAN_POINT('Ctrl Pts',(56.9412126504114,22.4977294219872,22.0414702860448));
#37387=CARTESIAN_POINT('Ctrl Pts',(56.9897394831863,22.4326482126616,22.0372390657398));
#37388=CARTESIAN_POINT('Ctrl Pts',(57.0349788184697,22.365214803018,22.0330078454349));
#37389=CARTESIAN_POINT('Ctrl Pts',(57.0801532837126,22.2978780881643,22.0287826924038));
#37390=CARTESIAN_POINT('Ctrl Pts',(57.1220493570732,22.228196254636,22.0245575393726));
#37391=CARTESIAN_POINT('Ctrl Pts',(57.1604179572537,22.1565225894793,22.0203323863415));
#37392=CARTESIAN_POINT('Ctrl Pts',(57.1988851248234,22.0846647975622,22.0160963790623));
#37393=CARTESIAN_POINT('Ctrl Pts',(57.2338063765807,22.0108052951242,22.0118603717831));
#37394=CARTESIAN_POINT('Ctrl Pts',(57.2649743458564,21.9353296010564,22.0076243645039));
#37395=CARTESIAN_POINT('Ctrl Pts',(57.2960065236381,21.8601827367937,22.0034068125097));
#37396=CARTESIAN_POINT('Ctrl Pts',(57.3233178689278,21.7834341635921,21.9991892605156));
#37397=CARTESIAN_POINT('Ctrl Pts',(57.3467504259977,21.7054875534548,21.9949717085214));
#37398=CARTESIAN_POINT('Ctrl Pts',(57.3701752461703,21.627566679515,21.990755549067));
#37399=CARTESIAN_POINT('Ctrl Pts',(57.389723687645,21.5484489990632,21.9865393896125));
#37400=CARTESIAN_POINT('Ctrl Pts',(57.4052872879839,21.4685544923089,21.9823232301581));
#37401=CARTESIAN_POINT('Ctrl Pts',(57.4208505174738,21.3886618892788,21.9781071711662));
#37402=CARTESIAN_POINT('Ctrl Pts',(57.432429006806,21.3079929533049,21.9738911121743));
#37403=CARTESIAN_POINT('Ctrl Pts',(57.4399654527367,21.2269776188338,21.9696750531824));
#37404=CARTESIAN_POINT('Ctrl Pts',(57.4475635892925,21.1452991220876,21.9654244830539));
#37405=CARTESIAN_POINT('Ctrl Pts',(57.4510531431762,21.0632690058505,21.9611739129255));
#37406=CARTESIAN_POINT('Ctrl Pts',(57.450428884532,20.9813309922273,21.956923342797));
#37407=CARTESIAN_POINT('Ctrl Pts',(57.4498087941161,20.899940085718,21.9527011540882));
#37408=CARTESIAN_POINT('Ctrl Pts',(57.445129749118,20.8186405207931,21.9484789653795));
#37409=CARTESIAN_POINT('Ctrl Pts',(57.4364389107779,20.737863234079,21.9442567766707));
#37410=CARTESIAN_POINT('Ctrl Pts',(57.4276604431248,20.6562714737934,21.9399920158324));
#37411=CARTESIAN_POINT('Ctrl Pts',(57.4147889015141,20.5752130629985,21.9357272549941));
#37412=CARTESIAN_POINT('Ctrl Pts',(57.3979256256363,20.4951208620703,21.9314624941558));
#37413=CARTESIAN_POINT('Ctrl Pts',(57.3810623497585,20.4150286611421,21.9271977333174));
#37414=CARTESIAN_POINT('Ctrl Pts',(57.3602075245332,20.3359031195936,21.9229329724791));
#37415=CARTESIAN_POINT('Ctrl Pts',(57.3355132204363,20.2581588801048,21.9186682116408));
#37416=CARTESIAN_POINT('Ctrl Pts',(57.3110131265572,20.1810260660535,21.9144369913358));
#37417=CARTESIAN_POINT('Ctrl Pts',(57.2826419008733,20.1049636518159,21.9102057710309));
#37418=CARTESIAN_POINT('Ctrl Pts',(57.2505117203525,20.0303880948772,21.905974550726));
#37419=CARTESIAN_POINT('Ctrl Pts',(57.2184276122618,19.9559194740675,21.9017493976948));
#37420=CARTESIAN_POINT('Ctrl Pts',(57.1825954368418,19.8829338995233,21.8975242446637));
#37421=CARTESIAN_POINT('Ctrl Pts',(57.1431769810457,19.8118322181124,21.8932990916325));
#37422=CARTESIAN_POINT('Ctrl Pts',(57.1036572608236,19.7405478793442,21.8890630843533));
#37423=CARTESIAN_POINT('Ctrl Pts',(57.0605329596327,19.6711575733102,21.8848270770741));
#37424=CARTESIAN_POINT('Ctrl Pts',(57.0140155653455,19.6040445735819,21.8805910697949));
#37425=CARTESIAN_POINT('Ctrl Pts',(56.9677008363784,19.5372239693712,21.8763735178008));
#37426=CARTESIAN_POINT('Ctrl Pts',(56.9180227782772,19.4726612586684,21.8721559658066));
#37427=CARTESIAN_POINT('Ctrl Pts',(56.8652349234924,19.4107080412384,21.8679384138125));
#37428=CARTESIAN_POINT('Ctrl Pts',(56.8124644980563,19.3487752793513,21.863722254358));
#37429=CARTESIAN_POINT('Ctrl Pts',(56.7565866162777,19.2894506533341,21.8595060949036));
#37430=CARTESIAN_POINT('Ctrl Pts',(56.6978953496814,19.2330530196041,21.8552899354492));
#37431=CARTESIAN_POINT('Ctrl Pts',(56.6392054815791,19.1766567297154,21.8510738764573));
#37432=CARTESIAN_POINT('Ctrl Pts',(56.5777026979492,19.1231876147786,21.8468578174654));
#37433=CARTESIAN_POINT('Ctrl Pts',(56.5137171738508,19.0729269428512,21.8426417584735));
#37434=CARTESIAN_POINT('Ctrl Pts',(56.4492078873559,19.0222548552113,21.838391188345));
#37435=CARTESIAN_POINT('Ctrl Pts',(56.3821753944835,18.9748442882929,21.8341406182165));
#37436=CARTESIAN_POINT('Ctrl Pts',(56.3129896904991,18.9309402322207,21.8298900480881));
#37437=CARTESIAN_POINT('Ctrl Pts',(56.2442659453685,18.8873293272801,21.8256678593793));
#37438=CARTESIAN_POINT('Ctrl Pts',(56.1734180948581,18.8471784269523,21.8214456706706));
#37439=CARTESIAN_POINT('Ctrl Pts',(56.1008337990187,18.8106815679445,21.8172234819618));
#37440=CARTESIAN_POINT('Ctrl Pts',(56.0275176391479,18.7738167128287,21.8129587211235));
#37441=CARTESIAN_POINT('Ctrl Pts',(55.9524302643044,18.7406801969708,21.8086939602851));
#37442=CARTESIAN_POINT('Ctrl Pts',(55.8759903276802,18.7114215775266,21.8044291994468));
#37443=CARTESIAN_POINT('Ctrl Pts',(55.7995503910559,18.6821629580824,21.8001644386084));
#37444=CARTESIAN_POINT('Ctrl Pts',(55.7217583706149,18.6567823234117,21.7958996777701));
#37445=CARTESIAN_POINT('Ctrl Pts',(55.6430451197363,18.6353767268372,21.7916349169317));
#37446=CARTESIAN_POINT('Ctrl Pts',(55.5649509151586,18.6141394761921,21.7874036966268));
#37447=CARTESIAN_POINT('Ctrl Pts',(55.4856570861675,18.5967352815704,21.7831724763219));
#37448=CARTESIAN_POINT('Ctrl Pts',(55.4055743798745,18.5832957002584,21.7789412560169));
#37449=CARTESIAN_POINT('Ctrl Pts',(55.3256065065773,18.5698753903654,21.7747161029858));
#37450=CARTESIAN_POINT('Ctrl Pts',(55.2448524572574,18.5604084792876,21.7704909499546));
#37451=CARTESIAN_POINT('Ctrl Pts',(55.1637367620508,18.5549763758292,21.7662657969234));
#37452=CARTESIAN_POINT('Ctrl Pts',(55.0824126838889,18.5495303175158,21.7620297896442));
#37453=CARTESIAN_POINT('Ctrl Pts',(55.0007255565105,18.54813994154,21.757793782365));
#37454=CARTESIAN_POINT('Ctrl Pts',(54.9191120932702,18.5508353676111,21.7535577750859));
#37455=CARTESIAN_POINT('Ctrl Pts',(54.837854200648,18.5535190503462,21.7493402230917));
#37456=CARTESIAN_POINT('Ctrl Pts',(54.7566697995148,18.5602530003514,21.7451226710975));
#37457=CARTESIAN_POINT('Ctrl Pts',(54.6759917872605,18.5710148357643,21.7409051191034));
#37458=CARTESIAN_POINT('Ctrl Pts',(54.5953404130505,18.5817731178639,21.7366889596489));
#37459=CARTESIAN_POINT('Ctrl Pts',(54.5151955561655,18.5965565829204,21.7324728001945));
#37460=CARTESIAN_POINT('Ctrl Pts',(54.4359845830484,18.6152910325491,21.72825664074));
#37461=CARTESIAN_POINT('Ctrl Pts',(54.3567754973683,18.6340250357738,21.7240405817481));
#37462=CARTESIAN_POINT('Ctrl Pts',(54.2785007033965,18.6567097283014,21.7198245227562));
#37463=CARTESIAN_POINT('Ctrl Pts',(54.2015755606311,18.6832201950512,21.7156084637643));
#37464=CARTESIAN_POINT('Ctrl Pts',(54.1240207364234,18.7099476669094,21.7113578936359));
#37465=CARTESIAN_POINT('Ctrl Pts',(54.0478382196937,18.7405636937724,21.7071073235074));
#37466=CARTESIAN_POINT('Ctrl Pts',(53.9734344793227,18.7748902315264,21.7028567533789));
#37467=CARTESIAN_POINT('Ctrl Pts',(53.8995275390797,18.8089875680566,21.6986345646702));
#37468=CARTESIAN_POINT('Ctrl Pts',(53.8273760807769,18.8467457431168,21.6944123759614));
#37469=CARTESIAN_POINT('Ctrl Pts',(53.7573533386638,18.88794424196,21.6901901872527));
#37470=CARTESIAN_POINT('Ctrl Pts',(53.6866245605454,18.9295581433234,21.6859254264143));
#37471=CARTESIAN_POINT('Ctrl Pts',(53.6180680735121,18.9746818691188,21.681660665576));
#37472=CARTESIAN_POINT('Ctrl Pts',(53.5520365436791,19.0230447452814,21.6773959047377));
#37473=CARTESIAN_POINT('Ctrl Pts',(53.4860050138461,19.0714076214441,21.6731311438994));
#37474=CARTESIAN_POINT('Ctrl Pts',(53.422498774619,19.1230092942825,21.6688663830611));
#37475=CARTESIAN_POINT('Ctrl Pts',(53.3618329917431,19.1775403699784,21.6646016222228));
#37476=CARTESIAN_POINT('Ctrl Pts',(53.3025376716798,19.2308395682001,21.660433203933));
#37477=CARTESIAN_POINT('Ctrl Pts',(53.2457192209134,19.2871501507394,21.6562647856433));
#37478=CARTESIAN_POINT('Ctrl Pts',(53.1917061066508,19.346209370786,21.6520963673536));
#37479=CARTESIAN_POINT('Ctrl Pts',(53.1377834356288,19.4051696980486,21.6479349289476));
#37480=CARTESIAN_POINT('Ctrl Pts',(53.0866570900373,19.4668691686288,21.6437734905416));
#37481=CARTESIAN_POINT('Ctrl Pts',(53.0386211593529,19.5310060267442,21.6396120521356));
#37482=CARTESIAN_POINT('Ctrl Pts',(52.9906304144984,19.5950825534136,21.6354545282587));
#37483=CARTESIAN_POINT('Ctrl Pts',(52.9457246053439,19.6615915387263,21.6312970043818));
#37484=CARTESIAN_POINT('Ctrl Pts',(52.9041589788881,19.7301966041057,21.6271394805048));
#37485=CARTESIAN_POINT('Ctrl Pts',(52.862618829397,19.7987596191427,21.6229845049136));
#37486=CARTESIAN_POINT('Ctrl Pts',(52.8244150485781,19.8694157556614,21.6188295293223));
#37487=CARTESIAN_POINT('Ctrl Pts',(52.789759837469,19.9417993224653,21.614674553731));
#37488=CARTESIAN_POINT('Ctrl Pts',(52.7551145136851,20.0141622378334,21.6105207635775));
#37489=CARTESIAN_POINT('Ctrl Pts',(52.7240159556443,20.0882511718659,21.6063669734239));
#37490=CARTESIAN_POINT('Ctrl Pts',(52.6966298602075,20.1636769469204,21.6022131832704));
#37491=CARTESIAN_POINT('Ctrl Pts',(52.6692293987635,20.2391422883029,21.5980572141505));
#37492=CARTESIAN_POINT('Ctrl Pts',(52.6455454572763,20.3159454208665,21.5939012450306));
#37493=CARTESIAN_POINT('Ctrl Pts',(52.6256947355255,20.393679324871,21.5897452759108));
#37494=CARTESIAN_POINT('Ctrl Pts',(52.6058384923861,20.4714348502102,21.5855881508269));
#37495=CARTESIAN_POINT('Ctrl Pts',(52.5898176915594,20.55012119254,21.5814310257429));
#37496=CARTESIAN_POINT('Ctrl Pts',(52.577697972034,20.6293207109754,21.577273900659));
#37497=CARTESIAN_POINT('Ctrl Pts',(52.565562925504,20.7086203877836,21.573111518335));
#37498=CARTESIAN_POINT('Ctrl Pts',(52.5573388603024,20.7884340588284,21.5689491360109));
#37499=CARTESIAN_POINT('Ctrl Pts',(52.5530394926665,20.8683393545888,21.5647867536869));
#37500=CARTESIAN_POINT('Ctrl Pts',(52.5506433964058,20.9128716664535,21.5624670012101));
#37501=CARTESIAN_POINT('Ctrl Pts',(52.5494653701911,20.9574324221442,21.5601472487332));
#37502=CARTESIAN_POINT('Ctrl Pts',(52.5495007750096,21.0019489283386,21.5578274962564));
#37503=CARTESIAN_POINT('',(52.5495006451703,20.9982218044437,20.7578274962121));
#37504=CARTESIAN_POINT('Ctrl Pts',(52.5495007750103,21.0019489291882,21.5578274962121));
#37505=CARTESIAN_POINT('Ctrl Pts',(52.549603842401,21.1315414062361,21.5510744399793));
#37506=CARTESIAN_POINT('Ctrl Pts',(52.5599894688701,21.2607346644996,21.5443213837466));
#37507=CARTESIAN_POINT('Ctrl Pts',(52.5804550312434,21.3882684563092,21.5375683275139));
#37508=CARTESIAN_POINT('Ctrl Pts',(52.5932780109556,21.4681765084389,21.5333371072089));
#37509=CARTESIAN_POINT('Ctrl Pts',(52.6100878594765,21.5475984594314,21.5291058869039));
#37510=CARTESIAN_POINT('Ctrl Pts',(52.6308352261214,21.6261058410628,21.5248746665989));
#37511=CARTESIAN_POINT('Ctrl Pts',(52.6515528424947,21.7045006486037,21.5206495135677));
#37512=CARTESIAN_POINT('Ctrl Pts',(52.6761966455775,21.7819830456807,21.5164243605364));
#37513=CARTESIAN_POINT('Ctrl Pts',(52.704665911512,21.8581326658652,21.5121992075052));
#37514=CARTESIAN_POINT('Ctrl Pts',(52.7332083138438,21.9344779113565,21.507963200226));
#37515=CARTESIAN_POINT('Ctrl Pts',(52.7655957779776,22.0094830584573,21.5037271929468));
#37516=CARTESIAN_POINT('Ctrl Pts',(52.8016758266753,22.0827377701809,21.4994911856677));
#37517=CARTESIAN_POINT('Ctrl Pts',(52.8375986831078,22.1556733283977,21.4952736336734));
#37518=CARTESIAN_POINT('Ctrl Pts',(52.8771818163744,22.2268732485597,21.4910560816792));
#37519=CARTESIAN_POINT('Ctrl Pts',(52.9202264825812,22.2959523009137,21.4868385296849));
#37520=CARTESIAN_POINT('Ctrl Pts',(52.9632569364185,22.3650085449361,21.4826223702304));
#37521=CARTESIAN_POINT('Ctrl Pts',(53.0097464078368,22.4319449174975,21.4784062107759));
#37522=CARTESIAN_POINT('Ctrl Pts',(53.0594512170528,22.4964025765155,21.4741900513214));
#37523=CARTESIAN_POINT('Ctrl Pts',(53.1091548419039,22.5608586996381,21.4699739923294));
#37524=CARTESIAN_POINT('Ctrl Pts',(53.162073367439,22.6228358591552,21.4657579333374));
#37525=CARTESIAN_POINT('Ctrl Pts',(53.217921848186,22.6820070483881,21.4615418743454));
#37526=CARTESIAN_POINT('Ctrl Pts',(53.2742274844283,22.7416625916081,21.457291304217));
#37527=CARTESIAN_POINT('Ctrl Pts',(53.3335109467948,22.798465655308,21.4530407340886));
#37528=CARTESIAN_POINT('Ctrl Pts',(53.3954425421333,22.8521192225136,21.4487901639602));
#37529=CARTESIAN_POINT('Ctrl Pts',(53.4569606149237,22.9054145402715,21.4445679752514));
#37530=CARTESIAN_POINT('Ctrl Pts',(53.5210911569203,22.9556020516917,21.4403457865426));
#37531=CARTESIAN_POINT('Ctrl Pts',(53.5874794686101,23.0024325203117,21.4361235978337));
#37532=CARTESIAN_POINT('Ctrl Pts',(53.6545371705108,23.0497351783348,21.4318588369956));
#37533=CARTESIAN_POINT('Ctrl Pts',(53.723898017794,23.0936124550003,21.4275940761574));
#37534=CARTESIAN_POINT('Ctrl Pts',(53.7951700802675,23.133854520467,21.4233293153193));
#37535=CARTESIAN_POINT('Ctrl Pts',(53.866442142741,23.1740965859337,21.4190645544811));
#37536=CARTESIAN_POINT('Ctrl Pts',(53.9396249607651,23.2107032821244,21.4147997936429));
#37537=CARTESIAN_POINT('Ctrl Pts',(54.0143067729884,23.2435149012707,21.4105350328048));
#37538=CARTESIAN_POINT('Ctrl Pts',(54.0884012444677,23.2760684709638,21.4063038124999));
#37539=CARTESIAN_POINT('Ctrl Pts',(54.1642490439065,23.305008557811,21.4020725921949));
#37540=CARTESIAN_POINT('Ctrl Pts',(54.2414633981289,23.3301443031756,21.39784137189));
#37541=CARTESIAN_POINT('Ctrl Pts',(54.3185670323716,23.3552440056407,21.3936162188589));
#37542=CARTESIAN_POINT('Ctrl Pts',(54.3970328912392,23.3765500582797,21.3893910658277));
#37543=CARTESIAN_POINT('Ctrl Pts',(54.4764531533141,23.3939191609838,21.3851659127966));
#37544=CARTESIAN_POINT('Ctrl Pts',(54.5560774428452,23.4113328842135,21.3809299055174));
#37545=CARTESIAN_POINT('Ctrl Pts',(54.6366606107811,23.4247892199005,21.3766938982382));
#37546=CARTESIAN_POINT('Ctrl Pts',(54.7177752009829,23.434193791139,21.372457890959));
#37547=CARTESIAN_POINT('Ctrl Pts',(54.7985363940386,23.4435573888778,21.3682403389648));
#37548=CARTESIAN_POINT('Ctrl Pts',(54.8798239246373,23.4489043916971,21.3640227869707));
#37549=CARTESIAN_POINT('Ctrl Pts',(54.9612063458353,23.4501929112616,21.3598052349765));
#37550=CARTESIAN_POINT('Ctrl Pts',(55.0425618964092,23.4514810053863,21.3555890755221));
#37551=CARTESIAN_POINT('Ctrl Pts',(55.1240118108655,23.4487132699912,21.3513729160677));
#37552=CARTESIAN_POINT('Ctrl Pts',(55.2051224488941,23.4418998814365,21.3471567566133));
#37553=CARTESIAN_POINT('Ctrl Pts',(55.2862311542206,23.4350866552311,21.3429406976214));
#37554=CARTESIAN_POINT('Ctrl Pts',(55.3670001359959,23.4242280075553,21.3387246386295));
#37555=CARTESIAN_POINT('Ctrl Pts',(55.4470001279844,23.4093860495118,21.3345085796376));
#37556=CARTESIAN_POINT('Ctrl Pts',(55.5276549710213,23.3944226005587,21.3302580095091));
#37557=CARTESIAN_POINT('Ctrl Pts',(55.6075277022202,23.3754104000805,21.3260074393806));
#37558=CARTESIAN_POINT('Ctrl Pts',(55.686189990587,23.3524654188358,21.3217568692522));
#37559=CARTESIAN_POINT('Ctrl Pts',(55.7643270441368,23.3296736431903,21.3175346805434));
#37560=CARTESIAN_POINT('Ctrl Pts',(55.8412693467259,23.3030016580496,21.3133124918347));
#37561=CARTESIAN_POINT('Ctrl Pts',(55.9166151552415,23.2726123530382,21.3090903031259));
#37562=CARTESIAN_POINT('Ctrl Pts',(55.9927206719904,23.2419166340977,21.3048255422876));
#37563=CARTESIAN_POINT('Ctrl Pts',(56.0671968778821,23.2074284143686,21.3005607814492));
#37564=CARTESIAN_POINT('Ctrl Pts',(56.1396549533528,23.1693632331397,21.2962960206109));
#37565=CARTESIAN_POINT('Ctrl Pts',(56.2121130288235,23.1312980519109,21.2920312597725));
#37566=CARTESIAN_POINT('Ctrl Pts',(56.2825525918245,23.0896562096749,21.2877664989342));
#37567=CARTESIAN_POINT('Ctrl Pts',(56.3506161842434,23.0446970858442,21.2835017380958));
#37568=CARTESIAN_POINT('Ctrl Pts',(56.4181444854036,23.0000915464356,21.2792705177909));
#37569=CARTESIAN_POINT('Ctrl Pts',(56.4835873031694,22.9520534895508,21.275039297486));
#37570=CARTESIAN_POINT('Ctrl Pts',(56.5465745545015,22.9008044079727,21.2708080771811));
#37571=CARTESIAN_POINT('Ctrl Pts',(56.6094714865237,22.8496288139906,21.26658292415));
#37572=CARTESIAN_POINT('Ctrl Pts',(56.6699194877135,22.7952516309173,21.2623577711188));
#37573=CARTESIAN_POINT('Ctrl Pts',(56.7275770225726,22.7379378242846,21.2581326180877));
#37574=CARTESIAN_POINT('Ctrl Pts',(56.7853826773179,22.6804767807897,21.2538966108085));
#37575=CARTESIAN_POINT('Ctrl Pts',(56.8403831198812,22.6200642717991,21.2496606035293));
#37576=CARTESIAN_POINT('Ctrl Pts',(56.8922672753953,22.5570082878611,21.2454245962501));
#37577=CARTESIAN_POINT('Ctrl Pts',(56.9439253838756,22.4942270239794,21.241207044256));
#37578=CARTESIAN_POINT('Ctrl Pts',(56.9924939989411,22.428825627201,21.2369894922618));
#37579=CARTESIAN_POINT('Ctrl Pts',(57.0377039845765,22.3611439017389,21.2327719402677));
#37580=CARTESIAN_POINT('Ctrl Pts',(57.0828990429031,22.2934845232429,21.2285557808133));
#37581=CARTESIAN_POINT('Ctrl Pts',(57.1247374159642,22.2235466975424,21.2243396213588));
#37582=CARTESIAN_POINT('Ctrl Pts',(57.162992525052,22.1517003024091,21.2201234619044));
#37583=CARTESIAN_POINT('Ctrl Pts',(57.2012467225981,22.0798556192298,21.2159074029125));
#37584=CARTESIAN_POINT('Ctrl Pts',(57.2359176084042,22.0061028679338,21.2116913439207));
#37585=CARTESIAN_POINT('Ctrl Pts',(57.266824612889,21.9308364111919,21.2074752849288));
#37586=CARTESIAN_POINT('Ctrl Pts',(57.2979846109529,21.8549538504116,21.2032247148003));
#37587=CARTESIAN_POINT('Ctrl Pts',(57.3253186266574,21.7775331261725,21.1989741446718));
#37588=CARTESIAN_POINT('Ctrl Pts',(57.3486918523176,21.6989970192045,21.1947235745433));
#37589=CARTESIAN_POINT('Ctrl Pts',(57.371909012954,21.6209853045299,21.1905013858346));
#37590=CARTESIAN_POINT('Ctrl Pts',(57.3912180642631,21.5418735275523,21.1862791971258));
#37591=CARTESIAN_POINT('Ctrl Pts',(57.4065380379803,21.4620875693566,21.1820570084171));
#37592=CARTESIAN_POINT('Ctrl Pts',(57.4220124822701,21.381497133107,21.1777922475787));
#37593=CARTESIAN_POINT('Ctrl Pts',(57.4334168853248,21.3002193247265,21.1735274867403));
#37594=CARTESIAN_POINT('Ctrl Pts',(57.4407215244208,21.2186977142746,21.169262725902));
#37595=CARTESIAN_POINT('Ctrl Pts',(57.4480261635168,21.1371761038228,21.1649979650636));
#37596=CARTESIAN_POINT('Ctrl Pts',(57.4512310839835,21.0554111752442,21.1607332042252));
#37597=CARTESIAN_POINT('Ctrl Pts',(57.4503604039834,20.9738439186702,21.1564684433868));
#37598=CARTESIAN_POINT('Ctrl Pts',(57.4494965715118,20.8929181539406,21.1522372230819));
#37599=CARTESIAN_POINT('Ctrl Pts',(57.4446178218065,20.8118835001941,21.148006002777));
#37600=CARTESIAN_POINT('Ctrl Pts',(57.4357095938325,20.7311710125144,21.143774782472));
#37601=CARTESIAN_POINT('Ctrl Pts',(57.4268141396339,20.650574260893,21.1395496294409));
#37602=CARTESIAN_POINT('Ctrl Pts',(57.4139007332612,20.5702992160609,21.1353244764097));
#37603=CARTESIAN_POINT('Ctrl Pts',(57.3970068201212,20.490776518322,21.1310993233785));
#37604=CARTESIAN_POINT('Ctrl Pts',(57.3800695071986,20.4110495299743,21.1268633160993));
#37605=CARTESIAN_POINT('Ctrl Pts',(57.3591312212664,20.3320792310835,21.1226273088201));
#37606=CARTESIAN_POINT('Ctrl Pts',(57.3342820752912,20.2542939969571,21.1183913015409));
#37607=CARTESIAN_POINT('Ctrl Pts',(57.3095411911866,20.1768476547571,21.1141737495468));
#37608=CARTESIAN_POINT('Ctrl Pts',(57.2809235879493,20.1005765209318,21.1099561975526));
#37609=CARTESIAN_POINT('Ctrl Pts',(57.248568849674,20.0258909823456,21.1057386455584));
#37610=CARTESIAN_POINT('Ctrl Pts',(57.2162247941972,19.9512301032252,21.101522486104));
#37611=CARTESIAN_POINT('Ctrl Pts',(57.1801462387363,19.8781542059672,21.0973063266495));
#37612=CARTESIAN_POINT('Ctrl Pts',(57.1405211117549,19.8070542258211,21.0930901671951));
#37613=CARTESIAN_POINT('Ctrl Pts',(57.1008969289601,19.7359559398434,21.0888741082032));
#37614=CARTESIAN_POINT('Ctrl Pts',(57.0577265699682,19.6668338829374,21.0846580492113));
#37615=CARTESIAN_POINT('Ctrl Pts',(57.0112434834743,19.6000536081042,21.0804419902193));
#37616=CARTESIAN_POINT('Ctrl Pts',(56.9643799032188,19.5327266940546,21.0761914200909));
#37617=CARTESIAN_POINT('Ctrl Pts',(56.9141493724349,19.4677804798977,21.0719408499624));
#37618=CARTESIAN_POINT('Ctrl Pts',(56.8608340307758,19.4055574767629,21.067690279834));
#37619=CARTESIAN_POINT('Ctrl Pts',(56.8078746802055,19.3437499419331,21.0634680911252));
#37620=CARTESIAN_POINT('Ctrl Pts',(56.7518719561585,19.2846296609929,21.0592459024164));
#37621=CARTESIAN_POINT('Ctrl Pts',(56.6931397962257,19.2284955883666,21.0550237137077));
#37622=CARTESIAN_POINT('Ctrl Pts',(56.6338154426954,19.1717955185344,21.0507589528694));
#37623=CARTESIAN_POINT('Ctrl Pts',(56.5717066695522,19.1181425331317,21.0464941920311));
#37624=CARTESIAN_POINT('Ctrl Pts',(56.5071700637402,19.0678021196148,21.0422294311927));
#37625=CARTESIAN_POINT('Ctrl Pts',(56.4426334579283,19.0174617060978,21.0379646703544));
#37626=CARTESIAN_POINT('Ctrl Pts',(56.3756694506535,18.9704340887847,21.0336999095161));
#37627=CARTESIAN_POINT('Ctrl Pts',(56.306661654817,18.9269381172211,21.0294351486778));
#37628=CARTESIAN_POINT('Ctrl Pts',(56.2381965759975,18.8837842230076,21.0252039283729));
#37629=CARTESIAN_POINT('Ctrl Pts',(56.1674630289766,18.8439447622647,21.020972708068));
#37630=CARTESIAN_POINT('Ctrl Pts',(56.0948153061716,18.8076656971683,21.0167414877631));
#37631=CARTESIAN_POINT('Ctrl Pts',(56.0222717551164,18.7714386537121,21.0125163347319));
#37632=CARTESIAN_POINT('Ctrl Pts',(55.9478198920762,18.7387620722398,21.0082911817008));
#37633=CARTESIAN_POINT('Ctrl Pts',(55.8718418599838,18.7098379923726,21.0040660286696));
#37634=CARTESIAN_POINT('Ctrl Pts',(55.7956686433856,18.6808396077086,20.9998300213904));
#37635=CARTESIAN_POINT('Ctrl Pts',(55.7179618090992,18.655613275635,20.9955940141112));
#37636=CARTESIAN_POINT('Ctrl Pts',(55.6391301544288,18.634315554496,20.991358006832));
#37637=CARTESIAN_POINT('Ctrl Pts',(55.5606419506927,18.6131106225068,20.9871404548379));
#37638=CARTESIAN_POINT('Ctrl Pts',(55.4810391568323,18.595800270702,20.9829229028437));
#37639=CARTESIAN_POINT('Ctrl Pts',(55.4007422799513,18.5824897363073,20.9787053508496));
#37640=CARTESIAN_POINT('Ctrl Pts',(55.3204719152723,18.5691835967483,20.9744891913951));
#37641=CARTESIAN_POINT('Ctrl Pts',(55.2395083809756,18.5598747279479,20.9702730319407));
#37642=CARTESIAN_POINT('Ctrl Pts',(55.1582820536027,18.5546171993924,20.9660568724863));
#37643=CARTESIAN_POINT('Ctrl Pts',(55.0770576616885,18.5493597961132,20.9618408134944));
#37644=CARTESIAN_POINT('Ctrl Pts',(54.9955709531706,18.5481535700658,20.9576247545025));
#37645=CARTESIAN_POINT('Ctrl Pts',(54.9142556595911,18.551000580219,20.9534086955106));
#37646=CARTESIAN_POINT('Ctrl Pts',(54.8322747483795,18.5538708949692,20.9491581253821));
#37647=CARTESIAN_POINT('Ctrl Pts',(54.750468551326,18.5608611081166,20.9449075552536));
#37648=CARTESIAN_POINT('Ctrl Pts',(54.6692778406778,18.5719198729586,20.9406569851252));
#37649=CARTESIAN_POINT('Ctrl Pts',(54.5886292473379,18.5829047974834,20.9364347964164));
#37650=CARTESIAN_POINT('Ctrl Pts',(54.5085883962111,18.5979039597923,20.9322126077077));
#37651=CARTESIAN_POINT('Ctrl Pts',(54.4295767031962,18.6168156780342,20.9279904189989));
#37652=CARTESIAN_POINT('Ctrl Pts',(54.3497683390076,18.6359180822391,20.9237256581606));
#37653=CARTESIAN_POINT('Ctrl Pts',(54.2710104698192,18.6590122500086,20.9194608973222));
#37654=CARTESIAN_POINT('Ctrl Pts',(54.1937195168102,18.6859425174756,20.9151961364839));
#37655=CARTESIAN_POINT('Ctrl Pts',(54.1164285638013,18.7128727849425,20.9109313756456));
#37656=CARTESIAN_POINT('Ctrl Pts',(54.040604949261,18.7436389114226,20.9066666148072));
#37657=CARTESIAN_POINT('Ctrl Pts',(53.9666405616107,18.77803723679,20.9024018539689));
#37658=CARTESIAN_POINT('Ctrl Pts',(53.8932578724681,18.812165033932,20.898170633664));
#37659=CARTESIAN_POINT('Ctrl Pts',(53.8214300745687,18.8499960365009,20.893939413359));
#37660=CARTESIAN_POINT('Ctrl Pts',(53.751555939118,18.8913659215387,20.8897081930541));
#37661=CARTESIAN_POINT('Ctrl Pts',(53.681781998287,18.9326764850568,20.885483040023));
#37662=CARTESIAN_POINT('Ctrl Pts',(53.6139565527698,18.9775156178237,20.8812578869918));
#37663=CARTESIAN_POINT('Ctrl Pts',(53.5484565696458,19.0256717801248,20.8770327339607));
#37664=CARTESIAN_POINT('Ctrl Pts',(53.482788319702,19.0739516536682,20.8727967266815));
#37665=CARTESIAN_POINT('Ctrl Pts',(53.4194579207677,19.1255654163242,20.8685607194023));
#37666=CARTESIAN_POINT('Ctrl Pts',(53.3588185775264,19.1802544714913,20.8643247121231));
#37667=CARTESIAN_POINT('Ctrl Pts',(53.2984434256075,19.2347052593383,20.8601071601289));
#37668=CARTESIAN_POINT('Ctrl Pts',(53.2407362826118,19.2922042916543,20.8558896081348));
#37669=CARTESIAN_POINT('Ctrl Pts',(53.1860135807132,19.3524553054187,20.8516720561406));
#37670=CARTESIAN_POINT('Ctrl Pts',(53.1313089470058,19.4126864256691,20.8474558966862));
#37671=CARTESIAN_POINT('Ctrl Pts',(53.0795871098758,19.4756673790442,20.8432397372318));
#37672=CARTESIAN_POINT('Ctrl Pts',(53.031126859977,19.5410658656074,20.8390235777773));
#37673=CARTESIAN_POINT('Ctrl Pts',(52.9826677647877,19.6064627938572,20.8348075187854));
#37674=CARTESIAN_POINT('Ctrl Pts',(52.9374703782139,19.6742767665566,20.8305914597936));
#37675=CARTESIAN_POINT('Ctrl Pts',(52.8957716089877,19.7441444635399,20.8263754008017));
#37676=CARTESIAN_POINT('Ctrl Pts',(52.8537315086929,19.8145840722631,20.8221248306732));
#37677=CARTESIAN_POINT('Ctrl Pts',(52.8152478265902,19.8871107788478,20.8178742605447));
#37678=CARTESIAN_POINT('Ctrl Pts',(52.7805164157013,19.9613263895579,20.8136236904162));
#37679=CARTESIAN_POINT('Ctrl Pts',(52.7460169094089,20.0350464562976,20.8094015017075));
#37680=CARTESIAN_POINT('Ctrl Pts',(52.7152198387914,20.1104324839184,20.8051793129987));
#37681=CARTESIAN_POINT('Ctrl Pts',(52.6882682680638,20.1870752497561,20.80095712429));
#37682=CARTESIAN_POINT('Ctrl Pts',(52.6610449459197,20.2644908009867,20.7966923634516));
#37683=CARTESIAN_POINT('Ctrl Pts',(52.637745246046,20.3431881105333,20.7924276026133));
#37684=CARTESIAN_POINT('Ctrl Pts',(52.6184641668122,20.4227328822438,20.7881628417749));
#37685=CARTESIAN_POINT('Ctrl Pts',(52.5991830875784,20.5022776539543,20.7838980809366));
#37686=CARTESIAN_POINT('Ctrl Pts',(52.5839206557274,20.5826694025021,20.7796333200982));
#37687=CARTESIAN_POINT('Ctrl Pts',(52.5727182392775,20.6634684204062,20.7753685592599));
#37688=CARTESIAN_POINT('Ctrl Pts',(52.5573596372609,20.7742445163375,20.769521538244));
#37689=CARTESIAN_POINT('Ctrl Pts',(52.5495820092598,20.8860954143571,20.763674517228));
#37690=CARTESIAN_POINT('Ctrl Pts',(52.5495006451703,20.9982218044437,20.7578274962121));
#37691=CARTESIAN_POINT('',(52.5497641805207,20.9991538160394,19.9578275400623));
#37692=CARTESIAN_POINT('Ctrl Pts',(52.5472108677062,20.9982398775261,20.7578264680766));
#37693=CARTESIAN_POINT('Ctrl Pts',(52.5529443810253,21.6987907323952,20.7213294002347));
#37694=CARTESIAN_POINT('Ctrl Pts',(53.2348022320658,23.221863456408,20.6424879008231));
#37695=CARTESIAN_POINT('Ctrl Pts',(55.8195806506902,23.7781630867416,20.521301969842));
#37696=CARTESIAN_POINT('Ctrl Pts',(57.778705419208,21.8177400398511,20.3942686751329));
#37697=CARTESIAN_POINT('Ctrl Pts',(57.1937688630138,19.1086299264319,20.2672353804239));
#37698=CARTESIAN_POINT('Ctrl Pts',(54.6003133464515,18.1311756487213,20.1402020857151));
#37699=CARTESIAN_POINT('Ctrl Pts',(52.7918351476342,19.4700594808486,20.0370663306344));
#37700=CARTESIAN_POINT('Ctrl Pts',(52.5521271605753,20.6428395652265,19.9762750071234));
#37701=CARTESIAN_POINT('Ctrl Pts',(52.5532271445043,20.9991439022597,19.9578281151821));
#37702=CARTESIAN_POINT('',(52.5495010013229,21.0022152838851,19.1578274961645));
#37703=CARTESIAN_POINT('Ctrl Pts',(52.5495001458373,20.9991545719183,19.9578274962121));
#37704=CARTESIAN_POINT('Ctrl Pts',(52.549471344841,21.0826351645882,19.9535120362847));
#37705=CARTESIAN_POINT('Ctrl Pts',(52.5537127576159,21.1660840188203,19.9491965763572));
#37706=CARTESIAN_POINT('Ctrl Pts',(52.5621884503673,21.2490483858156,19.9448811164298));
#37707=CARTESIAN_POINT('Ctrl Pts',(52.5706699431405,21.3320695263584,19.9405627033795));
#37708=CARTESIAN_POINT('Ctrl Pts',(52.5833914368997,21.4146050890858,19.9362442903292));
#37709=CARTESIAN_POINT('Ctrl Pts',(52.6002654346689,21.4962099011055,19.9319258772788));
#37710=CARTESIAN_POINT('Ctrl Pts',(52.6171689861287,21.577957638554,19.9275999008138));
#37711=CARTESIAN_POINT('Ctrl Pts',(52.6382394758439,21.658770945012,19.9232739243488));
#37712=CARTESIAN_POINT('Ctrl Pts',(52.6633387861678,21.7382171914635,19.9189479478837));
#37713=CARTESIAN_POINT('Ctrl Pts',(52.6884622139892,21.817739776453,19.914617814662));
#37714=CARTESIAN_POINT('Ctrl Pts',(52.7176220232487,21.8958922788628,19.9102876814402));
#37715=CARTESIAN_POINT('Ctrl Pts',(52.7506318224984,21.972261822784,19.9059575482185));
#37716=CARTESIAN_POINT('Ctrl Pts',(52.7837104239721,22.0487905435128,19.9016183897132));
#37717=CARTESIAN_POINT('Ctrl Pts',(52.8206548525578,22.1235284940726,19.897279231208));
#37718=CARTESIAN_POINT('Ctrl Pts',(52.861232598174,22.1960870582389,19.8929400727027));
#37719=CARTESIAN_POINT('Ctrl Pts',(52.8824436517367,22.2340153257557,19.8906718805675));
#37720=CARTESIAN_POINT('Ctrl Pts',(52.904646760021,22.271348570579,19.8884036884323));
#37721=CARTESIAN_POINT('Ctrl Pts',(52.9278041874616,22.3080346954489,19.8861354962971));
#37722=CARTESIAN_POINT('Ctrl Pts',(52.9710034278058,22.3764711713755,19.8819042759922));
#37723=CARTESIAN_POINT('Ctrl Pts',(53.0176775874499,22.4428936083075,19.8776730556872));
#37724=CARTESIAN_POINT('Ctrl Pts',(53.0676128757991,22.5069274210202,19.8734418353823));
#37725=CARTESIAN_POINT('Ctrl Pts',(53.1174765604398,22.5708694137272,19.8692166823511));
#37726=CARTESIAN_POINT('Ctrl Pts',(53.1705918029512,22.6324292212306,19.86499152932));
#37727=CARTESIAN_POINT('Ctrl Pts',(53.2267007588123,22.6912599005484,19.8607663762888));
#37728=CARTESIAN_POINT('Ctrl Pts',(53.2829538563221,22.750241713513,19.8565303690096));
#37729=CARTESIAN_POINT('Ctrl Pts',(53.342215810946,22.8064799625865,19.8522943617304));
#37730=CARTESIAN_POINT('Ctrl Pts',(53.404185132303,22.8596572689712,19.8480583544512));
#37731=CARTESIAN_POINT('Ctrl Pts',(53.4658844679367,22.912602894369,19.8438408024571));
#37732=CARTESIAN_POINT('Ctrl Pts',(53.5302672790467,22.962513882173,19.8396232504629));
#37733=CARTESIAN_POINT('Ctrl Pts',(53.5969994009295,23.0091141254314,19.8354056984688));
#37734=CARTESIAN_POINT('Ctrl Pts',(53.6637094893839,23.0556989823496,19.8311895390143));
#37735=CARTESIAN_POINT('Ctrl Pts',(53.7327669673213,23.0989749995541,19.8269733795599));
#37736=CARTESIAN_POINT('Ctrl Pts',(53.8038067226578,23.1387079962541,19.8227572201054));
#37737=CARTESIAN_POINT('Ctrl Pts',(53.8748447852608,23.1784400461973,19.8185411611135));
#37738=CARTESIAN_POINT('Ctrl Pts',(53.947864625042,23.2146290175103,19.8143251021216));
#37739=CARTESIAN_POINT('Ctrl Pts',(54.0224756986029,23.2470862222394,19.8101090431297));
#37740=CARTESIAN_POINT('Ctrl Pts',(54.0976975114716,23.2798091099268,19.8058584730013));
#37741=CARTESIAN_POINT('Ctrl Pts',(54.1745362953992,23.308738649168,19.8016079028728));
#37742=CARTESIAN_POINT('Ctrl Pts',(54.2525721484682,23.3337313163161,19.7973573327443));
#37743=CARTESIAN_POINT('Ctrl Pts',(54.3300869494825,23.3585571052915,19.7931351440356));
#37744=CARTESIAN_POINT('Ctrl Pts',(54.4087824128415,23.3794983747325,19.7889129553268));
#37745=CARTESIAN_POINT('Ctrl Pts',(54.4882344233204,23.3964653647666,19.784690766618));
#37746=CARTESIAN_POINT('Ctrl Pts',(54.568487544673,23.4136034321608,19.7804260057797));
#37747=CARTESIAN_POINT('Ctrl Pts',(54.6495120758896,23.4266865466672,19.7761612449414));
#37748=CARTESIAN_POINT('Ctrl Pts',(54.7308651565917,23.4356758171119,19.771896484103));
#37749=CARTESIAN_POINT('Ctrl Pts',(54.8122182372939,23.4446650875565,19.7676317232647));
#37750=CARTESIAN_POINT('Ctrl Pts',(54.893899382703,23.4495605492491,19.7633669624264));
#37751=CARTESIAN_POINT('Ctrl Pts',(54.9754671981716,23.4503771937468,19.759102201588));
#37752=CARTESIAN_POINT('Ctrl Pts',(55.0563935174008,23.4511874156822,19.7548709812831));
#37753=CARTESIAN_POINT('Ctrl Pts',(55.1375117469533,23.4479858315854,19.7506397609782));
#37754=CARTESIAN_POINT('Ctrl Pts',(55.2183912251447,23.4407489675876,19.7464085406732));
#37755=CARTESIAN_POINT('Ctrl Pts',(55.2991547278249,23.4335224807462,19.7421833876421));
#37756=CARTESIAN_POINT('Ctrl Pts',(55.3796796999174,23.4222722471323,19.7379582346109));
#37757=CARTESIAN_POINT('Ctrl Pts',(55.4595348187269,23.4070267967718,19.7337330815798));
#37758=CARTESIAN_POINT('Ctrl Pts',(55.5395950821221,23.3917421814631,19.7294970743006));
#37759=CARTESIAN_POINT('Ctrl Pts',(55.6189815741237,23.3724417977264,19.7252610670214));
#37760=CARTESIAN_POINT('Ctrl Pts',(55.6972641471716,23.3492068787293,19.7210250597422));
#37761=CARTESIAN_POINT('Ctrl Pts',(55.7752056615044,23.3260731887965,19.716807507748));
#37762=CARTESIAN_POINT('Ctrl Pts',(55.8520524049936,23.2990393010793,19.7125899557539));
#37763=CARTESIAN_POINT('Ctrl Pts',(55.9273911914125,23.2682362813628,19.7083724037597));
#37764=CARTESIAN_POINT('Ctrl Pts',(56.0027051026781,23.2374434321026,19.7041562443053));
#37765=CARTESIAN_POINT('Ctrl Pts',(56.0765116156152,23.2028840980203,19.6999400848509));
#37766=CARTESIAN_POINT('Ctrl Pts',(56.1484159914954,23.1647380812647,19.6957239253964));
#37767=CARTESIAN_POINT('Ctrl Pts',(56.2203186540399,23.1265929734515,19.6915078664046));
#37768=CARTESIAN_POINT('Ctrl Pts',(56.2903188594575,23.0848615717513,19.6872918074127));
#37769=CARTESIAN_POINT('Ctrl Pts',(56.3580463042962,23.0397697138127,19.6830757484208));
#37770=CARTESIAN_POINT('Ctrl Pts',(56.4263281415435,22.9943087502067,19.6788251782923));
#37771=CARTESIAN_POINT('Ctrl Pts',(56.4922994302679,22.9454323139594,19.6745746081638));
#37772=CARTESIAN_POINT('Ctrl Pts',(56.5556118968356,22.8934153998591,19.6703240380353));
#37773=CARTESIAN_POINT('Ctrl Pts',(56.6185016206574,22.8417458071362,19.6661018493266));
#37774=CARTESIAN_POINT('Ctrl Pts',(56.6787676146706,22.7869779088318,19.6618796606178));
#37775=CARTESIAN_POINT('Ctrl Pts',(56.7361044949192,22.7294193917964,19.6576574719091));
#37776=CARTESIAN_POINT('Ctrl Pts',(56.7940195002267,22.6712805149488,19.6533927110707));
#37777=CARTESIAN_POINT('Ctrl Pts',(56.8489456659615,22.6102947882438,19.6491279502324));
#37778=CARTESIAN_POINT('Ctrl Pts',(56.900610185816,22.5468132309922,19.6448631893941));
#37779=CARTESIAN_POINT('Ctrl Pts',(56.9522747056704,22.4833316737407,19.6405984285557));
#37780=CARTESIAN_POINT('Ctrl Pts',(57.0006773464554,22.4173547124163,19.6363336677174));
#37781=CARTESIAN_POINT('Ctrl Pts',(57.0455913707908,22.3492613511645,19.6320689068791));
#37782=CARTESIAN_POINT('Ctrl Pts',(57.0901521653928,22.2817035152903,19.6278376865741));
#37783=CARTESIAN_POINT('Ctrl Pts',(57.131446156631,22.2118091407379,19.6236064662692));
#37784=CARTESIAN_POINT('Ctrl Pts',(57.169220106761,22.1399273566433,19.6193752459643));
#37785=CARTESIAN_POINT('Ctrl Pts',(57.2069398916903,22.068148645996,19.6151500929331));
#37786=CARTESIAN_POINT('Ctrl Pts',(57.2411494457619,21.9943885938192,19.610924939902));
#37787=CARTESIAN_POINT('Ctrl Pts',(57.2716388683287,21.9190250823009,19.6066997868708));
#37788=CARTESIAN_POINT('Ctrl Pts',(57.3022066169946,21.8434679649555,19.6024637795916));
#37789=CARTESIAN_POINT('Ctrl Pts',(57.3290348414209,21.7662995368335,19.5982277723124));
#37790=CARTESIAN_POINT('Ctrl Pts',(57.3519585611881,21.6879252695271,19.5939917650332));
#37791=CARTESIAN_POINT('Ctrl Pts',(57.3747824077128,21.6098924604258,19.5897742130391));
#37792=CARTESIAN_POINT('Ctrl Pts',(57.3937355614453,21.5306647441038,19.5855566610449));
#37793=CARTESIAN_POINT('Ctrl Pts',(57.4087041098994,21.4506603609743,19.5813391090508));
#37794=CARTESIAN_POINT('Ctrl Pts',(57.4236677160794,21.3706823934722,19.5771229495963));
#37795=CARTESIAN_POINT('Ctrl Pts',(57.4346492441949,21.2899287250452,19.5729067901419));
#37796=CARTESIAN_POINT('Ctrl Pts',(57.4415857344128,21.2088285217872,19.5686906306875));
#37797=CARTESIAN_POINT('Ctrl Pts',(57.4485220593482,21.1277302509827,19.5644745716956));
#37798=CARTESIAN_POINT('Ctrl Pts',(57.4514134995091,21.0462859250897,19.5602585127037));
#37799=CARTESIAN_POINT('Ctrl Pts',(57.450249025058,20.9649291402713,19.5560424537118));
#37800=CARTESIAN_POINT('Ctrl Pts',(57.4490750186396,20.8829063981885,19.5517918835833));
#37801=CARTESIAN_POINT('Ctrl Pts',(57.4437783814331,20.8009731168526,19.5475413134549));
#37802=CARTESIAN_POINT('Ctrl Pts',(57.4344013322171,20.7195710362687,19.5432907433264));
#37803=CARTESIAN_POINT('Ctrl Pts',(57.4250868943595,20.6387124843282,19.5390685546176));
#37804=CARTESIAN_POINT('Ctrl Pts',(57.411746506964,20.5583785140341,19.5348463659089));
#37805=CARTESIAN_POINT('Ctrl Pts',(57.3944731135562,20.4789925543175,19.5306241772001));
#37806=CARTESIAN_POINT('Ctrl Pts',(57.3770255533374,20.3988061497138,19.5263594163618));
#37807=CARTESIAN_POINT('Ctrl Pts',(57.3555653550877,20.3195874496795,19.5220946555235));
#37808=CARTESIAN_POINT('Ctrl Pts',(57.3302395361106,20.2417560060594,19.5178298946851));
#37809=CARTESIAN_POINT('Ctrl Pts',(57.3049137171336,20.1639245624393,19.5135651338468));
#37810=CARTESIAN_POINT('Ctrl Pts',(57.2757225093273,20.0874808024105,19.5093003730085));
#37811=CARTESIAN_POINT('Ctrl Pts',(57.242861423422,20.0128207430637,19.5050356121701));
#37812=CARTESIAN_POINT('Ctrl Pts',(57.2102587760063,19.9387478533871,19.5008043918652));
#37813=CARTESIAN_POINT('Ctrl Pts',(57.1739215540254,19.866152925154,19.4965731715603));
#37814=CARTESIAN_POINT('Ctrl Pts',(57.1340057970936,19.7954380431165,19.4923419512554));
#37815=CARTESIAN_POINT('Ctrl Pts',(57.0941472765634,19.7248245612703,19.4881167982242));
#37816=CARTESIAN_POINT('Ctrl Pts',(57.0507206389732,19.656086172909,19.4838916451931));
#37817=CARTESIAN_POINT('Ctrl Pts',(57.0039295815891,19.589604139955,19.4796664921619));
#37818=CARTESIAN_POINT('Ctrl Pts',(56.9570183198623,19.5229513173347,19.4754304848827));
#37819=CARTESIAN_POINT('Ctrl Pts',(56.9067255261239,19.4585668873638,19.4711944776035));
#37820=CARTESIAN_POINT('Ctrl Pts',(56.8533024359616,19.3968093279779,19.4669584703243));
#37821=CARTESIAN_POINT('Ctrl Pts',(56.8001120976083,19.3353208317184,19.4627409183301));
#37822=CARTESIAN_POINT('Ctrl Pts',(56.7438189817862,19.2764367236666,19.458523366336));
#37823=CARTESIAN_POINT('Ctrl Pts',(56.6847127430469,19.2204794962082,19.4543058143418));
#37824=CARTESIAN_POINT('Ctrl Pts',(56.6256260198431,19.1645407445533,19.4500896548874));
#37825=CARTESIAN_POINT('Ctrl Pts',(56.5637283556014,19.1115272737598,19.445873495433));
#37826=CARTESIAN_POINT('Ctrl Pts',(56.4993462126577,19.0617246881341,19.4416573359785));
#37827=CARTESIAN_POINT('Ctrl Pts',(56.4349656038099,19.0119232892029,19.4374412769866));
#37828=CARTESIAN_POINT('Ctrl Pts',(56.3681010023832,18.9653329069072,19.4332252179947));
#37829=CARTESIAN_POINT('Ctrl Pts',(56.2991107505924,18.9221979142143,19.4290091590028));
#37830=CARTESIAN_POINT('Ctrl Pts',(56.2295557695115,18.8787098340465,19.4247585888743));
#37831=CARTESIAN_POINT('Ctrl Pts',(56.1578405760753,18.8387342416609,19.4205080187459));
#37832=CARTESIAN_POINT('Ctrl Pts',(56.0843592278049,18.8024751844235,19.4162574486174));
#37833=CARTESIAN_POINT('Ctrl Pts',(56.0113685207717,18.7664582320076,19.4120352599086));
#37834=CARTESIAN_POINT('Ctrl Pts',(55.9366356280391,18.7341084644212,19.4078130711999));
#37835=CARTESIAN_POINT('Ctrl Pts',(55.8605667255813,18.7055773796394,19.4035908824911));
#37836=CARTESIAN_POINT('Ctrl Pts',(55.7837308239684,18.6767586172757,19.3993261216528));
#37837=CARTESIAN_POINT('Ctrl Pts',(55.7055322819995,18.6518361258678,19.3950613608145));
#37838=CARTESIAN_POINT('Ctrl Pts',(55.6264033379672,18.630913866449,19.3907965999761));
#37839=CARTESIAN_POINT('Ctrl Pts',(55.547274393935,18.6099916070302,19.3865318391378));
#37840=CARTESIAN_POINT('Ctrl Pts',(55.467215532509,18.5930696163763,19.3822670782995));
#37841=CARTESIAN_POINT('Ctrl Pts',(55.3866655114437,18.5801983485707,19.3780023174611));
#37842=CARTESIAN_POINT('Ctrl Pts',(55.3067489820969,18.5674283078219,19.3737710971562));
#37843=CARTESIAN_POINT('Ctrl Pts',(55.2260493203515,18.5585975716892,19.3695398768513));
#37844=CARTESIAN_POINT('Ctrl Pts',(55.1449889801249,18.5537930493022,19.3653086565463));
#37845=CARTESIAN_POINT('Ctrl Pts',(55.0640448747525,18.5489954162639,19.3610835035152));
#37846=CARTESIAN_POINT('Ctrl Pts',(54.9827415782641,18.548212558023,19.356858350484));
#37847=CARTESIAN_POINT('Ctrl Pts',(54.9015098895185,18.5514800494712,19.3526331974529));
#37848=CARTESIAN_POINT('Ctrl Pts',(54.8200695198348,18.5547559349734,19.3483971901737));
#37849=CARTESIAN_POINT('Ctrl Pts',(54.7387015933923,18.562103075311,19.3441611828945));
#37850=CARTESIAN_POINT('Ctrl Pts',(54.6578435414544,18.5735047480212,19.3399251756153));
#37851=CARTESIAN_POINT('Ctrl Pts',(54.5773377689859,18.5848567463315,19.3357076236211));
#37852=CARTESIAN_POINT('Ctrl Pts',(54.4973379019118,18.600227964179,19.331490071627));
#37853=CARTESIAN_POINT('Ctrl Pts',(54.4182719667645,18.6195498859779,19.3272725196328));
#37854=CARTESIAN_POINT('Ctrl Pts',(54.3392321373901,18.6388654281177,19.3230563601784));
#37855=CARTESIAN_POINT('Ctrl Pts',(54.2611260788537,18.6621289735071,19.3188402007239));
#37856=CARTESIAN_POINT('Ctrl Pts',(54.1843707810034,18.6892210778357,19.3146240412695));
#37857=CARTESIAN_POINT('Ctrl Pts',(54.1076173120765,18.7163125366142,19.3104079822776));
#37858=CARTESIAN_POINT('Ctrl Pts',(54.0322149778859,18.7472322171586,19.3061919232857));
#37859=CARTESIAN_POINT('Ctrl Pts',(53.9585634102166,18.7818115320243,19.3019758642938));
#37860=CARTESIAN_POINT('Ctrl Pts',(53.8843089574083,18.8166739006757,19.2977252941654));
#37861=CARTESIAN_POINT('Ctrl Pts',(53.8118345067648,18.8552559037357,19.2934747240369));
#37862=CARTESIAN_POINT('Ctrl Pts',(53.7415251726937,18.8973370790741,19.2892241539084));
#37863=CARTESIAN_POINT('Ctrl Pts',(53.6716853000502,18.9391372748114,19.2850019651997));
#37864=CARTESIAN_POINT('Ctrl Pts',(53.6039820746839,18.9843897442918,19.2807797764909));
#37865=CARTESIAN_POINT('Ctrl Pts',(53.5387630280351,19.0328353496052,19.2765575877821));
#37866=CARTESIAN_POINT('Ctrl Pts',(53.4728863808154,19.0817694296717,19.2722928269438));
#37867=CARTESIAN_POINT('Ctrl Pts',(53.4095446649128,19.1339610915591,19.2680280661055));
#37868=CARTESIAN_POINT('Ctrl Pts',(53.3490596011056,19.1891035233072,19.2637633052671));
#37869=CARTESIAN_POINT('Ctrl Pts',(53.2885745372984,19.2442459550554,19.2594985444288));
#37870=CARTESIAN_POINT('Ctrl Pts',(53.2309464192854,19.3023387693685,19.2552337835905));
#37871=CARTESIAN_POINT('Ctrl Pts',(53.1764555444078,19.3630406637674,19.2509690227521));
#37872=CARTESIAN_POINT('Ctrl Pts',(53.1229452308608,19.4226502297632,19.2467810061315));
#37873=CARTESIAN_POINT('Ctrl Pts',(53.0722501301212,19.4850099234974,19.2425929895108));
#37874=CARTESIAN_POINT('Ctrl Pts',(53.024669961604,19.5498201872146,19.2384049728901));
#37875=CARTESIAN_POINT('Ctrl Pts',(52.9771527445824,19.6145447029582,19.2342224972736));
#37876=CARTESIAN_POINT('Ctrl Pts',(52.9327425628976,19.6817129783031,19.230040021657));
#37877=CARTESIAN_POINT('Ctrl Pts',(52.8917010163663,19.7509901339024,19.2258575460405));
#37878=CARTESIAN_POINT('Ctrl Pts',(52.8507005749442,19.8201979050539,19.2216792593771));
#37879=CARTESIAN_POINT('Ctrl Pts',(52.8130623143615,19.8915099588894,19.2175009727138));
#37880=CARTESIAN_POINT('Ctrl Pts',(52.7790054375102,19.9645612507778,19.2133226860504));
#37881=CARTESIAN_POINT('Ctrl Pts',(52.7449717254275,20.03756285472,19.2091472413694));
#37882=CARTESIAN_POINT('Ctrl Pts',(52.7145147606302,20.1123009185737,19.2049717966884));
#37883=CARTESIAN_POINT('Ctrl Pts',(52.687807788734,20.1883859118023,19.2007963520074));
#37884=CARTESIAN_POINT('Ctrl Pts',(52.661103833147,20.2644623119242,19.1966213789048));
#37885=CARTESIAN_POINT('Ctrl Pts',(52.6381491984721,20.3418848955061,19.1924464058023));
#37886=CARTESIAN_POINT('Ctrl Pts',(52.6190684795368,20.4202454442916,19.1882714326997));
#37887=CARTESIAN_POINT('Ctrl Pts',(52.5999890703565,20.4986006141851,19.1840967461792));
#37888=CARTESIAN_POINT('Ctrl Pts',(52.5847831532995,20.5778931578053,19.1799220596587));
#37889=CARTESIAN_POINT('Ctrl Pts',(52.5735245816719,20.6577029152193,19.1757473731382));
#37890=CARTESIAN_POINT('Ctrl Pts',(52.5622586284001,20.7375649996291,19.1715699494987));
#37891=CARTESIAN_POINT('Ctrl Pts',(52.5549452432902,20.8179445027518,19.1673925258593));
#37892=CARTESIAN_POINT('Ctrl Pts',(52.551606480764,20.8984154295032,19.1632151022198));
#37893=CARTESIAN_POINT('Ctrl Pts',(52.5501711513523,20.9330097700845,19.1614192335506));
#37894=CARTESIAN_POINT('Ctrl Pts',(52.5494697276278,20.9676209861166,19.1596233648813));
#37895=CARTESIAN_POINT('Ctrl Pts',(52.5495010013221,21.002215282968,19.1578274962121));
#37896=CARTESIAN_POINT('',(52.5495000435359,20.9995380808101,18.3578274961844));
#37897=CARTESIAN_POINT('Ctrl Pts',(52.5495010013229,21.002215283885,19.1578274961645));
#37898=CARTESIAN_POINT('Ctrl Pts',(52.5495930447091,21.104031681907,19.1525419752588));
#37899=CARTESIAN_POINT('Ctrl Pts',(52.5560343398191,21.2055657086561,19.1472564543532));
#37900=CARTESIAN_POINT('Ctrl Pts',(52.5686979300326,21.3061380318942,19.1419709334475));
#37901=CARTESIAN_POINT('Ctrl Pts',(52.5816081917137,21.4086693827194,19.1365824569678));
#37902=CARTESIAN_POINT('Ctrl Pts',(52.6009854926653,21.5102013902044,19.1311939804882));
#37903=CARTESIAN_POINT('Ctrl Pts',(52.6266470571175,21.6100377517098,19.1258055040085));
#37904=CARTESIAN_POINT('Ctrl Pts',(52.6296152044612,21.6215853341559,19.1251822453534));
#37905=CARTESIAN_POINT('Ctrl Pts',(52.6326673731257,21.633110255002,19.1245589866982));
#37906=CARTESIAN_POINT('Ctrl Pts',(52.6358032394755,21.6446114546962,19.123935728043));
#37907=CARTESIAN_POINT('Ctrl Pts',(52.6570922200026,21.7226915732393,19.1197045077381));
#37908=CARTESIAN_POINT('Ctrl Pts',(52.6822932908291,21.7998623146875,19.1154732874331));
#37909=CARTESIAN_POINT('Ctrl Pts',(52.7113115953108,21.8757029383536,19.1112420671282));
#37910=CARTESIAN_POINT('Ctrl Pts',(52.7402882895748,21.9514348118734,19.107016914097));
#37911=CARTESIAN_POINT('Ctrl Pts',(52.7730711816813,22.0258399250851,19.1027917610659));
#37912=CARTESIAN_POINT('Ctrl Pts',(52.8095152018074,22.0985110827329,19.0985666080347));
#37913=CARTESIAN_POINT('Ctrl Pts',(52.8460528451539,22.1713689296591,19.0943306007555));
#37914=CARTESIAN_POINT('Ctrl Pts',(52.8862703208193,22.2424834469941,19.0900945934763));
#37915=CARTESIAN_POINT('Ctrl Pts',(52.9299721737715,22.3114629421527,19.0858585861971));
#37916=CARTESIAN_POINT('Ctrl Pts',(52.9734836280536,22.3801419099134,19.0816410342029));
#37917=CARTESIAN_POINT('Ctrl Pts',(53.0204489182305,22.4467040206718,19.0774234822088));
#37918=CARTESIAN_POINT('Ctrl Pts',(53.0706292706656,22.5107874896185,19.0732059302146));
#37919=CARTESIAN_POINT('Ctrl Pts',(53.1207930546899,22.5748497996615,19.0689897707602));
#37920=CARTESIAN_POINT('Ctrl Pts',(53.1741695064926,22.6364347273397,19.0647736113058));
#37921=CARTESIAN_POINT('Ctrl Pts',(53.2304779938119,22.6952115265111,19.0605574518514));
#37922=CARTESIAN_POINT('Ctrl Pts',(53.2867851394142,22.7539869251506,19.0563413928595));
#37923=CARTESIAN_POINT('Ctrl Pts',(53.3460238591996,22.8099539933655,19.0521253338676));
#37924=CARTESIAN_POINT('Ctrl Pts',(53.4078758936407,22.8628180479987,19.0479092748757));
#37925=CARTESIAN_POINT('Ctrl Pts',(53.4702342265021,22.9161148286949,19.0436587047472));
#37926=CARTESIAN_POINT('Ctrl Pts',(53.5352485005538,22.9662572371502,19.0394081346188));
#37927=CARTESIAN_POINT('Ctrl Pts',(53.6025591697091,23.012985190168,19.0351575644903));
#37928=CARTESIAN_POINT('Ctrl Pts',(53.6694203997786,23.0594011366534,19.0309353757816));
#37929=CARTESIAN_POINT('Ctrl Pts',(53.7385470206645,23.102447890352,19.0267131870728));
#37930=CARTESIAN_POINT('Ctrl Pts',(53.8095597292185,23.1419155472851,19.0224909983641));
#37931=CARTESIAN_POINT('Ctrl Pts',(53.8812884555628,23.1817811547412,19.0182262375258));
#37932=CARTESIAN_POINT('Ctrl Pts',(53.9549410823697,23.2179948691113,19.0139614766875));
#37933=CARTESIAN_POINT('Ctrl Pts',(54.0301055002312,23.2503899460578,19.0096967158492));
#37934=CARTESIAN_POINT('Ctrl Pts',(54.1052699180927,23.2827850230044,19.0054319550108));
#37935=CARTESIAN_POINT('Ctrl Pts',(54.1819456531084,23.3113613544749,19.0011671941725));
#37936=CARTESIAN_POINT('Ctrl Pts',(54.2597062346072,23.3360041504502,18.9969024333342));
#37937=CARTESIAN_POINT('Ctrl Pts',(54.3368552621458,23.3604531412972,18.9926712130293));
#37938=CARTESIAN_POINT('Ctrl Pts',(54.4153614196718,23.3811219713792,18.9884399927244));
#37939=CARTESIAN_POINT('Ctrl Pts',(54.4948197526338,23.3978622078157,18.9842087724194));
#37940=CARTESIAN_POINT('Ctrl Pts',(54.5741641479076,23.4145784399249,18.9799836193883));
#37941=CARTESIAN_POINT('Ctrl Pts',(54.6544575558271,23.4273771715644,18.9757584663571));
#37942=CARTESIAN_POINT('Ctrl Pts',(54.7352791765095,23.4361595053712,18.971533313326));
#37943=CARTESIAN_POINT('Ctrl Pts',(54.8163084246817,23.44496440064,18.9672973060468));
#37944=CARTESIAN_POINT('Ctrl Pts',(54.8978681511069,23.4497320992601,18.9630612987676));
#37945=CARTESIAN_POINT('Ctrl Pts',(54.9795232618338,23.4504144451896,18.9588252914884));
#37946=CARTESIAN_POINT('Ctrl Pts',(55.0608226204942,23.4510938182988,18.9546077394942));
#37947=CARTESIAN_POINT('Ctrl Pts',(55.1422160662684,23.4477233502293,18.9503901875));
#37948=CARTESIAN_POINT('Ctrl Pts',(55.2232701464828,23.4403074994126,18.9461726355059));
#37949=CARTESIAN_POINT('Ctrl Pts',(55.3042974644839,23.4328940971412,18.9419564760514));
#37950=CARTESIAN_POINT('Ctrl Pts',(55.3849851768177,23.4214380069487,18.937740316597));
#37951=CARTESIAN_POINT('Ctrl Pts',(55.4649032139365,23.4059956882072,18.9335241571426));
#37952=CARTESIAN_POINT('Ctrl Pts',(55.5448193467704,23.3905537374248,18.9293080981507));
#37953=CARTESIAN_POINT('Ctrl Pts',(55.6239653845857,23.371125836238,18.9250920391587));
#37954=CARTESIAN_POINT('Ctrl Pts',(55.7019211569046,23.3478196139162,18.9208759801668));
#37955=CARTESIAN_POINT('Ctrl Pts',(55.7805150470274,23.3243226152739,18.9166254100384));
#37956=CARTESIAN_POINT('Ctrl Pts',(55.8578986313298,23.2968836313879,18.9123748399099));
#37957=CARTESIAN_POINT('Ctrl Pts',(55.9336584249708,23.2656637428094,18.9081242697814));
#37958=CARTESIAN_POINT('Ctrl Pts',(56.0089123640002,23.2346523120929,18.9039020810726));
#37959=CARTESIAN_POINT('Ctrl Pts',(56.0825637324469,23.1999105699802,18.8996798923639));
#37960=CARTESIAN_POINT('Ctrl Pts',(56.1542304951133,23.1616434058721,18.8954577036551));
#37961=CARTESIAN_POINT('Ctrl Pts',(56.2266198703669,23.1229903957536,18.8911929428168));
#37962=CARTESIAN_POINT('Ctrl Pts',(56.2969839767197,23.0807407202377,18.8869281819785));
#37963=CARTESIAN_POINT('Ctrl Pts',(56.3649592549612,23.0351502358047,18.8826634211401));
#37964=CARTESIAN_POINT('Ctrl Pts',(56.4329345332027,22.9895597513717,18.8783986603018));
#37965=CARTESIAN_POINT('Ctrl Pts',(56.4985206355842,22.9406287976213,18.8741338994635));
#37966=CARTESIAN_POINT('Ctrl Pts',(56.5613898697605,22.8886534686409,18.8698691386251));
#37967=CARTESIAN_POINT('Ctrl Pts',(56.6237646641009,22.837086903557,18.8656379183202));
#37968=CARTESIAN_POINT('Ctrl Pts',(56.6836990991716,22.7823303441399,18.8614066980153));
#37969=CARTESIAN_POINT('Ctrl Pts',(56.7408488812152,22.7246435639783,18.8571754777103));
#37970=CARTESIAN_POINT('Ctrl Pts',(56.7979167144712,22.667039502622,18.8529503246792));
#37971=CARTESIAN_POINT('Ctrl Pts',(56.8522075006449,22.6065138929718,18.848725171648));
#37972=CARTESIAN_POINT('Ctrl Pts',(56.9034099757883,22.5433666816637,18.8445000186169));
#37973=CARTESIAN_POINT('Ctrl Pts',(56.9547439880291,22.4800572477118,18.8402640113377));
#37974=CARTESIAN_POINT('Ctrl Pts',(57.0029734417368,22.4141130309847,18.8360280040585));
#37975=CARTESIAN_POINT('Ctrl Pts',(57.0478219570602,22.3458735015529,18.8317919967793));
#37976=CARTESIAN_POINT('Ctrl Pts',(57.0924750779757,22.2779312756628,18.8275744447852));
#37977=CARTESIAN_POINT('Ctrl Pts',(57.1337763951717,22.2077140821282,18.823356892791));
#37978=CARTESIAN_POINT('Ctrl Pts',(57.1714946272751,22.1355885406763,18.8191393407969));
#37979=CARTESIAN_POINT('Ctrl Pts',(57.2092004056763,22.0634868134374,18.8149231813424));
#37980=CARTESIAN_POINT('Ctrl Pts',(57.2433252330817,21.9894784012216,18.810707021888));
#37981=CARTESIAN_POINT('Ctrl Pts',(57.2736833555524,21.9139552771795,18.8064908624336));
#37982=CARTESIAN_POINT('Ctrl Pts',(57.3040407546505,21.8384339527004,18.8022748034417));
#37983=CARTESIAN_POINT('Ctrl Pts',(57.3306314548942,21.7613984199449,18.7980587444498));
#37984=CARTESIAN_POINT('Ctrl Pts',(57.3533180645943,21.6832600799506,18.7938426854579));
#37985=CARTESIAN_POINT('Ctrl Pts',(57.3761903786898,21.6044821277192,18.7895921153294));
#37986=CARTESIAN_POINT('Ctrl Pts',(57.3950942431044,21.5245836867684,18.785341545201));
#37987=CARTESIAN_POINT('Ctrl Pts',(57.4099408029048,21.4439995230792,18.7810909750725));
#37988=CARTESIAN_POINT('Ctrl Pts',(57.4246882309576,21.3639534267324,18.7768687863638));
#37989=CARTESIAN_POINT('Ctrl Pts',(57.4354323706634,21.2832312105769,18.772646597655));
#37990=CARTESIAN_POINT('Ctrl Pts',(57.4421382295174,21.2022649696059,18.7684244089463));
#37991=CARTESIAN_POINT('Ctrl Pts',(57.4489117032299,21.1204823498463,18.7641596481079));
#37992=CARTESIAN_POINT('Ctrl Pts',(57.4515649864324,21.0384512421352,18.7598948872696));
#37993=CARTESIAN_POINT('Ctrl Pts',(57.4501159290465,20.9566158527516,18.7556301264313));
#37994=CARTESIAN_POINT('Ctrl Pts',(57.4486668716607,20.874780463368,18.7513653655929));
#37995=CARTESIAN_POINT('Ctrl Pts',(57.4431155704733,20.793141268641,18.7471006047546));
#37996=CARTESIAN_POINT('Ctrl Pts',(57.4335331322646,20.7121341559499,18.7428358439163));
#37997=CARTESIAN_POINT('Ctrl Pts',(57.4240260558641,20.631764129809,18.7386046236113));
#37998=CARTESIAN_POINT('Ctrl Pts',(57.4105154173039,20.5517148952583,18.7343734033064));
#37999=CARTESIAN_POINT('Ctrl Pts',(57.3930328039482,20.4724165950035,18.7301421830015));
#38000=CARTESIAN_POINT('Ctrl Pts',(57.3755752594365,20.3932320029612,18.7259170299703));
#38001=CARTESIAN_POINT('Ctrl Pts',(57.3541571511383,20.3147966568229,18.7216918769392));
#38002=CARTESIAN_POINT('Ctrl Pts',(57.3288617307172,20.2375347291836,18.717466723908));
#38003=CARTESIAN_POINT('Ctrl Pts',(57.3035013273793,20.1600743187627,18.7132307166288));
#38004=CARTESIAN_POINT('Ctrl Pts',(57.2742437269267,20.0837938314776,18.7089947093496));
#38005=CARTESIAN_POINT('Ctrl Pts',(57.2412243049294,20.0091095595407,18.7047587020704));
#38006=CARTESIAN_POINT('Ctrl Pts',(57.2083487407692,19.9347506693691,18.7005411500763));
#38007=CARTESIAN_POINT('Ctrl Pts',(57.171744247155,19.8619745461055,18.6963235980821));
#38008=CARTESIAN_POINT('Ctrl Pts',(57.1315934651387,19.7911743097626,18.6921060460879));
#38009=CARTESIAN_POINT('Ctrl Pts',(57.0914559399972,19.7203974500471,18.6878898866335));
#38010=CARTESIAN_POINT('Ctrl Pts',(57.0477746808686,19.651595585791,18.6836737271791));
#38011=CARTESIAN_POINT('Ctrl Pts',(57.0007783176169,19.5851373304261,18.6794575677246));
#38012=CARTESIAN_POINT('Ctrl Pts',(56.9537830741934,19.5186806586267,18.6752415087327));
#38013=CARTESIAN_POINT('Ctrl Pts',(56.903473153044,19.4545678636454,18.6710254497408));
#38014=CARTESIAN_POINT('Ctrl Pts',(56.8501197310983,19.3931374574654,18.6668093907489));
#38015=CARTESIAN_POINT('Ctrl Pts',(56.7963295773054,19.3312042041617,18.6625588206204));
#38016=CARTESIAN_POINT('Ctrl Pts',(56.7394461691812,19.271997829198,18.658308250492));
#38017=CARTESIAN_POINT('Ctrl Pts',(56.679786633396,19.2158287312413,18.6540576803635));
#38018=CARTESIAN_POINT('Ctrl Pts',(56.6205254494258,19.160034679148,18.6498354916547));
#38019=CARTESIAN_POINT('Ctrl Pts',(56.5585254953154,19.1072377246015,18.645613302946));
#38020=CARTESIAN_POINT('Ctrl Pts',(56.4941308588617,19.0577015608828,18.6413911142372));
#38021=CARTESIAN_POINT('Ctrl Pts',(56.4290869343264,19.0076659263622,18.6371263533989));
#38022=CARTESIAN_POINT('Ctrl Pts',(56.3616001641577,18.9609574860517,18.6328615925606));
#38023=CARTESIAN_POINT('Ctrl Pts',(56.2920534648009,18.9178021001605,18.6285968317222));
#38024=CARTESIAN_POINT('Ctrl Pts',(56.2225067654441,18.8746467142693,18.6243320708839));
#38025=CARTESIAN_POINT('Ctrl Pts',(56.1509005896076,18.8350445597497,18.6200673100455));
#38026=CARTESIAN_POINT('Ctrl Pts',(56.0776397409345,18.7991722378254,18.6158025492072));
#38027=CARTESIAN_POINT('Ctrl Pts',(56.0049550577336,18.7635820364835,18.6115713289023));
#38028=CARTESIAN_POINT('Ctrl Pts',(55.9303690961449,18.7315297098856,18.6073401085974));
#38029=CARTESIAN_POINT('Ctrl Pts',(55.8542604046432,18.7032219499789,18.6031088882924));
#38030=CARTESIAN_POINT('Ctrl Pts',(55.7782608476783,18.6749547814186,18.5988837352613));
#38031=CARTESIAN_POINT('Ctrl Pts',(55.7007433294521,18.6504216761331,18.5946585822301));
#38032=CARTESIAN_POINT('Ctrl Pts',(55.6221093956525,18.6297826787738,18.590433429199));
#38033=CARTESIAN_POINT('Ctrl Pts',(55.5432734544425,18.609090660661,18.5861974219198));
#38034=CARTESIAN_POINT('Ctrl Pts',(55.4633157810082,18.592312985504,18.5819614146406));
#38035=CARTESIAN_POINT('Ctrl Pts',(55.3826595623816,18.5795616286883,18.5777254073614));
#38036=CARTESIAN_POINT('Ctrl Pts',(55.3023547438841,18.566865826528,18.5735078553672));
#38037=CARTESIAN_POINT('Ctrl Pts',(55.2213579151492,18.5581614135731,18.5692903033731));
#38038=CARTESIAN_POINT('Ctrl Pts',(55.1400984214831,18.5535080866069,18.5650727513789));
#38039=CARTESIAN_POINT('Ctrl Pts',(55.0588657578531,18.5488562960634,18.5608565919245));
#38040=CARTESIAN_POINT('Ctrl Pts',(54.9773710653145,18.548252961829,18.55664043247));
#38041=CARTESIAN_POINT('Ctrl Pts',(54.8960480340157,18.5517058512572,18.5524242730156));
#38042=CARTESIAN_POINT('Ctrl Pts',(54.81472694048,18.5551586584101,18.5482082140237));
#38043=CARTESIAN_POINT('Ctrl Pts',(54.7335779645077,18.5626674762272,18.5439921550318));
#38044=CARTESIAN_POINT('Ctrl Pts',(54.6530325738938,18.5741880008498,18.5397760960399));
#38045=CARTESIAN_POINT('Ctrl Pts',(54.5718278677954,18.5858028283272,18.5355255259115));
#38046=CARTESIAN_POINT('Ctrl Pts',(54.4912371512862,18.6014952904895,18.531274955783));
#38047=CARTESIAN_POINT('Ctrl Pts',(54.4116931853111,18.6211672312265,18.5270243856545));
#38048=CARTESIAN_POINT('Ctrl Pts',(54.3326803411896,18.6407078207353,18.5228021969458));
#38049=CARTESIAN_POINT('Ctrl Pts',(54.254700743462,18.6641747135276,18.518580008237));
#38050=CARTESIAN_POINT('Ctrl Pts',(54.178162528468,18.6914217751209,18.5143578195283));
#38051=CARTESIAN_POINT('Ctrl Pts',(54.1008525822625,18.718943567551,18.5100930586899));
#38052=CARTESIAN_POINT('Ctrl Pts',(54.0250136980734,18.7503220026461,18.5058282978516));
#38053=CARTESIAN_POINT('Ctrl Pts',(53.9510432772957,18.7853578068019,18.5015635370133));
#38054=CARTESIAN_POINT('Ctrl Pts',(53.877072856518,18.8203936109576,18.4972987761749));
#38055=CARTESIAN_POINT('Ctrl Pts',(53.8049712933018,18.8590864997399,18.4930340153366));
#38056=CARTESIAN_POINT('Ctrl Pts',(53.7351064676168,18.9011920998493,18.4887692544982));
#38057=CARTESIAN_POINT('Ctrl Pts',(53.665791099125,18.9429665572895,18.4845380341933));
#38058=CARTESIAN_POINT('Ctrl Pts',(53.5984174634729,18.9882568490248,18.4803068138884));
#38059=CARTESIAN_POINT('Ctrl Pts',(53.533364487795,19.0368569781243,18.4760755935835));
#38060=CARTESIAN_POINT('Ctrl Pts',(53.4684047935311,19.0853874180402,18.4718504405523));
#38061=CARTESIAN_POINT('Ctrl Pts',(53.4057595195666,19.1372179933486,18.4676252875211));
#38062=CARTESIAN_POINT('Ctrl Pts',(53.3457808679188,19.1920980908643,18.46340013449));
#38063=CARTESIAN_POINT('Ctrl Pts',(53.2856481335295,19.2471191731412,18.4591641272108));
#38064=CARTESIAN_POINT('Ctrl Pts',(53.2281961408405,19.3052052167382,18.4549281199316));
#38065=CARTESIAN_POINT('Ctrl Pts',(53.1737484367813,19.3660613604418,18.4506921126524));
#38066=CARTESIAN_POINT('Ctrl Pts',(53.1195379485322,19.4266523682746,18.4464745606582));
#38067=CARTESIAN_POINT('Ctrl Pts',(53.0683059436126,19.4899890459734,18.4422570086641));
#38068=CARTESIAN_POINT('Ctrl Pts',(53.0203353817722,19.5557430113249,18.4380394566699));
#38069=CARTESIAN_POINT('Ctrl Pts',(52.97238065872,19.6214752662129,18.4338232972155));
#38070=CARTESIAN_POINT('Ctrl Pts',(52.9276855140624,19.6896228484752,18.4296071377611));
#38071=CARTESIAN_POINT('Ctrl Pts',(52.8864916304736,19.7598255679374,18.4253909783066));
#38072=CARTESIAN_POINT('Ctrl Pts',(52.8452987284515,19.8300266146111,18.4211749193147));
#38073=CARTESIAN_POINT('Ctrl Pts',(52.8076071559581,19.9022822995731,18.4169588603229));
#38074=CARTESIAN_POINT('Ctrl Pts',(52.7736136385845,19.9762060658009,18.412742801331));
#38075=CARTESIAN_POINT('Ctrl Pts',(52.7393418625519,20.0507349452868,18.4084922312025));
#38076=CARTESIAN_POINT('Ctrl Pts',(52.7088291779766,20.1269589115716,18.404241661074));
#38077=CARTESIAN_POINT('Ctrl Pts',(52.6822277630573,20.2044611212155,18.3999910909455));
#38078=CARTESIAN_POINT('Ctrl Pts',(52.655803968057,20.2814458419873,18.3957689022368));
#38079=CARTESIAN_POINT('Ctrl Pts',(52.6332394407126,20.3596913199703,18.391546713528));
#38080=CARTESIAN_POINT('Ctrl Pts',(52.6146326940984,20.4387753872683,18.3873245248193));
#38081=CARTESIAN_POINT('Ctrl Pts',(52.5958383365359,20.5186568554863,18.383059763981));
#38082=CARTESIAN_POINT('Ctrl Pts',(52.5810821085045,20.5993934412349,18.3787950031426));
#38083=CARTESIAN_POINT('Ctrl Pts',(52.5704120529877,20.6805431833055,18.3745302423043));
#38084=CARTESIAN_POINT('Ctrl Pts',(52.559741997471,20.7616929253762,18.370265481466));
#38085=CARTESIAN_POINT('Ctrl Pts',(52.5531580891939,20.8432553383636,18.3660007206276));
#38086=CARTESIAN_POINT('Ctrl Pts',(52.5506544696196,20.9247888119655,18.3617359597893));
#38087=CARTESIAN_POINT('Ctrl Pts',(52.5498896509667,20.9496960790609,18.3604331385969));
#38088=CARTESIAN_POINT('Ctrl Pts',(52.549504741528,20.974615071646,18.3591303174045));
#38089=CARTESIAN_POINT('Ctrl Pts',(52.549500043536,20.9995380802805,18.3578274962121));
#38090=CARTESIAN_POINT('',(52.5495007596431,20.9980704896796,17.5578274962389));
#38091=CARTESIAN_POINT('Ctrl Pts',(52.5495000435359,20.9995380808101,18.3578274961844));
#38092=CARTESIAN_POINT('Ctrl Pts',(52.5494848634307,21.0800691517973,18.3536178284245));
#38093=CARTESIAN_POINT('Ctrl Pts',(52.5534437136658,21.1607581475281,18.3494081606647));
#38094=CARTESIAN_POINT('Ctrl Pts',(52.5613972293637,21.2411778950177,18.3451984929048));
#38095=CARTESIAN_POINT('Ctrl Pts',(52.5693394372043,21.3214833062722,18.3409948102117));
#38096=CARTESIAN_POINT('Ctrl Pts',(52.5812649878903,21.4015197655146,18.3367911275187));
#38097=CARTESIAN_POINT('Ctrl Pts',(52.5971425057765,21.4808597638128,18.3325874448257));
#38098=CARTESIAN_POINT('Ctrl Pts',(52.6130021184754,21.5601102898432,18.3283885026548));
#38099=CARTESIAN_POINT('Ctrl Pts',(52.6328047517819,21.6386654567809,18.324189560484));
#38100=CARTESIAN_POINT('Ctrl Pts',(52.6564673664993,21.716104074641,18.3199906183131));
#38101=CARTESIAN_POINT('Ctrl Pts',(52.680115551085,21.7934954682415,18.315794236776));
#38102=CARTESIAN_POINT('Ctrl Pts',(52.7076189086256,21.8697712155354,18.3115978552389));
#38103=CARTESIAN_POINT('Ctrl Pts',(52.7388438626034,21.944522721968,18.3074014737017));
#38104=CARTESIAN_POINT('Ctrl Pts',(52.7700595918591,22.0192521447211,18.3032063318927));
#38105=CARTESIAN_POINT('Ctrl Pts',(52.8049945533822,22.0924577871544,18.2990111900837));
#38106=CARTESIAN_POINT('Ctrl Pts',(52.8434666194345,22.163749985395,18.2948160482747));
#38107=CARTESIAN_POINT('Ctrl Pts',(52.8819394153157,22.235043536074,18.2906208268824));
#38108=CARTESIAN_POINT('Ctrl Pts',(52.9239492241089,22.3044231575566,18.28642560549));
#38109=CARTESIAN_POINT('Ctrl Pts',(52.969268164694,22.3715241387138,18.2822303840977));
#38110=CARTESIAN_POINT('Ctrl Pts',(53.0146326435224,22.4386925455603,18.2780309471829));
#38111=CARTESIAN_POINT('Ctrl Pts',(53.0633126302393,22.5035773495072,18.2738315102681));
#38112=CARTESIAN_POINT('Ctrl Pts',(53.1150374936316,22.5658437340888,18.2696320733533));
#38113=CARTESIAN_POINT('Ctrl Pts',(53.1667890131589,22.6281422073227,18.2654304722808));
#38114=CARTESIAN_POINT('Ctrl Pts',(53.2215882150173,22.6878192283477,18.2612288712084));
#38115=CARTESIAN_POINT('Ctrl Pts',(53.2791265630674,22.7445758407303,18.2570272701359));
#38116=CARTESIAN_POINT('Ctrl Pts',(53.3367653741261,22.8014315511968,18.2528183329911));
#38117=CARTESIAN_POINT('Ctrl Pts',(53.397152531953,22.8553563559036,18.2486093958463));
#38118=CARTESIAN_POINT('Ctrl Pts',(53.4599455767472,22.9060909273746,18.2444004587015));
#38119=CARTESIAN_POINT('Ctrl Pts',(53.508172636479,22.9450566952683,18.2411678608278));
#38120=CARTESIAN_POINT('Ctrl Pts',(53.5578181551207,22.9821414420203,18.237935262954));
#38121=CARTESIAN_POINT('Ctrl Pts',(53.6087162665811,23.0172456030746,18.2347026650802));
#38122=CARTESIAN_POINT('Ctrl Pts',(53.6753379532564,23.0631942316516,18.2304714447753));
#38123=CARTESIAN_POINT('Ctrl Pts',(53.7443632493421,23.1059250847526,18.2262402244704));
#38124=CARTESIAN_POINT('Ctrl Pts',(53.8154483383668,23.1451777574182,18.2220090041654));
#38125=CARTESIAN_POINT('Ctrl Pts',(53.8864314963489,23.1843741444985,18.2177838511343));
#38126=CARTESIAN_POINT('Ctrl Pts',(53.9594681776402,23.2201020337843,18.2135586981031));
#38127=CARTESIAN_POINT('Ctrl Pts',(54.0341849224833,23.252143753414,18.209333545072));
#38128=CARTESIAN_POINT('Ctrl Pts',(54.1090936116363,23.2842677869315,18.2050975377928));
#38129=CARTESIAN_POINT('Ctrl Pts',(54.1856906152162,23.312686424606,18.2008615305136));
#38130=CARTESIAN_POINT('Ctrl Pts',(54.2635739608335,23.3372263345336,18.1966255232344));
#38131=CARTESIAN_POINT('Ctrl Pts',(54.3411179870755,23.3616593298592,18.1924079712402));
#38132=CARTESIAN_POINT('Ctrl Pts',(54.419936726365,23.3822471759544,18.1881904192461));
#38133=CARTESIAN_POINT('Ctrl Pts',(54.4996143839329,23.3988673338126,18.1839728672519));
#38134=CARTESIAN_POINT('Ctrl Pts',(54.5792657337508,23.4154820040728,18.1797567077975));
#38135=CARTESIAN_POINT('Ctrl Pts',(54.6597749838983,23.428131492791,18.1755405483431));
#38136=CARTESIAN_POINT('Ctrl Pts',(54.7407143623583,23.4367439767265,18.1713243888886));
#38137=CARTESIAN_POINT('Ctrl Pts',(54.8216518121969,23.4453562554439,18.1671083298967));
#38138=CARTESIAN_POINT('Ctrl Pts',(54.9030189075409,23.4499316725456,18.1628922709049));
#38139=CARTESIAN_POINT('Ctrl Pts',(54.9843823731307,23.4504502320453,18.158676211913));
#38140=CARTESIAN_POINT('Ctrl Pts',(55.0664118506713,23.4509730362858,18.1544256417845));
#38141=CARTESIAN_POINT('Ctrl Pts',(55.1484371591545,23.4473722413147,18.150175071656));
#38142=CARTESIAN_POINT('Ctrl Pts',(55.2300157798258,23.4396809199219,18.1459245015275));
#38143=CARTESIAN_POINT('Ctrl Pts',(55.3110496930804,23.4320409541389,18.1417023128188));
#38144=CARTESIAN_POINT('Ctrl Pts',(55.3916424097103,23.4203650496643,18.13748012411));
#38145=CARTESIAN_POINT('Ctrl Pts',(55.4713686689262,23.4047373719296,18.1332579354013));
#38146=CARTESIAN_POINT('Ctrl Pts',(55.5518988042531,23.3889521210574,18.1289931745629));
#38147=CARTESIAN_POINT('Ctrl Pts',(55.6315444394973,23.3691350745922,18.1247284137246));
#38148=CARTESIAN_POINT('Ctrl Pts',(55.7098830716639,23.345424540369,18.1204636528863));
#38149=CARTESIAN_POINT('Ctrl Pts',(55.7882217038304,23.3217140061458,18.1161988920479));
#38150=CARTESIAN_POINT('Ctrl Pts',(55.8652529010369,23.2941102071775,18.1119341312096));
#38151=CARTESIAN_POINT('Ctrl Pts',(55.9405766869688,23.2628004211443,18.1076693703713));
#38152=CARTESIAN_POINT('Ctrl Pts',(56.0153080833027,23.2317368732859,18.1034381500663));
#38153=CARTESIAN_POINT('Ctrl Pts',(56.088639080374,23.196908979652,18.0992069297614));
#38154=CARTESIAN_POINT('Ctrl Pts',(56.1601644519263,23.1584644297478,18.0949757094565));
#38155=CARTESIAN_POINT('Ctrl Pts',(56.2315872611019,23.1200750066374,18.0907505564253));
#38156=CARTESIAN_POINT('Ctrl Pts',(56.3012091809258,23.0780794453609,18.0865254033942));
#38157=CARTESIAN_POINT('Ctrl Pts',(56.3686448177645,23.0326735135792,18.082300250363));
#38158=CARTESIAN_POINT('Ctrl Pts',(56.4362536940395,22.9871509357867,18.0780642430838));
#38159=CARTESIAN_POINT('Ctrl Pts',(56.5016646066119,22.9382006299537,18.0738282358047));
#38160=CARTESIAN_POINT('Ctrl Pts',(56.5645139576775,22.886066363157,18.0695922285255));
#38161=CARTESIAN_POINT('Ctrl Pts',(56.6270894889377,22.8341592330697,18.0653746765313));
#38162=CARTESIAN_POINT('Ctrl Pts',(56.6871253670562,22.7790961201122,18.0611571245371));
#38163=CARTESIAN_POINT('Ctrl Pts',(56.7442931774216,22.7211599464316,18.056939572543));
#38164=CARTESIAN_POINT('Ctrl Pts',(56.8014421122767,22.6632429019575,18.0527234130886));
#38165=CARTESIAN_POINT('Ctrl Pts',(56.8557245336385,22.6024550112615,18.0485072536341));
#38166=CARTESIAN_POINT('Ctrl Pts',(56.9068481457506,22.539116759394,18.0442910941797));
#38167=CARTESIAN_POINT('Ctrl Pts',(56.9579705396906,22.4757800167487,18.0400750351878));
#38168=CARTESIAN_POINT('Ctrl Pts',(57.0059339828864,22.4098933962318,18.0358589761959));
#38169=CARTESIAN_POINT('Ctrl Pts',(57.050486742696,22.3418101087813,18.031642917204));
#38170=CARTESIAN_POINT('Ctrl Pts',(57.0954041953105,22.2731695161231,18.0273923470756));
#38171=CARTESIAN_POINT('Ctrl Pts',(57.1368545934555,22.2022965209147,18.0231417769471));
#38172=CARTESIAN_POINT('Ctrl Pts',(57.1746257827272,22.1295808758553,18.0188912068186));
#38173=CARTESIAN_POINT('Ctrl Pts',(57.2121447705427,22.0573507593676,18.0146690181099));
#38174=CARTESIAN_POINT('Ctrl Pts',(57.2460333934679,21.9833029777984,18.0104468294011));
#38175=CARTESIAN_POINT('Ctrl Pts',(57.2761317845893,21.9078404866398,18.0062246406924));
#38176=CARTESIAN_POINT('Ctrl Pts',(57.3065336563686,21.8316171107425,18.001959879854));
#38177=CARTESIAN_POINT('Ctrl Pts',(57.3330682756203,21.753950795488,17.9976951190157));
#38178=CARTESIAN_POINT('Ctrl Pts',(57.3556227631297,21.6752715363655,17.9934303581774));
#38179=CARTESIAN_POINT('Ctrl Pts',(57.378177250639,21.596592277243,17.989165597339));
#38180=CARTESIAN_POINT('Ctrl Pts',(57.3967515596131,21.5169005580579,17.9849008365007));
#38181=CARTESIAN_POINT('Ctrl Pts',(57.4112861714913,21.4366339991052,17.9806360756623));
#38182=CARTESIAN_POINT('Ctrl Pts',(57.4257064748177,21.3569987025619,17.9764048553574));
#38183=CARTESIAN_POINT('Ctrl Pts',(57.4362045146124,21.2764989605317,17.9721736350525));
#38184=CARTESIAN_POINT('Ctrl Pts',(57.4426846622965,21.1955553389236,17.9679424147476));
#38185=CARTESIAN_POINT('Ctrl Pts',(57.4491555179023,21.1147277848037,17.9637172617164));
#38186=CARTESIAN_POINT('Ctrl Pts',(57.4516198871339,21.0334580747564,17.9594921086853));
#38187=CARTESIAN_POINT('Ctrl Pts',(57.4500332920609,20.9521761796451,17.9552669556541));
#38188=CARTESIAN_POINT('Ctrl Pts',(57.448442621089,20.8706854746175,17.9510309483749));
#38189=CARTESIAN_POINT('Ctrl Pts',(57.4427800678572,20.7891829874432,17.9467949410957));
#38190=CARTESIAN_POINT('Ctrl Pts',(57.4330533034165,20.7081064016906,17.9425589338165));
#38191=CARTESIAN_POINT('Ctrl Pts',(57.4233689161953,20.6273830475076,17.9383413818223));
#38192=CARTESIAN_POINT('Ctrl Pts',(57.409655705143,20.5470823568963,17.9341238298282));
#38193=CARTESIAN_POINT('Ctrl Pts',(57.391973317881,20.4676336819958,17.929906277834));
#38194=CARTESIAN_POINT('Ctrl Pts',(57.374296768941,20.3882112392403,17.9256901183796));
#38195=CARTESIAN_POINT('Ctrl Pts',(57.3526537472474,20.3096407070026,17.9214739589252));
#38196=CARTESIAN_POINT('Ctrl Pts',(57.3271550465332,20.2323414565087,17.9172577994707));
#38197=CARTESIAN_POINT('Ctrl Pts',(57.3016569534014,20.1550440478995,17.9130417404788));
#38198=CARTESIAN_POINT('Ctrl Pts',(57.2723035106134,20.0790183019785,17.908825681487));
#38199=CARTESIAN_POINT('Ctrl Pts',(57.2392550035574,20.0046672520996,17.9046096224951));
#38200=CARTESIAN_POINT('Ctrl Pts',(57.2059359733557,19.9297075913728,17.9003590523666));
#38201=CARTESIAN_POINT('Ctrl Pts',(57.1688612869247,19.8564506150345,17.8961084822381));
#38202=CARTESIAN_POINT('Ctrl Pts',(57.1282433935176,19.7852859151436,17.8918579121096));
#38203=CARTESIAN_POINT('Ctrl Pts',(57.0878967092534,19.7145963880308,17.8876357234009));
#38204=CARTESIAN_POINT('Ctrl Pts',(57.0440542953745,19.6459716442108,17.8834135346921));
#38205=CARTESIAN_POINT('Ctrl Pts',(56.9969680460069,19.5797645007861,17.8791913459834));
#38206=CARTESIAN_POINT('Ctrl Pts',(56.9494070282081,19.5128897938574,17.874926585145));
#38207=CARTESIAN_POINT('Ctrl Pts',(56.8985366929528,19.4484820960638,17.8706618243067));
#38208=CARTESIAN_POINT('Ctrl Pts',(56.8446571320856,19.3868694054585,17.8663970634683));
#38209=CARTESIAN_POINT('Ctrl Pts',(56.7907775712184,19.3252567148533,17.86213230263));
#38210=CARTESIAN_POINT('Ctrl Pts',(56.7338891658774,19.266439333083,17.8578675417917));
#38211=CARTESIAN_POINT('Ctrl Pts',(56.6743273478505,19.2107045570281,17.8536027809533));
#38212=CARTESIAN_POINT('Ctrl Pts',(56.6152339582357,19.1554081113249,17.8493715606484));
#38213=CARTESIAN_POINT('Ctrl Pts',(56.5532874940088,19.1029385689575,17.8451403403435));
#38214=CARTESIAN_POINT('Ctrl Pts',(56.4887894776188,19.0536043204601,17.8409091200385));
#38215=CARTESIAN_POINT('Ctrl Pts',(56.4243839468701,19.0043408138221,17.8366839670074));
#38216=CARTESIAN_POINT('Ctrl Pts',(56.3574344966697,18.9582039521519,17.8324588139762));
#38217=CARTESIAN_POINT('Ctrl Pts',(56.2882782868407,18.9154642469714,17.8282336609451));
#38218=CARTESIAN_POINT('Ctrl Pts',(56.2189444174929,18.8726147452088,17.8239976536659));
#38219=CARTESIAN_POINT('Ctrl Pts',(56.1473927848897,18.8331801944124,17.8197616463867));
#38220=CARTESIAN_POINT('Ctrl Pts',(56.0739953056582,18.7973914706821,17.8155256391075));
#38221=CARTESIAN_POINT('Ctrl Pts',(56.0009176019396,18.7617586699835,17.8113080871133));
#38222=CARTESIAN_POINT('Ctrl Pts',(55.9260105188456,18.7297402069917,17.8070905351192));
#38223=CARTESIAN_POINT('Ctrl Pts',(55.849667155473,18.7015187677707,17.802872983125));
#38224=CARTESIAN_POINT('Ctrl Pts',(55.7733489989423,18.6733066466269,17.7986568236706));
#38225=CARTESIAN_POINT('Ctrl Pts',(55.695595939619,18.6488892206766,17.7944406642161));
#38226=CARTESIAN_POINT('Ctrl Pts',(55.6168204228227,18.628400789343,17.7902245047617));
#38227=CARTESIAN_POINT('Ctrl Pts',(55.5380467830875,18.6079128462073,17.7860084457698));
#38228=CARTESIAN_POINT('Ctrl Pts',(55.4582511845508,18.5913538275009,17.7817923867779));
#38229=CARTESIAN_POINT('Ctrl Pts',(55.3778591803299,18.5788075892568,17.777576327786));
#38230=CARTESIAN_POINT('Ctrl Pts',(55.2968091161902,18.5661586520366,17.7733257576575));
#38231=CARTESIAN_POINT('Ctrl Pts',(55.2151533088805,18.5575885826804,17.7690751875291));
#38232=CARTESIAN_POINT('Ctrl Pts',(55.1333343020533,18.5531301191326,17.7648246174006));
#38233=CARTESIAN_POINT('Ctrl Pts',(55.0520616077217,18.5487014251267,17.7606024286918));
#38234=CARTESIAN_POINT('Ctrl Pts',(54.9706283564138,18.5483295373821,17.7563802399831));
#38235=CARTESIAN_POINT('Ctrl Pts',(54.8894675800346,18.5519941106818,17.7521580512743));
#38236=CARTESIAN_POINT('Ctrl Pts',(54.8074884633756,18.5556956337012,17.747893290436));
#38237=CARTESIAN_POINT('Ctrl Pts',(54.7257878308633,18.5635154285282,17.7436285295977));
#38238=CARTESIAN_POINT('Ctrl Pts',(54.6448039944149,18.5753791950871,17.7393637687593));
#38239=CARTESIAN_POINT('Ctrl Pts',(54.5638201579666,18.587242961646,17.735099007921));
#38240=CARTESIAN_POINT('Ctrl Pts',(54.4835535776978,18.6031505432506,17.7308342470827));
#38241=CARTESIAN_POINT('Ctrl Pts',(54.4044275290499,18.6229758768901,17.7265694862443));
#38242=CARTESIAN_POINT('Ctrl Pts',(54.3259237731819,18.6426452926973,17.7223382659394));
#38243=CARTESIAN_POINT('Ctrl Pts',(54.2482482821312,18.6662447714308,17.7181070456345));
#38244=CARTESIAN_POINT('Ctrl Pts',(54.171823668589,18.6936881793455,17.7138758253295));
#38245=CARTESIAN_POINT('Ctrl Pts',(54.0955086425936,18.7210922353341,17.7096506722984));
#38246=CARTESIAN_POINT('Ctrl Pts',(54.0204413656159,18.7523291176063,17.7054255192672));
#38247=CARTESIAN_POINT('Ctrl Pts',(53.9470319464238,18.7872622098071,17.7012003662361));
#38248=CARTESIAN_POINT('Ctrl Pts',(53.8734339413892,18.8222850437153,17.6969643589569));
#38249=CARTESIAN_POINT('Ctrl Pts',(53.8015027792818,18.8610229817423,17.6927283516777));
#38250=CARTESIAN_POINT('Ctrl Pts',(53.7316341116842,18.9032887124459,17.6884923443985));
#38251=CARTESIAN_POINT('Ctrl Pts',(53.662069845399,18.9453703013254,17.6842747924043));
#38252=CARTESIAN_POINT('Ctrl Pts',(53.5945505440541,18.9909487722947,17.6800572404101));
#38253=CARTESIAN_POINT('Ctrl Pts',(53.5294428538567,19.0397928859616,17.675839688416));
#38254=CARTESIAN_POINT('Ctrl Pts',(53.4643566607375,19.0886208724133,17.6716235289616));
#38255=CARTESIAN_POINT('Ctrl Pts',(53.4016808691158,19.1407120815445,17.6674073695071));
#38256=CARTESIAN_POINT('Ctrl Pts',(53.3417519589761,19.195792782289,17.6631912100527));
#38257=CARTESIAN_POINT('Ctrl Pts',(53.281824476821,19.250872170572,17.6589751510608));
#38258=CARTESIAN_POINT('Ctrl Pts',(53.2246440875646,19.3089405934097,17.6547590920689));
#38259=CARTESIAN_POINT('Ctrl Pts',(53.1705119942051,19.3696859545927,17.650543033077));
#38260=CARTESIAN_POINT('Ctrl Pts',(53.1159367950752,19.4309285553684,17.6462924629485));
#38261=CARTESIAN_POINT('Ctrl Pts',(53.0644603578258,19.4948917742077,17.6420418928201));
#38262=CARTESIAN_POINT('Ctrl Pts',(53.0163501468682,19.5612215215085,17.6377913226916));
#38263=CARTESIAN_POINT('Ctrl Pts',(52.9685611718975,19.6271083794225,17.6335691339828));
#38264=CARTESIAN_POINT('Ctrl Pts',(52.9240938115442,19.6953298319304,17.6293469452741));
#38265=CARTESIAN_POINT('Ctrl Pts',(52.8831657703922,19.7655109986877,17.6251247565653));
#38266=CARTESIAN_POINT('Ctrl Pts',(52.8418250537321,19.8363997988388,17.620859995727));
#38267=CARTESIAN_POINT('Ctrl Pts',(52.8040956548996,19.9092876236642,17.6165952348887));
#38268=CARTESIAN_POINT('Ctrl Pts',(52.7701528066361,19.9837659008637,17.6123304740504));
#38269=CARTESIAN_POINT('Ctrl Pts',(52.7362099583727,20.0582441780633,17.608065713212));
#38270=CARTESIAN_POINT('Ctrl Pts',(52.7060537785096,20.1343124360727,17.6038009523737));
#38271=CARTESIAN_POINT('Ctrl Pts',(52.6798078536335,20.2115466697773,17.5995361915354));
#38272=CARTESIAN_POINT('Ctrl Pts',(52.6490720914104,20.3019932078146,17.594541866676));
#38273=CARTESIAN_POINT('Ctrl Pts',(52.6236031156726,20.394314844502,17.5895475418167));
#38274=CARTESIAN_POINT('Ctrl Pts',(52.6035969650079,20.4879426361423,17.5845532169573));
#38275=CARTESIAN_POINT('Ctrl Pts',(52.5837963477951,20.5806085414351,17.5796102013601));
#38276=CARTESIAN_POINT('Ctrl Pts',(52.5693469521956,20.6745538000929,17.5746671857628));
#38277=CARTESIAN_POINT('Ctrl Pts',(52.5603925777194,20.7692059897799,17.5697241701655));
#38278=CARTESIAN_POINT('Ctrl Pts',(52.55320888784,20.8451411630212,17.56575861219));
#38279=CARTESIAN_POINT('Ctrl Pts',(52.5495610265067,20.9215309128402,17.5617930542144));
#38280=CARTESIAN_POINT('Ctrl Pts',(52.5495007596431,20.9980704896796,17.5578274962389));
#38281=CARTESIAN_POINT('',(52.5495004847658,21.0015413750748,16.7578274961829));
#38282=CARTESIAN_POINT('Ctrl Pts',(52.5495007596427,20.9980704901969,17.5578274962121));
#38283=CARTESIAN_POINT('Ctrl Pts',(52.5494367772744,21.0793288204041,17.5536174570045));
#38284=CARTESIAN_POINT('Ctrl Pts',(52.5534188806965,21.1606384794744,17.5494074177969));
#38285=CARTESIAN_POINT('Ctrl Pts',(52.5614357122365,21.2415666873648,17.5451973785892));
#38286=CARTESIAN_POINT('Ctrl Pts',(52.5694509585329,21.3224788925592,17.5409881718723));
#38287=CARTESIAN_POINT('Ctrl Pts',(52.5814993023512,21.403009332813,17.5367789651553));
#38288=CARTESIAN_POINT('Ctrl Pts',(52.5975174476653,21.4827295679027,17.5325697584384));
#38289=CARTESIAN_POINT('Ctrl Pts',(52.6135373592028,21.5624585932572,17.5283600875979));
#38290=CARTESIAN_POINT('Ctrl Pts',(52.6335278482383,21.6413767794714,17.5241504167573));
#38291=CARTESIAN_POINT('Ctrl Pts',(52.6573746430645,21.7190665386757,17.5199407459168));
#38292=CARTESIAN_POINT('Ctrl Pts',(52.6812481566356,21.7968433440793,17.5157263584205));
#38293=CARTESIAN_POINT('Ctrl Pts',(52.7089864656818,21.8733885280204,17.5115119709242));
#38294=CARTESIAN_POINT('Ctrl Pts',(52.7404257598847,21.9483008506836,17.507297583428));
#38295=CARTESIAN_POINT('Ctrl Pts',(52.7718833922335,22.023256868765,17.5030807377324));
#38296=CARTESIAN_POINT('Ctrl Pts',(52.8070461054362,22.0965777093617,17.4988638920367));
#38297=CARTESIAN_POINT('Ctrl Pts',(52.8457034792493,22.1678855897224,17.4946470463411));
#38298=CARTESIAN_POINT('Ctrl Pts',(52.8844312239934,22.239323277192,17.4904225244035));
#38299=CARTESIAN_POINT('Ctrl Pts',(52.9266660919556,22.3087402878762,17.4861980024658));
#38300=CARTESIAN_POINT('Ctrl Pts',(52.9721537441947,22.3757869794472,17.4819734805281));
#38301=CARTESIAN_POINT('Ctrl Pts',(53.0061453314308,22.4258890039142,17.4788166192942));
#38302=CARTESIAN_POINT('Ctrl Pts',(53.0419524019041,22.474668009185,17.4756597580604));
#38303=CARTESIAN_POINT('Ctrl Pts',(53.0794547754144,22.5219908969247,17.4725028968265));
#38304=CARTESIAN_POINT('Ctrl Pts',(53.1297201474162,22.5854189505058,17.4682716765215));
#38305=CARTESIAN_POINT('Ctrl Pts',(53.183225307717,22.6464731487859,17.4640404562166));
#38306=CARTESIAN_POINT('Ctrl Pts',(53.2397176596797,22.7048038985046,17.4598092359117));
#38307=CARTESIAN_POINT('Ctrl Pts',(53.2961290055637,22.7630510060108,17.4555840828805));
#38308=CARTESIAN_POINT('Ctrl Pts',(53.355518715193,22.8185820898921,17.4513589298494));
#38309=CARTESIAN_POINT('Ctrl Pts',(53.4175933442892,22.8710797486911,17.4471337768182));
#38310=CARTESIAN_POINT('Ctrl Pts',(53.4798274406086,22.9237122718622,17.442897769539));
#38311=CARTESIAN_POINT('Ctrl Pts',(53.5447599707556,22.9732953985627,17.4386617622598));
#38312=CARTESIAN_POINT('Ctrl Pts',(53.6120572539298,23.0195457864656,17.4344257549806));
#38313=CARTESIAN_POINT('Ctrl Pts',(53.679061338707,23.0655946723323,17.4302082029865));
#38314=CARTESIAN_POINT('Ctrl Pts',(53.7484092331817,23.108339527016,17.4259906509923));
#38315=CARTESIAN_POINT('Ctrl Pts',(53.8197391798873,23.1475415354556,17.4217730989982));
#38316=CARTESIAN_POINT('Ctrl Pts',(53.8910455750672,23.1867306002838,17.4175569395437));
#38317=CARTESIAN_POINT('Ctrl Pts',(53.9643323157518,23.2223789181121,17.4133407800893));
#38318=CARTESIAN_POINT('Ctrl Pts',(54.0392113547849,23.2542926671632,17.4091246206349));
#38319=CARTESIAN_POINT('Ctrl Pts',(54.1140886096023,23.2862056557744,17.404908561643));
#38320=CARTESIAN_POINT('Ctrl Pts',(54.1905576592002,23.314384071272,17.4006925026511));
#38321=CARTESIAN_POINT('Ctrl Pts',(54.2682100323667,23.3386820419354,17.3964764436592));
#38322=CARTESIAN_POINT('Ctrl Pts',(54.3464980398213,23.3631789070133,17.3922258735307));
#38323=CARTESIAN_POINT('Ctrl Pts',(54.4259883797476,23.3837313476125,17.3879753034022));
#38324=CARTESIAN_POINT('Ctrl Pts',(54.5062482170537,23.4002415351038,17.3837247332737));
#38325=CARTESIAN_POINT('Ctrl Pts',(54.5859721525723,23.4166414826633,17.379502544565));
#38326=CARTESIAN_POINT('Ctrl Pts',(54.6664548673223,23.4290529831988,17.3752803558562));
#38327=CARTESIAN_POINT('Ctrl Pts',(54.747265082537,23.4374321142331,17.3710581671475));
#38328=CARTESIAN_POINT('Ctrl Pts',(54.82889010334,23.4458957316504,17.3667934063091));
#38329=CARTESIAN_POINT('Ctrl Pts',(54.9108487810094,23.4502451797474,17.3625286454708));
#38330=CARTESIAN_POINT('Ctrl Pts',(54.9926966350904,23.4504891166583,17.3582638846324));
#38331=CARTESIAN_POINT('Ctrl Pts',(55.0745444891714,23.4507330535693,17.3539991237941));
#38332=CARTESIAN_POINT('Ctrl Pts',(55.1562810414348,23.4468715662079,17.3497343629558));
#38333=CARTESIAN_POINT('Ctrl Pts',(55.2374690269802,23.4389667302415,17.3454696021174));
#38334=CARTESIAN_POINT('Ctrl Pts',(55.3180185034872,23.4311240624541,17.3412383818125));
#38335=CARTESIAN_POINT('Ctrl Pts',(55.3983300667665,23.4192720537597,17.3370071615076));
#38336=CARTESIAN_POINT('Ctrl Pts',(55.4779730127825,23.4034333876876,17.3327759412026));
#38337=CARTESIAN_POINT('Ctrl Pts',(55.5575017563879,23.3876174331542,17.3285507881715));
#38338=CARTESIAN_POINT('Ctrl Pts',(55.6363633347351,23.3678262647335,17.3243256351403));
#38339=CARTESIAN_POINT('Ctrl Pts',(55.7141319439969,23.3441343426867,17.3201004821092));
#38340=CARTESIAN_POINT('Ctrl Pts',(55.7921003376853,23.3203815570459,17.31586447483));
#38341=CARTESIAN_POINT('Ctrl Pts',(55.8689696703445,23.2927080024995,17.3116284675508));
#38342=CARTESIAN_POINT('Ctrl Pts',(55.9443209387124,23.2612404150619,17.3073924602716));
#38343=CARTESIAN_POINT('Ctrl Pts',(56.0193439193687,23.2299099244841,17.3031749082774));
#38344=CARTESIAN_POINT('Ctrl Pts',(56.0928616009562,23.1948185642367,17.2989573562833));
#38345=CARTESIAN_POINT('Ctrl Pts',(56.1644771698154,23.1561408049983,17.2947398042891));
#38346=CARTESIAN_POINT('Ctrl Pts',(56.2360690928429,23.1174758162761,17.2905236448347));
#38347=CARTESIAN_POINT('Ctrl Pts',(56.305759741577,23.0752270008704,17.2863074853803));
#38348=CARTESIAN_POINT('Ctrl Pts',(56.3731758524629,23.0296153153277,17.2820913259258));
#38349=CARTESIAN_POINT('Ctrl Pts',(56.4405903569595,22.984004716619,17.2778752669339));
#38350=CARTESIAN_POINT('Ctrl Pts',(56.5057300469187,22.9350316685375,17.273659207942));
#38351=CARTESIAN_POINT('Ctrl Pts',(56.5682508737503,22.8829602882115,17.2694431489501));
#38352=CARTESIAN_POINT('Ctrl Pts',(56.6312834734953,22.8304626703681,17.2651925788217));
#38353=CARTESIAN_POINT('Ctrl Pts',(56.6916537591947,22.774816057167,17.2609420086932));
#38354=CARTESIAN_POINT('Ctrl Pts',(56.7490448391351,22.7163310871434,17.2566914385647));
#38355=CARTESIAN_POINT('Ctrl Pts',(56.8060527139339,22.6582366262589,17.252469249856));
#38356=CARTESIAN_POINT('Ctrl Pts',(56.8601207811346,22.597341989153,17.2482470611472));
#38357=CARTESIAN_POINT('Ctrl Pts',(56.9109782867531,22.533985735774,17.2440248724385));
#38358=CARTESIAN_POINT('Ctrl Pts',(56.9623485862017,22.4699906642809,17.2397601116001));
#38359=CARTESIAN_POINT('Ctrl Pts',(57.0104429311022,22.40348445004,17.2354953507618));
#38360=CARTESIAN_POINT('Ctrl Pts',(57.0550275893164,22.3348452558811,17.2312305899234));
#38361=CARTESIAN_POINT('Ctrl Pts',(57.0996122475307,22.2662060617222,17.2269658290851));
#38362=CARTESIAN_POINT('Ctrl Pts',(57.1406870327804,22.1954343365968,17.2227010682468));
#38363=CARTESIAN_POINT('Ctrl Pts',(57.1780670086594,22.1229311447233,17.2184363074084));
#38364=CARTESIAN_POINT('Ctrl Pts',(57.2151530068976,22.050998159673,17.2142050871035));
#38365=CARTESIAN_POINT('Ctrl Pts',(57.2487412133422,21.9770911255402,17.2099738667986));
#38366=CARTESIAN_POINT('Ctrl Pts',(57.2786171503632,21.9015842345953,17.2057426464936));
#38367=CARTESIAN_POINT('Ctrl Pts',(57.3084502473815,21.8261856152472,17.2015174934625));
#38368=CARTESIAN_POINT('Ctrl Pts',(57.3345814775107,21.7491921239713,17.1972923404313));
#38369=CARTESIAN_POINT('Ctrl Pts',(57.3568425247626,21.6710019101842,17.1930671874002));
#38370=CARTESIAN_POINT('Ctrl Pts',(57.3791607597486,21.5926108288857,17.188831180121));
#38371=CARTESIAN_POINT('Ctrl Pts',(57.3975886911264,21.5130172910209,17.1845951728418));
#38372=CARTESIAN_POINT('Ctrl Pts',(57.4120056142599,21.4326420769861,17.1803591655626));
#38373=CARTESIAN_POINT('Ctrl Pts',(57.4263597262582,21.3526170388096,17.1761416135684));
#38374=CARTESIAN_POINT('Ctrl Pts',(57.4367376165063,21.2718175804945,17.1719240615743));
#38375=CARTESIAN_POINT('Ctrl Pts',(57.4430707204082,21.1906717207252,17.1677065095801));
#38376=CARTESIAN_POINT('Ctrl Pts',(57.4494017332632,21.1095526534727,17.1634903501257));
#38377=CARTESIAN_POINT('Ctrl Pts',(57.4516905757335,21.0280878750446,17.1592741906712));
#38378=CARTESIAN_POINT('Ctrl Pts',(57.4499205116746,20.9467108221472,17.1550580312168));
#38379=CARTESIAN_POINT('Ctrl Pts',(57.4481504897927,20.8653357083001,17.1508419722249));
#38380=CARTESIAN_POINT('Ctrl Pts',(57.4423217648956,20.7840487806151,17.146625913233));
#38381=CARTESIAN_POINT('Ctrl Pts',(57.4324697068783,20.7032823309619,17.1424098542411));
#38382=CARTESIAN_POINT('Ctrl Pts',(57.4225370034714,20.6218547563151,17.1381592841126));
#38383=CARTESIAN_POINT('Ctrl Pts',(57.408514837968,20.5409566980519,17.1339087139841));
#38384=CARTESIAN_POINT('Ctrl Pts',(57.390492394246,20.461022854796,17.1296581438557));
#38385=CARTESIAN_POINT('Ctrl Pts',(57.3725902879197,20.3816227366374,17.1254359551469));
#38386=CARTESIAN_POINT('Ctrl Pts',(57.3507413466095,20.3031744321134,17.1212137664382));
#38387=CARTESIAN_POINT('Ctrl Pts',(57.3250832316369,20.2260890128955,17.1169915777294));
#38388=CARTESIAN_POINT('Ctrl Pts',(57.2991664071013,20.1482263450319,17.1127268168911));
#38389=CARTESIAN_POINT('Ctrl Pts',(57.2693633375133,20.0717546536215,17.1084620560528));
#38390=CARTESIAN_POINT('Ctrl Pts',(57.2358650339893,19.9970753768183,17.1041972952144));
#38391=CARTESIAN_POINT('Ctrl Pts',(57.2023667304652,19.9223961000151,17.0999325343761));
#38392=CARTESIAN_POINT('Ctrl Pts',(57.1651734692259,19.849509637768,17.0956677735378));
#38393=CARTESIAN_POINT('Ctrl Pts',(57.1245219620561,19.7787888459642,17.0914030126994));
#38394=CARTESIAN_POINT('Ctrl Pts',(57.0841901617316,19.7086242431636,17.0871717923945));
#38395=CARTESIAN_POINT('Ctrl Pts',(57.0403031164513,19.6403282362304,17.0829405720896));
#38396=CARTESIAN_POINT('Ctrl Pts',(56.9930589413419,19.5742839320758,17.0787093517847));
#38397=CARTESIAN_POINT('Ctrl Pts',(56.9458825110729,19.5083343308308,17.0744841987535));
#38398=CARTESIAN_POINT('Ctrl Pts',(56.8953587799322,19.4446303947001,17.0702590457223));
#38399=CARTESIAN_POINT('Ctrl Pts',(56.8417310225385,19.3835294340386,17.0660338926912));
#38400=CARTESIAN_POINT('Ctrl Pts',(56.787965497595,19.3222715074691,17.061797885412));
#38401=CARTESIAN_POINT('Ctrl Pts',(56.731080218543,19.2636303533888,17.0575618781328));
#38402=CARTESIAN_POINT('Ctrl Pts',(56.6713632912655,19.2079355484218,17.0533258708536));
#38403=CARTESIAN_POINT('Ctrl Pts',(56.6119065365613,19.1524833925895,17.0491083188594));
#38404=CARTESIAN_POINT('Ctrl Pts',(56.5496430924026,19.0999522914064,17.0448907668653));
#38405=CARTESIAN_POINT('Ctrl Pts',(56.4848954180064,19.0506319363487,17.0406732148711));
#38406=CARTESIAN_POINT('Ctrl Pts',(56.4201691218193,19.0013278657502,17.0364570554167));
#38407=CARTESIAN_POINT('Ctrl Pts',(56.3529605938229,18.9552327175379,17.0322408959622));
#38408=CARTESIAN_POINT('Ctrl Pts',(56.2836249481658,18.9125955728593,17.0280247365078));
#38409=CARTESIAN_POINT('Ctrl Pts',(56.2142909546365,18.8699594441375,17.0238086775159));
#38410=CARTESIAN_POINT('Ctrl Pts',(56.1428303408352,18.8307813977141,17.019592618524));
#38411=CARTESIAN_POINT('Ctrl Pts',(56.0696255120111,18.7952661126442,17.0153765595321));
#38412=CARTESIAN_POINT('Ctrl Pts',(55.9958214548911,18.7594601122746,17.0111259894036));
#38413=CARTESIAN_POINT('Ctrl Pts',(55.9202449205161,18.7273773379552,17.0068754192751));
#38414=CARTESIAN_POINT('Ctrl Pts',(55.8433095154918,18.6991785573233,17.0026248491467));
#38415=CARTESIAN_POINT('Ctrl Pts',(55.7668878147366,18.6711680623577,16.9984026604379));
#38416=CARTESIAN_POINT('Ctrl Pts',(55.6891258013491,18.6469899318883,16.9941804717292));
#38417=CARTESIAN_POINT('Ctrl Pts',(55.6104435152623,18.6267513900406,16.9899582830204));
#38418=CARTESIAN_POINT('Ctrl Pts',(55.5309678793967,18.6063087839302,16.9856935221821));
#38419=CARTESIAN_POINT('Ctrl Pts',(55.4505537842166,18.5898857561827,16.9814287613438));
#38420=CARTESIAN_POINT('Ctrl Pts',(55.3696421026568,18.5775394810351,16.9771640005054));
#38421=CARTESIAN_POINT('Ctrl Pts',(55.2887304210971,18.5651932058876,16.9728992396671));
#38422=CARTESIAN_POINT('Ctrl Pts',(55.2073216389819,18.5569236681106,16.9686344788288));
#38423=CARTESIAN_POINT('Ctrl Pts',(55.125857393315,18.5527341446937,16.9643697179904));
#38424=CARTESIAN_POINT('Ctrl Pts',(55.0450338293549,18.5485775700999,16.9601384976855));
#38425=CARTESIAN_POINT('Ctrl Pts',(54.9638525942866,18.5484214315561,16.9559072773806));
#38426=CARTESIAN_POINT('Ctrl Pts',(54.8827430104361,18.5523069946584,16.9516760570757));
#38427=CARTESIAN_POINT('Ctrl Pts',(54.8017497320516,18.556186986135,16.9474509040445));
#38428=CARTESIAN_POINT('Ctrl Pts',(54.7208283613012,18.5640971468667,16.9432257510133));
#38429=CARTESIAN_POINT('Ctrl Pts',(54.6404110317942,18.5760268103907,16.9390005979822));
#38430=CARTESIAN_POINT('Ctrl Pts',(54.5597871134052,18.58798712074,16.934764590703));
#38431=CARTESIAN_POINT('Ctrl Pts',(54.4796703010171,18.6039876300277,16.9305285834238));
#38432=CARTESIAN_POINT('Ctrl Pts',(54.4004937338682,18.6239649651428,16.9262925761446));
#38433=CARTESIAN_POINT('Ctrl Pts',(54.3216621203559,18.6438552637186,16.9220750241504));
#38434=CARTESIAN_POINT('Ctrl Pts',(54.24376303197,18.6676877016687,16.9178574721563));
#38435=CARTESIAN_POINT('Ctrl Pts',(54.1672147221646,18.6953484143974,16.9136399201621));
#38436=CARTESIAN_POINT('Ctrl Pts',(54.0906916868695,18.7229999941881,16.9094237607077));
#38437=CARTESIAN_POINT('Ctrl Pts',(54.0155189813761,18.7544771807362,16.9052076012532));
#38438=CARTESIAN_POINT('Ctrl Pts',(53.9420984431211,18.7896166518106,16.9009914417988));
#38439=CARTESIAN_POINT('Ctrl Pts',(53.8686796543287,18.8247552855825,16.8967753828069));
#38440=CARTESIAN_POINT('Ctrl Pts',(53.7970133686507,18.8635558286649,16.892559323815));
#38441=CARTESIAN_POINT('Ctrl Pts',(53.7274789131453,18.9058079520946,16.8883432648231));
#38442=CARTESIAN_POINT('Ctrl Pts',(53.6573752736946,18.9484059361503,16.8840926946946));
#38443=CARTESIAN_POINT('Ctrl Pts',(53.5894389445941,18.9945120327593,16.8798421245662));
#38444=CARTESIAN_POINT('Ctrl Pts',(53.5240292750327,19.0438658867451,16.8755915544377));
#38445=CARTESIAN_POINT('Ctrl Pts',(53.4590563514206,19.0928902008334,16.8713693657289));
#38446=CARTESIAN_POINT('Ctrl Pts',(53.3965767692371,19.1451186847214,16.8671471770202));
#38447=CARTESIAN_POINT('Ctrl Pts',(53.336908376809,19.2002565452621,16.8629249883114));
#38448=CARTESIAN_POINT('Ctrl Pts',(53.2766383507949,19.2559503582496,16.8586602274731));
#38449=CARTESIAN_POINT('Ctrl Pts',(53.2192368635663,19.3146122011117,16.8543954666348));
#38450=CARTESIAN_POINT('Ctrl Pts',(53.1649910058721,19.375902637934,16.8501307057964));
#38451=CARTESIAN_POINT('Ctrl Pts',(53.1107451481779,19.4371930747563,16.8458659449581));
#38452=CARTESIAN_POINT('Ctrl Pts',(53.0596551706464,19.5011116890745,16.8416011841198));
#38453=CARTESIAN_POINT('Ctrl Pts',(53.0119632919475,19.5672891787119,16.8373364232815));
#38454=CARTESIAN_POINT('Ctrl Pts',(52.9642693426104,19.6334695415775,16.83307147728));
#38455=CARTESIAN_POINT('Ctrl Pts',(52.9197953624586,19.7021563126665,16.8288065312786));
#38456=CARTESIAN_POINT('Ctrl Pts',(52.8788124314755,19.7730062962113,16.8245415852771));
#38457=CARTESIAN_POINT('Ctrl Pts',(52.8378901528898,19.8437514258265,16.8202829511522));
#38458=CARTESIAN_POINT('Ctrl Pts',(52.8004488875799,19.9166530190759,16.8160243170272));
#38459=CARTESIAN_POINT('Ctrl Pts',(52.7667177235425,19.9913372597043,16.8117656829023));
#38460=CARTESIAN_POINT('Ctrl Pts',(52.733026705015,20.0659326140753,16.8075121172369));
#38461=CARTESIAN_POINT('Ctrl Pts',(52.7030372009587,20.1423059881466,16.8032585515714));
#38462=CARTESIAN_POINT('Ctrl Pts',(52.6769327916645,20.2200583383636,16.799004985906));
#38463=CARTESIAN_POINT('Ctrl Pts',(52.6508537261519,20.2977352017704,16.7947555498662));
#38464=CARTESIAN_POINT('Ctrl Pts',(52.628652398988,20.376787948993,16.7905061138265));
#38465=CARTESIAN_POINT('Ctrl Pts',(52.6104640516671,20.4567981943839,16.7862566777868));
#38466=CARTESIAN_POINT('Ctrl Pts',(52.592285823686,20.5367639249625,16.7820096059798));
#38467=CARTESIAN_POINT('Ctrl Pts',(52.5781162378917,20.6176856516973,16.7777625341729));
#38468=CARTESIAN_POINT('Ctrl Pts',(52.5680402033317,20.6991315945648,16.773515462366));
#38469=CARTESIAN_POINT('Ctrl Pts',(52.5579660429577,20.780562388135,16.7692691805328));
#38470=CARTESIAN_POINT('Ctrl Pts',(52.551983977712,20.8625167527755,16.7650228986996));
#38471=CARTESIAN_POINT('Ctrl Pts',(52.5501273132381,20.9445557157339,16.7607766168664));
#38472=CARTESIAN_POINT('Ctrl Pts',(52.5496974840555,20.9635482374755,16.7597935766483));
#38473=CARTESIAN_POINT('Ctrl Pts',(52.549488536141,20.9825452782313,16.7588105364302));
#38474=CARTESIAN_POINT('Ctrl Pts',(52.5495004847655,21.0015413745099,16.7578274962121));
#38475=CARTESIAN_POINT('',(52.5495002472464,21.0011007971719,15.957827496239));
#38476=CARTESIAN_POINT('Ctrl Pts',(52.5495004847658,21.0015413750748,16.7578274961829));
#38477=CARTESIAN_POINT('Ctrl Pts',(52.5495581962121,21.0932918344117,16.7530794474136));
#38478=CARTESIAN_POINT('Ctrl Pts',(52.5547728996673,21.1848479458307,16.7483313986442));
#38479=CARTESIAN_POINT('Ctrl Pts',(52.565054999287,21.2756684485081,16.7435833498749));
#38480=CARTESIAN_POINT('Ctrl Pts',(52.5753836098533,21.366899776572,16.7388138233675));
#38481=CARTESIAN_POINT('Ctrl Pts',(52.5908254338274,21.4573886044141,16.7340442968602));
#38482=CARTESIAN_POINT('Ctrl Pts',(52.6112400460042,21.5466041823713,16.7292747703528));
#38483=CARTESIAN_POINT('Ctrl Pts',(52.6317667984321,21.6363098336761,16.7244790441852));
#38484=CARTESIAN_POINT('Ctrl Pts',(52.6573209987667,21.7247279934454,16.7196833180177));
#38485=CARTESIAN_POINT('Ctrl Pts',(52.6877117586267,21.8113404580119,16.7148875918502));
#38486=CARTESIAN_POINT('Ctrl Pts',(52.6973957506987,21.8389394527082,16.7133594374243));
#38487=CARTESIAN_POINT('Ctrl Pts',(52.7075704774109,21.866355276581,16.7118312829984));
#38488=CARTESIAN_POINT('Ctrl Pts',(52.7182287750057,21.8935716685236,16.7103031285726));
#38489=CARTESIAN_POINT('Ctrl Pts',(52.7477399320168,21.9689295958798,16.7060719082677));
#38490=CARTESIAN_POINT('Ctrl Pts',(52.7810435953473,22.0429652853492,16.7018406879627));
#38491=CARTESIAN_POINT('Ctrl Pts',(52.8180004887935,22.1152705425566,16.6976094676578));
#38492=CARTESIAN_POINT('Ctrl Pts',(52.8549043886411,22.1874721190857,16.6933843146267));
#38493=CARTESIAN_POINT('Ctrl Pts',(52.8954509047876,22.2579477809502,16.6891591615955));
#38494=CARTESIAN_POINT('Ctrl Pts',(52.939452282941,22.3263081677058,16.6849340085644));
#38495=CARTESIAN_POINT('Ctrl Pts',(52.9835666988637,22.3948441695432,16.6806980012852));
#38496=CARTESIAN_POINT('Ctrl Pts',(53.0311535722193,22.4612535770766,16.676461994006));
#38497=CARTESIAN_POINT('Ctrl Pts',(53.0819767087438,22.5251678282073,16.6722259867268));
#38498=CARTESIAN_POINT('Ctrl Pts',(53.1325784208443,22.5888036200142,16.6680084347326));
#38499=CARTESIAN_POINT('Ctrl Pts',(53.1863879708527,22.6499655803971,16.6637908827385));
#38500=CARTESIAN_POINT('Ctrl Pts',(53.2431292900819,22.7083195130396,16.6595733307443));
#38501=CARTESIAN_POINT('Ctrl Pts',(53.2998518746183,22.7666541785411,16.6553571712899));
#38502=CARTESIAN_POINT('Ctrl Pts',(53.3595039821995,22.8221823244247,16.6511410118355));
#38503=CARTESIAN_POINT('Ctrl Pts',(53.4217712421883,22.8746050885497,16.646924852381));
#38504=CARTESIAN_POINT('Ctrl Pts',(53.4840370184745,22.9270266035463,16.6427087933891));
#38505=CARTESIAN_POINT('Ctrl Pts',(53.5489174668984,22.9763425853237,16.6384927343972));
#38506=CARTESIAN_POINT('Ctrl Pts',(53.6160646589281,23.0222940492748,16.6342766754053));
#38507=CARTESIAN_POINT('Ctrl Pts',(53.6837614936266,23.0686216553178,16.6300261052769));
#38508=CARTESIAN_POINT('Ctrl Pts',(53.7537619658826,23.1115291236671,16.6257755351484));
#38509=CARTESIAN_POINT('Ctrl Pts',(53.8256807945839,23.1507962836566,16.6215249650199));
#38510=CARTESIAN_POINT('Ctrl Pts',(53.8971194151244,23.1898012534655,16.6173027763111));
#38511=CARTESIAN_POINT('Ctrl Pts',(53.9704504023963,23.2252142316627,16.6130805876024));
#38512=CARTESIAN_POINT('Ctrl Pts',(54.0452741938042,23.2568670507994,16.6088583988936));
#38513=CARTESIAN_POINT('Ctrl Pts',(54.1208524299715,23.2888390238184,16.6045936380553));
#38514=CARTESIAN_POINT('Ctrl Pts',(54.197953287101,23.3169744174355,16.6003288772169));
#38515=CARTESIAN_POINT('Ctrl Pts',(54.2761491964903,23.3411514825526,16.5960641163786));
#38516=CARTESIAN_POINT('Ctrl Pts',(54.3543451058797,23.3653285476697,16.5917993555402));
#38517=CARTESIAN_POINT('Ctrl Pts',(54.433635584795,23.3855472274969,16.5875345947019));
#38518=CARTESIAN_POINT('Ctrl Pts',(54.5135843376472,23.4017389644626,16.5832698338635));
#38519=CARTESIAN_POINT('Ctrl Pts',(54.5929043275,23.4178033602912,16.5790386135586));
#38520=CARTESIAN_POINT('Ctrl Pts',(54.673169706054,23.4299642119077,16.5748073932536));
#38521=CARTESIAN_POINT('Ctrl Pts',(54.7539619753578,23.4381172122009,16.5705761729487));
#38522=CARTESIAN_POINT('Ctrl Pts',(54.8346383942022,23.4462585216623,16.5663510199175));
#38523=CARTESIAN_POINT('Ctrl Pts',(54.9158397445982,23.4504033474446,16.5621258668864));
#38524=CARTESIAN_POINT('Ctrl Pts',(54.9971370676512,23.4504983276098,16.5579007138552));
#38525=CARTESIAN_POINT('Ctrl Pts',(55.0786432402543,23.4505935517752,16.553664706576));
#38526=CARTESIAN_POINT('Ctrl Pts',(55.1602454153505,23.4466180085095,16.5494286992968));
#38527=CARTESIAN_POINT('Ctrl Pts',(55.2415058443402,23.4385703141697,16.5451926920176));
#38528=CARTESIAN_POINT('Ctrl Pts',(55.3224122407987,23.4305576817368,16.5409751400235));
#38529=CARTESIAN_POINT('Ctrl Pts',(55.402979396355,23.4185083450086,16.5367575880293));
#38530=CARTESIAN_POINT('Ctrl Pts',(55.4827768169721,23.4024730581204,16.5325400360352));
#38531=CARTESIAN_POINT('Ctrl Pts',(55.5625478902963,23.3864430657191,16.5283238765807));
#38532=CARTESIAN_POINT('Ctrl Pts',(55.6415492779336,23.3664298282112,16.5241077171263));
#38533=CARTESIAN_POINT('Ctrl Pts',(55.7193594067178,23.342535441347,16.5198915576719));
#38534=CARTESIAN_POINT('Ctrl Pts',(55.7971676814443,23.3186416238375,16.51567549868));
#38535=CARTESIAN_POINT('Ctrl Pts',(55.8737843096423,23.2908669783861,16.5114594396881));
#38536=CARTESIAN_POINT('Ctrl Pts',(55.9488030288365,23.2593634197425,16.5072433806962));
#38537=CARTESIAN_POINT('Ctrl Pts',(56.0244358241783,23.2276019843432,16.5029928105677));
#38538=CARTESIAN_POINT('Ctrl Pts',(56.0984439814427,23.1920504778421,16.4987422404392));
#38539=CARTESIAN_POINT('Ctrl Pts',(56.1704335976159,23.1529132457143,16.4944916703108));
#38540=CARTESIAN_POINT('Ctrl Pts',(56.2419425329744,23.1140373362275,16.490269481602));
#38541=CARTESIAN_POINT('Ctrl Pts',(56.311459432492,23.0716237369869,16.4860472928933));
#38542=CARTESIAN_POINT('Ctrl Pts',(56.3786263443655,23.0259169905555,16.4818251041845));
#38543=CARTESIAN_POINT('Ctrl Pts',(56.4464704970428,22.979749385156,16.4775603433462));
#38544=CARTESIAN_POINT('Ctrl Pts',(56.5119166183364,22.9302221426357,16.4732955825079));
#38545=CARTESIAN_POINT('Ctrl Pts',(56.5746305732602,22.8776285063223,16.4690308216695));
#38546=CARTESIAN_POINT('Ctrl Pts',(56.637344528184,22.825034870009,16.4647660608312));
#38547=CARTESIAN_POINT('Ctrl Pts',(56.6973260072724,22.7693752147199,16.4605012999929));
#38548=CARTESIAN_POINT('Ctrl Pts',(56.754280837033,22.7109789580292,16.4562365391545));
#38549=CARTESIAN_POINT('Ctrl Pts',(56.8107877412375,22.6530419631055,16.4520053188496));
#38550=CARTESIAN_POINT('Ctrl Pts',(56.8645273599191,22.5921940322417,16.4477740985447));
#38551=CARTESIAN_POINT('Ctrl Pts',(56.9151851318255,22.5287302446261,16.4435428782398));
#38552=CARTESIAN_POINT('Ctrl Pts',(56.9657702640325,22.4653574596401,16.4393177252086));
#38553=CARTESIAN_POINT('Ctrl Pts',(57.013282038641,22.3993766278748,16.4350925721775));
#38554=CARTESIAN_POINT('Ctrl Pts',(57.0574430281834,22.3311192417584,16.4308674191463));
#38555=CARTESIAN_POINT('Ctrl Pts',(57.1017174655301,22.2626865051649,16.4266314118671));
#38556=CARTESIAN_POINT('Ctrl Pts',(57.1426235547403,22.1919658448864,16.4223954045879));
#38557=CARTESIAN_POINT('Ctrl Pts',(57.1799227763783,22.1193243225388,16.4181593973087));
#38558=CARTESIAN_POINT('Ctrl Pts',(57.2170594941013,22.0469992821782,16.4139418453146));
#38559=CARTESIAN_POINT('Ctrl Pts',(57.250620486266,21.9727704948047,16.4097242933204));
#38560=CARTESIAN_POINT('Ctrl Pts',(57.2804149750245,21.8970271967359,16.4055067413262));
#38561=CARTESIAN_POINT('Ctrl Pts',(57.3101996263207,21.8213089073809,16.4012905818718));
#38562=CARTESIAN_POINT('Ctrl Pts',(57.336220073798,21.7440775326862,16.3970744224174));
#38563=CARTESIAN_POINT('Ctrl Pts',(57.3583335157403,21.6657426518827,16.3928582629629));
#38564=CARTESIAN_POINT('Ctrl Pts',(57.3804464307642,21.5874096376408,16.388642203971));
#38565=CARTESIAN_POINT('Ctrl Pts',(57.3986524001108,21.5079736173066,16.3844261449791));
#38566=CARTESIAN_POINT('Ctrl Pts',(57.4128587835408,21.4278583184769,16.3802100859873));
#38567=CARTESIAN_POINT('Ctrl Pts',(57.427181455296,21.3470872247388,16.3759595158588));
#38568=CARTESIAN_POINT('Ctrl Pts',(57.4374386610082,21.2656261500641,16.3717089457303));
#38569=CARTESIAN_POINT('Ctrl Pts',(57.4435885161579,21.1839168662768,16.3674583756018));
#38570=CARTESIAN_POINT('Ctrl Pts',(57.4496973081996,21.1027531623549,16.3632361868931));
#38571=CARTESIAN_POINT('Ctrl Pts',(57.451753482844,21.0213450247708,16.3590139981843));
#38572=CARTESIAN_POINT('Ctrl Pts',(57.4497684241177,20.9401258136087,16.3547918094756));
#38573=CARTESIAN_POINT('Ctrl Pts',(57.4477633501379,20.8580876729716,16.3505270486372));
#38574=CARTESIAN_POINT('Ctrl Pts',(57.4416351252318,20.7762427745138,16.3462622877989));
#38575=CARTESIAN_POINT('Ctrl Pts',(57.4314489675299,20.6950308732054,16.3419975269605));
#38576=CARTESIAN_POINT('Ctrl Pts',(57.421262809828,20.6138189718969,16.3377327661222));
#38577=CARTESIAN_POINT('Ctrl Pts',(57.407018866466,20.5332405309958,16.3334680052839));
#38578=CARTESIAN_POINT('Ctrl Pts',(57.3888344184503,20.453721342878,16.3292032444455));
#38579=CARTESIAN_POINT('Ctrl Pts',(57.3707929833981,20.3748275394152,16.3249720241406));
#38580=CARTESIAN_POINT('Ctrl Pts',(57.3488051943653,20.2966805340988,16.3207408038357));
#38581=CARTESIAN_POINT('Ctrl Pts',(57.3229484253431,20.2197046307994,16.3165095835307));
#38582=CARTESIAN_POINT('Ctrl Pts',(57.2971287331179,20.1428391055576,16.3122844304996));
#38583=CARTESIAN_POINT('Ctrl Pts',(57.2674512261356,20.0671417841638,16.3080592774684));
#38584=CARTESIAN_POINT('Ctrl Pts',(57.2340440088283,19.9930255134224,16.3038341244373));
#38585=CARTESIAN_POINT('Ctrl Pts',(57.2005509697248,19.9187188409653,16.2995981171581));
#38586=CARTESIAN_POINT('Ctrl Pts',(57.1633091442996,19.8460018115726,16.2953621098789));
#38587=CARTESIAN_POINT('Ctrl Pts',(57.1224976202594,19.7752738665346,16.2911261025997));
#38588=CARTESIAN_POINT('Ctrl Pts',(57.0818639024078,19.7048540664783,16.2869085506055));
#38589=CARTESIAN_POINT('Ctrl Pts',(57.0376917524969,19.6364064643124,16.2826909986114));
#38590=CARTESIAN_POINT('Ctrl Pts',(56.9902047767333,19.5703024107638,16.2784734466172));
#38591=CARTESIAN_POINT('Ctrl Pts',(56.9427334800888,19.5042201832698,16.2742572871628));
#38592=CARTESIAN_POINT('Ctrl Pts',(56.8919498021123,19.4404803450574,16.2700411277083));
#38593=CARTESIAN_POINT('Ctrl Pts',(56.8381204555523,19.3794249659827,16.2658249682539));
#38594=CARTESIAN_POINT('Ctrl Pts',(56.7842923916366,19.318371041734,16.261608909262));
#38595=CARTESIAN_POINT('Ctrl Pts',(56.7274191117251,19.2600017974482,16.2573928502701));
#38596=CARTESIAN_POINT('Ctrl Pts',(56.6678064151717,19.2046248270871,16.2531767912782));
#38597=CARTESIAN_POINT('Ctrl Pts',(56.6077057506092,19.1487945608421,16.2489262211497));
#38598=CARTESIAN_POINT('Ctrl Pts',(56.544820955192,19.096006120237,16.2446756510213));
#38599=CARTESIAN_POINT('Ctrl Pts',(56.4795005105318,19.0465342364566,16.2404250808928));
#38600=CARTESIAN_POINT('Ctrl Pts',(56.4146162160586,18.9973926806689,16.236202892184));
#38601=CARTESIAN_POINT('Ctrl Pts',(56.3473291221265,18.9515237400961,16.2319807034753));
#38602=CARTESIAN_POINT('Ctrl Pts',(56.2780095258749,18.9091528267774,16.2277585147665));
#38603=CARTESIAN_POINT('Ctrl Pts',(56.2079909834042,18.8663546895384,16.2234937539282));
#38604=CARTESIAN_POINT('Ctrl Pts',(56.1358991473785,18.8271257496791,16.2192289930899));
#38605=CARTESIAN_POINT('Ctrl Pts',(56.0621388781727,18.791649653367,16.2149642322515));
#38606=CARTESIAN_POINT('Ctrl Pts',(55.988378608967,18.756173557055,16.2106994714132));
#38607=CARTESIAN_POINT('Ctrl Pts',(55.9129503756073,18.7244504318501,16.2064347105749));
#38608=CARTESIAN_POINT('Ctrl Pts',(55.8362755362313,18.6966126080268,16.2021699497365));
#38609=CARTESIAN_POINT('Ctrl Pts',(55.7602037119151,18.6689937168694,16.1979387294316));
#38610=CARTESIAN_POINT('Ctrl Pts',(55.6826195745121,18.6450956221778,16.1937075091267));
#38611=CARTESIAN_POINT('Ctrl Pts',(55.6039215930101,18.6250833784118,16.1894762888218));
#38612=CARTESIAN_POINT('Ctrl Pts',(55.5253364589055,18.6050998308026,16.1852511357906));
#38613=CARTESIAN_POINT('Ctrl Pts',(55.4456410995906,18.5889911812454,16.1810259827594));
#38614=CARTESIAN_POINT('Ctrl Pts',(55.3652518645743,18.5768736464177,16.1768008297283));
#38615=CARTESIAN_POINT('Ctrl Pts',(55.2846561128495,18.5647249821309,16.1725648224491));
#38616=CARTESIAN_POINT('Ctrl Pts',(55.2033633616496,18.5565881198942,16.1683288151699));
#38617=CARTESIAN_POINT('Ctrl Pts',(55.1218063409409,18.552529169672,16.1640928078907));
#38618=CARTESIAN_POINT('Ctrl Pts',(55.0406046449437,18.548487903339,16.1598752558965));
#38619=CARTESIAN_POINT('Ctrl Pts',(54.9591414442423,18.5484891215448,16.1556577039024));
#38620=CARTESIAN_POINT('Ctrl Pts',(54.8778500050207,18.5525462969187,16.1514401519082));
#38621=CARTESIAN_POINT('Ctrl Pts',(54.796585406383,18.5566021327055,16.1472239924538));
#38622=CARTESIAN_POINT('Ctrl Pts',(54.7154929205828,18.5647112430706,16.1430078329994));
#38623=CARTESIAN_POINT('Ctrl Pts',(54.6350045842893,18.5768350042743,16.1387916735449));
#38624=CARTESIAN_POINT('Ctrl Pts',(54.5545181658697,18.5889584765934,16.134575614553));
#38625=CARTESIAN_POINT('Ctrl Pts',(54.4746363279049,18.6050963392071,16.1303595555611));
#38626=CARTESIAN_POINT('Ctrl Pts',(54.3957833328088,18.6251584328448,16.1261434965692));
#38627=CARTESIAN_POINT('Ctrl Pts',(54.316284875567,18.645384747537,16.1218929264408));
#38628=CARTESIAN_POINT('Ctrl Pts',(54.2378326512754,18.6695997317385,16.1176423563123));
#38629=CARTESIAN_POINT('Ctrl Pts',(54.1608464531326,18.6976595441204,16.1133917861838));
#38630=CARTESIAN_POINT('Ctrl Pts',(54.084374298409,18.7255319987389,16.1091695974751));
#38631=CARTESIAN_POINT('Ctrl Pts',(54.0093490604099,18.757197853887,16.1049474087663));
#38632=CARTESIAN_POINT('Ctrl Pts',(53.9361609214986,18.79246819614,16.1007252200576));
#38633=CARTESIAN_POINT('Ctrl Pts',(53.862234830035,18.8280941675903,16.0964604592192));
#38634=CARTESIAN_POINT('Ctrl Pts',(53.7901835194177,18.8673974903808,16.0921956983809));
#38635=CARTESIAN_POINT('Ctrl Pts',(53.7203808197885,18.9101375634662,16.0879309375426));
#38636=CARTESIAN_POINT('Ctrl Pts',(53.6505781201594,18.9528776365517,16.0836661767042));
#38637=CARTESIAN_POINT('Ctrl Pts',(53.5830243930152,18.9990541350055,16.0794014158659));
#38638=CARTESIAN_POINT('Ctrl Pts',(53.5180592965164,19.0483847711809,16.0751366550276));
#38639=CARTESIAN_POINT('Ctrl Pts',(53.4542839150827,19.09681200839,16.0709499953619));
#38640=CARTESIAN_POINT('Ctrl Pts',(53.3927529352554,19.1484689909858,16.0667633356962));
#38641=CARTESIAN_POINT('Ctrl Pts',(53.3338170830797,19.2031180513559,16.0625766760305));
#38642=CARTESIAN_POINT('Ctrl Pts',(53.2723770701508,19.2600891284123,16.0582121268725));
#38643=CARTESIAN_POINT('Ctrl Pts',(53.2137581038291,19.3203119934272,16.0538475777146));
#38644=CARTESIAN_POINT('Ctrl Pts',(53.1583232212213,19.3834676333252,16.0494830285566));
#38645=CARTESIAN_POINT('Ctrl Pts',(53.1052868869398,19.443890664309,16.045307324068));
#38646=CARTESIAN_POINT('Ctrl Pts',(53.0551651738979,19.5069975449245,16.0411316195794));
#38647=CARTESIAN_POINT('Ctrl Pts',(53.0082400431393,19.5724697816697,16.0369559150908));
#38648=CARTESIAN_POINT('Ctrl Pts',(52.9613429297233,19.6379029272486,16.0327827037682));
#38649=CARTESIAN_POINT('Ctrl Pts',(52.9176388882398,19.7056982411438,16.0286094924457));
#38650=CARTESIAN_POINT('Ctrl Pts',(52.8773691903924,19.7755047178104,16.0244362811231));
#38651=CARTESIAN_POINT('Ctrl Pts',(52.837110562581,19.8452920048568,16.0202642170056));
#38652=CARTESIAN_POINT('Ctrl Pts',(52.8002846413469,19.9170889450323,16.0160921528881));
#38653=CARTESIAN_POINT('Ctrl Pts',(52.767088143579,19.9905175130521,16.0119200887706));
#38654=CARTESIAN_POINT('Ctrl Pts',(52.7338900768914,20.0639495514237,16.0077478274746));
#38655=CARTESIAN_POINT('Ctrl Pts',(52.704321967636,20.1390129361383,16.0035755661786));
#38656=CARTESIAN_POINT('Ctrl Pts',(52.6785328728113,20.215308578241,15.9994033048827));
#38657=CARTESIAN_POINT('Ctrl Pts',(52.6527194470096,20.291676202223,15.9952271072255));
#38658=CARTESIAN_POINT('Ctrl Pts',(52.6306923017233,20.3692779518662,15.9910509095682));
#38659=CARTESIAN_POINT('Ctrl Pts',(52.6125507009076,20.4476992718971,15.986874711911));
#38660=CARTESIAN_POINT('Ctrl Pts',(52.5943989802482,20.5261643373231,15.9826961846652));
#38661=CARTESIAN_POINT('Ctrl Pts',(52.5801371996134,20.605449414732,15.9785176574193));
#38662=CARTESIAN_POINT('Ctrl Pts',(52.5698131067276,20.6851319105291,15.9743391301735));
#38663=CARTESIAN_POINT('Ctrl Pts',(52.5594734701288,20.7649343744304,15.9701543118346));
#38664=CARTESIAN_POINT('Ctrl Pts',(52.5530833841282,20.8451349771926,15.9659694934957));
#38665=CARTESIAN_POINT('Ctrl Pts',(52.5506385518353,20.9253089948896,15.9617846751568));
#38666=CARTESIAN_POINT('Ctrl Pts',(52.5498679378346,20.9505799391215,15.9604656155176));
#38667=CARTESIAN_POINT('Ctrl Pts',(52.5494889034741,20.9758482693652,15.9591465558783));
#38668=CARTESIAN_POINT('Ctrl Pts',(52.5495002472464,21.0011007971719,15.957827496239));
#38669=CARTESIAN_POINT('',(52.5495010097513,20.9977754123675,15.1578274961792));
#38670=CARTESIAN_POINT('Ctrl Pts',(52.5495002472466,21.0011007976877,15.9578274962121));
#38671=CARTESIAN_POINT('Ctrl Pts',(52.5495281227704,21.0631548561835,15.9545861175809));
#38672=CARTESIAN_POINT('Ctrl Pts',(52.5519128814938,21.1251536128192,15.9513447389498));
#38673=CARTESIAN_POINT('Ctrl Pts',(52.5566432426686,21.1869706030453,15.9481033603187));
#38674=CARTESIAN_POINT('Ctrl Pts',(52.562818146168,21.2676650648772,15.9438721400138));
#38675=CARTESIAN_POINT('Ctrl Pts',(52.573006453828,21.348204593641,15.9396409197089));
#38676=CARTESIAN_POINT('Ctrl Pts',(52.5871943956603,21.4281581082579,15.935409699404));
#38677=CARTESIAN_POINT('Ctrl Pts',(52.601361992977,21.5079969751308,15.9311845463729));
#38678=CARTESIAN_POINT('Ctrl Pts',(52.6195177533904,21.5872510428542,15.9269593933418));
#38679=CARTESIAN_POINT('Ctrl Pts',(52.6415960399012,21.6654930585591,15.9227342403107));
#38680=CARTESIAN_POINT('Ctrl Pts',(52.6637310446412,21.7439360748525,15.9184982330315));
#38681=CARTESIAN_POINT('Ctrl Pts',(52.6898087124821,21.8213613624831,15.9142622257523));
#38682=CARTESIAN_POINT('Ctrl Pts',(52.7197110011918,21.8973473864198,15.9100262184731));
#38683=CARTESIAN_POINT('Ctrl Pts',(52.7494830126794,21.9730023571645,15.9058086664789));
#38684=CARTESIAN_POINT('Ctrl Pts',(52.783046224873,22.0472301407583,15.9015911144848));
#38685=CARTESIAN_POINT('Ctrl Pts',(52.8202344121191,22.1196303996811,15.8973735624906));
#38686=CARTESIAN_POINT('Ctrl Pts',(52.8574103206717,22.1920067536854,15.8931574030361));
#38687=CARTESIAN_POINT('Ctrl Pts',(52.8982086151773,22.2625563680684,15.8889412435817));
#38688=CARTESIAN_POINT('Ctrl Pts',(52.9424161069486,22.3309014888622,15.8847250841272));
#38689=CARTESIAN_POINT('Ctrl Pts',(52.986622545345,22.3992449811302,15.8805090251353));
#38690=CARTESIAN_POINT('Ctrl Pts',(53.0342377660559,22.4653836944759,15.8762929661434));
#38691=CARTESIAN_POINT('Ctrl Pts',(53.0850048247631,22.5289681909115,15.8720769071515));
#38692=CARTESIAN_POINT('Ctrl Pts',(53.1361874442819,22.5930731670759,15.867826337023));
#38693=CARTESIAN_POINT('Ctrl Pts',(53.1905734528108,22.6545815326246,15.8635757668945));
#38694=CARTESIAN_POINT('Ctrl Pts',(53.2478588328643,22.7131700383874,15.859325196766));
#38695=CARTESIAN_POINT('Ctrl Pts',(53.3047617135433,22.7713673436941,15.8551030080572));
#38696=CARTESIAN_POINT('Ctrl Pts',(53.364524978402,22.8266833892191,15.8508808193484));
#38697=CARTESIAN_POINT('Ctrl Pts',(53.4268157402014,22.878840476124,15.8466586306396));
#38698=CARTESIAN_POINT('Ctrl Pts',(53.4897345768136,22.9315234604758,15.8423938698013));
#38699=CARTESIAN_POINT('Ctrl Pts',(53.5552317788347,22.9809831316379,15.8381291089629));
#38700=CARTESIAN_POINT('Ctrl Pts',(53.6229340988568,23.026977985551,15.8338643481245));
#38701=CARTESIAN_POINT('Ctrl Pts',(53.6906364188788,23.0729728394642,15.8295995872862));
#38702=CARTESIAN_POINT('Ctrl Pts',(53.7605434118993,23.1155026806039,15.8253348264478));
#38703=CARTESIAN_POINT('Ctrl Pts',(53.8322579247294,23.1543743165111,15.8210700656095));
#38704=CARTESIAN_POINT('Ctrl Pts',(53.9034084333622,23.1929402435047,15.8168388453045));
#38705=CARTESIAN_POINT('Ctrl Pts',(53.9766049171274,23.2280499582696,15.8126076249996));
#38706=CARTESIAN_POINT('Ctrl Pts',(54.0514777000664,23.2594812892628,15.8083764046947));
#38707=CARTESIAN_POINT('Ctrl Pts',(54.1262431206751,23.2908675499273,15.8041512516635));
#38708=CARTESIAN_POINT('Ctrl Pts',(54.2026796414736,23.3185857240215,15.7999260986323));
#38709=CARTESIAN_POINT('Ctrl Pts',(54.2803926796746,23.3424592962385,15.7957009456012));
#38710=CARTESIAN_POINT('Ctrl Pts',(54.3583053595421,23.3663941987014,15.791464938322));
#38711=CARTESIAN_POINT('Ctrl Pts',(54.4375007058176,23.3864645014641,15.7872289310428));
#38712=CARTESIAN_POINT('Ctrl Pts',(54.517560524782,23.4025408222861,15.7829929237636));
#38713=CARTESIAN_POINT('Ctrl Pts',(54.59727154199,23.4185471023685,15.7787753717694));
#38714=CARTESIAN_POINT('Ctrl Pts',(54.6778390578833,23.4305940294786,15.7745578197753));
#38715=CARTESIAN_POINT('Ctrl Pts',(54.7588365635377,23.4386042005446,15.7703402677811));
#38716=CARTESIAN_POINT('Ctrl Pts',(54.8398073256583,23.4466117268343,15.7661241083267));
#38717=CARTESIAN_POINT('Ctrl Pts',(54.9212073333003,23.450585098204,15.7619079488723));
#38718=CARTESIAN_POINT('Ctrl Pts',(55.0026035886565,23.450498616879,15.7576917894179));
#38719=CARTESIAN_POINT('Ctrl Pts',(55.0839979045049,23.4504121376148,15.753475730426));
#38720=CARTESIAN_POINT('Ctrl Pts',(55.1653880033248,23.4462659995988,15.7492596714341));
#38721=CARTESIAN_POINT('Ctrl Pts',(55.2463409541387,23.4380866236281,15.7450436124422));
#38722=CARTESIAN_POINT('Ctrl Pts',(55.3279565565775,23.429840294239,15.7407930423138));
#38723=CARTESIAN_POINT('Ctrl Pts',(55.4091273424047,23.4174944251171,15.7365424721853));
#38724=CARTESIAN_POINT('Ctrl Pts',(55.4894168613141,23.4011291897483,15.7322919020569));
#38725=CARTESIAN_POINT('Ctrl Pts',(55.5691702802496,23.3848732264536,15.7280697133481));
#38726=CARTESIAN_POINT('Ctrl Pts',(55.6480537255664,23.3646515852234,15.7238475246394));
#38727=CARTESIAN_POINT('Ctrl Pts',(55.7256533661477,23.3405933953163,15.7196253359306));
#38728=CARTESIAN_POINT('Ctrl Pts',(55.8040354402445,23.3162926278153,15.7153605750923));
#38729=CARTESIAN_POINT('Ctrl Pts',(55.8811072186142,23.2880776756983,15.711095814254));
#38730=CARTESIAN_POINT('Ctrl Pts',(55.956463398109,23.256131205865,15.7068310534157));
#38731=CARTESIAN_POINT('Ctrl Pts',(56.0318195776037,23.2241847360317,15.7025662925774));
#38732=CARTESIAN_POINT('Ctrl Pts',(56.1054597526467,23.1885070163714,15.698301531739));
#38733=CARTESIAN_POINT('Ctrl Pts',(56.1770062509688,23.1493269958711,15.6940367709007));
#38734=CARTESIAN_POINT('Ctrl Pts',(56.2479900664563,23.1104551095984,15.6898055505958));
#38735=CARTESIAN_POINT('Ctrl Pts',(56.3171792225727,23.0679900889066,15.6855743302909));
#38736=CARTESIAN_POINT('Ctrl Pts',(56.3841865965516,23.0221220823498,15.6813431099859));
#38737=CARTESIAN_POINT('Ctrl Pts',(56.4510978866461,22.9763198473042,15.6771179569548));
#38738=CARTESIAN_POINT('Ctrl Pts',(56.5158332276734,22.9271245781314,15.6728928039236));
#38739=CARTESIAN_POINT('Ctrl Pts',(56.578030353825,22.8747721067925,15.6686676508925));
#38740=CARTESIAN_POINT('Ctrl Pts',(56.6403872618897,22.8222851440622,15.6644316436133));
#38741=CARTESIAN_POINT('Ctrl Pts',(56.7001924863258,22.7666249692974,15.6601956363341));
#38742=CARTESIAN_POINT('Ctrl Pts',(56.7571105618316,22.7080728097771,15.6559596290549));
#38743=CARTESIAN_POINT('Ctrl Pts',(56.8137806587014,22.6497757482116,15.6517420770607));
#38744=CARTESIAN_POINT('Ctrl Pts',(56.8675883794462,22.5886121785131,15.6475245250666));
#38745=CARTESIAN_POINT('Ctrl Pts',(56.9182374248148,22.5248984989303,15.6433069730724));
#38746=CARTESIAN_POINT('Ctrl Pts',(56.9688697470208,22.461205856155,15.639090813618));
#38747=CARTESIAN_POINT('Ctrl Pts',(57.0163451758642,22.3949651392182,15.6348746541635));
#38748=CARTESIAN_POINT('Ctrl Pts',(57.0604073382992,22.3265262342987,15.6306584947091));
#38749=CARTESIAN_POINT('Ctrl Pts',(57.1044684508222,22.2580889601396,15.6264424357172));
#38750=CARTESIAN_POINT('Ctrl Pts',(57.1451162079009,22.187453993651,15.6222263767253));
#38751=CARTESIAN_POINT('Ctrl Pts',(57.1821380645935,22.1149994246869,15.6180103177334));
#38752=CARTESIAN_POINT('Ctrl Pts',(57.2194629688372,22.0419517687831,15.6137597476049));
#38753=CARTESIAN_POINT('Ctrl Pts',(57.2531021055102,21.9670550035654,15.6095091774764));
#38754=CARTESIAN_POINT('Ctrl Pts',(57.2828861863247,21.8907193218338,15.6052586073479));
#38755=CARTESIAN_POINT('Ctrl Pts',(57.3124713962881,21.8148933399678,15.6010364186392));
#38756=CARTESIAN_POINT('Ctrl Pts',(57.3382527846846,21.7376480635334,15.5968142299304));
#38757=CARTESIAN_POINT('Ctrl Pts',(57.3601144622165,21.6594012247765,15.5925920412216));
#38758=CARTESIAN_POINT('Ctrl Pts',(57.3821965700116,21.5803654268354,15.5883272803833));
#38759=CARTESIAN_POINT('Ctrl Pts',(57.4002793704857,21.5003082293385,15.584062519545));
#38760=CARTESIAN_POINT('Ctrl Pts',(57.4142965826117,21.4196692283088,15.5797977587066));
#38761=CARTESIAN_POINT('Ctrl Pts',(57.4283137947378,21.3390302272791,15.5755329978683));
#38762=CARTESIAN_POINT('Ctrl Pts',(57.4382654236932,21.2578099087519,15.5712682370299));
#38763=CARTESIAN_POINT('Ctrl Pts',(57.4441390583637,21.176449747467,15.5670034761916));
#38764=CARTESIAN_POINT('Ctrl Pts',(57.4499664993911,21.0957294493094,15.5627722558867));
#38765=CARTESIAN_POINT('Ctrl Pts',(57.4518017582841,21.01456881149,15.5585410355817));
#38766=CARTESIAN_POINT('Ctrl Pts',(57.4495946981662,20.9333962109485,15.5543098152768));
#38767=CARTESIAN_POINT('Ctrl Pts',(57.4473908028181,20.8523400062349,15.5500846622456));
#38768=CARTESIAN_POINT('Ctrl Pts',(57.4411561130793,20.7712723336967,15.5458595092145));
#38769=CARTESIAN_POINT('Ctrl Pts',(57.430892354873,20.6906254551192,15.5416343561833));
#38770=CARTESIAN_POINT('Ctrl Pts',(57.420602229485,20.6097713979573,15.5373983489041));
#38771=CARTESIAN_POINT('Ctrl Pts',(57.4062622805198,20.5293407707785,15.5331623416249));
#38772=CARTESIAN_POINT('Ctrl Pts',(57.3879269084726,20.4497679309669,15.5289263343457));
#38773=CARTESIAN_POINT('Ctrl Pts',(57.3696714193187,20.3705417712585,15.5247087823516));
#38774=CARTESIAN_POINT('Ctrl Pts',(57.3474553457982,20.2921663979111,15.5204912303574));
#38775=CARTESIAN_POINT('Ctrl Pts',(57.3213838769868,20.2150623300758,15.5162736783633));
#38776=CARTESIAN_POINT('Ctrl Pts',(57.2953210163812,20.1379837202497,15.5120575189089));
#38777=CARTESIAN_POINT('Ctrl Pts',(57.2654054372177,20.0621760224383,15.5078413594544));
#38778=CARTESIAN_POINT('Ctrl Pts',(57.2317921151758,19.9880443662694,15.5036252));
#38779=CARTESIAN_POINT('Ctrl Pts',(57.1981795940713,19.9139144765077,15.4994091410081));
#38780=CARTESIAN_POINT('Ctrl Pts',(57.1608696982766,19.8414609719537,15.4951930820162));
#38781=CARTESIAN_POINT('Ctrl Pts',(57.1200648657519,19.7710674489606,15.4909770230243));
#38782=CARTESIAN_POINT('Ctrl Pts',(57.0789260196019,19.7000977100059,15.4867264528958));
#38783=CARTESIAN_POINT('Ctrl Pts',(57.0342349827378,19.6312222558862,15.4824758827674));
#38784=CARTESIAN_POINT('Ctrl Pts',(56.9862446218527,19.5648057441025,15.4782253126389));
#38785=CARTESIAN_POINT('Ctrl Pts',(56.9385746967054,19.4988327010396,15.4740031239302));
#38786=CARTESIAN_POINT('Ctrl Pts',(56.8876497149417,19.435286190896,15.4697809352214));
#38787=CARTESIAN_POINT('Ctrl Pts',(56.8337578322622,19.3744900915045,15.4655587465127));
#38788=CARTESIAN_POINT('Ctrl Pts',(56.7793225602719,19.3130809879107,15.4612939856743));
#38789=CARTESIAN_POINT('Ctrl Pts',(56.721860560484,19.254478418646,15.457029224836));
#38790=CARTESIAN_POINT('Ctrl Pts',(56.6617052580061,19.1989764339368,15.4527644639977));
#38791=CARTESIAN_POINT('Ctrl Pts',(56.6015499555282,19.1434744492277,15.4484997031593));
#38792=CARTESIAN_POINT('Ctrl Pts',(56.5387017615516,19.0910733082628,15.444234942321));
#38793=CARTESIAN_POINT('Ctrl Pts',(56.4735248891911,19.042022816544,15.4399701814827));
#38794=CARTESIAN_POINT('Ctrl Pts',(56.4088606052612,18.9933580861183,15.4357389611778));
#38795=CARTESIAN_POINT('Ctrl Pts',(56.3416616840414,18.9478089665511,15.4315077408728));
#38796=CARTESIAN_POINT('Ctrl Pts',(56.2722608776796,18.9056498599504,15.4272765205679));
#38797=CARTESIAN_POINT('Ctrl Pts',(56.2029595872167,18.8635512065578,15.4230513675368));
#38798=CARTESIAN_POINT('Ctrl Pts',(56.131463076343,18.8248331510826,15.4188262145056));
#38799=CARTESIAN_POINT('Ctrl Pts',(56.0581354825333,18.7897286251222,15.4146010614744));
#38800=CARTESIAN_POINT('Ctrl Pts',(55.9846195130871,18.7545339170479,15.4103650541952));
#38801=CARTESIAN_POINT('Ctrl Pts',(55.9092634217106,18.7229716069748,15.4061290469161));
#38802=CARTESIAN_POINT('Ctrl Pts',(55.8324616679782,18.6952315037412,15.4018930396369));
#38803=CARTESIAN_POINT('Ctrl Pts',(55.7559945213801,18.6676122575975,15.3976754876427));
#38804=CARTESIAN_POINT('Ctrl Pts',(55.6780947202454,18.6437821494739,15.3934579356486));
#38805=CARTESIAN_POINT('Ctrl Pts',(55.599172635453,18.6238808104549,15.3892403836544));
#38806=CARTESIAN_POINT('Ctrl Pts',(55.5202766089375,18.6039860424054,15.3850242242));
#38807=CARTESIAN_POINT('Ctrl Pts',(55.4403594195168,18.5880175810119,15.3808080647455));
#38808=CARTESIAN_POINT('Ctrl Pts',(55.3598455026322,18.5760648803577,15.3765919052911));
#38809=CARTESIAN_POINT('Ctrl Pts',(55.2793335042311,18.5641124645121,15.3723758462992));
#38810=CARTESIAN_POINT('Ctrl Pts',(55.1982252666811,18.5561756863297,15.3681597873073));
#38811=CARTESIAN_POINT('Ctrl Pts',(55.1169528674894,18.5522924445951,15.3639437283154));
#38812=CARTESIAN_POINT('Ctrl Pts',(55.0350152017837,18.5483774160459,15.3596931581869));
#38813=CARTESIAN_POINT('Ctrl Pts',(54.9529111529,18.5485826307513,15.3554425880585));
#38814=CARTESIAN_POINT('Ctrl Pts',(54.8710842288119,18.5528933464315,15.35119201793));
#38815=CARTESIAN_POINT('Ctrl Pts',(54.7898036700836,18.5571752790951,15.3469698292212));
#38816=CARTESIAN_POINT('Ctrl Pts',(54.7087970073659,18.565507944601,15.3427476405125));
#38817=CARTESIAN_POINT('Ctrl Pts',(54.6284926185837,18.5778248379704,15.3385254518037));
#38818=CARTESIAN_POINT('Ctrl Pts',(54.5473785244376,18.5902659219946,15.3342606909654));
#38819=CARTESIAN_POINT('Ctrl Pts',(54.4669814217996,18.6067719339737,15.3299959301271));
#38820=CARTESIAN_POINT('Ctrl Pts',(54.3877291724453,18.6272221587925,15.3257311692887));
#38821=CARTESIAN_POINT('Ctrl Pts',(54.308476923091,18.6476723836113,15.3214664084504));
#38822=CARTESIAN_POINT('Ctrl Pts',(54.2303699677568,18.6720666163101,15.3172016476121));
#38823=CARTESIAN_POINT('Ctrl Pts',(54.1538156861656,18.7002342821451,15.3129368867737));
#38824=CARTESIAN_POINT('Ctrl Pts',(54.0778634714983,18.7281804212468,15.3087056664688));
#38825=CARTESIAN_POINT('Ctrl Pts',(54.0031547675905,18.7599456044963,15.3044744461639));
#38826=CARTESIAN_POINT('Ctrl Pts',(53.9301005622805,18.7953990285842,15.300243225859));
#38827=CARTESIAN_POINT('Ctrl Pts',(53.8571511115877,18.8308016149434,15.2960180728278));
#38828=CARTESIAN_POINT('Ctrl Pts',(53.7858518623981,18.8698817371529,15.2917929197966));
#38829=CARTESIAN_POINT('Ctrl Pts',(53.7165959753696,18.9124597346249,15.2875677667655));
#38830=CARTESIAN_POINT('Ctrl Pts',(53.6471621727555,18.9551471132582,15.2833317594863));
#38831=CARTESIAN_POINT('Ctrl Pts',(53.5797826851319,19.0013501929421,15.2790957522071));
#38832=CARTESIAN_POINT('Ctrl Pts',(53.5148308811937,19.0508404532866,15.2748597449279));
#38833=CARTESIAN_POINT('Ctrl Pts',(53.4501620569523,19.1001150962345,15.2706421929337));
#38834=CARTESIAN_POINT('Ctrl Pts',(53.3879001839283,19.1526480595771,15.2664246409396));
#38835=CARTESIAN_POINT('Ctrl Pts',(53.3283850971496,19.2081702462096,15.2622070889454));
#38836=CARTESIAN_POINT('Ctrl Pts',(53.2688896608987,19.2636741006792,15.257990929491));
#38837=CARTESIAN_POINT('Ctrl Pts',(53.2121395495531,19.3221649015494,15.2537747700365));
#38838=CARTESIAN_POINT('Ctrl Pts',(53.1584400637624,19.3833345271069,15.2495586105821));
#38839=CARTESIAN_POINT('Ctrl Pts',(53.1047418575217,19.4445026951162,15.2453425515902));
#38840=CARTESIAN_POINT('Ctrl Pts',(53.0540944381981,19.5083492107785,15.2411264925983));
#38841=CARTESIAN_POINT('Ctrl Pts',(53.0067639315506,19.5745315768379,15.2369104336064));
#38842=CARTESIAN_POINT('Ctrl Pts',(52.9590459944656,19.6412556878489,15.2326598634779));
#38843=CARTESIAN_POINT('Ctrl Pts',(52.91469981491,19.7103536857576,15.2284092933495));
#38844=CARTESIAN_POINT('Ctrl Pts',(52.8739534856068,19.781444925891,15.224158723221));
#38845=CARTESIAN_POINT('Ctrl Pts',(52.8334792230239,19.8520614837433,15.2199365345122));
#38846=CARTESIAN_POINT('Ctrl Pts',(52.7965570418537,19.9246443002822,15.2157143458035));
#38847=CARTESIAN_POINT('Ctrl Pts',(52.7633633381258,19.9987973767712,15.2114921570947));
#38848=CARTESIAN_POINT('Ctrl Pts',(52.729834943849,20.0736981352324,15.2072273962564));
#38849=CARTESIAN_POINT('Ctrl Pts',(52.7001108142751,20.1502005447704,15.2029626354181));
#38850=CARTESIAN_POINT('Ctrl Pts',(52.6743215162923,20.2278796464157,15.1986978745797));
#38851=CARTESIAN_POINT('Ctrl Pts',(52.6485322183096,20.3055587480609,15.1944331137414));
#38852=CARTESIAN_POINT('Ctrl Pts',(52.6266778186805,20.3844140603575,15.190168352903));
#38853=CARTESIAN_POINT('Ctrl Pts',(52.6088358846536,20.4640107991018,15.1859035920647));
#38854=CARTESIAN_POINT('Ctrl Pts',(52.5846673824411,20.5718317311566,15.1801265904459));
#38855=CARTESIAN_POINT('Ctrl Pts',(52.5677836834025,20.6813408102256,15.174349588827));
#38856=CARTESIAN_POINT('Ctrl Pts',(52.558368406975,20.7917083440411,15.1685725872082));
#38857=CARTESIAN_POINT('Ctrl Pts',(52.5525310073086,20.8601353743076,15.1649908902095));
#38858=CARTESIAN_POINT('Ctrl Pts',(52.549563542799,20.9288920271857,15.1614091932108));
#38859=CARTESIAN_POINT('Ctrl Pts',(52.5495010097519,20.9977754117357,15.1578274962121));
#38860=CARTESIAN_POINT('',(52.5495000127026,21.0002495104095,14.357827496162));
#38861=CARTESIAN_POINT('Ctrl Pts',(52.5495010097513,20.9977754123675,15.1578274961792));
#38862=CARTESIAN_POINT('Ctrl Pts',(52.5494282960771,21.0778733067042,15.1536626835815));
#38863=CARTESIAN_POINT('Ctrl Pts',(52.5532869724308,21.1580880860891,15.1494978709838));
#38864=CARTESIAN_POINT('Ctrl Pts',(52.561084728881,21.237996954398,15.1453330583861));
#38865=CARTESIAN_POINT('Ctrl Pts',(52.5688767052554,21.3178465903721,15.1411713329498));
#38866=CARTESIAN_POINT('Ctrl Pts',(52.5806019247079,21.3973902904168,15.1370096075135));
#38867=CARTESIAN_POINT('Ctrl Pts',(52.5962160347525,21.476206781156,15.1328478820771));
#38868=CARTESIAN_POINT('Ctrl Pts',(52.611823660692,21.5549905416011,15.1286878848895));
#38869=CARTESIAN_POINT('Ctrl Pts',(52.6313168800144,21.6330472229495,15.1245278877019));
#38870=CARTESIAN_POINT('Ctrl Pts',(52.6545998963697,21.7099638046343,15.1203678905143));
#38871=CARTESIAN_POINT('Ctrl Pts',(52.6778808328632,21.7868735153944,15.1162082649374));
#38872=CARTESIAN_POINT('Ctrl Pts',(52.7049507542299,21.8626428709612,15.1120486393605));
#38873=CARTESIAN_POINT('Ctrl Pts',(52.735663910154,21.936873695981,15.1078890137836));
#38874=CARTESIAN_POINT('Ctrl Pts',(52.7664052381512,22.0111726102662,15.1037255727318));
#38875=CARTESIAN_POINT('Ctrl Pts',(52.8007962928464,22.083929731569,15.09956213168));
#38876=CARTESIAN_POINT('Ctrl Pts',(52.8386433136779,22.1547673031788,15.0953986906283));
#38877=CARTESIAN_POINT('Ctrl Pts',(52.8765069502239,22.2256359741152,15.0912334217299));
#38878=CARTESIAN_POINT('Ctrl Pts',(52.917829326728,22.2945830068287,15.0870681528315));
#38879=CARTESIAN_POINT('Ctrl Pts',(52.9623722310994,22.3612579936974,15.0829028839331));
#38880=CARTESIAN_POINT('Ctrl Pts',(53.0069942770859,22.4280514453636,15.0787302143923));
#38881=CARTESIAN_POINT('Ctrl Pts',(53.0548479948803,22.4925644025959,15.0745575448515));
#38882=CARTESIAN_POINT('Ctrl Pts',(53.105653842797,22.5544783326538,15.0703848753107));
#38883=CARTESIAN_POINT('Ctrl Pts',(53.1523871463164,22.6114293059004,15.066546682659));
#38884=CARTESIAN_POINT('Ctrl Pts',(53.2016176127437,22.6661814128854,15.0627084900074));
#38885=CARTESIAN_POINT('Ctrl Pts',(53.2531015155089,22.7185156196214,15.0588702973557));
#38886=CARTESIAN_POINT('Ctrl Pts',(53.3098573259975,22.776208804482,15.0546390770508));
#38887=CARTESIAN_POINT('Ctrl Pts',(53.3695806882398,22.8311955056827,15.0504078567458));
#38888=CARTESIAN_POINT('Ctrl Pts',(53.4319830925651,22.8831551258455,15.0461766364409));
#38889=CARTESIAN_POINT('Ctrl Pts',(53.49429601621,22.9350402395496,15.0419514834098));
#38890=CARTESIAN_POINT('Ctrl Pts',(53.559279998046,22.9839065980349,15.0377263303786));
#38891=CARTESIAN_POINT('Ctrl Pts',(53.6266093548769,23.029469976592,15.0335011773475));
#38892=CARTESIAN_POINT('Ctrl Pts',(53.6941116781151,23.0751504056344,15.0292651700683));
#38893=CARTESIAN_POINT('Ctrl Pts',(53.7639711065245,23.1175105305989,15.0250291627891));
#38894=CARTESIAN_POINT('Ctrl Pts',(53.8358255905565,23.1563042907709,15.0207931555099));
#38895=CARTESIAN_POINT('Ctrl Pts',(53.9073670215419,23.1949290356757,15.0165756035157));
#38896=CARTESIAN_POINT('Ctrl Pts',(53.9808857526134,23.2300181971312,15.0123580515216));
#38897=CARTESIAN_POINT('Ctrl Pts',(54.0559965767771,23.2613729871349,15.0081404995274));
#38898=CARTESIAN_POINT('Ctrl Pts',(54.1310826010555,23.2927174245003,15.003924340073));
#38899=CARTESIAN_POINT('Ctrl Pts',(54.2077592458107,23.3203297600269,14.9997081806186));
#38900=CARTESIAN_POINT('Ctrl Pts',(54.2856199731486,23.3440587508072,14.9954920211641));
#38901=CARTESIAN_POINT('Ctrl Pts',(54.3634788452231,23.3677871761737,14.9912759621722));
#38902=CARTESIAN_POINT('Ctrl Pts',(54.4425212987326,23.3876323062963,14.9870599031803));
#38903=CARTESIAN_POINT('Ctrl Pts',(54.5223256129035,23.4034927563677,14.9828438441884));
#38904=CARTESIAN_POINT('Ctrl Pts',(54.6027831763745,23.4194830343565,14.9785932740599));
#38905=CARTESIAN_POINT('Ctrl Pts',(54.6840146633237,23.4314229876311,14.9743427039315));
#38906=CARTESIAN_POINT('Ctrl Pts',(54.7655792627784,23.4392616030185,14.970092133803));
#38907=CARTESIAN_POINT('Ctrl Pts',(54.8465992484373,23.4470478793016,14.9658699450943));
#38908=CARTESIAN_POINT('Ctrl Pts',(54.9279474398575,23.4507874610616,14.9616477563855));
#38909=CARTESIAN_POINT('Ctrl Pts',(55.0091903341992,23.4504827662641,14.9574255676768));
#38910=CARTESIAN_POINT('Ctrl Pts',(55.0912523968123,23.4501749992433,14.9531608068384));
#38911=CARTESIAN_POINT('Ctrl Pts',(55.1732065418967,23.4457409663673,14.9488960460001));
#38912=CARTESIAN_POINT('Ctrl Pts',(55.2546117595896,23.4372367759163,14.9446312851617));
#38913=CARTESIAN_POINT('Ctrl Pts',(55.3360169772825,23.4287325854653,14.9403665243234));
#38914=CARTESIAN_POINT('Ctrl Pts',(55.4168728013817,23.4161583749615,14.9361017634851));
#38915=CARTESIAN_POINT('Ctrl Pts',(55.496751104762,23.3996225932254,14.9318370026467));
#38916=CARTESIAN_POINT('Ctrl Pts',(55.5760011991983,23.3832168583924,14.9276057823418));
#38917=CARTESIAN_POINT('Ctrl Pts',(55.6545862816944,23.3628501670674,14.9233745620369));
#38918=CARTESIAN_POINT('Ctrl Pts',(55.7320805387498,23.3385911003816,14.919143341732));
#38919=CARTESIAN_POINT('Ctrl Pts',(55.8094636744645,23.3143668194994,14.9149181887008));
#38920=CARTESIAN_POINT('Ctrl Pts',(55.8857586513455,23.2862613860456,14.9106930356696));
#38921=CARTESIAN_POINT('Ctrl Pts',(55.9605500611977,23.2543943377176,14.9064678826385));
#38922=CARTESIAN_POINT('Ctrl Pts',(56.0355336071709,23.2224454242252,14.9022318753593));
#38923=CARTESIAN_POINT('Ctrl Pts',(56.1090053901096,23.1867156462173,14.8979958680801));
#38924=CARTESIAN_POINT('Ctrl Pts',(56.1805623499266,23.1473757910379,14.8937598608009));
#38925=CARTESIAN_POINT('Ctrl Pts',(56.2518075529398,23.1082073303328,14.8895423088067));
#38926=CARTESIAN_POINT('Ctrl Pts',(56.3211541689651,23.0654604016027,14.8853247568126));
#38927=CARTESIAN_POINT('Ctrl Pts',(56.3882263016474,23.0193508821932,14.8811072048184));
#38928=CARTESIAN_POINT('Ctrl Pts',(56.4552762886373,22.973256587098,14.876891045364));
#38929=CARTESIAN_POINT('Ctrl Pts',(56.5200529008093,22.9238021693007,14.8726748859096));
#38930=CARTESIAN_POINT('Ctrl Pts',(56.5822086247988,22.8712472091127,14.8684587264551));
#38931=CARTESIAN_POINT('Ctrl Pts',(56.6443628677435,22.8186935012029,14.8642426674632));
#38932=CARTESIAN_POINT('Ctrl Pts',(56.7038959923662,22.7630396988257,14.8600266084713));
#38933=CARTESIAN_POINT('Ctrl Pts',(56.7604941453531,22.7045851736353,14.8558105494794));
#38934=CARTESIAN_POINT('Ctrl Pts',(56.817555590384,22.6456521608086,14.8515599793509));
#38935=CARTESIAN_POINT('Ctrl Pts',(56.871633447534,22.5838726955937,14.8473094092225));
#38936=CARTESIAN_POINT('Ctrl Pts',(56.9224458363955,22.5195895025058,14.843058839094));
#38937=CARTESIAN_POINT('Ctrl Pts',(56.9729189465974,22.4557355337875,14.8388366503853));
#38938=CARTESIAN_POINT('Ctrl Pts',(57.0201698412542,22.3894115888414,14.8346144616765));
#38939=CARTESIAN_POINT('Ctrl Pts',(57.06396549732,22.3209832231608,14.8303922729677));
#38940=CARTESIAN_POINT('Ctrl Pts',(57.1082027429201,22.251864897497,14.8261275121294));
#38941=CARTESIAN_POINT('Ctrl Pts',(57.1489144387557,22.1805998965061,14.8218627512911));
#38942=CARTESIAN_POINT('Ctrl Pts',(57.1859086038108,22.1075891954087,14.8175979904528));
#38943=CARTESIAN_POINT('Ctrl Pts',(57.2229027688658,22.0345784943113,14.8133332296144));
#38944=CARTESIAN_POINT('Ctrl Pts',(57.2561792659063,21.9598225593947,14.8090684687761));
#38945=CARTESIAN_POINT('Ctrl Pts',(57.2855970775908,21.8837399215314,14.8048037079378));
#38946=CARTESIAN_POINT('Ctrl Pts',(57.3147835306757,21.8082556413142,14.8005724876328));
#38947=CARTESIAN_POINT('Ctrl Pts',(57.3402812640153,21.7311824105463,14.7963412673279));
#38948=CARTESIAN_POINT('Ctrl Pts',(57.3619170165232,21.6529151989793,14.792110047023));
#38949=CARTESIAN_POINT('Ctrl Pts',(57.3835217448763,21.5747602171159,14.7878848939918));
#38950=CARTESIAN_POINT('Ctrl Pts',(57.4012753680749,21.4954150991174,14.7836597409607));
#38951=CARTESIAN_POINT('Ctrl Pts',(57.4150530825258,21.4152937015926,14.7794345879295));
#38952=CARTESIAN_POINT('Ctrl Pts',(57.4288661913705,21.3349664754231,14.7751985806503));
#38953=CARTESIAN_POINT('Ctrl Pts',(57.4386827731848,21.2538594187254,14.7709625733711));
#38954=CARTESIAN_POINT('Ctrl Pts',(57.4444277815552,21.172403801469,14.7667265660919));
#38955=CARTESIAN_POINT('Ctrl Pts',(57.4501477602786,21.0913030671333,14.7625090140978));
#38956=CARTESIAN_POINT('Ctrl Pts',(57.4518315282674,21.0098572692345,14.7582914621036));
#38957=CARTESIAN_POINT('Ctrl Pts',(57.449456654091,20.9284993025971,14.7540739101095));
#38958=CARTESIAN_POINT('Ctrl Pts',(57.4470825640441,20.8471681985094,14.749857750655));
#38959=CARTESIAN_POINT('Ctrl Pts',(57.4406525065804,20.7659253324522,14.7456415912006));
#38960=CARTESIAN_POINT('Ctrl Pts',(57.4301961609244,20.68520344756,14.7414254317462));
#38961=CARTESIAN_POINT('Ctrl Pts',(57.419740064422,20.6044834861068,14.7372093727543));
#38962=CARTESIAN_POINT('Ctrl Pts',(57.4052579313016,20.5242849420636,14.7329933137624));
#38963=CARTESIAN_POINT('Ctrl Pts',(57.3868311260961,20.4450338519344,14.7287772547705));
#38964=CARTESIAN_POINT('Ctrl Pts',(57.3682534857167,20.3651340409973,14.724526684642));
#38965=CARTESIAN_POINT('Ctrl Pts',(57.3456663888561,20.2861977374888,14.7202761145136));
#38966=CARTESIAN_POINT('Ctrl Pts',(57.3192049630619,20.2086476200142,14.7160255443851));
#38967=CARTESIAN_POINT('Ctrl Pts',(57.2929202224673,20.1316153112963,14.7118033556763));
#38968=CARTESIAN_POINT('Ctrl Pts',(57.2628129648474,20.0559511470064,14.7075811669676));
#38969=CARTESIAN_POINT('Ctrl Pts',(57.2290639926738,19.9820491335211,14.7033589782588));
#38970=CARTESIAN_POINT('Ctrl Pts',(57.1949747312058,19.9074019695199,14.6990942174205));
#38971=CARTESIAN_POINT('Ctrl Pts',(57.1571701271272,19.8345531228955,14.6948294565822));
#38972=CARTESIAN_POINT('Ctrl Pts',(57.1158829977023,19.7638813204088,14.6905646957438));
#38973=CARTESIAN_POINT('Ctrl Pts',(57.0745958682774,19.6932095179222,14.6862999349055));
#38974=CARTESIAN_POINT('Ctrl Pts',(57.0298265308859,19.6247151277135,14.6820351740672));
#38975=CARTESIAN_POINT('Ctrl Pts',(56.9818501872891,19.5587435741194,14.6777704132288));
#38976=CARTESIAN_POINT('Ctrl Pts',(56.9342511572664,19.4932908587863,14.6735391929239));
#38977=CARTESIAN_POINT('Ctrl Pts',(56.8833169303911,19.4300759725721,14.669307972619));
#38978=CARTESIAN_POINT('Ctrl Pts',(56.8292854282746,19.3694586567946,14.6650767523141));
#38979=CARTESIAN_POINT('Ctrl Pts',(56.7753314035505,19.3089282620052,14.6608515992829));
#38980=CARTESIAN_POINT('Ctrl Pts',(56.7182892310374,19.2509883841845,14.6566264462518));
#38981=CARTESIAN_POINT('Ctrl Pts',(56.6584389764634,19.1959682898167,14.6524012932206));
#38982=CARTESIAN_POINT('Ctrl Pts',(56.5984349689949,19.1408068510414,14.6481652859414));
#38983=CARTESIAN_POINT('Ctrl Pts',(56.5356087161047,19.0885805944986,14.6439292786622));
#38984=CARTESIAN_POINT('Ctrl Pts',(56.4702818942719,19.0395864208346,14.639693271383));
#38985=CARTESIAN_POINT('Ctrl Pts',(56.4052396860006,18.9908057032345,14.6354757193889));
#38986=CARTESIAN_POINT('Ctrl Pts',(56.3377190215193,18.9452292516613,14.6312581673947));
#38987=CARTESIAN_POINT('Ctrl Pts',(56.26807147156,18.9031106388234,14.6270406154005));
#38988=CARTESIAN_POINT('Ctrl Pts',(56.1984469176373,18.8610059325932,14.6228244559461));
#38989=CARTESIAN_POINT('Ctrl Pts',(56.1266972703255,18.8223570382393,14.6186082964917));
#38990=CARTESIAN_POINT('Ctrl Pts',(56.0532022284365,18.7873736610045,14.6143921370373));
#38991=CARTESIAN_POINT('Ctrl Pts',(55.9797089377853,18.7523911173528,14.6101760780454));
#38992=CARTESIAN_POINT('Ctrl Pts',(55.9044707555147,18.7210741159802,14.6059600190535));
#38993=CARTESIAN_POINT('Ctrl Pts',(55.8278897701911,18.6935852978242,14.6017439600616));
#38994=CARTESIAN_POINT('Ctrl Pts',(55.7506819205734,18.6658714661283,14.5974933899331));
#38995=CARTESIAN_POINT('Ctrl Pts',(55.6721096291193,18.6420489563563,14.5932428198046));
#38996=CARTESIAN_POINT('Ctrl Pts',(55.5926013144509,18.6222334151328,14.5889922496761));
#38997=CARTESIAN_POINT('Ctrl Pts',(55.5136238835892,18.6025501839702,14.5847700609674));
#38998=CARTESIAN_POINT('Ctrl Pts',(55.4337233638658,18.5868206046054,14.5805478722586));
#38999=CARTESIAN_POINT('Ctrl Pts',(55.3533288484233,18.5751063992678,14.5763256835499));
#39000=CARTESIAN_POINT('Ctrl Pts',(55.2721237188736,18.5632740801503,14.5720609227115));
#39001=CARTESIAN_POINT('Ctrl Pts',(55.1904150592977,18.5555386102629,14.5677961618732));
#39002=CARTESIAN_POINT('Ctrl Pts',(55.108647327921,18.5519097222252,14.5635314010349));
#39003=CARTESIAN_POINT('Ctrl Pts',(55.0268795965444,18.5482808341875,14.5592666401965));
#39004=CARTESIAN_POINT('Ctrl Pts',(54.9450532747815,18.5487584609394,14.5550018793582));
#39005=CARTESIAN_POINT('Ctrl Pts',(54.8636078207827,18.5532986648452,14.5507371185198));
#39006=CARTESIAN_POINT('Ctrl Pts',(54.7828029007025,18.5578031619748,14.5465058982149));
#39007=CARTESIAN_POINT('Ctrl Pts',(54.7020698672391,18.5663234092867,14.54227467791));
#39008=CARTESIAN_POINT('Ctrl Pts',(54.6218399940656,18.5788545562252,14.5380434576051));
#39009=CARTESIAN_POINT('Ctrl Pts',(54.541725164915,18.591367734376,14.5338183045739));
#39010=CARTESIAN_POINT('Ctrl Pts',(54.4621125185849,18.6078803184009,14.5295931515428));
#39011=CARTESIAN_POINT('Ctrl Pts',(54.3834305741755,18.6283355226469,14.5253679985116));
#39012=CARTESIAN_POINT('Ctrl Pts',(54.3045464990183,18.6488432754892,14.5211319912324));
#39013=CARTESIAN_POINT('Ctrl Pts',(54.2265983846976,18.6733138986637,14.5168959839532));
#39014=CARTESIAN_POINT('Ctrl Pts',(54.1500101176497,18.7016380942284,14.512659976674));
#39015=CARTESIAN_POINT('Ctrl Pts',(54.0737555276249,18.7298388879507,14.5084424246799));
#39016=CARTESIAN_POINT('Ctrl Pts',(53.9988494021766,18.7618595912587,14.5042248726857));
#39017=CARTESIAN_POINT('Ctrl Pts',(53.9256954313916,18.7975422946474,14.5000073206915));
#39018=CARTESIAN_POINT('Ctrl Pts',(53.8525656143835,18.8332132164192,14.4957911612371));
#39019=CARTESIAN_POINT('Ctrl Pts',(53.7811872207097,18.872543533488,14.4915750017827));
#39020=CARTESIAN_POINT('Ctrl Pts',(53.7119423331204,18.9153279162437,14.4873588423282));
#39021=CARTESIAN_POINT('Ctrl Pts',(53.6426990954968,18.9581112795341,14.4831427833363));
#39022=CARTESIAN_POINT('Ctrl Pts',(53.5755896578124,19.0043482995508,14.4789267243445));
#39023=CARTESIAN_POINT('Ctrl Pts',(53.510968697937,19.0537893147255,14.4747106653526));
#39024=CARTESIAN_POINT('Ctrl Pts',(53.4458187742172,19.1036350361984,14.4704600952241));
#39025=CARTESIAN_POINT('Ctrl Pts',(53.3831986466606,19.1567371696865,14.4662095250956));
#39026=CARTESIAN_POINT('Ctrl Pts',(53.3234377835841,19.2127984488349,14.4619589549671));
#39027=CARTESIAN_POINT('Ctrl Pts',(53.2640759488937,19.2684854020352,14.4577367662584));
#39028=CARTESIAN_POINT('Ctrl Pts',(53.207535593352,19.3270917234887,14.4535145775496));
#39029=CARTESIAN_POINT('Ctrl Pts',(53.1541012418314,19.3882903411,14.4492923888409));
#39030=CARTESIAN_POINT('Ctrl Pts',(53.100128114265,19.4501060214858,14.4450276280025));
#39031=CARTESIAN_POINT('Ctrl Pts',(53.0493242793575,19.5145661867257,14.4407628671642));
#39032=CARTESIAN_POINT('Ctrl Pts',(53.0019389097557,19.5813026645363,14.4364981063258));
#39033=CARTESIAN_POINT('Ctrl Pts',(52.9545535401539,19.648039142347,14.4322333454875));
#39034=CARTESIAN_POINT('Ctrl Pts',(52.910586840545,19.7170514918654,14.4279685846492));
#39035=CARTESIAN_POINT('Ctrl Pts',(52.8702401767789,19.7879466408639,14.4237038238108));
#39036=CARTESIAN_POINT('Ctrl Pts',(52.8284883593983,19.8613108558412,14.4192905341092));
#39037=CARTESIAN_POINT('Ctrl Pts',(52.7904674409891,19.9369463614327,14.4148772444075));
#39038=CARTESIAN_POINT('Ctrl Pts',(52.756419745081,20.0144555363974,14.4104639547059));
#39039=CARTESIAN_POINT('Ctrl Pts',(52.7224608961013,20.091762452386,14.4060621814145));
#39040=CARTESIAN_POINT('Ctrl Pts',(52.6924547829151,20.1709329286654,14.4016604081231));
#39041=CARTESIAN_POINT('Ctrl Pts',(52.666597893662,20.2515450179622,14.3972586348317));
#39042=CARTESIAN_POINT('Ctrl Pts',(52.6407808104884,20.3320330068224,14.3928636379679));
#39043=CARTESIAN_POINT('Ctrl Pts',(52.619100371865,20.4139578091949,14.3884686411041));
#39044=CARTESIAN_POINT('Ctrl Pts',(52.6017052240549,20.4968773333724,14.3840736442403));
#39045=CARTESIAN_POINT('Ctrl Pts',(52.5843426400325,20.5796416318623,14.3796868748286));
#39046=CARTESIAN_POINT('Ctrl Pts',(52.5712494539419,20.6633965462017,14.3753001054169));
#39047=CARTESIAN_POINT('Ctrl Pts',(52.5625242722944,20.7476860549908,14.3709133360052));
#39048=CARTESIAN_POINT('Ctrl Pts',(52.5538484626429,20.8314986062273,14.3665513894075));
#39049=CARTESIAN_POINT('Ctrl Pts',(52.5494914180731,20.9158393193652,14.3621894428098));
#39050=CARTESIAN_POINT('Ctrl Pts',(52.5495000127025,21.0002495094391,14.3578274962121));
#39051=CARTESIAN_POINT('',(52.5495008975342,21.0020973350978,13.5578274962436));
#39052=CARTESIAN_POINT('Ctrl Pts',(52.5495000127026,21.0002495104095,14.357827496162));
#39053=CARTESIAN_POINT('Ctrl Pts',(52.5495087833097,21.086387690449,14.3533762546587));
#39054=CARTESIAN_POINT('Ctrl Pts',(52.5540636293478,21.1724239248653,14.3489250131554));
#39055=CARTESIAN_POINT('Ctrl Pts',(52.5631068447131,21.2578798164185,14.3444737716521));
#39056=CARTESIAN_POINT('Ctrl Pts',(52.5721783102097,21.3436026639214,14.3400086249004));
#39057=CARTESIAN_POINT('Ctrl Pts',(52.5857661358387,21.4287411624085,14.3355434781487));
#39058=CARTESIAN_POINT('Ctrl Pts',(52.6037610884995,21.5128248521774,14.3310783313969));
#39059=CARTESIAN_POINT('Ctrl Pts',(52.6217854790889,21.5970460943875,14.3266058801152));
#39060=CARTESIAN_POINT('Ctrl Pts',(52.644231278249,21.6802087171782,14.3221334288335));
#39061=CARTESIAN_POINT('Ctrl Pts',(52.6709395064187,21.7618579048871,14.3176609775517));
#39062=CARTESIAN_POINT('Ctrl Pts',(52.697723286547,21.8437380609705,14.3131758746462));
#39063=CARTESIAN_POINT('Ctrl Pts',(52.7287934648449,21.9240958649999,14.3086907717407));
#39064=CARTESIAN_POINT('Ctrl Pts',(52.7639427262882,22.0024959444708,14.3042056688353));
#39065=CARTESIAN_POINT('Ctrl Pts',(52.7836267485637,22.0464009611722,14.3016939555908));
#39066=CARTESIAN_POINT('Ctrl Pts',(52.804589200067,22.089692456157,14.2991822423463));
#39067=CARTESIAN_POINT('Ctrl Pts',(52.8267876118373,22.1322977373184,14.2966705291019));
#39068=CARTESIAN_POINT('Ctrl Pts',(52.864182951782,22.2040703933512,14.292439308797));
#39069=CARTESIAN_POINT('Ctrl Pts',(52.9052077781994,22.2741230943974,14.288208088492));
#39070=CARTESIAN_POINT('Ctrl Pts',(52.9496799904678,22.3420648674755,14.2839768681871));
#39071=CARTESIAN_POINT('Ctrl Pts',(52.9940884326965,22.4099092168063,14.2797517151559));
#39072=CARTESIAN_POINT('Ctrl Pts',(53.0419341905162,22.4756482641494,14.2755265621248));
#39073=CARTESIAN_POINT('Ctrl Pts',(53.0929889755298,22.5389149432471,14.2713014090936));
#39074=CARTESIAN_POINT('Ctrl Pts',(53.1441749182307,22.6023441518962,14.2670654018144));
#39075=CARTESIAN_POINT('Ctrl Pts',(53.1985861731568,22.6632878575766,14.2628293945352));
#39076=CARTESIAN_POINT('Ctrl Pts',(53.2559485119627,22.7214048498465,14.258593387256));
#39077=CARTESIAN_POINT('Ctrl Pts',(53.3130609365822,22.7792686400826,14.2543758352619));
#39078=CARTESIAN_POINT('Ctrl Pts',(53.3730984615083,22.8343299574548,14.2501582832677));
#39079=CARTESIAN_POINT('Ctrl Pts',(53.4357508848395,22.8862860217156,14.2459407312735));
#39080=CARTESIAN_POINT('Ctrl Pts',(53.4983826217658,22.9382249312659,14.2417245718191));
#39081=CARTESIAN_POINT('Ctrl Pts',(53.5636271849506,22.9870603272302,14.2375084123647));
#39082=CARTESIAN_POINT('Ctrl Pts',(53.6311400658923,23.0325286543601,14.2332922529102));
#39083=CARTESIAN_POINT('Ctrl Pts',(53.6986513381388,23.0779958980718,14.2290761939183));
#39084=CARTESIAN_POINT('Ctrl Pts',(53.7684304344367,23.1200959736802,14.2248601349264));
#39085=CARTESIAN_POINT('Ctrl Pts',(53.8401037421017,23.1586085612991,14.2206440759345));
#39086=CARTESIAN_POINT('Ctrl Pts',(53.9123637415835,23.197436399054,14.216393505806));
#39087=CARTESIAN_POINT('Ctrl Pts',(53.9865486912519,23.2326175047625,14.2121429356776));
#39088=CARTESIAN_POINT('Ctrl Pts',(54.0622519876235,23.2639741419203,14.2078923655491));
#39089=CARTESIAN_POINT('Ctrl Pts',(54.1374498066208,23.2951214081342,14.2036701768403));
#39090=CARTESIAN_POINT('Ctrl Pts',(54.2141452948428,23.3224950232675,14.1994479881316));
#39091=CARTESIAN_POINT('Ctrl Pts',(54.291923206468,23.3459704824361,14.1952257994228));
#39092=CARTESIAN_POINT('Ctrl Pts',(54.3704853491071,23.3696826435521,14.1909610385845));
#39093=CARTESIAN_POINT('Ctrl Pts',(54.450151394513,23.3894174795893,14.1866962777461));
#39094=CARTESIAN_POINT('Ctrl Pts',(54.5304832116662,23.4050996310907,14.1824315169078));
#39095=CARTESIAN_POINT('Ctrl Pts',(54.6108150288194,23.4207817825921,14.1781667560695));
#39096=CARTESIAN_POINT('Ctrl Pts',(54.6918121316814,23.4324112446808,14.1739019952312));
#39097=CARTESIAN_POINT('Ctrl Pts',(54.773033396672,23.4399664774283,14.1696372343928));
#39098=CARTESIAN_POINT('Ctrl Pts',(54.8536158908956,23.4474622914777,14.1654060140879));
#39099=CARTESIAN_POINT('Ctrl Pts',(54.9347212049248,23.45097588546,14.161174793783));
#39100=CARTESIAN_POINT('Ctrl Pts',(55.0159220904974,23.4504482726706,14.156943573478));
#39101=CARTESIAN_POINT('Ctrl Pts',(55.0970065396835,23.4499214164409,14.1527184204469));
#39102=CARTESIAN_POINT('Ctrl Pts',(55.1781858272457,23.4453648653576,14.1484932674157));
#39103=CARTESIAN_POINT('Ctrl Pts',(55.2590277481769,23.4367714040661,14.1442681143846));
#39104=CARTESIAN_POINT('Ctrl Pts',(55.3400773487485,23.4281558665185,14.1400321071054));
#39105=CARTESIAN_POINT('Ctrl Pts',(55.4207873765294,23.4154826135697,14.1357960998262));
#39106=CARTESIAN_POINT('Ctrl Pts',(55.5007224418401,23.3987970498226,14.131560092547));
#39107=CARTESIAN_POINT('Ctrl Pts',(55.5803092489166,23.3821841811431,14.1273425405528));
#39108=CARTESIAN_POINT('Ctrl Pts',(55.6591273724268,23.3615939777363,14.1231249885587));
#39109=CARTESIAN_POINT('Ctrl Pts',(55.7367542074522,23.3371229081504,14.1189074365645));
#39110=CARTESIAN_POINT('Ctrl Pts',(55.8143554118625,23.312659918355,14.1146912771101));
#39111=CARTESIAN_POINT('Ctrl Pts',(55.8907656658357,23.2843187466799,14.1104751176557));
#39112=CARTESIAN_POINT('Ctrl Pts',(55.9655767208969,23.2522459559431,14.1062589582012));
#39113=CARTESIAN_POINT('Ctrl Pts',(56.0403859933623,23.2201739294359,14.1020428992093));
#39114=CARTESIAN_POINT('Ctrl Pts',(56.1135957158085,23.18437064487,14.0978268402174));
#39115=CARTESIAN_POINT('Ctrl Pts',(56.1848181867184,23.1450305625844,14.0936107812255));
#39116=CARTESIAN_POINT('Ctrl Pts',(56.2566236590583,23.1053684565902,14.0893602110971));
#39117=CARTESIAN_POINT('Ctrl Pts',(56.3264087681686,23.0621116016115,14.0851096409686));
#39118=CARTESIAN_POINT('Ctrl Pts',(56.3938037042642,23.0155052676635,14.0808590708401));
#39119=CARTESIAN_POINT('Ctrl Pts',(56.4607486386162,22.9692101281873,14.0766368821314));
#39120=CARTESIAN_POINT('Ctrl Pts',(56.525334886809,22.9196104380325,14.0724146934226));
#39121=CARTESIAN_POINT('Ctrl Pts',(56.5872326800828,22.8669875921594,14.0681925047139));
#39122=CARTESIAN_POINT('Ctrl Pts',(56.6497545858865,22.8138341526136,14.0639277438755));
#39123=CARTESIAN_POINT('Ctrl Pts',(56.7095331626611,22.7575965824059,14.0596629830372));
#39124=CARTESIAN_POINT('Ctrl Pts',(56.766267526519,22.6986021531731,14.0553982221989));
#39125=CARTESIAN_POINT('Ctrl Pts',(56.823001890377,22.6396077239403,14.0511334613605));
#39126=CARTESIAN_POINT('Ctrl Pts',(56.87669177368,22.5778568414246,14.0468687005222));
#39127=CARTESIAN_POINT('Ctrl Pts',(56.9270798909799,22.5137084738419,14.0426039396839));
#39128=CARTESIAN_POINT('Ctrl Pts',(56.9770717271293,22.4500646059364,14.0383727193789));
#39129=CARTESIAN_POINT('Ctrl Pts',(57.0240010454368,22.3838221996572,14.034141499074));
#39130=CARTESIAN_POINT('Ctrl Pts',(57.0675866198488,22.3153082602273,14.0299102787691));
#39131=CARTESIAN_POINT('Ctrl Pts',(57.1111096955978,22.2468925649912,14.0256851257379));
#39132=CARTESIAN_POINT('Ctrl Pts',(57.151298302633,22.1762121946507,14.0214599727068));
#39133=CARTESIAN_POINT('Ctrl Pts',(57.1879120273654,22.103626390818,14.0172348196756));
#39134=CARTESIAN_POINT('Ctrl Pts',(57.2246198112825,22.0308541169774,14.0129988123964));
#39135=CARTESIAN_POINT('Ctrl Pts',(57.2577340354098,21.9561669823079,14.0087628051172));
#39136=CARTESIAN_POINT('Ctrl Pts',(57.2870567725089,21.8799554359858,14.0045267978381));
#39137=CARTESIAN_POINT('Ctrl Pts',(57.3162517573556,21.8040759254035,14.0003092458439));
#39138=CARTESIAN_POINT('Ctrl Pts',(57.3416880478648,21.726685692201,13.9960916938497));
#39139=CARTESIAN_POINT('Ctrl Pts',(57.3632175547077,21.6481921313324,13.9918741418556));
#39140=CARTESIAN_POINT('Ctrl Pts',(57.3847399529972,21.5697244872519,13.9876579824012));
#39141=CARTESIAN_POINT('Ctrl Pts',(57.4023580063605,21.4901546869514,13.9834418229467));
#39142=CARTESIAN_POINT('Ctrl Pts',(57.4159735008235,21.4099052248002,13.9792256634923));
#39143=CARTESIAN_POINT('Ctrl Pts',(57.4295886708569,21.3296576748311,13.9750096045004));
#39144=CARTESIAN_POINT('Ctrl Pts',(57.4392013949395,21.2487309537676,13.9707935455085));
#39145=CARTESIAN_POINT('Ctrl Pts',(57.4447648452976,21.1675562627805,13.9665774865166));
#39146=CARTESIAN_POINT('Ctrl Pts',(57.4503738360515,21.0857171050834,13.9623269163881));
#39147=CARTESIAN_POINT('Ctrl Pts',(57.4518669064955,21.0036263766372,13.9580763462597));
#39148=CARTESIAN_POINT('Ctrl Pts',(57.4492496222306,20.9217277954623,13.9538257761312));
#39149=CARTESIAN_POINT('Ctrl Pts',(57.4466498137962,20.8403760581075,13.9496035874224));
#39150=CARTESIAN_POINT('Ctrl Pts',(57.4399944738528,20.7592143727547,13.9453813987137));
#39151=CARTESIAN_POINT('Ctrl Pts',(57.4293412325764,20.6786724012723,13.9411592100049));
#39152=CARTESIAN_POINT('Ctrl Pts',(57.4185805751708,20.5973183288908,13.9368944491666));
#39153=CARTESIAN_POINT('Ctrl Pts',(57.4037410291872,20.5165970156022,13.9326296883283));
#39154=CARTESIAN_POINT('Ctrl Pts',(57.3849344340167,20.4369387285195,13.9283649274899));
#39155=CARTESIAN_POINT('Ctrl Pts',(57.3661278388462,20.3572804414367,13.9241001666516));
#39156=CARTESIAN_POINT('Ctrl Pts',(57.3433543902884,20.2786856254416,13.9198354058133));
#39157=CARTESIAN_POINT('Ctrl Pts',(57.3167762003472,20.2015651012732,13.9155706449749));
#39158=CARTESIAN_POINT('Ctrl Pts',(57.2904070365862,20.1250510972863,13.91133942467));
#39159=CARTESIAN_POINT('Ctrl Pts',(57.2601939249194,20.0497013448655,13.9071082043651));
#39160=CARTESIAN_POINT('Ctrl Pts',(57.2262591397946,19.975929449461,13.9028769840602));
#39161=CARTESIAN_POINT('Ctrl Pts',(57.1923730147765,19.9022633377913,13.898651831029));
#39162=CARTESIAN_POINT('Ctrl Pts',(57.1547760078794,19.8301710083846,13.8944266779979));
#39163=CARTESIAN_POINT('Ctrl Pts',(57.1136396091149,19.7600492538893,13.8902015249667));
#39164=CARTESIAN_POINT('Ctrl Pts',(57.072397532598,19.6897473594296,13.8859655176875));
#39165=CARTESIAN_POINT('Ctrl Pts',(57.0275980156906,19.6214266216587,13.8817295104083));
#39166=CARTESIAN_POINT('Ctrl Pts',(56.9794618071307,19.5554650561129,13.8774935031291));
#39167=CARTESIAN_POINT('Ctrl Pts',(56.9315353166829,19.4897908695571,13.8732759511349));
#39168=CARTESIAN_POINT('Ctrl Pts',(56.8803014175048,19.4264557241399,13.8690583991408));
#39169=CARTESIAN_POINT('Ctrl Pts',(56.826022119979,19.365804948194,13.8648408471466));
#39170=CARTESIAN_POINT('Ctrl Pts',(56.7717607442425,19.3051741977545,13.8606246876922));
#39171=CARTESIAN_POINT('Ctrl Pts',(56.7144562767869,19.2472264028543,13.8564085282378));
#39172=CARTESIAN_POINT('Ctrl Pts',(56.6544104585641,19.1922731720213,13.8521923687833));
#39173=CARTESIAN_POINT('Ctrl Pts',(56.5943660711114,19.1373212506125,13.8479763097914));
#39174=CARTESIAN_POINT('Ctrl Pts',(56.5315808064862,19.0853640644655,13.8437602507995));
#39175=CARTESIAN_POINT('Ctrl Pts',(56.4663915841226,19.0366747666231,13.8395441918076));
#39176=CARTESIAN_POINT('Ctrl Pts',(56.4006687463233,18.9875869157693,13.8352936216792));
#39177=CARTESIAN_POINT('Ctrl Pts',(56.3325027880108,18.9418209995924,13.8310430515507));
#39178=CARTESIAN_POINT('Ctrl Pts',(56.2622695545512,18.8996129352776,13.8267924814222));
#39179=CARTESIAN_POINT('Ctrl Pts',(56.1925052743889,18.8576866978126,13.8225702927135));
#39180=CARTESIAN_POINT('Ctrl Pts',(56.1207016848963,18.8192711117173,13.8183481040047));
#39181=CARTESIAN_POINT('Ctrl Pts',(56.047251051513,18.7845507261269,13.8141259152959));
#39182=CARTESIAN_POINT('Ctrl Pts',(55.9730598188581,18.7494802565264,13.8098611544576));
#39183=CARTESIAN_POINT('Ctrl Pts',(55.897188590317,18.7181801091831,13.8055963936193));
#39184=CARTESIAN_POINT('Ctrl Pts',(55.8200595332974,18.6907896129092,13.8013316327809));
#39185=CARTESIAN_POINT('Ctrl Pts',(55.7429304762778,18.6633991166354,13.7970668719426));
#39186=CARTESIAN_POINT('Ctrl Pts',(55.6645440707518,18.6399183481377,13.7928021111043));
#39187=CARTESIAN_POINT('Ctrl Pts',(55.5853334035044,18.6204338511523,13.7885373502659));
#39188=CARTESIAN_POINT('Ctrl Pts',(55.5067456945264,18.6011025914636,13.784306129961));
#39189=CARTESIAN_POINT('Ctrl Pts',(55.4270519584008,18.5856324353945,13.7800749096561));
#39190=CARTESIAN_POINT('Ctrl Pts',(55.3466660209323,18.5741449095358,13.7758436893511));
#39191=CARTESIAN_POINT('Ctrl Pts',(55.266395351272,18.5626738559852,13.77161853632));
#39192=CARTESIAN_POINT('Ctrl Pts',(55.1854349079469,18.5551741557584,13.7673933832888));
#39193=CARTESIAN_POINT('Ctrl Pts',(55.1042110758042,18.5517168665206,13.7631682302577));
#39194=CARTESIAN_POINT('Ctrl Pts',(55.0227785829066,18.5482506956459,13.7589322229785));
#39195=CARTESIAN_POINT('Ctrl Pts',(54.9410818060719,18.5488478384384,13.7546962156993));
#39196=CARTESIAN_POINT('Ctrl Pts',(54.8595580621108,18.5535277822787,13.7504602084201));
#39197=CARTESIAN_POINT('Ctrl Pts',(54.7783894978822,18.5581873367071,13.7462426564259));
#39198=CARTESIAN_POINT('Ctrl Pts',(54.6973929295162,18.5668941721216,13.7420251044318));
#39199=CARTESIAN_POINT('Ctrl Pts',(54.6170005818436,18.5796153826939,13.7378075524376));
#39200=CARTESIAN_POINT('Ctrl Pts',(54.5366347778953,18.5923323930119,13.7335913929832));
#39201=CARTESIAN_POINT('Ctrl Pts',(54.4568732573093,18.609061073712,13.7293752335287));
#39202=CARTESIAN_POINT('Ctrl Pts',(54.3781414551259,18.6297168523219,13.7251590740743));
#39203=CARTESIAN_POINT('Ctrl Pts',(54.2994115289618,18.6503721387463,13.7209430150824));
#39204=CARTESIAN_POINT('Ctrl Pts',(54.2217117218376,18.6749542179751,13.7167269560905));
#39205=CARTESIAN_POINT('Ctrl Pts',(54.1454542316759,18.7033281079267,13.7125108970986));
#39206=CARTESIAN_POINT('Ctrl Pts',(54.0685725252348,18.7319342562963,13.7082603269702));
#39207=CARTESIAN_POINT('Ctrl Pts',(53.9931573125182,18.7643944264607,13.7040097568417));
#39208=CARTESIAN_POINT('Ctrl Pts',(53.919610611055,18.8005207392987,13.6997591867132));
#39209=CARTESIAN_POINT('Ctrl Pts',(53.8465549871979,18.8364058336609,13.6955369980045));
#39210=CARTESIAN_POINT('Ctrl Pts',(53.7753433787473,18.8759079796906,13.6913148092957));
#39211=CARTESIAN_POINT('Ctrl Pts',(53.7063435453016,18.9187976486614,13.687092620587));
#39212=CARTESIAN_POINT('Ctrl Pts',(53.6366479897902,18.9621197721412,13.6828278597486));
#39213=CARTESIAN_POINT('Ctrl Pts',(53.5692094619455,19.008897838649,13.6785630989103));
#39214=CARTESIAN_POINT('Ctrl Pts',(53.5043739391514,19.0588526753205,13.6742983380719));
#39215=CARTESIAN_POINT('Ctrl Pts',(53.4395384163572,19.108807511992,13.6700335772336));
#39216=CARTESIAN_POINT('Ctrl Pts',(53.3773062233166,19.1619387571298,13.6657688163953));
#39217=CARTESIAN_POINT('Ctrl Pts',(53.31798490625,19.2179294418017,13.6615040555569));
#39218=CARTESIAN_POINT('Ctrl Pts',(53.2578972260675,19.2746434616538,13.6571841989189));
#39219=CARTESIAN_POINT('Ctrl Pts',(53.2005478250414,19.3345261821984,13.6528643422808));
#39220=CARTESIAN_POINT('Ctrl Pts',(53.1462943772196,19.3972755339509,13.6485444856428));
#39221=CARTESIAN_POINT('Ctrl Pts',(53.0940287468598,19.4577257828418,13.6443829062535));
#39222=CARTESIAN_POINT('Ctrl Pts',(53.0446365371086,19.5208358806471,13.6402213268642));
#39223=CARTESIAN_POINT('Ctrl Pts',(52.9984030747795,19.5862956465556,13.6360597474749));
#39224=CARTESIAN_POINT('Ctrl Pts',(52.9522128951036,19.6516941306087,13.631902064056));
#39225=CARTESIAN_POINT('Ctrl Pts',(52.9091758730547,19.7194375302414,13.627744380637));
#39226=CARTESIAN_POINT('Ctrl Pts',(52.8695374951604,19.789182191462,13.6235866972181));
#39227=CARTESIAN_POINT('Ctrl Pts',(52.8299232378496,19.8588844119469,13.6194315438156));
#39228=CARTESIAN_POINT('Ctrl Pts',(52.7937037573007,19.9305850612507,13.6152763904132));
#39229=CARTESIAN_POINT('Ctrl Pts',(52.7610806557317,20.0039124436771,13.6111212370107));
#39230=CARTESIAN_POINT('Ctrl Pts',(52.7284667201144,20.0772192236713,13.6069672510612));
#39231=CARTESIAN_POINT('Ctrl Pts',(52.6994473506741,20.15215139047,13.6028132651117));
#39232=CARTESIAN_POINT('Ctrl Pts',(52.6741769814409,20.2283151314556,13.5986592791622));
#39233=CARTESIAN_POINT('Ctrl Pts',(52.6488948802354,20.3045142320704,13.5945033646912));
#39234=CARTESIAN_POINT('Ctrl Pts',(52.627365408381,20.3819455933885,13.5903474502203));
#39235=CARTESIAN_POINT('Ctrl Pts',(52.6096934889834,20.4601990798528,13.5861915357494));
#39236=CARTESIAN_POINT('Ctrl Pts',(52.5920165263288,20.5384748984951,13.5820344352531));
#39237=CARTESIAN_POINT('Ctrl Pts',(52.5781993940604,20.6175728371252,13.5778773347568));
#39238=CARTESIAN_POINT('Ctrl Pts',(52.5682956870323,20.6970736322232,13.5737202342605));
#39239=CARTESIAN_POINT('Ctrl Pts',(52.558381081092,20.776661917005,13.5695585589243));
#39240=CARTESIAN_POINT('Ctrl Pts',(52.55238852971,20.8566534647325,13.5653968835882));
#39241=CARTESIAN_POINT('Ctrl Pts',(52.5503196152149,20.9366260116536,13.561235208252));
#39242=CARTESIAN_POINT('Ctrl Pts',(52.5497549175711,20.9584540325404,13.5600993042492));
#39243=CARTESIAN_POINT('Ctrl Pts',(52.5494822250542,20.9802806517921,13.5589634002464));
#39244=CARTESIAN_POINT('Ctrl Pts',(52.5495008975342,21.0020973350977,13.5578274962436));
#39245=CARTESIAN_POINT('',(52.5495004842277,20.9984594806585,12.7578274961836));
#39246=CARTESIAN_POINT('Ctrl Pts',(52.5495008975348,21.0020973357021,13.5578274962121));
#39247=CARTESIAN_POINT('Ctrl Pts',(52.5496050215771,21.1237544800426,13.5514933144627));
#39248=CARTESIAN_POINT('Ctrl Pts',(52.5587720373766,21.2450363613145,13.5451591327133));
#39249=CARTESIAN_POINT('Ctrl Pts',(52.5768166350929,21.3648734438646,13.5388249509639));
#39250=CARTESIAN_POINT('Ctrl Pts',(52.5809513237883,21.3923325780772,13.5373735542586));
#39251=CARTESIAN_POINT('Ctrl Pts',(52.5855519468644,21.419715988469,13.5359221575533));
#39252=CARTESIAN_POINT('Ctrl Pts',(52.5906159685464,21.4470110054308,13.534470760848));
#39253=CARTESIAN_POINT('Ctrl Pts',(52.6053789835698,21.5265834817712,13.5302395405431));
#39254=CARTESIAN_POINT('Ctrl Pts',(52.6241158628056,21.6055730169194,13.5260083202382));
#39255=CARTESIAN_POINT('Ctrl Pts',(52.6467668473267,21.6835524699388,13.5217770999333));
#39256=CARTESIAN_POINT('Ctrl Pts',(52.6693853519214,21.7614201058803,13.5175519469021));
#39257=CARTESIAN_POINT('Ctrl Pts',(52.6959066862571,21.8382800935975,13.513326793871));
#39258=CARTESIAN_POINT('Ctrl Pts',(52.7262199305186,21.9137146412471,13.5091016408398));
#39259=CARTESIAN_POINT('Ctrl Pts',(52.7566110482845,21.9893429772131,13.5048656335606));
#39260=CARTESIAN_POINT('Ctrl Pts',(52.7908134910257,22.0635380770193,13.5006296262814));
#39261=CARTESIAN_POINT('Ctrl Pts',(52.8286648448361,22.1358934342399,13.4963936190022));
#39262=CARTESIAN_POINT('Ctrl Pts',(52.8663512892215,22.2079335562271,13.4921760670081));
#39263=CARTESIAN_POINT('Ctrl Pts',(52.9076547064636,22.2781495144851,13.4879585150139));
#39264=CARTESIAN_POINT('Ctrl Pts',(52.9523670404461,22.3461610278672,13.4837409630198));
#39265=CARTESIAN_POINT('Ctrl Pts',(52.9970646114331,22.4141500853948,13.4795248035654));
#39266=CARTESIAN_POINT('Ctrl Pts',(53.0451686087826,22.4799357552867,13.475308644111));
#39267=CARTESIAN_POINT('Ctrl Pts',(53.0964266956879,22.5431652293616,13.4710924846565));
#39268=CARTESIAN_POINT('Ctrl Pts',(53.147683561217,22.6063931968062,13.4668764256646));
#39269=CARTESIAN_POINT('Ctrl Pts',(53.2020940732346,22.6670647290788,13.4626603666728));
#39270=CARTESIAN_POINT('Ctrl Pts',(53.2593654158795,22.7248598478032,13.4584443076809));
#39271=CARTESIAN_POINT('Ctrl Pts',(53.3171055610562,22.7831280565013,13.4541937375524));
#39272=CARTESIAN_POINT('Ctrl Pts',(53.377753262231,22.838472191678,13.4499431674239));
#39273=CARTESIAN_POINT('Ctrl Pts',(53.4409716986284,22.8906033443116,13.4456925972954));
#39274=CARTESIAN_POINT('Ctrl Pts',(53.503768020127,22.9423864127871,13.4414704085866));
#39275=CARTESIAN_POINT('Ctrl Pts',(53.5691004377833,22.9909990440902,13.4372482198779));
#39276=CARTESIAN_POINT('Ctrl Pts',(53.6366082941618,23.0362007038727,13.4330260311692));
#39277=CARTESIAN_POINT('Ctrl Pts',(53.7047968290724,23.081858129859,13.4287612703308));
#39278=CARTESIAN_POINT('Ctrl Pts',(53.7752045025753,23.124035162188,13.4244965094924));
#39279=CARTESIAN_POINT('Ctrl Pts',(53.8474343961711,23.1625315671385,13.420231748654));
#39280=CARTESIAN_POINT('Ctrl Pts',(53.9196642897669,23.201027972089,13.4159669878157));
#39281=CARTESIAN_POINT('Ctrl Pts',(53.9937159401067,23.2358436028115,13.4117022269773));
#39282=CARTESIAN_POINT('Ctrl Pts',(54.0691738226618,23.2668288152355,13.4074374661389));
#39283=CARTESIAN_POINT('Ctrl Pts',(54.1440382610055,23.2975703421182,13.403206245834));
#39284=CARTESIAN_POINT('Ctrl Pts',(54.2205676074931,23.324656804284,13.398975025529));
#39285=CARTESIAN_POINT('Ctrl Pts',(54.2983705606061,23.347906808154,13.3947438052241));
#39286=CARTESIAN_POINT('Ctrl Pts',(54.3760619497298,23.3711234731457,13.390518652193));
#39287=CARTESIAN_POINT('Ctrl Pts',(54.455022876685,23.3905144736688,13.3862934991618));
#39288=CARTESIAN_POINT('Ctrl Pts',(54.5348421548412,23.4059464726147,13.3820683461306));
#39289=CARTESIAN_POINT('Ctrl Pts',(54.6148664855094,23.4214181157446,13.3778323388514));
#39290=CARTESIAN_POINT('Ctrl Pts',(54.6957531440898,23.4329102168745,13.3735963315722));
#39291=CARTESIAN_POINT('Ctrl Pts',(54.7770725051384,23.4403388252525,13.369360324293));
#39292=CARTESIAN_POINT('Ctrl Pts',(54.8580375769028,23.4477350689351,13.3651427722989));
#39293=CARTESIAN_POINT('Ctrl Pts',(54.9394311234451,23.4511031026776,13.3609252203047));
#39294=CARTESIAN_POINT('Ctrl Pts',(55.0208208065253,23.4504115458461,13.3567076683106));
#39295=CARTESIAN_POINT('Ctrl Pts',(55.1021836165837,23.4497202173509,13.3524915088561));
#39296=CARTESIAN_POINT('Ctrl Pts',(55.1835421011733,23.4449719640442,13.3482753494017));
#39297=CARTESIAN_POINT('Ctrl Pts',(55.264462995854,23.4361875079361,13.3440591899472));
#39298=CARTESIAN_POINT('Ctrl Pts',(55.3453819623538,23.4274032611438,13.3398431309553));
#39299=CARTESIAN_POINT('Ctrl Pts',(55.4258628975894,23.4145830540475,13.3356270719634));
#39300=CARTESIAN_POINT('Ctrl Pts',(55.5054781732568,23.3977994216283,13.3314110129715));
#39301=CARTESIAN_POINT('Ctrl Pts',(55.585745150823,23.3808784044544,13.3271604428431));
#39302=CARTESIAN_POINT('Ctrl Pts',(55.6651317587422,23.3599288593701,13.3229098727146));
#39303=CARTESIAN_POINT('Ctrl Pts',(55.7432126138556,23.3350771423244,13.3186593025861));
#39304=CARTESIAN_POINT('Ctrl Pts',(55.8207721164321,23.3103913623155,13.3144371138774));
#39305=CARTESIAN_POINT('Ctrl Pts',(55.8970428322707,23.2818555843418,13.3102149251686));
#39306=CARTESIAN_POINT('Ctrl Pts',(55.9716270995667,23.2496424225614,13.3059927364599));
#39307=CARTESIAN_POINT('Ctrl Pts',(56.0469633965112,23.2171044569904,13.3017279756216));
#39308=CARTESIAN_POINT('Ctrl Pts',(56.120578609002,23.1808147472378,13.2974632147832));
#39309=CARTESIAN_POINT('Ctrl Pts',(56.1920892757065,23.1409982271701,13.2931984539449));
#39310=CARTESIAN_POINT('Ctrl Pts',(56.2635999424109,23.1011817071024,13.2889336931066));
#39311=CARTESIAN_POINT('Ctrl Pts',(56.3330056887029,23.0578386864169,13.2846689322683));
#39312=CARTESIAN_POINT('Ctrl Pts',(56.399955471868,23.0112371632373,13.28040417143));
#39313=CARTESIAN_POINT('Ctrl Pts',(56.4663787234119,22.9650021412529,13.276172951125));
#39314=CARTESIAN_POINT('Ctrl Pts',(56.530633609848,22.9153863486505,13.2719417308201));
#39315=CARTESIAN_POINT('Ctrl Pts',(56.5923555456466,22.8626202152475,13.2677105105152));
#39316=CARTESIAN_POINT('Ctrl Pts',(56.6539889765092,22.8099297447866,13.263485357484));
#39317=CARTESIAN_POINT('Ctrl Pts',(56.7130963199011,22.7540982049184,13.2592602044529));
#39318=CARTESIAN_POINT('Ctrl Pts',(56.769342586897,22.6953987909022,13.2550350514217));
#39319=CARTESIAN_POINT('Ctrl Pts',(56.8257333482884,22.6365485804545,13.2507990441425));
#39320=CARTESIAN_POINT('Ctrl Pts',(56.8792479307538,22.5748160170196,13.2465630368633));
#39321=CARTESIAN_POINT('Ctrl Pts',(56.9295828436043,22.510516567161,13.2423270295841));
#39322=CARTESIAN_POINT('Ctrl Pts',(56.9796984591065,22.4464972548463,13.23810947759));
#39323=CARTESIAN_POINT('Ctrl Pts',(57.0266617585143,22.3799337394739,13.2338919255958));
#39324=CARTESIAN_POINT('Ctrl Pts',(57.0702119514747,22.3111722716605,13.2296743736017));
#39325=CARTESIAN_POINT('Ctrl Pts',(57.1137477651521,22.2424335073195,13.2254582141473));
#39326=CARTESIAN_POINT('Ctrl Pts',(57.1538724617397,22.1714986241666,13.2212420546928));
#39327=CARTESIAN_POINT('Ctrl Pts',(57.190368527163,22.0987429022359,13.2170258952384));
#39328=CARTESIAN_POINT('Ctrl Pts',(57.2268637229589,22.0259889139267,13.2128098362465));
#39329=CARTESIAN_POINT('Ctrl Pts',(57.2597302520328,21.9514145891694,13.2085937772546));
#39330=CARTESIAN_POINT('Ctrl Pts',(57.2887971914368,21.8754185664417,13.2043777182627));
#39331=CARTESIAN_POINT('Ctrl Pts',(57.3181020623113,21.7988004677125,13.2001271481342));
#39332=CARTESIAN_POINT('Ctrl Pts',(57.3435446658933,21.7207377308969,13.1958765780058));
#39333=CARTESIAN_POINT('Ctrl Pts',(57.3650005188826,21.6416562909259,13.1916260078773));
#39334=CARTESIAN_POINT('Ctrl Pts',(57.3863131093094,21.5631028844827,13.1874038191685));
#39335=CARTESIAN_POINT('Ctrl Pts',(57.4036919869534,21.483544809274,13.1831816304598));
#39336=CARTESIAN_POINT('Ctrl Pts',(57.4170665674218,21.40340978998,13.178959441751));
#39337=CARTESIAN_POINT('Ctrl Pts',(57.4305760031542,21.3224667730666,13.1746946809127));
#39338=CARTESIAN_POINT('Ctrl Pts',(57.4399998811463,21.2409355945664,13.1704299200744));
#39339=CARTESIAN_POINT('Ctrl Pts',(57.4453192776807,21.1592604163091,13.166165159236));
#39340=CARTESIAN_POINT('Ctrl Pts',(57.4506386742152,21.0775852380518,13.1619003983977));
#39341=CARTESIAN_POINT('Ctrl Pts',(57.4518536463803,20.9957665427361,13.1576356375594));
#39342=CARTESIAN_POINT('Ctrl Pts',(57.4489990326534,20.9142446033025,13.153370876721));
#39343=CARTESIAN_POINT('Ctrl Pts',(57.4461668692516,20.8333637993128,13.1491396564161));
#39344=CARTESIAN_POINT('Ctrl Pts',(57.4393183278817,20.7524718047301,13.1449084361112));
#39345=CARTESIAN_POINT('Ctrl Pts',(57.4284493375912,20.6719999012911,13.1406772158063));
#39346=CARTESIAN_POINT('Ctrl Pts',(57.417595932672,20.5916433889294,13.1364520627751));
#39347=CARTESIAN_POINT('Ctrl Pts',(57.4027335903438,20.511706228188,13.132226909744));
#39348=CARTESIAN_POINT('Ctrl Pts',(57.3839102206162,20.4326180210462,13.1280017567128));
#39349=CARTESIAN_POINT('Ctrl Pts',(57.3650384944096,20.3533266394841,13.1237657494336));
#39350=CARTESIAN_POINT('Ctrl Pts',(57.3421853862492,20.2748890504587,13.1195297421544));
#39351=CARTESIAN_POINT('Ctrl Pts',(57.3154514030215,20.1977313104415,13.1152937348752));
#39352=CARTESIAN_POINT('Ctrl Pts',(57.2888338934559,20.120909728507,13.1110761828811));
#39353=CARTESIAN_POINT('Ctrl Pts',(57.2583693998657,20.0453573116013,13.1068586308869));
#39354=CARTESIAN_POINT('Ctrl Pts',(57.2242074480419,19.9714809296493,13.1026410788927));
#39355=CARTESIAN_POINT('Ctrl Pts',(57.1900567757174,19.897628939998,13.0984249194383));
#39356=CARTESIAN_POINT('Ctrl Pts',(57.1522112645126,19.8254523080053,13.0942087599839));
#39357=CARTESIAN_POINT('Ctrl Pts',(57.1108682971053,19.7553372817201,13.0899926005295));
#39358=CARTESIAN_POINT('Ctrl Pts',(57.0695263148171,19.6852239261339,13.0857765415376));
#39359=CARTESIAN_POINT('Ctrl Pts',(57.0246872791213,19.6171724785061,13.0815604825457));
#39360=CARTESIAN_POINT('Ctrl Pts',(56.9765934620127,19.5515427048309,13.0773444235538));
#39361=CARTESIAN_POINT('Ctrl Pts',(56.9281059662828,19.4853757095258,13.0730938534253));
#39362=CARTESIAN_POINT('Ctrl Pts',(56.8763104288674,19.421670613497,13.0688432832968));
#39363=CARTESIAN_POINT('Ctrl Pts',(56.8214972377978,19.3607629632372,13.0645927131683));
#39364=CARTESIAN_POINT('Ctrl Pts',(56.7670500390859,19.3002619985594,13.0603705244596));
#39365=CARTESIAN_POINT('Ctrl Pts',(56.7096257371693,19.2425215251593,13.0561483357508));
#39366=CARTESIAN_POINT('Ctrl Pts',(56.6495454490545,19.1878327722024,13.0519261470421));
#39367=CARTESIAN_POINT('Ctrl Pts',(56.5888593742285,19.132592595129,13.0476613862037));
#39368=CARTESIAN_POINT('Ctrl Pts',(56.5254638266102,19.0804663341252,13.0433966253654));
#39369=CARTESIAN_POINT('Ctrl Pts',(56.4597217458266,19.0317107238109,13.0391318645271));
#39370=CARTESIAN_POINT('Ctrl Pts',(56.393979665043,18.9829551134966,13.0348671036887));
#39371=CARTESIAN_POINT('Ctrl Pts',(56.3258914876291,18.937570367634,13.0306023428504));
#39372=CARTESIAN_POINT('Ctrl Pts',(56.255846036666,18.8957659393047,13.026337582012));
#39373=CARTESIAN_POINT('Ctrl Pts',(56.1863514634373,18.8542902850563,13.0221063617071));
#39374=CARTESIAN_POINT('Ctrl Pts',(56.1146697196367,18.8161832658581,13.0178751414022));
#39375=CARTESIAN_POINT('Ctrl Pts',(56.041160976075,18.7816821526439,13.0136439210972));
#39376=CARTESIAN_POINT('Ctrl Pts',(55.9677576389066,18.7472305116113,13.0094187680661));
#39377=CARTESIAN_POINT('Ctrl Pts',(55.8925329223964,18.7163747031977,13.0051936150349));
#39378=CARTESIAN_POINT('Ctrl Pts',(55.8158737711765,18.6893074112928,13.0009684620038));
#39379=CARTESIAN_POINT('Ctrl Pts',(55.7390176856833,18.6621705846047,12.9967324547246));
#39380=CARTESIAN_POINT('Ctrl Pts',(55.6607201946426,18.6388420008193,12.9924964474454));
#39381=CARTESIAN_POINT('Ctrl Pts',(55.5813937828006,18.6194682276179,12.9882604401662));
#39382=CARTESIAN_POINT('Ctrl Pts',(55.5024129774331,18.6001788613788,12.984042888172));
#39383=CARTESIAN_POINT('Ctrl Pts',(55.4224126506704,18.5848100361842,12.9798253361779));
#39384=CARTESIAN_POINT('Ctrl Pts',(55.341815745164,18.5734567289335,12.9756077841837));
#39385=CARTESIAN_POINT('Ctrl Pts',(55.2612454509223,18.5621071702866,12.9713916247293));
#39386=CARTESIAN_POINT('Ctrl Pts',(55.1800794291201,18.5547705614661,12.9671754652748));
#39387=CARTESIAN_POINT('Ctrl Pts',(55.0987492442285,18.5514904866911,12.9629593058204));
#39388=CARTESIAN_POINT('Ctrl Pts',(55.0174209972704,18.5482104900736,12.9587432468285));
#39389=CARTESIAN_POINT('Ctrl Pts',(54.9359290595891,18.548986852946,12.9545271878366));
#39390=CARTESIAN_POINT('Ctrl Pts',(54.8547070844642,18.5538110827871,12.9503111288447));
#39391=CARTESIAN_POINT('Ctrl Pts',(54.7728202555785,18.5586748020318,12.9460605587162));
#39392=CARTESIAN_POINT('Ctrl Pts',(54.6912083091062,18.5676529504591,12.9418099885878));
#39393=CARTESIAN_POINT('Ctrl Pts',(54.6103106378111,18.5806834744092,12.9375594184593));
#39394=CARTESIAN_POINT('Ctrl Pts',(54.5299531271754,18.5936269924381,12.9333372297505));
#39395=CARTESIAN_POINT('Ctrl Pts',(54.4503008285854,18.6105687765357,12.9291150410418));
#39396=CARTESIAN_POINT('Ctrl Pts',(54.3717725597401,18.6313969236479,12.924892852333));
#39397=CARTESIAN_POINT('Ctrl Pts',(54.2924524940645,18.6524350799849,12.9206280914947));
#39398=CARTESIAN_POINT('Ctrl Pts',(54.2142797154996,18.6774382644917,12.9163633306564));
#39399=CARTESIAN_POINT('Ctrl Pts',(54.1376667353455,18.7062407295729,12.912098569818));
#39400=CARTESIAN_POINT('Ctrl Pts',(54.0610537551914,18.7350431946541,12.9078338089797));
#39401=CARTESIAN_POINT('Ctrl Pts',(53.9860009897574,18.7676446894243,12.9035690481414));
#39402=CARTESIAN_POINT('Ctrl Pts',(53.9128952572967,18.803832081012,12.899304287303));
#39403=CARTESIAN_POINT('Ctrl Pts',(53.840364470385,18.8397348741281,12.8950730669981));
#39404=CARTESIAN_POINT('Ctrl Pts',(53.7694781981508,18.8793019528073,12.8908418466932));
#39405=CARTESIAN_POINT('Ctrl Pts',(53.700631096504,18.922359342276,12.8866106263883));
#39406=CARTESIAN_POINT('Ctrl Pts',(53.6318827167823,18.9653549904619,12.8823854733571));
#39407=CARTESIAN_POINT('Ctrl Pts',(53.5651680911645,19.0118307649638,12.878160320326));
#39408=CARTESIAN_POINT('Ctrl Pts',(53.5008589292994,19.0615660186278,12.8739351672948));
#39409=CARTESIAN_POINT('Ctrl Pts',(53.4363845597864,19.1114290401561,12.8696991600156));
#39410=CARTESIAN_POINT('Ctrl Pts',(53.3743284490996,19.1645680940725,12.8654631527364));
#39411=CARTESIAN_POINT('Ctrl Pts',(53.315037406826,19.2207160683004,12.8612271454572));
#39412=CARTESIAN_POINT('Ctrl Pts',(53.2560046816452,19.276619419042,12.857009593463));
#39413=CARTESIAN_POINT('Ctrl Pts',(53.1997133269616,19.3355052106891,12.8527920414689));
#39414=CARTESIAN_POINT('Ctrl Pts',(53.146472474467,19.3970695704144,12.8485744894747));
#39415=CARTESIAN_POINT('Ctrl Pts',(53.0932492008907,19.4586136029886,12.8443583300203));
#39416=CARTESIAN_POINT('Ctrl Pts',(53.0430747332105,19.5228340959575,12.8401421705659));
#39417=CARTESIAN_POINT('Ctrl Pts',(52.9962196961089,19.5893920659027,12.8359260111114));
#39418=CARTESIAN_POINT('Ctrl Pts',(52.9493657754679,19.6559484499065,12.8317099521195));
#39419=CARTESIAN_POINT('Ctrl Pts',(52.9058313948651,19.7248418193401,12.8274938931276));
#39420=CARTESIAN_POINT('Ctrl Pts',(52.8658445548617,19.7957031985484,12.8232778341357));
#39421=CARTESIAN_POINT('Ctrl Pts',(52.8255303970245,19.8671446234203,12.8190272640073));
#39422=CARTESIAN_POINT('Ctrl Pts',(52.7888223753672,19.940586015715,12.8147766938788));
#39423=CARTESIAN_POINT('Ctrl Pts',(52.7559065985614,20.015624535241,12.8105261237503));
#39424=CARTESIAN_POINT('Ctrl Pts',(52.723210603208,20.0901620161643,12.8063039350416));
#39425=CARTESIAN_POINT('Ctrl Pts',(52.6942564738011,20.1662749001549,12.8020817463328));
#39426=CARTESIAN_POINT('Ctrl Pts',(52.6691772775385,20.2435506054883,12.7978595576241));
#39427=CARTESIAN_POINT('Ctrl Pts',(52.643845208923,20.3216054781133,12.7935947967857));
#39428=CARTESIAN_POINT('Ctrl Pts',(52.6224667813494,20.4008462843846,12.7893300359474));
#39429=CARTESIAN_POINT('Ctrl Pts',(52.6051264004603,20.4808365457511,12.7850652751091));
#39430=CARTESIAN_POINT('Ctrl Pts',(52.5877860195712,20.5608268071176,12.7808005142707));
#39431=CARTESIAN_POINT('Ctrl Pts',(52.5744837002957,20.6415660377458,12.7765357534324));
#39432=CARTESIAN_POINT('Ctrl Pts',(52.5652501021603,20.7226136539601,12.7722709925941));
#39433=CARTESIAN_POINT('Ctrl Pts',(52.5548262709602,20.8141085033343,12.7674564938001));
#39434=CARTESIAN_POINT('Ctrl Pts',(52.5495584825478,20.9062017589285,12.7626419950061));
#39435=CARTESIAN_POINT('Ctrl Pts',(52.5495004842281,20.998459480112,12.7578274962121));
#39436=CARTESIAN_POINT('',(52.5495002652713,20.9988597830668,11.957827496262));
#39437=CARTESIAN_POINT('Ctrl Pts',(52.5495004842277,20.9984594806585,12.7578274961836));
#39438=CARTESIAN_POINT('Ctrl Pts',(52.5494502298631,21.0783989483802,12.7536558294006));
#39439=CARTESIAN_POINT('Ctrl Pts',(52.5533158347715,21.1584933142817,12.7494841626176));
#39440=CARTESIAN_POINT('Ctrl Pts',(52.5611163582093,21.2383208589397,12.7453124958346));
#39441=CARTESIAN_POINT('Ctrl Pts',(52.5689133596593,21.3181123609344,12.7411427125867));
#39442=CARTESIAN_POINT('Ctrl Pts',(52.5806417568019,21.3976368040027,12.7369729293388));
#39443=CARTESIAN_POINT('Ctrl Pts',(52.5962684716246,21.4764713942033,12.7328031460909));
#39444=CARTESIAN_POINT('Ctrl Pts',(52.611868507349,21.5551713920849,12.7286404818094));
#39445=CARTESIAN_POINT('Ctrl Pts',(52.6313535083502,21.6331834148886,12.7244778175279));
#39446=CARTESIAN_POINT('Ctrl Pts',(52.6546388108824,21.7100923479246,12.7203151532463));
#39447=CARTESIAN_POINT('Ctrl Pts',(52.6779137748999,21.7869671339215,12.7161543371592));
#39448=CARTESIAN_POINT('Ctrl Pts',(52.7049855542601,21.8627393445095,12.7119935210721));
#39449=CARTESIAN_POINT('Ctrl Pts',(52.7357190674315,21.9370069948547,12.707832704985));
#39450=CARTESIAN_POINT('Ctrl Pts',(52.7664489467307,22.011265863934,12.7036723808649));
#39451=CARTESIAN_POINT('Ctrl Pts',(52.800839516234,22.0840200842678,12.6995120567448));
#39452=CARTESIAN_POINT('Ctrl Pts',(52.8387073866657,22.1548872194057,12.6953517326246));
#39453=CARTESIAN_POINT('Ctrl Pts',(52.8767194845923,22.2260242664573,12.691175563063));
#39454=CARTESIAN_POINT('Ctrl Pts',(52.9182352066916,22.2952593910474,12.6869993935014));
#39455=CARTESIAN_POINT('Ctrl Pts',(52.9630232435531,22.3622319713232,12.6828232239397));
#39456=CARTESIAN_POINT('Ctrl Pts',(53.0076998559111,22.4290379359796,12.6786574439297));
#39457=CARTESIAN_POINT('Ctrl Pts',(53.0556322019289,22.4935922376309,12.6744916639197));
#39458=CARTESIAN_POINT('Ctrl Pts',(53.1065492809538,22.555568907038,12.6703258839096));
#39459=CARTESIAN_POINT('Ctrl Pts',(53.1576568425362,22.6177774333135,12.6661445195722));
#39460=CARTESIAN_POINT('Ctrl Pts',(53.2117711769549,22.6773886538559,12.6619631552348));
#39461=CARTESIAN_POINT('Ctrl Pts',(53.2685813071997,22.7341105963063,12.6577817908973));
#39462=CARTESIAN_POINT('Ctrl Pts',(53.3253914374445,22.7908325387567,12.6536004265599));
#39463=CARTESIAN_POINT('Ctrl Pts',(53.3848969618111,22.8446649320933,12.6494190622225));
#39464=CARTESIAN_POINT('Ctrl Pts',(53.4467556182776,22.8953580507777,12.645237697885));
#39465=CARTESIAN_POINT('Ctrl Pts',(53.5093518385911,22.9466556024351,12.6410064775801));
#39466=CARTESIAN_POINT('Ctrl Pts',(53.5746093865146,22.9949450396391,12.6367752572752));
#39467=CARTESIAN_POINT('Ctrl Pts',(53.642207143667,23.0399384327207,12.6325440369703));
#39468=CARTESIAN_POINT('Ctrl Pts',(53.7097079703668,23.0848673084257,12.6283188839391));
#39469=CARTESIAN_POINT('Ctrl Pts',(53.7795419578684,23.1265092713537,12.624093730908));
#39470=CARTESIAN_POINT('Ctrl Pts',(53.8513549141328,23.1646165287905,12.6198685778768));
#39471=CARTESIAN_POINT('Ctrl Pts',(53.9233523549909,23.2028216822377,12.6156325705976));
#39472=CARTESIAN_POINT('Ctrl Pts',(53.9973385762571,23.2374736516977,12.6113965633184));
#39473=CARTESIAN_POINT('Ctrl Pts',(54.072927306216,23.2683664762203,12.6071605560392));
#39474=CARTESIAN_POINT('Ctrl Pts',(54.1481867138992,23.2991247079897,12.6029430040451));
#39475=CARTESIAN_POINT('Ctrl Pts',(54.2250342658871,23.3261562973527,12.5987254520509));
#39476=CARTESIAN_POINT('Ctrl Pts',(54.303065717464,23.3493047600995,12.5945079000568));
#39477=CARTESIAN_POINT('Ctrl Pts',(54.3810714048307,23.3724455797505,12.5902917406023));
#39478=CARTESIAN_POINT('Ctrl Pts',(54.460259770148,23.3917056867734,12.5860755811479));
#39479=CARTESIAN_POINT('Ctrl Pts',(54.5402104408931,23.4069781493267,12.5818594216935));
#39480=CARTESIAN_POINT('Ctrl Pts',(54.6201592065758,23.4222502479682,12.5776433627016));
#39481=CARTESIAN_POINT('Ctrl Pts',(54.7008697846985,23.4335348049145,12.5734273037097));
#39482=CARTESIAN_POINT('Ctrl Pts',(54.7819120349269,23.4407760834395,12.5692112447178));
#39483=CARTESIAN_POINT('Ctrl Pts',(54.8636176677529,23.4480766364558,12.5649606745893));
#39484=CARTESIAN_POINT('Ctrl Pts',(54.9456599512586,23.4512673532029,12.5607101044609));
#39485=CARTESIAN_POINT('Ctrl Pts',(55.0275951472322,23.4503446202217,12.5564595343324));
#39486=CARTESIAN_POINT('Ctrl Pts',(55.1089832549055,23.4494280484074,12.5522373456236));
#39487=CARTESIAN_POINT('Ctrl Pts',(55.1902652359041,23.4444528816744,12.5480151569149));
#39488=CARTESIAN_POINT('Ctrl Pts',(55.2710103282567,23.435467850738,12.5437929682061));
#39489=CARTESIAN_POINT('Ctrl Pts',(55.3525695695665,23.4263922241584,12.5395282073678));
#39490=CARTESIAN_POINT('Ctrl Pts',(55.4335805549402,23.4132254936289,12.5352634465295));
#39491=CARTESIAN_POINT('Ctrl Pts',(55.5136107960271,23.3960705749632,12.5309986856912));
#39492=CARTESIAN_POINT('Ctrl Pts',(55.593641037114,23.3789156562974,12.5267339248528));
#39493=CARTESIAN_POINT('Ctrl Pts',(55.6726900850779,23.3577727360512,12.5224691640145));
#39494=CARTESIAN_POINT('Ctrl Pts',(55.7503438539423,23.332795394125,12.5182044031762));
#39495=CARTESIAN_POINT('Ctrl Pts',(55.8273869088823,23.3080144883891,12.5139731828712));
#39496=CARTESIAN_POINT('Ctrl Pts',(55.9033454696026,23.2793663757153,12.5097419625663));
#39497=CARTESIAN_POINT('Ctrl Pts',(55.9778034900124,23.2469647493718,12.5055107422614));
#39498=CARTESIAN_POINT('Ctrl Pts',(56.0521547428323,23.2146095846927,12.5012855892302));
#39499=CARTESIAN_POINT('Ctrl Pts',(56.12500930601,23.1785117798965,12.497060436199));
#39500=CARTESIAN_POINT('Ctrl Pts',(56.1959669246842,23.1388345810421,12.4928352831679));
#39501=CARTESIAN_POINT('Ctrl Pts',(56.267106830624,23.0990554530612,12.4885992758887));
#39502=CARTESIAN_POINT('Ctrl Pts',(56.3363395858625,23.0556786674869,12.4843632686095));
#39503=CARTESIAN_POINT('Ctrl Pts',(56.4032826897653,23.0089171069521,12.4801272613303));
#39504=CARTESIAN_POINT('Ctrl Pts',(56.4699341383468,22.9623592755122,12.4759097093361));
#39505=CARTESIAN_POINT('Ctrl Pts',(56.5343154566839,22.9124463621612,12.471692157342));
#39506=CARTESIAN_POINT('Ctrl Pts',(56.5960759708961,22.859433178452,12.4674746053478));
#39507=CARTESIAN_POINT('Ctrl Pts',(56.6578160931914,22.8064374984901,12.4632584458934));
#39508=CARTESIAN_POINT('Ctrl Pts',(56.7169367772811,22.7503438835511,12.4590422864389));
#39509=CARTESIAN_POINT('Ctrl Pts',(56.7731202400878,22.6914475647181,12.4548261269845));
#39510=CARTESIAN_POINT('Ctrl Pts',(56.8293023641565,22.6325526492651,12.4506100679926));
#39511=CARTESIAN_POINT('Ctrl Pts',(56.8825470859884,22.5708554998705,12.4463940090007));
#39512=CARTESIAN_POINT('Ctrl Pts',(56.9325743421322,22.5066873139879,12.4421779500088));
#39513=CARTESIAN_POINT('Ctrl Pts',(56.9830111033311,22.4419938705055,12.4379273798803));
#39514=CARTESIAN_POINT('Ctrl Pts',(57.0301771740755,22.3747891182426,12.4336768097519));
#39515=CARTESIAN_POINT('Ctrl Pts',(57.073828913661,22.305443942444,12.4294262396234));
#39516=CARTESIAN_POINT('Ctrl Pts',(57.1171891868536,22.2365617903059,12.4252040509146));
#39517=CARTESIAN_POINT('Ctrl Pts',(57.1570817408366,22.1655681507613,12.4209818622059));
#39518=CARTESIAN_POINT('Ctrl Pts',(57.1933139523331,22.0928513881132,12.4167596734971));
#39519=CARTESIAN_POINT('Ctrl Pts',(57.229911491509,22.0194014257775,12.4124949126588));
#39520=CARTESIAN_POINT('Ctrl Pts',(57.2627742640968,21.9441938415729,12.4082301518205));
#39521=CARTESIAN_POINT('Ctrl Pts',(57.2917542389756,21.867647830711,12.4039653909821));
#39522=CARTESIAN_POINT('Ctrl Pts',(57.3207342138544,21.791101819849,12.3997006301438));
#39523=CARTESIAN_POINT('Ctrl Pts',(57.3458313044062,21.7132178606124,12.3954358693055));
#39524=CARTESIAN_POINT('Ctrl Pts',(57.3669500274368,21.6344271570612,12.3911711084671));
#39525=CARTESIAN_POINT('Ctrl Pts',(57.3879026606768,21.556256108943,12.3869398881622));
#39526=CARTESIAN_POINT('Ctrl Pts',(57.4050178934107,21.4768994071786,12.3827086678573));
#39527=CARTESIAN_POINT('Ctrl Pts',(57.4181656654684,21.3967682753822,12.3784774475523));
#39528=CARTESIAN_POINT('Ctrl Pts',(57.4312945845412,21.3167520460204,12.3742522945212));
#39529=CARTESIAN_POINT('Ctrl Pts',(57.4404672671976,21.2359640470366,12.37002714149));
#39530=CARTESIAN_POINT('Ctrl Pts',(57.4456038516245,21.154829102301,12.3658019884588));
#39531=CARTESIAN_POINT('Ctrl Pts',(57.45075363173,21.0734857251587,12.3615659811796));
#39532=CARTESIAN_POINT('Ctrl Pts',(57.4518464339143,20.9917940749852,12.3573299739004));
#39533=CARTESIAN_POINT('Ctrl Pts',(57.4488537294991,20.9101909719555,12.3530939666213));
#39534=CARTESIAN_POINT('Ctrl Pts',(57.4458740635915,20.8289433944071,12.3488764146271));
#39535=CARTESIAN_POINT('Ctrl Pts',(57.4388444249965,20.7477840619109,12.3446588626329));
#39536=CARTESIAN_POINT('Ctrl Pts',(57.4277887723585,20.6671457874534,12.3404413106388));
#39537=CARTESIAN_POINT('Ctrl Pts',(57.4167367700455,20.5865341379195,12.3362251511843));
#39538=CARTESIAN_POINT('Ctrl Pts',(57.4016614565903,20.5064436650254,12.3320089917299));
#39539=CARTESIAN_POINT('Ctrl Pts',(57.382638586668,20.4273014620932,12.3277928322755));
#39540=CARTESIAN_POINT('Ctrl Pts',(57.3636161700222,20.3481611449593,12.3235767732836));
#39541=CARTESIAN_POINT('Ctrl Pts',(57.3406464936627,20.2699695046497,12.3193607142917));
#39542=CARTESIAN_POINT('Ctrl Pts',(57.3138559848859,20.1931414428738,12.3151446552998));
#39543=CARTESIAN_POINT('Ctrl Pts',(57.2868461786778,20.1156844943254,12.3108940851713));
#39544=CARTESIAN_POINT('Ctrl Pts',(57.2559528422172,20.0396140091258,12.3066435150428));
#39545=CARTESIAN_POINT('Ctrl Pts',(57.2213554990952,19.9653358048915,12.3023929449144));
#39546=CARTESIAN_POINT('Ctrl Pts',(57.1869891653876,19.8915535625697,12.2981707562056));
#39547=CARTESIAN_POINT('Ctrl Pts',(57.1489684121945,19.8195401260059,12.2939485674968));
#39548=CARTESIAN_POINT('Ctrl Pts',(57.1075151123934,19.7496679236965,12.2897263787881));
#39549=CARTESIAN_POINT('Ctrl Pts',(57.065643840926,19.6790912032674,12.2854616179498));
#39550=CARTESIAN_POINT('Ctrl Pts',(57.0202706813945,19.6106995448714,12.2811968571114));
#39551=CARTESIAN_POINT('Ctrl Pts',(56.971667590737,19.54484462629,12.2769320962731));
#39552=CARTESIAN_POINT('Ctrl Pts',(56.9230645000795,19.4789897077085,12.2726673354348));
#39553=CARTESIAN_POINT('Ctrl Pts',(56.8712318331998,19.4156718610565,12.2684025745965));
#39554=CARTESIAN_POINT('Ctrl Pts',(56.8164801299285,19.3552051229485,12.2641378137581));
#39555=CARTESIAN_POINT('Ctrl Pts',(56.7621590255587,19.2952139300647,12.2599065934532));
#39556=CARTESIAN_POINT('Ctrl Pts',(56.7047609707054,19.2378041695224,12.2556753731483));
#39557=CARTESIAN_POINT('Ctrl Pts',(56.6445609685304,19.1833080969008,12.2514441528433));
#39558=CARTESIAN_POINT('Ctrl Pts',(56.5844472889451,19.128890167833,12.2472189998122));
#39559=CARTESIAN_POINT('Ctrl Pts',(56.5215399834475,19.0773779381981,12.242993846781));
#39560=CARTESIAN_POINT('Ctrl Pts',(56.4561527012609,19.0290688594954,12.2387686937499));
#39561=CARTESIAN_POINT('Ctrl Pts',(56.3905974417789,18.9806356767146,12.2345326864707));
#39562=CARTESIAN_POINT('Ctrl Pts',(56.322549768956,18.9354224690416,12.2302966791915));
#39563=CARTESIAN_POINT('Ctrl Pts',(56.252361245682,18.893690060719,12.2260606719123));
#39564=CARTESIAN_POINT('Ctrl Pts',(56.1824785172564,18.8521394706607,12.2218431199181));
#39565=CARTESIAN_POINT('Ctrl Pts',(56.1104739518147,18.8140396593022,12.2176255679239));
#39566=CARTESIAN_POINT('Ctrl Pts',(56.0367242050376,18.7796051763956,12.2134080159298));
#39567=CARTESIAN_POINT('Ctrl Pts',(55.9629988087491,18.7451820629719,12.2091918564754));
#39568=CARTESIAN_POINT('Ctrl Pts',(55.8875297963499,18.7144220712353,12.2049756970209));
#39569=CARTESIAN_POINT('Ctrl Pts',(55.8107171025951,18.687493128754,12.2007595375665));
#39570=CARTESIAN_POINT('Ctrl Pts',(55.7339062391314,18.6605648279349,12.1965434785746));
#39571=CARTESIAN_POINT('Ctrl Pts',(55.6557521970783,18.637467547638,12.1923274195827));
#39572=CARTESIAN_POINT('Ctrl Pts',(55.5766721431692,18.618320027944,12.1881113605908));
#39573=CARTESIAN_POINT('Ctrl Pts',(55.4969447684926,18.5990157735675,12.1838607904624));
#39574=CARTESIAN_POINT('Ctrl Pts',(55.4162766144555,18.5837263693793,12.1796102203339));
#39575=CARTESIAN_POINT('Ctrl Pts',(55.3351060049849,18.5725210164817,12.1753596502054));
#39576=CARTESIAN_POINT('Ctrl Pts',(55.2544773786052,18.5613904826822,12.1711374614967));
#39577=CARTESIAN_POINT('Ctrl Pts',(55.1733534593422,18.5542896065041,12.1669152727879));
#39578=CARTESIAN_POINT('Ctrl Pts',(55.092167479111,18.5512339013711,12.1626930840791));
#39579=CARTESIAN_POINT('Ctrl Pts',(55.0101629044709,18.5481473857074,12.1584283232408));
#39580=CARTESIAN_POINT('Ctrl Pts',(54.9280954960608,18.5491880686115,12.1541635624025));
#39581=CARTESIAN_POINT('Ctrl Pts',(54.8464082069827,18.5543181296175,12.1498988015641));
#39582=CARTESIAN_POINT('Ctrl Pts',(54.7647209179046,18.5594481906234,12.1456340407258));
#39583=CARTESIAN_POINT('Ctrl Pts',(54.6834142196497,18.5686675116084,12.1413692798875));
#39584=CARTESIAN_POINT('Ctrl Pts',(54.602920358367,18.5818854435324,12.1371045190491));
#39585=CARTESIAN_POINT('Ctrl Pts',(54.52305954713,18.5949994220334,12.1328732987442));
#39586=CARTESIAN_POINT('Ctrl Pts',(54.4436993569119,18.6120984721533,12.1286420784393));
#39587=CARTESIAN_POINT('Ctrl Pts',(54.3652680733224,18.6331316827385,12.1244108581344));
#39588=CARTESIAN_POINT('Ctrl Pts',(54.2869492547042,18.6541347331719,12.1201857051032));
#39589=CARTESIAN_POINT('Ctrl Pts',(54.2095571425543,18.6790606205957,12.1159605520721));
#39590=CARTESIAN_POINT('Ctrl Pts',(54.1335117336019,18.7078070905366,12.1117353990409));
#39591=CARTESIAN_POINT('Ctrl Pts',(54.0572709670552,18.7366274090015,12.1074993917617));
#39592=CARTESIAN_POINT('Ctrl Pts',(53.9823842965493,18.769287882134,12.1032633844825));
#39593=CARTESIAN_POINT('Ctrl Pts',(53.9092615009143,18.8056345389584,12.0990273772033));
#39594=CARTESIAN_POINT('Ctrl Pts',(53.8364572840606,18.8418228419681,12.0948098252092));
#39595=CARTESIAN_POINT('Ctrl Pts',(53.765402027165,18.8816650750567,12.090592273215));
#39596=CARTESIAN_POINT('Ctrl Pts',(53.6964802334532,18.9249610923595,12.0863747212209));
#39597=CARTESIAN_POINT('Ctrl Pts',(53.6275811961498,18.9682428143023,12.0821585617664));
#39598=CARTESIAN_POINT('Ctrl Pts',(53.5608146165273,19.014975808746,12.077942402312));
#39599=CARTESIAN_POINT('Ctrl Pts',(53.4965384466261,19.0649150903574,12.0737262428576));
#39600=CARTESIAN_POINT('Ctrl Pts',(53.4322638082958,19.1148531820169,12.0695101838657));
#39601=CARTESIAN_POINT('Ctrl Pts',(53.3704798281551,19.1679971228223,12.0652941248738));
#39602=CARTESIAN_POINT('Ctrl Pts',(53.3115124727321,19.2240607779936,12.0610780658819));
#39603=CARTESIAN_POINT('Ctrl Pts',(53.2520624318294,19.2805833500027,12.0568274957534));
#39604=CARTESIAN_POINT('Ctrl Pts',(53.1954756989531,19.3400733375517,12.0525769256249));
#39605=CARTESIAN_POINT('Ctrl Pts',(53.142048088122,19.4021999677216,12.0483263554964));
#39606=CARTESIAN_POINT('Ctrl Pts',(53.0889772180107,19.4639117730766,12.0441041667877));
#39607=CARTESIAN_POINT('Ctrl Pts',(53.0390236501508,19.5282247093893,12.0398819780789));
#39608=CARTESIAN_POINT('Ctrl Pts',(52.9924353272746,19.5947831715977,12.0356597893702));
#39609=CARTESIAN_POINT('Ctrl Pts',(52.9453772565365,19.6620127396408,12.0313950285319));
#39610=CARTESIAN_POINT('Ctrl Pts',(52.9017529341781,19.731532960029,12.0271302676935));
#39611=CARTESIAN_POINT('Ctrl Pts',(52.8617707609506,19.8029511408157,12.0228655068552));
#39612=CARTESIAN_POINT('Ctrl Pts',(52.8217885877232,19.8743693216024,12.0186007460168));
#39613=CARTESIAN_POINT('Ctrl Pts',(52.7854487200286,19.947685002575,12.0143359851785));
#39614=CARTESIAN_POINT('Ctrl Pts',(52.752909364638,20.0224858433412,12.0100712243402));
#39615=CARTESIAN_POINT('Ctrl Pts',(52.7173238434928,20.1042891510222,12.0054072187024));
#39616=CARTESIAN_POINT('Ctrl Pts',(52.6861685079812,20.1881309433786,12.0007432130646));
#39617=CARTESIAN_POINT('Ctrl Pts',(52.6596573132858,20.2735384671277,11.9960792074268));
#39618=CARTESIAN_POINT('Ctrl Pts',(52.6332226283103,20.3586995098786,11.99142866183));
#39619=CARTESIAN_POINT('Ctrl Pts',(52.6114054762756,20.4454169984112,11.9867781162331));
#39620=CARTESIAN_POINT('Ctrl Pts',(52.5943717616921,20.5331991548254,11.9821275706363));
#39621=CARTESIAN_POINT('Ctrl Pts',(52.5774219366889,20.620548991664,11.9774999285768));
#39622=CARTESIAN_POINT('Ctrl Pts',(52.5652086737941,20.708952755731,11.9728722865173));
#39623=CARTESIAN_POINT('Ctrl Pts',(52.5578475305062,20.7979070368733,11.9682446444578));
#39624=CARTESIAN_POINT('Ctrl Pts',(52.5523240465134,20.8646544874749,11.9647722617259));
#39625=CARTESIAN_POINT('Ctrl Pts',(52.5495315093585,20.9317114843349,11.961299878994));
#39626=CARTESIAN_POINT('Ctrl Pts',(52.5495002652713,20.9988597830668,11.957827496262));
#39627=CARTESIAN_POINT('',(52.5495009324152,21.0021377010802,11.1578274961736));
#39628=CARTESIAN_POINT('Ctrl Pts',(52.5495002652709,20.9988597840325,11.9578274962121));
#39629=CARTESIAN_POINT('Ctrl Pts',(52.5494617060243,21.0817295440113,11.9535421229565));
#39630=CARTESIAN_POINT('Ctrl Pts',(52.5536311635913,21.1645874816312,11.9492567497009));
#39631=CARTESIAN_POINT('Ctrl Pts',(52.5619786838129,21.2469864607974,11.9449713764453));
#39632=CARTESIAN_POINT('Ctrl Pts',(52.5703298476175,21.3294214060365,11.9406841326805));
#39633=CARTESIAN_POINT('Ctrl Pts',(52.5828626554615,21.4113965534959,11.9363968889157));
#39634=CARTESIAN_POINT('Ctrl Pts',(52.5994954785962,21.4924716161569,11.9321096451509));
#39635=CARTESIAN_POINT('Ctrl Pts',(52.61615360331,21.5736700088794,11.9278158797009));
#39636=CARTESIAN_POINT('Ctrl Pts',(52.6369241088679,21.6539651472636,11.9235221142509));
#39637=CARTESIAN_POINT('Ctrl Pts',(52.6616745845297,21.7329287150642,11.9192283488009));
#39638=CARTESIAN_POINT('Ctrl Pts',(52.6864445431347,21.8119544409714,11.9149312034083));
#39639=CARTESIAN_POINT('Ctrl Pts',(52.7152005586122,21.8896460925574,11.9106340580156));
#39640=CARTESIAN_POINT('Ctrl Pts',(52.7477617165096,21.9655946170004,11.906336912623));
#39641=CARTESIAN_POINT('Ctrl Pts',(52.7803906220155,22.0417011619573,11.9020308264757));
#39642=CARTESIAN_POINT('Ctrl Pts',(52.8168402938814,22.1160569342268,11.8977247403284));
#39643=CARTESIAN_POINT('Ctrl Pts',(52.856883369401,22.1882766334696,11.8934186541811));
#39644=CARTESIAN_POINT('Ctrl Pts',(52.8890607823993,22.2463102150313,11.8899584126644));
#39645=CARTESIAN_POINT('Ctrl Pts',(52.9235576151699,22.3029649191521,11.8864981711478));
#39646=CARTESIAN_POINT('Ctrl Pts',(52.9602364172642,22.3580555130572,11.8830379296311));
#39647=CARTESIAN_POINT('Ctrl Pts',(53.0050876484384,22.4254208800177,11.8788067093262));
#39648=CARTESIAN_POINT('Ctrl Pts',(53.0533637774511,22.4906882736688,11.8745754890213));
#39649=CARTESIAN_POINT('Ctrl Pts',(53.1048419648748,22.5534884202659,11.8703442687164));
#39650=CARTESIAN_POINT('Ctrl Pts',(53.1562463361806,22.6161985158481,11.8661191156852));
#39651=CARTESIAN_POINT('Ctrl Pts',(53.2108433545295,22.6764480343051,11.8618939626541));
#39652=CARTESIAN_POINT('Ctrl Pts',(53.2683668120242,22.7338964076037,11.8576688096229));
#39653=CARTESIAN_POINT('Ctrl Pts',(53.3260380449656,22.7914923634606,11.8534328023437));
#39654=CARTESIAN_POINT('Ctrl Pts',(53.3866505051754,22.8462723743405,11.8491967950645));
#39655=CARTESIAN_POINT('Ctrl Pts',(53.4498950709855,22.8979264893681,11.8449607877853));
#39656=CARTESIAN_POINT('Ctrl Pts',(53.5128640951328,22.9493555595943,11.8407432357912));
#39657=CARTESIAN_POINT('Ctrl Pts',(53.5784419805868,22.9976856124538,11.836525683797));
#39658=CARTESIAN_POINT('Ctrl Pts',(53.6462879449976,23.0426487515334,11.8323081318029));
#39659=CARTESIAN_POINT('Ctrl Pts',(53.7141115082144,23.0875970448075,11.8280919723484));
#39660=CARTESIAN_POINT('Ctrl Pts',(53.7842012760034,23.1291803753072,11.823875812894));
#39661=CARTESIAN_POINT('Ctrl Pts',(53.8561865476807,23.1671735131949,11.8196596534396));
#39662=CARTESIAN_POINT('Ctrl Pts',(53.9281701040951,23.2051657457832,11.8154435944477));
#39663=CARTESIAN_POINT('Ctrl Pts',(54.002048662911,23.2395677398193,11.8112275354558));
#39664=CARTESIAN_POINT('Ctrl Pts',(54.0774272063071,23.2702003634784,11.8070114764639));
#39665=CARTESIAN_POINT('Ctrl Pts',(54.1534227712417,23.3010837347341,11.8027609063354));
#39666=CARTESIAN_POINT('Ctrl Pts',(54.2309425523896,23.328135545893,11.798510336207));
#39667=CARTESIAN_POINT('Ctrl Pts',(54.309563280757,23.3512225302427,11.7942597660785));
#39668=CARTESIAN_POINT('Ctrl Pts',(54.3876590518073,23.3741553608265,11.7900375773697));
#39669=CARTESIAN_POINT('Ctrl Pts',(54.466840641655,23.3931761007768,11.785815388661));
#39670=CARTESIAN_POINT('Ctrl Pts',(54.5466818770947,23.4082053337383,11.7815931999523));
#39671=CARTESIAN_POINT('Ctrl Pts',(54.6273281479452,23.4233861057468,11.7773284391139));
#39672=CARTESIAN_POINT('Ctrl Pts',(54.7086469602838,23.4344943596096,11.7730636782756));
#39673=CARTESIAN_POINT('Ctrl Pts',(54.7901946387221,23.4415019886085,11.7687989174373));
#39674=CARTESIAN_POINT('Ctrl Pts',(54.8717423171605,23.4485096176073,11.7645341565989));
#39675=CARTESIAN_POINT('Ctrl Pts',(54.9535183779222,23.4514166688341,11.7602693957606));
#39676=CARTESIAN_POINT('Ctrl Pts',(55.0350819216579,23.4502488667017,11.7560046349223));
#39677=CARTESIAN_POINT('Ctrl Pts',(55.1160040027493,23.4490902488372,11.7517734146174));
#39678=CARTESIAN_POINT('Ctrl Pts',(55.1970203468551,23.4439163437233,11.7475421943124));
#39679=CARTESIAN_POINT('Ctrl Pts',(55.2776998487097,23.4347141606412,11.7433109740075));
#39680=CARTESIAN_POINT('Ctrl Pts',(55.3582636618055,23.4255251728455,11.7390858209764));
#39681=CARTESIAN_POINT('Ctrl Pts',(55.438491133911,23.4123194314266,11.7348606679452));
#39682=CARTESIAN_POINT('Ctrl Pts',(55.5179517639833,23.3951359502514,11.7306355149141));
#39683=CARTESIAN_POINT('Ctrl Pts',(55.5976165252156,23.3779083254048,11.7263995076349));
#39684=CARTESIAN_POINT('Ctrl Pts',(55.6765100275266,23.3566825105134,11.7221635003557));
#39685=CARTESIAN_POINT('Ctrl Pts',(55.7542042267086,23.3315501784038,11.7179274930765));
#39686=CARTESIAN_POINT('Ctrl Pts',(55.8315599305816,23.3065273419402,11.7137099410824));
#39687=CARTESIAN_POINT('Ctrl Pts',(55.9077263120162,23.2776320930379,11.7094923890882));
#39688=CARTESIAN_POINT('Ctrl Pts',(55.9822934953388,23.2450055097962,11.7052748370941));
#39689=CARTESIAN_POINT('Ctrl Pts',(56.0568360582737,23.21238969911,11.7010586776396));
#39690=CARTESIAN_POINT('Ctrl Pts',(56.1297800460681,23.1760451868864,11.6968425181852));
#39691=CARTESIAN_POINT('Ctrl Pts',(56.2007352106399,23.1361613244157,11.6926263587308));
#39692=CARTESIAN_POINT('Ctrl Pts',(56.2716886844939,23.0962784122967,11.6884102997389));
#39693=CARTESIAN_POINT('Ctrl Pts',(56.3406530246077,23.0528565463878,11.684194240747));
#39694=CARTESIAN_POINT('Ctrl Pts',(56.407263530797,23.0061305054479,11.6799781817551));
#39695=CARTESIAN_POINT('Ctrl Pts',(56.4744192865388,22.9590219820084,11.6757276116266));
#39696=CARTESIAN_POINT('Ctrl Pts',(56.5391820932744,22.9085552026386,11.6714770414982));
#39697=CARTESIAN_POINT('Ctrl Pts',(56.601210469907,22.8550135527969,11.6672264713697));
#39698=CARTESIAN_POINT('Ctrl Pts',(56.6628246777715,22.8018294051238,11.6630042826609));
#39699=CARTESIAN_POINT('Ctrl Pts',(56.7217405633723,22.7456116931203,11.6587820939522));
#39700=CARTESIAN_POINT('Ctrl Pts',(56.7776603178603,22.6866754413061,11.6545599052434));
#39701=CARTESIAN_POINT('Ctrl Pts',(56.8341439085955,22.6271449380442,11.6502951444051));
#39702=CARTESIAN_POINT('Ctrl Pts',(56.8875702922149,22.5648411333649,11.6460303835667));
#39703=CARTESIAN_POINT('Ctrl Pts',(56.9376752819753,22.5001215789469,11.6417656227283));
#39704=CARTESIAN_POINT('Ctrl Pts',(56.9877802717357,22.4354020245288,11.63750086189));
#39705=CARTESIAN_POINT('Ctrl Pts',(57.0345636448914,22.368267152392,11.6332361010516));
#39706=CARTESIAN_POINT('Ctrl Pts',(57.0778079507488,22.2991013701037,11.6289713402132));
#39707=CARTESIAN_POINT('Ctrl Pts',(57.1207121584999,22.2304795473288,11.6247401199082));
#39708=CARTESIAN_POINT('Ctrl Pts',(57.1602936913421,22.1596013450064,11.6205088996033));
#39709=CARTESIAN_POINT('Ctrl Pts',(57.1963078793248,22.0868219491782,11.6162776792983));
#39710=CARTESIAN_POINT('Ctrl Pts',(57.2322704254826,22.01414691391,11.6120525262671));
#39711=CARTESIAN_POINT('Ctrl Pts',(57.2646755817379,21.9395765127103,11.6078273732359));
#39712=CARTESIAN_POINT('Ctrl Pts',(57.2933227018554,21.8634936219536,11.6036022202047));
#39713=CARTESIAN_POINT('Ctrl Pts',(57.3220434152709,21.7872152773144,11.5993662129255));
#39714=CARTESIAN_POINT('Ctrl Pts',(57.3469865145598,21.7094170657506,11.5951302056463));
#39715=CARTESIAN_POINT('Ctrl Pts',(57.3679969315569,21.6305083521548,11.5908941983672));
#39716=CARTESIAN_POINT('Ctrl Pts',(57.3889158111208,21.5519434252198,11.586676646373));
#39717=CARTESIAN_POINT('Ctrl Pts',(57.4059360761835,21.4722781024795,11.5824590943788));
#39718=CARTESIAN_POINT('Ctrl Pts',(57.4189540220132,21.391933271599,11.5782415423846));
#39719=CARTESIAN_POINT('Ctrl Pts',(57.4319676696133,21.3116149687539,11.5740253829301));
#39720=CARTESIAN_POINT('Ctrl Pts',(57.4409815479425,21.2306180618886,11.5698092234756));
#39721=CARTESIAN_POINT('Ctrl Pts',(57.4459431556209,21.1493731216499,11.5655930640212));
#39722=CARTESIAN_POINT('Ctrl Pts',(57.4509046450741,21.0681301173136,11.5613770050292));
#39723=CARTESIAN_POINT('Ctrl Pts',(57.4518140286243,20.9866395554796,11.5571609460373));
#39724=CARTESIAN_POINT('Ctrl Pts',(57.4486708272855,20.9053351723125,11.5529448870454));
#39725=CARTESIAN_POINT('Ctrl Pts',(57.4455018968355,20.8233652608236,11.5486943169169));
#39726=CARTESIAN_POINT('Ctrl Pts',(57.4382137317604,20.7415850700323,11.5444437467885));
#39727=CARTESIAN_POINT('Ctrl Pts',(57.4268592840387,20.6604351822186,11.5401931766601));
#39728=CARTESIAN_POINT('Ctrl Pts',(57.4155806509339,20.579827139134,11.5359709879513));
#39729=CARTESIAN_POINT('Ctrl Pts',(57.4002900205224,20.4998414570351,11.5317487992425));
#39730=CARTESIAN_POINT('Ctrl Pts',(57.3810906090871,20.4208991786248,11.5275266105337));
#39731=CARTESIAN_POINT('Ctrl Pts',(57.3616976108925,20.3411609289476,11.5232618496955));
#39732=CARTESIAN_POINT('Ctrl Pts',(57.338316702293,20.2624877082379,11.5189970888572));
#39733=CARTESIAN_POINT('Ctrl Pts',(57.311105063035,20.18529536787,11.514732328019));
#39734=CARTESIAN_POINT('Ctrl Pts',(57.2838934237769,20.108103027502,11.5104675671807));
#39735=CARTESIAN_POINT('Ctrl Pts',(57.2528512960813,20.0323919888855,11.5062028063425));
#39736=CARTESIAN_POINT('Ctrl Pts',(57.2181837662685,19.9585533959617,11.5019380455042));
#39737=CARTESIAN_POINT('Ctrl Pts',(57.1837888818592,19.8852955122224,11.4977068251993));
#39738=CARTESIAN_POINT('Ctrl Pts',(57.14569648065,19.8136059992063,11.4934756048944));
#39739=CARTESIAN_POINT('Ctrl Pts',(57.1040723371263,19.7438830268881,11.4892443845895));
#39740=CARTESIAN_POINT('Ctrl Pts',(57.0625078797113,19.6742600324325,11.4850192315584));
#39741=CARTESIAN_POINT('Ctrl Pts',(57.0174219743112,19.6065983740059,11.4807940785273));
#39742=CARTESIAN_POINT('Ctrl Pts',(56.9690275324282,19.5412742456035,11.4765689254962));
#39743=CARTESIAN_POINT('Ctrl Pts',(56.9205087671717,19.4757823021442,11.472332918217));
#39744=CARTESIAN_POINT('Ctrl Pts',(56.8686646510941,19.4126403386582,11.4680969109378));
#39745=CARTESIAN_POINT('Ctrl Pts',(56.8137550657124,19.3522006154867,11.4638609036586));
#39746=CARTESIAN_POINT('Ctrl Pts',(56.7590847084494,19.2920242139405,11.4596433516645));
#39747=CARTESIAN_POINT('Ctrl Pts',(56.7013758457917,19.2345269075629,11.4554257996703));
#39748=CARTESIAN_POINT('Ctrl Pts',(56.6409258914727,19.1800240472208,11.4512082476762));
#39749=CARTESIAN_POINT('Ctrl Pts',(56.5804958963534,19.1255391824832,11.4469920882218));
#39750=CARTESIAN_POINT('Ctrl Pts',(56.5173269518917,19.0740471114464,11.4427759287674));
#39751=CARTESIAN_POINT('Ctrl Pts',(56.45175237138,19.0258254124337,11.438559769313));
#39752=CARTESIAN_POINT('Ctrl Pts',(56.3861793533778,18.9776048624465,11.4343437103211));
#39753=CARTESIAN_POINT('Ctrl Pts',(56.318201188503,18.9326548040867,11.4301276513293));
#39754=CARTESIAN_POINT('Ctrl Pts',(56.2481820575066,18.8912108210353,11.4259115923374));
#39755=CARTESIAN_POINT('Ctrl Pts',(56.1775897751851,18.8494275925025,11.4216610222089));
#39756=CARTESIAN_POINT('Ctrl Pts',(56.1049233639389,18.8112083613104,11.4174104520804));
#39757=CARTESIAN_POINT('Ctrl Pts',(56.0305817283029,18.776747528667,11.4131598819519));
#39758=CARTESIAN_POINT('Ctrl Pts',(55.9567364781175,18.7425167939465,11.4089376932431));
#39759=CARTESIAN_POINT('Ctrl Pts',(55.8812387650967,18.7119945389902,11.4047155045344));
#39760=CARTESIAN_POINT('Ctrl Pts',(55.8044983303346,18.6853223363741,11.4004933158257));
#39761=CARTESIAN_POINT('Ctrl Pts',(55.726984125387,18.6583811991965,11.3962285549873));
#39762=CARTESIAN_POINT('Ctrl Pts',(55.648202463344,18.6353683273631,11.3919637941489));
#39763=CARTESIAN_POINT('Ctrl Pts',(55.5685879835304,18.6163771365871,11.3876990333105));
#39764=CARTESIAN_POINT('Ctrl Pts',(55.4889735037168,18.5973859458111,11.383434272472));
#39765=CARTESIAN_POINT('Ctrl Pts',(55.4085266915533,18.5824164610675,11.3791695116336));
#39766=CARTESIAN_POINT('Ctrl Pts',(55.3276874022963,18.5715084483622,11.3749047507952));
#39767=CARTESIAN_POINT('Ctrl Pts',(55.247483879732,18.5606862225462,11.3706735304904));
#39768=CARTESIAN_POINT('Ctrl Pts',(55.1665932833734,18.5538211859867,11.3664423101855));
#39769=CARTESIAN_POINT('Ctrl Pts',(55.0854400562631,18.5509899455523,11.3622110898807));
#39770=CARTESIAN_POINT('Ctrl Pts',(55.0044031972008,18.5481627649186,11.3579859368496));
#39771=CARTESIAN_POINT('Ctrl Pts',(54.9231049160502,18.5493579086654,11.3537607838185));
#39772=CARTESIAN_POINT('Ctrl Pts',(54.8419767495782,18.5546004616165,11.3495356307875));
#39773=CARTESIAN_POINT('Ctrl Pts',(54.7606401681106,18.5598564824753,11.3452996235082));
#39774=CARTESIAN_POINT('Ctrl Pts',(54.6794750451078,18.5691807911745,11.341063616229));
#39775=CARTESIAN_POINT('Ctrl Pts',(54.5989182756023,18.5825460293205,11.3368276089498));
#39776=CARTESIAN_POINT('Ctrl Pts',(54.5187124729514,18.5958530382746,11.3326100569557));
#39777=CARTESIAN_POINT('Ctrl Pts',(54.4391101968478,18.6131657708415,11.3283925049616));
#39778=CARTESIAN_POINT('Ctrl Pts',(54.3605376804652,18.6344053196088,11.3241749529675));
#39779=CARTESIAN_POINT('Ctrl Pts',(54.28199110694,18.6556378555602,11.3199587935132));
#39780=CARTESIAN_POINT('Ctrl Pts',(54.2044740663978,18.680794511728,11.3157426340588));
#39781=CARTESIAN_POINT('Ctrl Pts',(54.12840051971,18.7097457355223,11.3115264746044));
#39782=CARTESIAN_POINT('Ctrl Pts',(54.052328785701,18.7386962694676,11.3073104156126));
#39783=CARTESIAN_POINT('Ctrl Pts',(53.977700911284,18.7714410248668,11.3030943566208));
#39784=CARTESIAN_POINT('Ctrl Pts',(53.9049123089564,18.8078017427877,11.298878297629));
#39785=CARTESIAN_POINT('Ctrl Pts',(53.8315278854098,18.8444600964178,11.2946277275004));
#39786=CARTESIAN_POINT('Ctrl Pts',(53.760013420497,18.8847936837206,11.2903771573719));
#39787=CARTESIAN_POINT('Ctrl Pts',(53.690748551739,18.9285727395763,11.2861265872433));
#39788=CARTESIAN_POINT('Ctrl Pts',(53.621946170427,18.972059478936,11.2819043985346));
#39789=CARTESIAN_POINT('Ctrl Pts',(53.5553637835531,19.0189454947302,11.2776822098259));
#39790=CARTESIAN_POINT('Ctrl Pts',(53.491342515972,19.0689632717407,11.2734600211172));
#39791=CARTESIAN_POINT('Ctrl Pts',(53.4266757249664,19.1194853756401,11.2691952602787));
#39792=CARTESIAN_POINT('Ctrl Pts',(53.3646223585371,19.1732024330741,11.2649304994403));
#39793=CARTESIAN_POINT('Ctrl Pts',(53.3054965788037,19.2297998967478,11.2606657386018));
#39794=CARTESIAN_POINT('Ctrl Pts',(53.2463707990704,19.2863973604215,11.2564009777633));
#39795=CARTESIAN_POINT('Ctrl Pts',(53.1901728902236,19.3458748360093,11.2521362169248));
#39796=CARTESIAN_POINT('Ctrl Pts',(53.1371747641931,19.4078843035631,11.2478714560863));
#39797=CARTESIAN_POINT('Ctrl Pts',(53.084978212308,19.4689559042584,11.243671197944));
#39798=CARTESIAN_POINT('Ctrl Pts',(53.0356821499323,19.5327212540277,11.2394709398018));
#39799=CARTESIAN_POINT('Ctrl Pts',(52.989579824359,19.5988715378754,11.2352706816595));
#39800=CARTESIAN_POINT('Ctrl Pts',(52.9435395644599,19.6649327663031,11.2310760781529));
#39801=CARTESIAN_POINT('Ctrl Pts',(52.9006847776686,19.7333721750804,11.2268814746463));
#39802=CARTESIAN_POINT('Ctrl Pts',(52.861269680317,19.8038466362256,11.2226868711397));
#39803=CARTESIAN_POINT('Ctrl Pts',(52.821895136695,19.8742485870276,11.2184965834112));
#39804=CARTESIAN_POINT('Ctrl Pts',(52.7859534871032,19.9466810246936,11.2143062956827));
#39805=CARTESIAN_POINT('Ctrl Pts',(52.753655799209,20.0207717418433,11.2101160079543));
#39806=CARTESIAN_POINT('Ctrl Pts',(52.7200702369489,20.0978168356555,11.2057586319758));
#39807=CARTESIAN_POINT('Ctrl Pts',(52.6904256377389,20.1766547953242,11.2014012559973));
#39808=CARTESIAN_POINT('Ctrl Pts',(52.6649062967312,20.2568394204786,11.1970438800187));
#39809=CARTESIAN_POINT('Ctrl Pts',(52.6403884442667,20.3338772565604,11.1928575061879));
#39810=CARTESIAN_POINT('Ctrl Pts',(52.6196782504374,20.4121575423248,11.1886711323571));
#39811=CARTESIAN_POINT('Ctrl Pts',(52.6028890948132,20.4912667120831,11.1844847585263));
#39812=CARTESIAN_POINT('Ctrl Pts',(52.5861014055014,20.5703689726942,11.1802987503203));
#39813=CARTESIAN_POINT('Ctrl Pts',(52.5732341644404,20.6502995101256,11.1761127421143));
#39814=CARTESIAN_POINT('Ctrl Pts',(52.5643497089472,20.7306342455053,11.1719267339082));
#39815=CARTESIAN_POINT('Ctrl Pts',(52.5554609560948,20.8110078383281,11.1677387009544));
#39816=CARTESIAN_POINT('Ctrl Pts',(52.5505588735669,20.8917855489702,11.1635506680006));
#39817=CARTESIAN_POINT('Ctrl Pts',(52.5496538719983,20.9725390643463,11.1593626350468));
#39818=CARTESIAN_POINT('Ctrl Pts',(52.5495432947839,20.9824058967282,11.1588509221019));
#39819=CARTESIAN_POINT('Ctrl Pts',(52.5494923263623,20.9922723686099,11.158339209157));
#39820=CARTESIAN_POINT('Ctrl Pts',(52.5495009324145,21.0021377003384,11.1578274962121));
#39821=CARTESIAN_POINT('',(52.5495000019056,20.9999033600977,10.3578274961648));
#39822=CARTESIAN_POINT('Ctrl Pts',(52.5495009324152,21.0021377010802,11.1578274961736));
#39823=CARTESIAN_POINT('Ctrl Pts',(52.5495871706129,21.1009946578049,11.152699803984));
#39824=CARTESIAN_POINT('Ctrl Pts',(52.5556592523511,21.1995889286046,11.1475721117945));
#39825=CARTESIAN_POINT('Ctrl Pts',(52.5675996184674,21.2972854418235,11.1424444196049));
#39826=CARTESIAN_POINT('Ctrl Pts',(52.5797203219372,21.3964574818786,11.1372392830196));
#39827=CARTESIAN_POINT('Ctrl Pts',(52.5978878444661,21.494704482279,11.1320341464343));
#39828=CARTESIAN_POINT('Ctrl Pts',(52.6219304938964,21.5913845399908,11.126829009849));
#39829=CARTESIAN_POINT('Ctrl Pts',(52.6311544509903,21.6284758225782,11.1248320603584));
#39830=CARTESIAN_POINT('Ctrl Pts',(52.6412426517189,21.6653366993448,11.1228351108679));
#39831=CARTESIAN_POINT('Ctrl Pts',(52.6521835550092,21.7019317563914,11.1208381613774));
#39832=CARTESIAN_POINT('Ctrl Pts',(52.6753655996086,21.779470897545,11.1166069410728));
#39833=CARTESIAN_POINT('Ctrl Pts',(52.7024364554993,21.8560057658528,11.1123757207682));
#39834=CARTESIAN_POINT('Ctrl Pts',(52.7332910592392,21.9311180525987,11.1081445004636));
#39835=CARTESIAN_POINT('Ctrl Pts',(52.764101419637,22.0061226335826,11.1039193474328));
#39836=CARTESIAN_POINT('Ctrl Pts',(52.7986845770104,22.0797082579402,11.0996941944019));
#39837=CARTESIAN_POINT('Ctrl Pts',(52.836885599102,22.1514713798561,11.0954690413711));
#39838=CARTESIAN_POINT('Ctrl Pts',(52.875184758085,22.2234188583499,11.0912330340918));
#39839=CARTESIAN_POINT('Ctrl Pts',(52.9171202525201,22.2935340081507,11.0869970268126));
#39840=CARTESIAN_POINT('Ctrl Pts',(52.9624871569658,22.3614300071875,11.0827610195333));
#39841=CARTESIAN_POINT('Ctrl Pts',(53.0076564085001,22.4290301993572,11.0785434675394));
#39842=CARTESIAN_POINT('Ctrl Pts',(53.056226979573,22.4944301435069,11.0743259155456));
#39843=CARTESIAN_POINT('Ctrl Pts',(53.1079513664885,22.5572739702529,11.0701083635518));
#39844=CARTESIAN_POINT('Ctrl Pts',(53.1596586751881,22.620097047397,11.0658922040976));
#39845=CARTESIAN_POINT('Ctrl Pts',(53.2145174365962,22.6803653244593,11.0616760446435));
#39846=CARTESIAN_POINT('Ctrl Pts',(53.2722390558199,22.7377549797845,11.0574598851894));
#39847=CARTESIAN_POINT('Ctrl Pts',(53.3299592996544,22.7951432676306,11.0532438261978));
#39848=CARTESIAN_POINT('Ctrl Pts',(53.3905419351955,22.8496527431039,11.0490277672062));
#39849=CARTESIAN_POINT('Ctrl Pts',(53.4536616286813,22.9009965521767,11.0448117082146));
#39850=CARTESIAN_POINT('Ctrl Pts',(53.5172979971973,22.9527606431399,11.0405611380858));
#39851=CARTESIAN_POINT('Ctrl Pts',(53.5835127882373,23.0013066873144,11.0363105679569));
#39852=CARTESIAN_POINT('Ctrl Pts',(53.6519402353701,23.0463834247242,11.032059997828));
#39853=CARTESIAN_POINT('Ctrl Pts',(53.7199107865843,23.0911591809019,11.0278378091196));
#39854=CARTESIAN_POINT('Ctrl Pts',(53.7900640998296,23.1325116337779,11.0236156204111));
#39855=CARTESIAN_POINT('Ctrl Pts',(53.8620158781113,23.1702401683521,11.0193934317027));
#39856=CARTESIAN_POINT('Ctrl Pts',(53.9346931427967,23.20834911797,11.0151286708636));
#39857=CARTESIAN_POINT('Ctrl Pts',(54.0092049032931,23.2427604546778,11.0108639100245));
#39858=CARTESIAN_POINT('Ctrl Pts',(54.0851351159479,23.2733175083847,11.0065991491855));
#39859=CARTESIAN_POINT('Ctrl Pts',(54.1610653286027,23.3038745620916,11.0023343883464));
#39860=CARTESIAN_POINT('Ctrl Pts',(54.2384135170271,23.3305772363051,10.9980696275074));
#39861=CARTESIAN_POINT('Ctrl Pts',(54.3167505443871,23.3533211492282,10.9938048666683));
#39862=CARTESIAN_POINT('Ctrl Pts',(54.3944714842643,23.375886190926,10.9895736463638));
#39863=CARTESIAN_POINT('Ctrl Pts',(54.4734571969759,23.394639177157,10.9853424260592));
#39864=CARTESIAN_POINT('Ctrl Pts',(54.55329923705,23.4094415698207,10.9811112057547));
#39865=CARTESIAN_POINT('Ctrl Pts',(54.6330267892266,23.4242227368892,10.9768860527239));
#39866=CARTESIAN_POINT('Ctrl Pts',(54.7136077767622,23.4350644772212,10.9726608996931));
#39867=CARTESIAN_POINT('Ctrl Pts',(54.7946191185351,23.4418781590261,10.9684357466624));
#39868=CARTESIAN_POINT('Ctrl Pts',(54.875838575193,23.448709344906,10.9641997393831));
#39869=CARTESIAN_POINT('Ctrl Pts',(54.9574901449595,23.4514916244867,10.9599637321038));
#39870=CARTESIAN_POINT('Ctrl Pts',(55.0391376911991,23.4501874399987,10.9557277248245));
#39871=CARTESIAN_POINT('Ctrl Pts',(55.1204295183194,23.4488889375353,10.9515101728307));
#39872=CARTESIAN_POINT('Ctrl Pts',(55.2017168889558,23.4435395035627,10.947292620837));
#39873=CARTESIAN_POINT('Ctrl Pts',(55.2825665871558,23.4341541392901,10.9430750688432));
#39874=CARTESIAN_POINT('Ctrl Pts',(55.3633895906246,23.4247718738513,10.9388589093892));
#39875=CARTESIAN_POINT('Ctrl Pts',(55.4437747471745,23.4113563779819,10.9346427499351));
#39876=CARTESIAN_POINT('Ctrl Pts',(55.5232934879438,23.3939745561462,10.9304265904811));
#39877=CARTESIAN_POINT('Ctrl Pts',(55.6028103339426,23.3765931484842,10.9262105314896));
#39878=CARTESIAN_POINT('Ctrl Pts',(55.6814603512475,23.3552457031302,10.9219944724981));
#39879=CARTESIAN_POINT('Ctrl Pts',(55.7588261118878,23.3300500385007,10.9177784135066));
#39880=CARTESIAN_POINT('Ctrl Pts',(55.8368251607256,23.304648131253,10.9135278433777));
#39881=CARTESIAN_POINT('Ctrl Pts',(55.9135183698222,23.2753348469565,10.9092772732488));
#39882=CARTESIAN_POINT('Ctrl Pts',(55.9884962951118,23.2422812768585,10.9050267031198));
#39883=CARTESIAN_POINT('Ctrl Pts',(56.0629735863762,23.2094484082775,10.9008045144115));
#39884=CARTESIAN_POINT('Ctrl Pts',(56.1357580383577,23.1729253160255,10.8965823257031));
#39885=CARTESIAN_POINT('Ctrl Pts',(56.2064727130147,23.1329261221972,10.8923601369948));
#39886=CARTESIAN_POINT('Ctrl Pts',(56.2779004004225,23.0925236183718,10.8880953761555));
#39887=CARTESIAN_POINT('Ctrl Pts',(56.3472159263617,23.0485747798123,10.8838306153163));
#39888=CARTESIAN_POINT('Ctrl Pts',(56.4140620631266,23.0013442311672,10.8795658544771));
#39889=CARTESIAN_POINT('Ctrl Pts',(56.4809081998916,22.954113682522,10.8753010936378));
#39890=CARTESIAN_POINT('Ctrl Pts',(56.5452846080975,22.9036017717496,10.8710363327986));
#39891=CARTESIAN_POINT('Ctrl Pts',(56.6068708951037,22.8501124767074,10.8667715719594));
#39892=CARTESIAN_POINT('Ctrl Pts',(56.6679728321258,22.7970438522474,10.8625403516524));
#39893=CARTESIAN_POINT('Ctrl Pts',(56.7265575327523,22.7408455411942,10.8583091313454));
#39894=CARTESIAN_POINT('Ctrl Pts',(56.7822871243166,22.6817856154978,10.8540779110384));
#39895=CARTESIAN_POINT('Ctrl Pts',(56.8379368035473,22.6228103776011,10.8498527580051));
#39896=CARTESIAN_POINT('Ctrl Pts',(56.8907391883744,22.5609820099245,10.8456276049719));
#39897=CARTESIAN_POINT('Ctrl Pts',(56.9403904034097,22.4966079420996,10.8414024519387));
#39898=CARTESIAN_POINT('Ctrl Pts',(56.9901691703871,22.4320684999255,10.83716644466));
#39899=CARTESIAN_POINT('Ctrl Pts',(57.0367802042399,22.3649705756235,10.8329304373813));
#39900=CARTESIAN_POINT('Ctrl Pts',(57.0799554647948,22.2956602619786,10.8286944301026));
#39901=CARTESIAN_POINT('Ctrl Pts',(57.1229426209447,22.2266519169874,10.8244768781064));
#39902=CARTESIAN_POINT('Ctrl Pts',(57.1625236247463,22.1554508129655,10.8202593261102));
#39903=CARTESIAN_POINT('Ctrl Pts',(57.1984761815963,22.0824290872633,10.8160417741139));
#39904=CARTESIAN_POINT('Ctrl Pts',(57.2344168677299,22.0094314716739,10.8118256146574));
#39905=CARTESIAN_POINT('Ctrl Pts',(57.2667312808295,21.9346148449387,10.8076094552009));
#39906=CARTESIAN_POINT('Ctrl Pts',(57.295243256997,21.8583755828364,10.8033932957444));
#39907=CARTESIAN_POINT('Ctrl Pts',(57.3237545537818,21.7821381373614,10.7991772367505));
#39908=CARTESIAN_POINT('Ctrl Pts',(57.3484634319622,21.7044785597722,10.7949611777565));
#39909=CARTESIAN_POINT('Ctrl Pts',(57.369242548178,21.6258114715336,10.7907451187626));
#39910=CARTESIAN_POINT('Ctrl Pts',(57.3901917547139,21.5465004430002,10.7864945486366));
#39911=CARTESIAN_POINT('Ctrl Pts',(57.4071464290845,21.4661657931605,10.7822439785105));
#39912=CARTESIAN_POINT('Ctrl Pts',(57.4200283186945,21.3852443208103,10.7779934083845));
#39913=CARTESIAN_POINT('Ctrl Pts',(57.4328241948411,21.3048631679564,10.7737712196737));
#39914=CARTESIAN_POINT('Ctrl Pts',(57.4416015201006,21.2239034786879,10.769549030963));
#39915=CARTESIAN_POINT('Ctrl Pts',(57.4463358233932,21.1427980713562,10.7653268422522));
#39916=CARTESIAN_POINT('Ctrl Pts',(57.4511178624351,21.0608748821574,10.7610620814186));
#39917=CARTESIAN_POINT('Ctrl Pts',(57.4517748855337,20.978803505601,10.7567973205849));
#39918=CARTESIAN_POINT('Ctrl Pts',(57.4483355430156,20.897027582302,10.7525325597513));
#39919=CARTESIAN_POINT('Ctrl Pts',(57.4448962004975,20.815251659003,10.7482677989176));
#39920=CARTESIAN_POINT('Ctrl Pts',(57.437360600708,20.7337716627951,10.744003038084));
#39921=CARTESIAN_POINT('Ctrl Pts',(57.425810432708,20.6530216223381,10.7397382772503));
#39922=CARTESIAN_POINT('Ctrl Pts',(57.4143511018711,20.5729066466346,10.7355070569483));
#39923=CARTESIAN_POINT('Ctrl Pts',(57.3988971971231,20.4932097575724,10.7312758366463));
#39924=CARTESIAN_POINT('Ctrl Pts',(57.37949076006,20.4143602021813,10.7270446163443));
#39925=CARTESIAN_POINT('Ctrl Pts',(57.3601121504693,20.3356237115338,10.7228194633161));
#39926=CARTESIAN_POINT('Ctrl Pts',(57.3367923751243,20.257732589083,10.7185943102879));
#39927=CARTESIAN_POINT('Ctrl Pts',(57.3096249794038,20.1811088567375,10.7143691572596));
#39928=CARTESIAN_POINT('Ctrl Pts',(57.2823877917139,20.104288281042,10.7101331499797));
#39929=CARTESIAN_POINT('Ctrl Pts',(57.2512832627651,20.028742081885,10.7058971426998));
#39930=CARTESIAN_POINT('Ctrl Pts',(57.216456854722,19.9548831351683,10.7016611354198));
#39931=CARTESIAN_POINT('Ctrl Pts',(57.1817821771579,19.8813459745324,10.6974435834286));
#39932=CARTESIAN_POINT('Ctrl Pts',(57.1434181757188,19.809481821746,10.6932260314373));
#39933=CARTESIAN_POINT('Ctrl Pts',(57.101557000381,19.7396792375948,10.689008479446));
#39934=CARTESIAN_POINT('Ctrl Pts',(57.0597096466508,19.6698997006687,10.6847923199944));
#39935=CARTESIAN_POINT('Ctrl Pts',(57.0143676509957,19.6021807790421,10.6805761605429));
#39936=CARTESIAN_POINT('Ctrl Pts',(56.9657685424522,19.536885415456,10.6763600010913));
#39937=CARTESIAN_POINT('Ctrl Pts',(56.9171705919267,19.4715916077256,10.6721439421022));
#39938=CARTESIAN_POINT('Ctrl Pts',(56.8653159613015,19.4087216155108,10.6679278831131));
#39939=CARTESIAN_POINT('Ctrl Pts',(56.8104839818457,19.3486072540186,10.6637118241241));
#39940=CARTESIAN_POINT('Ctrl Pts',(56.7552031675232,19.2880008179797,10.6594612539922));
#39941=CARTESIAN_POINT('Ctrl Pts',(56.696896347794,19.2301956993413,10.6552106838603));
#39942=CARTESIAN_POINT('Ctrl Pts',(56.6358881061925,19.1754944905488,10.6509601137284));
#39943=CARTESIAN_POINT('Ctrl Pts',(56.575287221918,19.1211585264775,10.6467379250224));
#39944=CARTESIAN_POINT('Ctrl Pts',(56.5120212848464,19.06988539592,10.6425157363164));
#39945=CARTESIAN_POINT('Ctrl Pts',(56.4464406955112,19.0219303439037,10.6382935476104));
#39946=CARTESIAN_POINT('Ctrl Pts',(56.3801988600434,18.9734917632548,10.6340287867655));
#39947=CARTESIAN_POINT('Ctrl Pts',(56.3115958385816,18.9284388165062,10.6297640259207));
#39948=CARTESIAN_POINT('Ctrl Pts',(56.2410199284995,18.886987982271,10.6254992650758));
#39949=CARTESIAN_POINT('Ctrl Pts',(56.1704440184173,18.8455371480358,10.621234504231));
#39950=CARTESIAN_POINT('Ctrl Pts',(56.0978956765939,18.8076885922014,10.6169697433862));
#39951=CARTESIAN_POINT('Ctrl Pts',(56.023783882858,18.7736090165471,10.6127049825413));
#39952=CARTESIAN_POINT('Ctrl Pts',(55.9502549470577,18.7397974623522,10.6084737622381));
#39953=CARTESIAN_POINT('Ctrl Pts',(55.8749113572368,18.7095689861589,10.6042425419349));
#39954=CARTESIAN_POINT('Ctrl Pts',(55.7981365778044,18.6831210102444,10.6000113216317));
#39955=CARTESIAN_POINT('Ctrl Pts',(55.7214718880329,18.6567109588765,10.5957861686022));
#39956=CARTESIAN_POINT('Ctrl Pts',(55.6433805203861,18.6340707914778,10.5915610155728));
#39957=CARTESIAN_POINT('Ctrl Pts',(55.5642677949466,18.6153507374068,10.5873358625434));
#39958=CARTESIAN_POINT('Ctrl Pts',(55.4849518320595,18.596582592261,10.5830998552638));
#39959=CARTESIAN_POINT('Ctrl Pts',(55.4046096885351,18.5817549188206,10.5788638479842));
#39960=CARTESIAN_POINT('Ctrl Pts',(55.3236671500716,18.5709693649596,10.5746278407045));
#39961=CARTESIAN_POINT('Ctrl Pts',(55.2430772592082,18.5602308012198,10.5704102887122));
#39962=CARTESIAN_POINT('Ctrl Pts',(55.1618926567472,18.5534992792872,10.5661927367199));
#39963=CARTESIAN_POINT('Ctrl Pts',(55.080544013118,18.5508240340982,10.5619751847275));
#39964=CARTESIAN_POINT('Ctrl Pts',(54.9992222289608,18.5481496722144,10.5577590252749));
#39965=CARTESIAN_POINT('Ctrl Pts',(54.9177369755005,18.5495289427011,10.5535428658223));
#39966=CARTESIAN_POINT('Ctrl Pts',(54.8365220034965,18.5549590607396,10.5493267063697));
#39967=CARTESIAN_POINT('Ctrl Pts',(54.755308966681,18.5603890493895,10.5451106473797));
#39968=CARTESIAN_POINT('Ctrl Pts',(54.674366662329,18.5698696615555,10.5408945883897));
#39969=CARTESIAN_POINT('Ctrl Pts',(54.5941253528281,18.5833461106764,10.5366785293996));
#39970=CARTESIAN_POINT('Ctrl Pts',(54.5132272168649,18.5969328731565,10.532427959269));
#39971=CARTESIAN_POINT('Ctrl Pts',(54.4330420806568,18.6145811278778,10.5281773891384));
#39972=CARTESIAN_POINT('Ctrl Pts',(54.3540001893596,18.6361822205059,10.5239268190078));
#39973=CARTESIAN_POINT('Ctrl Pts',(54.2754860675948,18.6576390807735,10.5197046303009));
#39974=CARTESIAN_POINT('Ctrl Pts',(54.1981003970615,18.6829959478841,10.5154824415941));
#39975=CARTESIAN_POINT('Ctrl Pts',(54.1222476384813,18.7120968023432,10.5112602528872));
#39976=CARTESIAN_POINT('Ctrl Pts',(54.0456300600057,18.7414910793867,10.5069954920448));
#39977=CARTESIAN_POINT('Ctrl Pts',(53.9705769242785,18.7747050730503,10.5027307312023));
#39978=CARTESIAN_POINT('Ctrl Pts',(53.897480667602,18.8115299015777,10.4984659703598));
#39979=CARTESIAN_POINT('Ctrl Pts',(53.8243844109255,18.8483547301051,10.4942012095173));
#39980=CARTESIAN_POINT('Ctrl Pts',(53.7532454204141,18.8887900995583,10.4899364486748));
#39981=CARTESIAN_POINT('Ctrl Pts',(53.6844255225931,18.9325827599646,10.4856716878324));
#39982=CARTESIAN_POINT('Ctrl Pts',(53.6161468638785,18.9760310097988,10.4814404675126));
#39983=CARTESIAN_POINT('Ctrl Pts',(53.5498948890266,19.0229468192873,10.4772092471929));
#39984=CARTESIAN_POINT('Ctrl Pts',(53.4860434019957,19.0731150347363,10.4729780268731));
#39985=CARTESIAN_POINT('Ctrl Pts',(53.4222834735272,19.1232113124765,10.4687528738271));
#39986=CARTESIAN_POINT('Ctrl Pts',(53.3609175590427,19.176550448862,10.4645277207811));
#39987=CARTESIAN_POINT('Ctrl Pts',(53.3022916599641,19.2328733372584,10.4603025677351));
#39988=CARTESIAN_POINT('Ctrl Pts',(53.2435151535691,19.2893409166395,10.4560665604596));
#39989=CARTESIAN_POINT('Ctrl Pts',(53.1874931533305,19.3488073390837,10.4518305531841));
#39990=CARTESIAN_POINT('Ctrl Pts',(53.1345419376873,19.410969960085,10.4475945459086));
#39991=CARTESIAN_POINT('Ctrl Pts',(53.0818214177749,19.4728617534743,10.4433769938996));
#39992=CARTESIAN_POINT('Ctrl Pts',(53.0321452905348,19.5374259501685,10.4391594418906));
#39993=CARTESIAN_POINT('Ctrl Pts',(52.9857884438147,19.6043273818944,10.4349418898816));
#39994=CARTESIAN_POINT('Ctrl Pts',(52.9394469030711,19.6712067242892,10.4307257304123));
#39995=CARTESIAN_POINT('Ctrl Pts',(52.8964227310292,19.7404213873773,10.426509570943));
#39996=CARTESIAN_POINT('Ctrl Pts',(52.8569487769205,19.8116054084365,10.4222934114738));
#39997=CARTESIAN_POINT('Ctrl Pts',(52.8174757633966,19.8827877333238,10.4180773524671));
#39998=CARTESIAN_POINT('Ctrl Pts',(52.781553024109,19.9559389157528,10.4138612934604));
#39999=CARTESIAN_POINT('Ctrl Pts',(52.7493678231144,20.0306677275737,10.4096452344537));
#40000=CARTESIAN_POINT('Ctrl Pts',(52.716919165934,20.1060082418888,10.4053946643429));
#40001=CARTESIAN_POINT('Ctrl Pts',(52.6882697221966,20.1829518983535,10.401144094232));
#40002=CARTESIAN_POINT('Ctrl Pts',(52.6635614850033,20.2610782750249,10.3968935241212));
#40003=CARTESIAN_POINT('Ctrl Pts',(52.6390182266337,20.3386829957958,10.3926713353979));
#40004=CARTESIAN_POINT('Ctrl Pts',(52.6183637628908,20.4174542208098,10.3884491466747));
#40005=CARTESIAN_POINT('Ctrl Pts',(52.6016863081134,20.4969675106823,10.3842269579514));
#40006=CARTESIAN_POINT('Ctrl Pts',(52.584840695537,20.5772825283961,10.3799621971467));
#40007=CARTESIAN_POINT('Ctrl Pts',(52.5720528189215,20.6583541797246,10.3756974363421));
#40008=CARTESIAN_POINT('Ctrl Pts',(52.5633599559602,20.7397394655701,10.3714326755374));
#40009=CARTESIAN_POINT('Ctrl Pts',(52.5546670929989,20.8211247514157,10.3671679147327));
#40010=CARTESIAN_POINT('Ctrl Pts',(52.5500692066164,20.9028231871315,10.3629031539281));
#40011=CARTESIAN_POINT('Ctrl Pts',(52.5495496974743,20.984393435621,10.3586383931234));
#40012=CARTESIAN_POINT('Ctrl Pts',(52.549516771176,20.989563327954,10.358368094153));
#40013=CARTESIAN_POINT('Ctrl Pts',(52.5495002057972,20.9947333245982,10.3580977951825));
#40014=CARTESIAN_POINT('Ctrl Pts',(52.5495000019056,20.9999033591928,10.3578274962121));
#40015=CARTESIAN_POINT('',(52.5495008814216,20.9979215759409,9.55782751980551));
#40016=CARTESIAN_POINT('Ctrl Pts',(52.5495000019056,20.9999033600977,10.3578274961648));
#40017=CARTESIAN_POINT('Ctrl Pts',(52.5494968138749,21.0807423211251,10.3536010857728));
#40018=CARTESIAN_POINT('Ctrl Pts',(52.5534980935076,21.1617346655812,10.3493746753808));
#40019=CARTESIAN_POINT('Ctrl Pts',(52.5615234123392,21.242450369004,10.3451482649887));
#40020=CARTESIAN_POINT('Ctrl Pts',(52.5695372224051,21.3230503214972,10.3409279155107));
#40021=CARTESIAN_POINT('Ctrl Pts',(52.5815635655934,21.4033739609398,10.3367075660326));
#40022=CARTESIAN_POINT('Ctrl Pts',(52.5975700052744,21.4829910666281,10.3324872165545));
#40023=CARTESIAN_POINT('Ctrl Pts',(52.6135579296484,21.5625160759366,10.3282717489282));
#40024=CARTESIAN_POINT('Ctrl Pts',(52.6335167096718,21.6413357210847,10.3240562813019));
#40025=CARTESIAN_POINT('Ctrl Pts',(52.6573622609584,21.7190261981445,10.3198408136756));
#40026=CARTESIAN_POINT('Ctrl Pts',(52.6811926990023,21.7966674352005,10.3156280178007));
#40027=CARTESIAN_POINT('Ctrl Pts',(52.7089048822194,21.8731804803106,10.3114152219258));
#40028=CARTESIAN_POINT('Ctrl Pts',(52.7403641984882,21.9481541512465,10.307202426051));
#40029=CARTESIAN_POINT('Ctrl Pts',(52.771813273478,22.0231034152221,10.3029910016114));
#40030=CARTESIAN_POINT('Ctrl Pts',(52.807006878973,22.0965138706649,10.2987795771719));
#40031=CARTESIAN_POINT('Ctrl Pts',(52.845761842108,22.1679932401696,10.2945681527323));
#40032=CARTESIAN_POINT('Ctrl Pts',(52.8845161352268,22.2394713739015,10.2903568011021));
#40033=CARTESIAN_POINT('Ctrl Pts',(52.926831440305,22.3090180788987,10.2861454494719));
#40034=CARTESIAN_POINT('Ctrl Pts',(52.9724787890595,22.3762659587399,10.2819340978416));
#40035=CARTESIAN_POINT('Ctrl Pts',(53.0181712833848,22.4435803472396,10.277718581153));
#40036=CARTESIAN_POINT('Ctrl Pts',(53.0672021422222,22.508590982125,10.2735030644644));
#40037=CARTESIAN_POINT('Ctrl Pts',(53.1192995361303,22.5709602207568,10.2692875477758));
#40038=CARTESIAN_POINT('Ctrl Pts',(53.1714214988697,22.6333588723628,10.2650700430737));
#40039=CARTESIAN_POINT('Ctrl Pts',(53.2266125609176,22.6931133033122,10.2608525383716));
#40040=CARTESIAN_POINT('Ctrl Pts',(53.2845628387948,22.7499215970884,10.2566350336696));
#40041=CARTESIAN_POINT('Ctrl Pts',(53.3426183863275,22.8068330860473,10.2524098676537));
#40042=CARTESIAN_POINT('Ctrl Pts',(53.4034428159728,22.8607874332666,10.2481847016378));
#40043=CARTESIAN_POINT('Ctrl Pts',(53.4666919790198,22.9115221062802,10.2439595356219));
#40044=CARTESIAN_POINT('Ctrl Pts',(53.5283390882967,22.9609717081519,10.239841389886));
#40045=CARTESIAN_POINT('Ctrl Pts',(53.5922891706085,23.0073626493486,10.2357232441502));
#40046=CARTESIAN_POINT('Ctrl Pts',(53.6581991488266,23.0504928007165,10.2316050984144));
#40047=CARTESIAN_POINT('Ctrl Pts',(53.7259188595341,23.0948072042769,10.2273738781133));
#40048=CARTESIAN_POINT('Ctrl Pts',(53.7959631933162,23.1358463147716,10.2231426578122));
#40049=CARTESIAN_POINT('Ctrl Pts',(53.8679821008772,23.1733581679202,10.2189114375111));
#40050=CARTESIAN_POINT('Ctrl Pts',(53.9398977383606,23.2108162316944,10.2146862844841));
#40051=CARTESIAN_POINT('Ctrl Pts',(54.0137819173865,23.2447568704125,10.210461131457));
#40052=CARTESIAN_POINT('Ctrl Pts',(54.0892559936636,23.2749715613436,10.20623597843));
#40053=CARTESIAN_POINT('Ctrl Pts',(54.1649239598955,23.305263872636,10.2019999711498));
#40054=CARTESIAN_POINT('Ctrl Pts',(54.2421896041229,23.3318108149255,10.1977639638696));
#40055=CARTESIAN_POINT('Ctrl Pts',(54.3206468564639,23.354448885911,10.1935279565894));
#40056=CARTESIAN_POINT('Ctrl Pts',(54.3987622889479,23.3769883281279,10.1893104046));
#40057=CARTESIAN_POINT('Ctrl Pts',(54.4780585208188,23.3956527505162,10.1850928526105));
#40058=CARTESIAN_POINT('Ctrl Pts',(54.5581168994866,23.410329764883,10.1808753006211));
#40059=CARTESIAN_POINT('Ctrl Pts',(54.6381488446949,23.4250019332327,10.1766591411716));
#40060=CARTESIAN_POINT('Ctrl Pts',(54.7189419800299,23.435689224277,10.1724429817221));
#40061=CARTESIAN_POINT('Ctrl Pts',(54.8000669129004,23.4423302419376,10.1682268222726));
#40062=CARTESIAN_POINT('Ctrl Pts',(54.881189912724,23.4489711013558,10.1640107632858));
#40063=CARTESIAN_POINT('Ctrl Pts',(54.9626442309016,23.4515658422601,10.1597947042991));
#40064=CARTESIAN_POINT('Ctrl Pts',(55.0439962339691,23.4501050143609,10.1555786453123));
#40065=CARTESIAN_POINT('Ctrl Pts',(55.1260141553641,23.4486322286484,10.1513280751784));
#40066=CARTESIAN_POINT('Ctrl Pts',(55.2079275989598,23.4430371653713,10.1470775050445));
#40067=CARTESIAN_POINT('Ctrl Pts',(55.2892949814708,23.4333636521687,10.1428269349106));
#40068=CARTESIAN_POINT('Ctrl Pts',(55.3701190668101,23.4237547298649,10.1386047462075));
#40069=CARTESIAN_POINT('Ctrl Pts',(55.4504039085215,23.4101217956555,10.1343825575043));
#40070=CARTESIAN_POINT('Ctrl Pts',(55.5297264190529,23.3925593348875,10.1301603688011));
#40071=CARTESIAN_POINT('Ctrl Pts',(55.6098487350281,23.374819792587,10.1258956079519));
#40072=CARTESIAN_POINT('Ctrl Pts',(55.6889887358762,23.3530711639465,10.1216308471026));
#40073=CARTESIAN_POINT('Ctrl Pts',(55.7667274080766,23.3274619936111,10.1173660862533));
#40074=CARTESIAN_POINT('Ctrl Pts',(55.844466080277,23.3018528232757,10.113101325404));
#40075=CARTESIAN_POINT('Ctrl Pts',(55.9208029975002,23.2723833446981,10.1088365645547));
#40076=CARTESIAN_POINT('Ctrl Pts',(55.9953428574725,23.239250509898,10.1045718037054));
#40077=CARTESIAN_POINT('Ctrl Pts',(56.0692964947102,23.2063782500578,10.100340583297));
#40078=CARTESIAN_POINT('Ctrl Pts',(56.141758576123,23.1697768240893,10.0961093628887));
#40079=CARTESIAN_POINT('Ctrl Pts',(56.2123275880256,23.1296037352785,10.0918781424803));
#40080=CARTESIAN_POINT('Ctrl Pts',(56.2827954089131,23.0894882518602,10.0876529893453));
#40081=CARTESIAN_POINT('Ctrl Pts',(56.3513751509179,23.0458115053795,10.0834278362102));
#40082=CARTESIAN_POINT('Ctrl Pts',(56.4176862966516,22.9987785806052,10.0792026830752));
#40083=CARTESIAN_POINT('Ctrl Pts',(56.4841677910085,22.9516248315881,10.074966675822));
#40084=CARTESIAN_POINT('Ctrl Pts',(56.5483685897364,22.9010978362283,10.0707306685687));
#40085=CARTESIAN_POINT('Ctrl Pts',(56.6099311324859,22.8474501342804,10.0664946613154));
#40086=CARTESIAN_POINT('Ctrl Pts',(56.6712254636377,22.7940361610775,10.0622771092172));
#40087=CARTESIAN_POINT('Ctrl Pts',(56.7299041211222,22.7375289179703,10.058059557119));
#40088=CARTESIAN_POINT('Ctrl Pts',(56.7856456698187,22.6782192323584,10.0538420050208));
#40089=CARTESIAN_POINT('Ctrl Pts',(56.8413688139224,22.6189291294571,10.0496258454624));
#40090=CARTESIAN_POINT('Ctrl Pts',(56.894156456908,22.5568387600887,10.0454096859041));
#40091=CARTESIAN_POINT('Ctrl Pts',(56.9437241855704,22.4922756248189,10.0411935263458));
#40092=CARTESIAN_POINT('Ctrl Pts',(56.9932907331308,22.4277140279624,10.0369774672503));
#40093=CARTESIAN_POINT('Ctrl Pts',(57.0396372366727,22.3606801518038,10.0327614081548));
#40094=CARTESIAN_POINT('Ctrl Pts',(57.0825206301869,22.2915332263809,10.0285453490593));
#40095=CARTESIAN_POINT('Ctrl Pts',(57.1257550493604,22.221820292928,10.0242947790541));
#40096=CARTESIAN_POINT('Ctrl Pts',(57.1654691351802,22.1499599566717,10.0200442090488));
#40097=CARTESIAN_POINT('Ctrl Pts',(57.2014602771032,22.0763470157605,10.0157936390436));
#40098=CARTESIAN_POINT('Ctrl Pts',(57.2372111049968,22.0032255908587,10.011571450233));
#40099=CARTESIAN_POINT('Ctrl Pts',(57.2692884259045,21.9283753503223,10.0073492614225));
#40100=CARTESIAN_POINT('Ctrl Pts',(57.2975422224359,21.852203019312,10.0031270726119));
#40101=CARTESIAN_POINT('Ctrl Pts',(57.3260808983991,21.7752626523898,9.99886231200933));
#40102=CARTESIAN_POINT('Ctrl Pts',(57.350718365958,21.6969738473857,9.99459755140675));
#40103=CARTESIAN_POINT('Ctrl Pts',(57.3713522393082,21.6177692183397,9.99033279080417));
#40104=CARTESIAN_POINT('Ctrl Pts',(57.3919861126584,21.5385645892937,9.9860680302016));
#40105=CARTESIAN_POINT('Ctrl Pts',(57.4086163567899,21.4584446210061,9.98180326959902));
#40106=CARTESIAN_POINT('Ctrl Pts',(57.4211941162249,21.3778482520243,9.97753850899644));
#40107=CARTESIAN_POINT('Ctrl Pts',(57.4336729570077,21.2978857387173,9.9733072888963));
#40108=CARTESIAN_POINT('Ctrl Pts',(57.4422096669418,21.2171544480391,9.96907606879615));
#40109=CARTESIAN_POINT('Ctrl Pts',(57.4467188763498,21.1360771476538,9.96484484869601));
#40110=CARTESIAN_POINT('Ctrl Pts',(57.451221619867,21.0551161064445,9.96061969586944));
#40111=CARTESIAN_POINT('Ctrl Pts',(57.4517083071476,20.9738105012146,9.95639454304287));
#40112=CARTESIAN_POINT('Ctrl Pts',(57.4481449328091,20.8925912575201,9.9521693902163));
#40113=CARTESIAN_POINT('Ctrl Pts',(57.4445724040893,20.8111633599318,9.94793338288593));
#40114=CARTESIAN_POINT('Ctrl Pts',(57.436928911295,20.7298227355339,9.94369737555556));
#40115=CARTESIAN_POINT('Ctrl Pts',(57.4252327702162,20.6490067518182,9.9394613682252));
#40116=CARTESIAN_POINT('Ctrl Pts',(57.4135875871669,20.5685428691288,9.9352438164337));
#40117=CARTESIAN_POINT('Ctrl Pts',(57.3979250544606,20.4885995293403,9.9310262646422));
#40118=CARTESIAN_POINT('Ctrl Pts',(57.3783152464065,20.4096045065293,9.9268087128507));
#40119=CARTESIAN_POINT('Ctrl Pts',(57.3587119130597,20.3306355660571,9.92259255359776));
#40120=CARTESIAN_POINT('Ctrl Pts',(57.33516400446,20.2526147716374,9.91837639434482));
#40121=CARTESIAN_POINT('Ctrl Pts',(57.3077924830991,20.1759586752162,9.91416023509187));
#40122=CARTESIAN_POINT('Ctrl Pts',(57.2804216139367,20.0993044053283,9.90994417630003));
#40123=CARTESIAN_POINT('Ctrl Pts',(57.2492274705443,20.0240152062594,9.90572811750818));
#40124=CARTESIAN_POINT('Ctrl Pts',(57.2143800949908,19.9504900929918,9.90151205871634));
#40125=CARTESIAN_POINT('Ctrl Pts',(57.179247467748,19.8763631219821,9.89726148834727));
#40126=CARTESIAN_POINT('Ctrl Pts',(57.1404017143843,19.8040296911584,9.8930109179782));
#40127=CARTESIAN_POINT('Ctrl Pts',(57.0980646984976,19.7338741093722,9.88876034760913));
#40128=CARTESIAN_POINT('Ctrl Pts',(57.0560103747993,19.6641869695517,9.8845381590949));
#40129=CARTESIAN_POINT('Ctrl Pts',(57.0105115838098,19.5966490383781,9.88031597058068));
#40130=CARTESIAN_POINT('Ctrl Pts',(56.9618287276784,19.5316069009778,9.87609378206645));
#40131=CARTESIAN_POINT('Ctrl Pts',(56.9126549970567,19.4659089366896,9.87182902076996));
#40132=CARTESIAN_POINT('Ctrl Pts',(56.8602329396191,19.4027577539757,9.86756425947346));
#40133=CARTESIAN_POINT('Ctrl Pts',(56.8048705373686,19.3424739539486,9.86329949817697));
#40134=CARTESIAN_POINT('Ctrl Pts',(56.7495081351182,19.2821901539216,9.85903473688047));
#40135=CARTESIAN_POINT('Ctrl Pts',(56.6912057764184,19.2247740288675,9.85476997558398));
#40136=CARTESIAN_POINT('Ctrl Pts',(56.6303057826845,19.1705046310675,9.85050521428748));
#40137=CARTESIAN_POINT('Ctrl Pts',(56.5698847474868,19.1166620443349,9.84627399394399));
#40138=CARTESIAN_POINT('Ctrl Pts',(56.5066802486927,19.0657149278249,9.8420427736005));
#40139=CARTESIAN_POINT('Ctrl Pts',(56.441001221378,19.0179642460372,9.83781155325701));
#40140=CARTESIAN_POINT('Ctrl Pts',(56.3754163732205,18.970282035406,9.8335864001892));
#40141=CARTESIAN_POINT('Ctrl Pts',(56.3073644166057,18.9257874274795,9.82936124712139));
#40142=CARTESIAN_POINT('Ctrl Pts',(56.2371889920002,18.884742652046,9.82513609405359));
#40143=CARTESIAN_POINT('Ctrl Pts',(56.1668332903206,18.8435924346851,9.82090008678379));
#40144=CARTESIAN_POINT('Ctrl Pts',(56.0943435531916,18.805910106625,9.816664079514));
#40145=CARTESIAN_POINT('Ctrl Pts',(56.020097203423,18.7719174284671,9.8124280722442));
#40146=CARTESIAN_POINT('Ctrl Pts',(55.9461743267744,18.7380728480635,9.80821052021823));
#40147=CARTESIAN_POINT('Ctrl Pts',(55.8705105338275,18.7078860370133,9.80399296819226));
#40148=CARTESIAN_POINT('Ctrl Pts',(55.7935032513437,18.6815300648689,9.79977541616629));
#40149=CARTESIAN_POINT('Ctrl Pts',(55.7165213949469,18.6551827948785,9.79555925668192));
#40150=CARTESIAN_POINT('Ctrl Pts',(55.6381973694481,18.6326640023938,9.79134309719755));
#40151=CARTESIAN_POINT('Ctrl Pts',(55.5589467650632,18.6140979140322,9.78712693771319));
#40152=CARTESIAN_POINT('Ctrl Pts',(55.4796980490954,18.5955322680713,9.78291087869327));
#40153=CARTESIAN_POINT('Ctrl Pts',(55.3995232510588,18.5809192439327,9.77869481967335));
#40154=CARTESIAN_POINT('Ctrl Pts',(55.318849838012,18.5703323209131,9.77447876065343));
#40155=CARTESIAN_POINT('Ctrl Pts',(55.2375160628204,18.5596587373329,9.77022819056385));
#40156=CARTESIAN_POINT('Ctrl Pts',(55.1556759455423,18.5530775497303,9.76597762047427));
#40157=CARTESIAN_POINT('Ctrl Pts',(55.0737726952354,18.5506107211311,9.7617270503847));
#40158=CARTESIAN_POINT('Ctrl Pts',(54.9924163187349,18.5481603637213,9.75750486165282));
#40159=CARTESIAN_POINT('Ctrl Pts',(54.9109981179188,18.5497695178218,9.75328267292095));
#40160=CARTESIAN_POINT('Ctrl Pts',(54.8299505016417,18.5554073103872,9.74906048418907));
#40161=CARTESIAN_POINT('Ctrl Pts',(54.7480856878631,18.5611019484247,9.74479572342064));
#40162=CARTESIAN_POINT('Ctrl Pts',(54.6665994561608,18.5709068651232,9.74053096265221));
#40163=CARTESIAN_POINT('Ctrl Pts',(54.5859281813169,18.5847371201104,9.73626620188378));
#40164=CARTESIAN_POINT('Ctrl Pts',(54.505256906473,18.5985673750977,9.73200144111536));
#40165=CARTESIAN_POINT('Ctrl Pts',(54.4254010446554,18.616422800541,9.72773668034693));
#40166=CARTESIAN_POINT('Ctrl Pts',(54.3467806794472,18.6381670742289,9.7234719195785));
#40167=CARTESIAN_POINT('Ctrl Pts',(54.2687786158218,18.6597403423662,9.71924069857201));
#40168=CARTESIAN_POINT('Ctrl Pts',(54.1917001746333,18.6852223634556,9.71500947756553));
#40169=CARTESIAN_POINT('Ctrl Pts',(54.1159657483402,18.7145167487176,9.71077825655904));
#40170=CARTESIAN_POINT('Ctrl Pts',(54.0403399198364,18.7437691279114,9.70655310282302));
#40171=CARTESIAN_POINT('Ctrl Pts',(53.966054708576,18.7768228477731,9.702327949087));
#40172=CARTESIAN_POINT('Ctrl Pts',(53.8935167787501,18.8135313560235,9.69810279535097));
#40173=CARTESIAN_POINT('Ctrl Pts',(53.8207925170533,18.8503341592867,9.69386678824758));
#40174=CARTESIAN_POINT('Ctrl Pts',(53.7498249781623,18.8908104194393,9.68963078114419));
#40175=CARTESIAN_POINT('Ctrl Pts',(53.6810051399095,18.9347632559305,9.68539477404079));
#40176=CARTESIAN_POINT('Ctrl Pts',(53.6124851191255,18.9785246094348,9.68117722133891));
#40177=CARTESIAN_POINT('Ctrl Pts',(53.546094523564,19.0257320657081,9.67695966863703));
#40178=CARTESIAN_POINT('Ctrl Pts',(53.4821942659225,19.0761455347139,9.67274211593515));
#40179=CARTESIAN_POINT('Ctrl Pts',(53.4183151066963,19.1265423583359,9.66852595577348));
#40180=CARTESIAN_POINT('Ctrl Pts',(53.3569250172281,19.1801428048135,9.66430979561181));
#40181=CARTESIAN_POINT('Ctrl Pts',(53.2983537192706,19.2366650388313,9.66009363545015));
#40182=CARTESIAN_POINT('Ctrl Pts',(53.2397838169685,19.2931859260194,9.65587757575247));
#40183=CARTESIAN_POINT('Ctrl Pts',(53.1840329064109,19.3526281386796,9.6516615160548));
#40184=CARTESIAN_POINT('Ctrl Pts',(53.1313945095377,19.4146723458496,9.64744545635713));
#40185=CARTESIAN_POINT('Ctrl Pts',(53.0783252530987,19.4772244016955,9.6431948870665));
#40186=CARTESIAN_POINT('Ctrl Pts',(53.0284200216479,19.5424208892982,9.63894431777586));
#40187=CARTESIAN_POINT('Ctrl Pts',(52.9819375867258,19.6099013178447,9.63469374848523));
#40188=CARTESIAN_POINT('Ctrl Pts',(52.9357655022891,19.6769311980541,9.63047155908142));
#40189=CARTESIAN_POINT('Ctrl Pts',(52.892970841555,19.746214181651,9.62624936967762));
#40190=CARTESIAN_POINT('Ctrl Pts',(52.8537621254998,19.8173702032923,9.62202718027381));
#40191=CARTESIAN_POINT('Ctrl Pts',(52.8141580912278,19.8892436488746,9.61776242103976));
#40192=CARTESIAN_POINT('Ctrl Pts',(52.7782129312753,19.9630276778113,9.61349766180572));
#40193=CARTESIAN_POINT('Ctrl Pts',(52.7460918875118,20.0383095765996,9.60923290257167));
#40194=CARTESIAN_POINT('Ctrl Pts',(52.7139708437484,20.1135914753878,9.60496814333762));
#40195=CARTESIAN_POINT('Ctrl Pts',(52.685674022499,20.1903707697382,9.60070338410357));
#40196=CARTESIAN_POINT('Ctrl Pts',(52.6613146594614,20.2682205742508,9.59643862486952));
#40197=CARTESIAN_POINT('Ctrl Pts',(52.6320142325393,20.3618614672617,9.59130880000159));
#40198=CARTESIAN_POINT('Ctrl Pts',(52.608319660546,20.4573346692796,9.58617897513365));
#40199=CARTESIAN_POINT('Ctrl Pts',(52.5904230808027,20.554029910788,9.58104915026572));
#40200=CARTESIAN_POINT('Ctrl Pts',(52.5727560657076,20.6494848142315,9.57598512715752));
#40201=CARTESIAN_POINT('Ctrl Pts',(52.5607392937498,20.7461305939467,9.57092110404933));
#40202=CARTESIAN_POINT('Ctrl Pts',(52.5545115088973,20.8433593606867,9.56585708094114));
#40203=CARTESIAN_POINT('Ctrl Pts',(52.5512198981138,20.894748299876,9.5631805605626));
#40204=CARTESIAN_POINT('Ctrl Pts',(52.549544665176,20.9462997469006,9.56050404018405));
#40205=CARTESIAN_POINT('Ctrl Pts',(52.5495008814216,20.9979215759409,9.55782751980551));
#40206=CARTESIAN_POINT('',(52.5495637068299,21.001288087881,8.75782746859915));
#40207=CARTESIAN_POINT('Ctrl Pts',(52.5511529243446,20.9979234318819,9.55782749621206));
#40208=CARTESIAN_POINT('Ctrl Pts',(52.5557236291845,21.5660081702359,9.52835344086155));
#40209=CARTESIAN_POINT('Ctrl Pts',(53.0353472451824,22.9572037199135,9.45653495394137));
#40210=CARTESIAN_POINT('Ctrl Pts',(55.3507382576877,23.8752188638192,9.34237203545155));
#40211=CARTESIAN_POINT('Ctrl Pts',(57.6060389677743,22.2643044328178,9.21533874074257));
#40212=CARTESIAN_POINT('Ctrl Pts',(57.4753636898807,19.4958460434894,9.08830544603359));
#40213=CARTESIAN_POINT('Ctrl Pts',(55.0783545536393,18.1045293080376,8.96127215132461));
#40214=CARTESIAN_POINT('Ctrl Pts',(52.9375321800744,19.1968516022151,8.85111283471743));
#40215=CARTESIAN_POINT('Ctrl Pts',(52.5551646396964,20.5095195307769,8.78329794967991));
#40216=CARTESIAN_POINT('Ctrl Pts',(52.5528298189475,21.0012858378839,8.75782749621206));
#40217=CARTESIAN_POINT('Ctrl Pts',(52.5495003385601,21.0012881315349,8.75782746806341));
#40218=CARTESIAN_POINT('Ctrl Pts',(52.5495477704209,21.0915209655461,8.75316030218582));
#40219=CARTESIAN_POINT('Ctrl Pts',(52.5545832033599,21.1815800967497,8.74849313630823));
#40220=CARTESIAN_POINT('Ctrl Pts',(52.5645245535201,21.2709420594764,8.74382597043064));
#40221=CARTESIAN_POINT('Ctrl Pts',(52.5745011987725,21.3606212868266,8.73914223456534));
#40222=CARTESIAN_POINT('Ctrl Pts',(52.5894185286338,21.4495981186264,8.73445849870003));
#40223=CARTESIAN_POINT('Ctrl Pts',(52.6091435960903,21.5373601268089,8.72977476283472));
#40224=CARTESIAN_POINT('Ctrl Pts',(52.6289649037067,21.6255503327513,8.72506817465271));
#40225=CARTESIAN_POINT('Ctrl Pts',(52.653640845938,21.7125135706083,8.7203615864707));
#40226=CARTESIAN_POINT('Ctrl Pts',(52.6829880937164,21.7977506353117,8.71565499828869));
#40227=CARTESIAN_POINT('Ctrl Pts',(52.7005498386225,21.8487575167122,8.71283851949467));
#40228=CARTESIAN_POINT('Ctrl Pts',(52.7197834453385,21.8991466775342,8.71002204070066));
#40229=CARTESIAN_POINT('Ctrl Pts',(52.7406417105928,21.9488152454968,8.70720556190665));
#40230=CARTESIAN_POINT('Ctrl Pts',(52.7719779732677,22.0234344563173,8.70297424553249));
#40231=CARTESIAN_POINT('Ctrl Pts',(52.807073594722,22.0966394811059,8.69874292915832));
#40232=CARTESIAN_POINT('Ctrl Pts',(52.8457793995175,22.168025622346,8.69451161278415));
#40233=CARTESIAN_POINT('Ctrl Pts',(52.8844296988496,22.2393093933893,8.69028636426409));
#40234=CARTESIAN_POINT('Ctrl Pts',(52.9266796796226,22.3087790560095,8.68606111574402));
#40235=CARTESIAN_POINT('Ctrl Pts',(52.9723321610904,22.3760499209882,8.68183586722395));
#40236=CARTESIAN_POINT('Ctrl Pts',(53.0181006288515,22.4434916966824,8.67759988388952));
#40237=CARTESIAN_POINT('Ctrl Pts',(53.0672887193487,22.5087230553778,8.6733639005551));
#40238=CARTESIAN_POINT('Ctrl Pts',(53.1196513535387,22.5713813088334,8.66912791722067));
#40239=CARTESIAN_POINT('Ctrl Pts',(53.1717873054375,22.6337683093875,8.66491027181791));
#40240=CARTESIAN_POINT('Ctrl Pts',(53.2270700786933,22.6936040725748,8.66069262641515));
#40241=CARTESIAN_POINT('Ctrl Pts',(53.2852155477713,22.7505612049839,8.65647498101239));
#40242=CARTESIAN_POINT('Ctrl Pts',(53.3433418054185,22.8074995185921,8.65225872913184));
#40243=CARTESIAN_POINT('Ctrl Pts',(53.4043285487249,22.8615607651248,8.6480424772513));
#40244=CARTESIAN_POINT('Ctrl Pts',(53.4678542208604,22.912453806361,8.64382622537076));
#40245=CARTESIAN_POINT('Ctrl Pts',(53.5313783627541,22.9633456216572,8.63961007505364));
#40246=CARTESIAN_POINT('Ctrl Pts',(53.5974409483611,23.0110690935869,8.63539392473653));
#40247=CARTESIAN_POINT('Ctrl Pts',(53.6656878424604,23.0553737655818,8.63117777441941));
#40248=CARTESIAN_POINT('Ctrl Pts',(53.7344900907205,23.1000389636382,8.62692731548427));
#40249=CARTESIAN_POINT('Ctrl Pts',(53.8055119663668,23.1412291913691,8.62267685654912));
#40250=CARTESIAN_POINT('Ctrl Pts',(53.8783629920347,23.1787337314052,8.61842639761398));
#40251=CARTESIAN_POINT('Ctrl Pts',(53.9507309817837,23.2159895990335,8.61420412118304));
#40252=CARTESIAN_POINT('Ctrl Pts',(54.0249034856629,23.2496083690804,8.60998184475211));
#40253=CARTESIAN_POINT('Ctrl Pts',(54.100476958074,23.2794316280696,8.60575956832118));
#40254=CARTESIAN_POINT('Ctrl Pts',(54.1768070779025,23.3095534798213,8.60149501813393));
#40255=CARTESIAN_POINT('Ctrl Pts',(54.2545659161888,23.3358032384644,8.59723046794667));
#40256=CARTESIAN_POINT('Ctrl Pts',(54.3333231470371,23.3580695968787,8.59296591775942));
#40257=CARTESIAN_POINT('Ctrl Pts',(54.4120803778855,23.380335955293,8.58870136757217));
#40258=CARTESIAN_POINT('Ctrl Pts',(54.4918355175178,23.3986188684309,8.58443681738492));
#40259=CARTESIAN_POINT('Ctrl Pts',(54.57215080854,23.4128604019642,8.58017226719767));
#40260=CARTESIAN_POINT('Ctrl Pts',(54.6518415404474,23.4269911884721,8.57594087960817));
#40261=CARTESIAN_POINT('Ctrl Pts',(54.7323823939831,23.4371962311709,8.57170949201866));
#40262=CARTESIAN_POINT('Ctrl Pts',(54.8133524211428,23.4433814543183,8.56747810442916));
#40263=CARTESIAN_POINT('Ctrl Pts',(54.8942063794495,23.4495578110768,8.56325278244593));
#40264=CARTESIAN_POINT('Ctrl Pts',(54.9754878298991,23.4517257576195,8.55902746046269));
#40265=CARTESIAN_POINT('Ctrl Pts',(55.0567666096346,23.449842403509,8.55480213847945));
#40266=CARTESIAN_POINT('Ctrl Pts',(55.1382501244665,23.4479543053719,8.55056617322983));
#40267=CARTESIAN_POINT('Ctrl Pts',(55.2197304893137,23.4419943955299,8.54633020798022));
#40268=CARTESIAN_POINT('Ctrl Pts',(55.3007700875323,23.4319719579892,8.5420942427306));
#40269=CARTESIAN_POINT('Ctrl Pts',(55.3814607014307,23.4219926805039,8.537876519001));
#40270=CARTESIAN_POINT('Ctrl Pts',(55.461713871787,23.4079858414377,8.53365879527139));
#40271=CARTESIAN_POINT('Ctrl Pts',(55.5411004392141,23.390012670402,8.52944107154179));
#40272=CARTESIAN_POINT('Ctrl Pts',(55.6204608084765,23.3720454306481,8.52522473969276));
#40273=CARTESIAN_POINT('Ctrl Pts',(55.6989546896901,23.3501145608329,8.52100840784372));
#40274=CARTESIAN_POINT('Ctrl Pts',(55.7761630923624,23.3243323996482,8.51679207599469));
#40275=CARTESIAN_POINT('Ctrl Pts',(55.8533696631064,23.2985508501984,8.5125758441868));
#40276=CARTESIAN_POINT('Ctrl Pts',(55.9292903753601,23.2689183393628,8.50835961237891));
#40277=CARTESIAN_POINT('Ctrl Pts',(56.0035227578039,23.2355966372693,8.50414338057102));
#40278=CARTESIAN_POINT('Ctrl Pts',(56.0783561418065,23.2020051554079,8.49989301323083));
#40279=CARTESIAN_POINT('Ctrl Pts',(56.1514732890126,23.1646646543371,8.49564264589063));
#40280=CARTESIAN_POINT('Ctrl Pts',(56.2224854615699,23.1237889599135,8.49139227855044));
#40281=CARTESIAN_POINT('Ctrl Pts',(56.2930297199746,23.0831826040444,8.48716991777532));
#40282=CARTESIAN_POINT('Ctrl Pts',(56.3614962992116,23.0390878089128,8.48294755700019));
#40283=CARTESIAN_POINT('Ctrl Pts',(56.4275332754918,22.9917577657345,8.47872519622507));
#40284=CARTESIAN_POINT('Ctrl Pts',(56.494227278364,22.9439568182429,8.47446082560234));
#40285=CARTESIAN_POINT('Ctrl Pts',(56.5584426838162,22.8928561899661,8.47019645497961));
#40286=CARTESIAN_POINT('Ctrl Pts',(56.6198526878366,22.8387570583708,8.46593208435688));
#40287=CARTESIAN_POINT('Ctrl Pts',(56.6812626918571,22.7846579267755,8.46166771373415));
#40288=CARTESIAN_POINT('Ctrl Pts',(56.7398669943921,22.7275606737917,8.45740334311141));
#40289=CARTESIAN_POINT('Ctrl Pts',(56.7953795976417,22.6678016519874,8.45313897248868));
#40290=CARTESIAN_POINT('Ctrl Pts',(56.8504512593943,22.6085173013567,8.4489084741374));
#40291=CARTESIAN_POINT('Ctrl Pts',(56.9026868253623,22.5463909028656,8.44467797578611));
#40292=CARTESIAN_POINT('Ctrl Pts',(56.9517790360638,22.4817249557127,8.44044747743483));
#40293=CARTESIAN_POINT('Ctrl Pts',(57.0008008247607,22.4171517708446,8.43622304766694));
#40294=CARTESIAN_POINT('Ctrl Pts',(57.0466879346531,22.3500466397073,8.43199861789905));
#40295=CARTESIAN_POINT('Ctrl Pts',(57.0891711073709,22.280747568464,8.42777418813116));
#40296=CARTESIAN_POINT('Ctrl Pts',(57.1317725266013,22.2112556120624,8.42353800019985));
#40297=CARTESIAN_POINT('Ctrl Pts',(57.1709507150789,22.139557834909,8.41930181226854));
#40298=CARTESIAN_POINT('Ctrl Pts',(57.2064760286778,22.0660271032531,8.41506562433723));
#40299=CARTESIAN_POINT('Ctrl Pts',(57.2418390103262,21.9928323682677,8.410848793551));
#40300=CARTESIAN_POINT('Ctrl Pts',(57.2735822177393,21.9178218121813,8.40663196276477));
#40301=CARTESIAN_POINT('Ctrl Pts',(57.3015244230522,21.8413890777127,8.40241513197854));
#40302=CARTESIAN_POINT('Ctrl Pts',(57.3294574165103,21.7649815412284,8.39819969137725));
#40303=CARTESIAN_POINT('Ctrl Pts',(57.3535917367447,21.6871531939148,8.39398425077595));
#40304=CARTESIAN_POINT('Ctrl Pts',(57.3737946118408,21.608316850659,8.38976881017466));
#40305=CARTESIAN_POINT('Ctrl Pts',(57.3939970213169,21.5294823243612,8.38555346672753));
#40306=CARTESIAN_POINT('Ctrl Pts',(57.4102680514289,21.4496402991265,8.3813381232804));
#40307=CARTESIAN_POINT('Ctrl Pts',(57.4225254210937,21.3692165139245,8.37712277983327));
#40308=CARTESIAN_POINT('Ctrl Pts',(57.4348877091442,21.2881043319507,8.37287135466214));
#40309=CARTESIAN_POINT('Ctrl Pts',(57.4431672060169,21.2064008553631,8.36861992949101));
#40310=CARTESIAN_POINT('Ctrl Pts',(57.4473327865741,21.1245491138444,8.36436850431988));
#40311=CARTESIAN_POINT('Ctrl Pts',(57.4514690349426,21.0432737363395,8.36014701581754));
#40312=CARTESIAN_POINT('Ctrl Pts',(57.4515491806293,20.9618526451025,8.35592552731521));
#40313=CARTESIAN_POINT('Ctrl Pts',(57.4475951901096,20.8807186714009,8.35170403881287));
#40314=CARTESIAN_POINT('Ctrl Pts',(57.4435991400281,20.7987216558253,8.34743764530734));
#40315=CARTESIAN_POINT('Ctrl Pts',(57.4354826687089,20.7170183872165,8.34317125180181));
#40316=CARTESIAN_POINT('Ctrl Pts',(57.4233218554622,20.6360474827134,8.33890485829629));
#40317=CARTESIAN_POINT('Ctrl Pts',(57.4111610422155,20.5550765782103,8.33463846479076));
#40318=CARTESIAN_POINT('Ctrl Pts',(57.3949560460808,20.4748384987183,8.33037207128523));
#40319=CARTESIAN_POINT('Ctrl Pts',(57.3748347618231,20.395756585442,8.3261056777797));
#40320=CARTESIAN_POINT('Ctrl Pts',(57.3548751534193,20.3173101005858,8.32187356502907));
#40321=CARTESIAN_POINT('Ctrl Pts',(57.3309870960226,20.2397068125228,8.31764145227843));
#40322=CARTESIAN_POINT('Ctrl Pts',(57.3032583570211,20.1633691430432,8.31340933952779));
#40323=CARTESIAN_POINT('Ctrl Pts',(57.2755693942215,20.0871409780941,8.30918329763998));
#40324=CARTESIAN_POINT('Ctrl Pts',(57.2440508492727,20.0121752590847,8.30495725575217));
#40325=CARTESIAN_POINT('Ctrl Pts',(57.2088409242349,19.9388817118601,8.30073121386437));
#40326=CARTESIAN_POINT('Ctrl Pts',(57.1735498261391,19.8654191934901,8.29649542924796));
#40327=CARTESIAN_POINT('Ctrl Pts',(57.1345504327932,19.7936370202747,8.29225964463156));
#40328=CARTESIAN_POINT('Ctrl Pts',(57.0920314325559,19.7239299646186,8.28802386001516));
#40329=CARTESIAN_POINT('Ctrl Pts',(57.0496866806833,19.6545085774965,8.28380543419222));
#40330=CARTESIAN_POINT('Ctrl Pts',(57.0038513476989,19.5871457373076,8.27958700836927));
#40331=CARTESIAN_POINT('Ctrl Pts',(56.9547580837715,19.5222073609839,8.27536858254633));
#40332=CARTESIAN_POINT('Ctrl Pts',(56.9056811137512,19.4572905375126,8.27115155680627));
#40333=CARTESIAN_POINT('Ctrl Pts',(56.8533486401505,19.394796950326,8.26693453106621));
#40334=CARTESIAN_POINT('Ctrl Pts',(56.7980356953539,19.3350621968875,8.26271750532615));
#40335=CARTESIAN_POINT('Ctrl Pts',(56.7427241819707,19.2753289892919,8.25850058871618));
#40336=CARTESIAN_POINT('Ctrl Pts',(56.6844326672896,19.2183548137282,8.25428367210622));
#40337=CARTESIAN_POINT('Ctrl Pts',(56.6234744229128,19.164439854391,8.25006675549625));
#40338=CARTESIAN_POINT('Ctrl Pts',(56.5620447160188,19.1101079066268,8.24581722446079));
#40339=CARTESIAN_POINT('Ctrl Pts',(56.497907197533,19.0588830315937,8.24156769342533));
#40340=CARTESIAN_POINT('Ctrl Pts',(56.4314165356043,19.0110311838547,8.23731816238987));
#40341=CARTESIAN_POINT('Ctrl Pts',(56.3653407351787,18.9634779026947,8.23309514585707));
#40342=CARTESIAN_POINT('Ctrl Pts',(56.2969414985436,18.9192558818546,8.22887212932427));
#40343=CARTESIAN_POINT('Ctrl Pts',(56.2265945774173,18.8785816082982,8.22464911279147));
#40344=CARTESIAN_POINT('Ctrl Pts',(56.1555851392443,18.8375242703638,8.22038632450468));
#40345=CARTESIAN_POINT('Ctrl Pts',(56.0825915681277,18.800082076633,8.21612353621788));
#40346=CARTESIAN_POINT('Ctrl Pts',(56.0080223597124,18.7664286059497,8.21186074793109));
#40347=CARTESIAN_POINT('Ctrl Pts',(55.9334531512972,18.7327751352665,8.2075979596443));
#40348=CARTESIAN_POINT('Ctrl Pts',(55.8573087757509,18.7029105036105,8.20333517135751));
#40349=CARTESIAN_POINT('Ctrl Pts',(55.7800129604173,18.6769567305836,8.19907238307072));
#40350=CARTESIAN_POINT('Ctrl Pts',(55.7032737514635,18.6511898504121,8.19484029107901));
#40351=CARTESIAN_POINT('Ctrl Pts',(55.6251131108804,18.6291814369582,8.19060819908731));
#40352=CARTESIAN_POINT('Ctrl Pts',(55.5459336251255,18.611086705852,8.1863761070956));
#40353=CARTESIAN_POINT('Ctrl Pts',(55.4668674168221,18.5930178618174,8.18215006970996));
#40354=CARTESIAN_POINT('Ctrl Pts',(55.3867857075107,18.5788516824413,8.17792403232432));
#40355=CARTESIAN_POINT('Ctrl Pts',(55.3061077488199,18.568694117123,8.17369799493868));
#40356=CARTESIAN_POINT('Ctrl Pts',(55.225243648512,18.5585131160898,8.16946220716464));
#40357=CARTESIAN_POINT('Ctrl Pts',(55.1437809937648,18.5523593893563,8.1652264193906));
#40358=CARTESIAN_POINT('Ctrl Pts',(55.0621538300848,18.5502883534167,8.16099063161656));
#40359=CARTESIAN_POINT('Ctrl Pts',(54.980860580322,18.5482257895064,8.15677217126668));
#40360=CARTESIAN_POINT('Ctrl Pts',(54.8994046318173,18.550212601245,8.1525537109168));
#40361=CARTESIAN_POINT('Ctrl Pts',(54.8182196120141,18.5562516208612,8.14833525056691));
#40362=CARTESIAN_POINT('Ctrl Pts',(54.7370612582481,18.5622886569005,8.14411817581281));
#40363=CARTESIAN_POINT('Ctrl Pts',(54.6561741195106,18.572375223175,8.13990110105871));
#40364=CARTESIAN_POINT('Ctrl Pts',(54.5759893141387,18.5864621013385,8.1356840263046));
#40365=CARTESIAN_POINT('Ctrl Pts',(54.4958063114778,18.6005486628014,8.13146704635857));
#40366=CARTESIAN_POINT('Ctrl Pts',(54.4163260682756,18.6186352758291,8.12725006641254));
#40367=CARTESIAN_POINT('Ctrl Pts',(54.3379706678704,18.6406213925273,8.12303308646651));
#40368=CARTESIAN_POINT('Ctrl Pts',(54.2590110176211,18.6627770585802,8.11878358662445));
#40369=CARTESIAN_POINT('Ctrl Pts',(54.1811940994258,18.6888925188956,8.11453408678238));
#40370=CARTESIAN_POINT('Ctrl Pts',(54.1049356366204,18.7188138972438,8.11028458694032));
#40371=CARTESIAN_POINT('Ctrl Pts',(54.0291506767195,18.748549488218,8.106061473029));
#40372=CARTESIAN_POINT('Ctrl Pts',(53.9549052765364,18.782043620346,8.10183835911767));
#40373=CARTESIAN_POINT('Ctrl Pts',(53.8825850493592,18.8190978751708,8.09761524520635));
#40374=CARTESIAN_POINT('Ctrl Pts',(53.8095870391957,18.8564994013535,8.09335255239891));
#40375=CARTESIAN_POINT('Ctrl Pts',(53.7385508952453,18.8975278882631,8.08908985959148));
#40376=CARTESIAN_POINT('Ctrl Pts',(53.6698438676303,18.9419341814414,8.08482716678404));
#40377=CARTESIAN_POINT('Ctrl Pts',(53.6011368400152,18.9863404746197,8.08056447397661));
#40378=CARTESIAN_POINT('Ctrl Pts',(53.5347592808768,19.0341242418496,8.07630178116917));
#40379=CARTESIAN_POINT('Ctrl Pts',(53.471043371659,19.0849955930463,8.07203908836174));
#40380=CARTESIAN_POINT('Ctrl Pts',(53.4086618184736,19.1348015824648,8.06786566603528));
#40381=CARTESIAN_POINT('Ctrl Pts',(53.3485836087252,19.1877652519427,8.06369224370881));
#40382=CARTESIAN_POINT('Ctrl Pts',(53.2911525345021,19.2436428069264,8.05951882138235));
#40383=CARTESIAN_POINT('Ctrl Pts',(53.2328446520373,19.3003734523563,8.05528168283359));
#40384=CARTESIAN_POINT('Ctrl Pts',(53.1772658553803,19.3601074698068,8.05104454428482));
#40385=CARTESIAN_POINT('Ctrl Pts',(53.1247437317707,19.4225450312396,8.04680740573606));
#40386=CARTESIAN_POINT('Ctrl Pts',(53.0731462051794,19.4838834447485,8.04264485757701));
#40387=CARTESIAN_POINT('Ctrl Pts',(53.0244989369235,19.5478306134058,8.03848230941795));
#40388=CARTESIAN_POINT('Ctrl Pts',(52.9790762828846,19.6140643667182,8.0343197612589));
#40389=CARTESIAN_POINT('Ctrl Pts',(52.933681050335,19.680258134957,8.03015972601488));
#40390=CARTESIAN_POINT('Ctrl Pts',(52.8915068401811,19.7487353555256,8.02599969077085));
#40391=CARTESIAN_POINT('Ctrl Pts',(52.8527866955541,19.8191421443668,8.02183965552683));
#40392=CARTESIAN_POINT('Ctrl Pts',(52.8140773001988,19.8895293872661,8.0176807751687));
#40393=CARTESIAN_POINT('Ctrl Pts',(52.778820296948,19.9618447155347,8.01352189481057));
#40394=CARTESIAN_POINT('Ctrl Pts',(52.7472036377794,20.0357081352798,8.00936301445244));
#40395=CARTESIAN_POINT('Ctrl Pts',(52.7145550085216,20.111982462498,8.00506838793241));
#40396=CARTESIAN_POINT('Ctrl Pts',(52.6857887308971,20.1899072118895,8.00077376141238));
#40397=CARTESIAN_POINT('Ctrl Pts',(52.6610579011033,20.2690416509753,7.99647913489234));
#40398=CARTESIAN_POINT('Ctrl Pts',(52.6370856091149,20.3457488984041,7.9923162320792));
#40399=CARTESIAN_POINT('Ctrl Pts',(52.6169048605921,20.4235922076928,7.98815332926606));
#40400=CARTESIAN_POINT('Ctrl Pts',(52.6006037241118,20.5021568909248,7.98399042645292));
#40401=CARTESIAN_POINT('Ctrl Pts',(52.5835288801176,20.5844505218781,7.97962993807944));
#40402=CARTESIAN_POINT('Ctrl Pts',(52.5707111745886,20.6675351198086,7.97526944970597));
#40403=CARTESIAN_POINT('Ctrl Pts',(52.5621909383103,20.7509272621433,7.97090896133249));
#40404=CARTESIAN_POINT('Ctrl Pts',(52.553670702032,20.8343194044779,7.96654847295901));
#40405=CARTESIAN_POINT('Ctrl Pts',(52.5494478931564,20.9180184923135,7.96218798458554));
#40406=CARTESIAN_POINT('Ctrl Pts',(52.5495004857877,21.0015429988506,7.95782749621206));
#40407=CARTESIAN_POINT('Origin',(55.,21.,6.22095488139522));
#40408=CARTESIAN_POINT('',(53.00502528211,20.9993602050363,26.6209548194543));
#40409=CARTESIAN_POINT('Ctrl Pts',(55.164372889159,22.9868942741083,26.4105573801159));
#40410=CARTESIAN_POINT('Ctrl Pts',(54.6931881369,23.0214673262749,26.440680792387));
#40411=CARTESIAN_POINT('Ctrl Pts',(53.5591487190497,22.7217611434947,26.5108130101989));
#40412=CARTESIAN_POINT('Ctrl Pts',(53.0048473617801,21.6235590597841,26.5809452280106));
#40413=CARTESIAN_POINT('Ctrl Pts',(53.0021727671314,20.9993715498994,26.6209540335512));
#40414=CARTESIAN_POINT('',(56.9679107878093,20.6738793264392,26.9999963704729));
#40415=CARTESIAN_POINT('Ctrl Pts',(53.0052501028907,20.9993593108917,26.6209548813952));
#40416=CARTESIAN_POINT('Ctrl Pts',(53.0052617870906,20.9629812046206,26.6232902248096));
#40417=CARTESIAN_POINT('Ctrl Pts',(53.0062685406323,20.9266205928135,26.625625568224));
#40418=CARTESIAN_POINT('Ctrl Pts',(53.008267908903,20.8903148150642,26.6279609116383));
#40419=CARTESIAN_POINT('Ctrl Pts',(53.0120769023975,20.8211487323132,26.6324099708752));
#40420=CARTESIAN_POINT('Ctrl Pts',(53.019500686615,20.7520426805399,26.6368590301121));
#40421=CARTESIAN_POINT('Ctrl Pts',(53.0305342119411,20.6834055083144,26.6413080893491));
#40422=CARTESIAN_POINT('Ctrl Pts',(53.0415511297092,20.614871648112,26.645750451904));
#40423=CARTESIAN_POINT('Ctrl Pts',(53.056166928241,20.5468057473348,26.650192814459));
#40424=CARTESIAN_POINT('Ctrl Pts',(53.0743246331812,20.4796136587808,26.654635177014));
#40425=CARTESIAN_POINT('Ctrl Pts',(53.0924609870389,20.4125005793219,26.6590723159325));
#40426=CARTESIAN_POINT('Ctrl Pts',(53.1141308487093,20.3462597429776,26.663509454851));
#40427=CARTESIAN_POINT('Ctrl Pts',(53.1392261439035,20.2812871095023,26.6679465937695));
#40428=CARTESIAN_POINT('Ctrl Pts',(53.1643056781146,20.216355281786,26.6723809459636));
#40429=CARTESIAN_POINT('Ctrl Pts',(53.1928062020456,20.1526905337474,26.6768152981578));
#40430=CARTESIAN_POINT('Ctrl Pts',(53.2245701952823,20.0906724621897,26.6812496503519));
#40431=CARTESIAN_POINT('Ctrl Pts',(53.256325095761,20.0286721439198,26.6856827331687));
#40432=CARTESIAN_POINT('Ctrl Pts',(53.2913413875328,19.9683180030185,26.6901158159856));
#40433=CARTESIAN_POINT('Ctrl Pts',(53.3294146902202,19.9099668421338,26.6945488988024));
#40434=CARTESIAN_POINT('Ctrl Pts',(53.3674901066498,19.8516124417268,26.6989822277338));
#40435=CARTESIAN_POINT('Ctrl Pts',(53.4086226007211,19.7952616517772,26.7034155566652));
#40436=CARTESIAN_POINT('Ctrl Pts',(53.4525643718967,19.7412424620378,26.7078488855967));
#40437=CARTESIAN_POINT('Ctrl Pts',(53.496553397549,19.6871651806814,26.7122869820791));
#40438=CARTESIAN_POINT('Ctrl Pts',(53.5433574196601,19.6354248854047,26.7167250785616));
#40439=CARTESIAN_POINT('Ctrl Pts',(53.5926888493941,19.5863158457844,26.7211631750441));
#40440=CARTESIAN_POINT('Ctrl Pts',(53.642049523441,19.5371776936869,26.7256039024879));
#40441=CARTESIAN_POINT('Ctrl Pts',(53.6939402212742,19.4906742290622,26.7300446299317));
#40442=CARTESIAN_POINT('Ctrl Pts',(53.7480391520969,19.4470603367105,26.7344853573755));
#40443=CARTESIAN_POINT('Ctrl Pts',(53.8022335380262,19.4033694896264,26.7389339202812));
#40444=CARTESIAN_POINT('Ctrl Pts',(53.8586435366931,19.3625786792873,26.7433824831869));
#40445=CARTESIAN_POINT('Ctrl Pts',(53.9169178693461,19.3248998057554,26.7478310460926));
#40446=CARTESIAN_POINT('Ctrl Pts',(53.9481960140994,19.3046760604662,26.7502187661775));
#40447=CARTESIAN_POINT('Ctrl Pts',(53.9800108165797,19.2853480491996,26.7526064862624));
#40448=CARTESIAN_POINT('Ctrl Pts',(54.0123053327775,19.2669429302991,26.7549942063473));
#40449=CARTESIAN_POINT('Ctrl Pts',(54.0726664323319,19.2325422534952,26.7594570510256));
#40450=CARTESIAN_POINT('Ctrl Pts',(54.1349441451365,19.2012319967431,26.7639198957039));
#40451=CARTESIAN_POINT('Ctrl Pts',(54.1987898135051,19.1732296806777,26.7683827403822));
#40452=CARTESIAN_POINT('Ctrl Pts',(54.2625395383733,19.1452694448394,26.772838878561));
#40453=CARTESIAN_POINT('Ctrl Pts',(54.3278520988388,19.1206074765866,26.7772950167399));
#40454=CARTESIAN_POINT('Ctrl Pts',(54.394353341559,19.0994159614426,26.7817511549187));
#40455=CARTESIAN_POINT('Ctrl Pts',(54.4607754279747,19.0782496705192,26.7862019889647));
#40456=CARTESIAN_POINT('Ctrl Pts',(54.5283829238227,19.0605457743145,26.7906528230106));
#40457=CARTESIAN_POINT('Ctrl Pts',(54.5967824054927,19.0464281088274,26.7951036570565));
#40458=CARTESIAN_POINT('Ctrl Pts',(54.665138176523,19.0323194652243,26.7995516468002));
#40459=CARTESIAN_POINT('Ctrl Pts',(54.7342844529156,19.021792603608,26.8039996365438));
#40460=CARTESIAN_POINT('Ctrl Pts',(54.803814824814,19.014920923606,26.8084476262874));
#40461=CARTESIAN_POINT('Ctrl Pts',(54.8733241422802,19.0080513244115,26.8128942691391));
#40462=CARTESIAN_POINT('Ctrl Pts',(54.9432168394968,19.0048347572317,26.8173409119907));
#40463=CARTESIAN_POINT('Ctrl Pts',(55.0130802840506,19.0052928864946,26.8217875548424));
#40464=CARTESIAN_POINT('Ctrl Pts',(55.0829460631963,19.0057510310665,26.8262343462853));
#40465=CARTESIAN_POINT('Ctrl Pts',(55.1527821003074,19.0098841103251,26.8306811377282));
#40466=CARTESIAN_POINT('Ctrl Pts',(55.2221764182933,19.0176616833511,26.8351279291711));
#40467=CARTESIAN_POINT('Ctrl Pts',(55.2916414064181,19.0254471769416,26.8395792491602));
#40468=CARTESIAN_POINT('Ctrl Pts',(55.3606632921501,19.0368845181813,26.8440305691492));
#40469=CARTESIAN_POINT('Ctrl Pts',(55.428836833603,19.0518915500811,26.8484818891382));
#40470=CARTESIAN_POINT('Ctrl Pts',(55.4970488881697,19.0669070598671,26.8529357238007));
#40471=CARTESIAN_POINT('Ctrl Pts',(55.5644111741879,19.0854961455472,26.8573895584631));
#40472=CARTESIAN_POINT('Ctrl Pts',(55.6305328944282,19.1075265308216,26.8618433931256));
#40473=CARTESIAN_POINT('Ctrl Pts',(55.6967661972704,19.1295940931039,26.8663047437822));
#40474=CARTESIAN_POINT('Ctrl Pts',(55.761754301392,19.1551143698067,26.8707660944387));
#40475=CARTESIAN_POINT('Ctrl Pts',(55.8251264421699,19.1839069635803,26.8752274450953));
#40476=CARTESIAN_POINT('Ctrl Pts',(55.857324023637,19.1985356611799,26.8774941304156));
#40477=CARTESIAN_POINT('Ctrl Pts',(55.8891048586513,19.2140083261596,26.8797608157359));
#40478=CARTESIAN_POINT('Ctrl Pts',(55.9204230327013,19.2302969166064,26.8820275010562));
#40479=CARTESIAN_POINT('Ctrl Pts',(55.9813755574437,19.2619983405348,26.8864390032354));
#40480=CARTESIAN_POINT('Ctrl Pts',(56.0408183362336,19.29692023275,26.8908505054146));
#40481=CARTESIAN_POINT('Ctrl Pts',(56.0983850698236,19.3348940571578,26.8952620075938));
#40482=CARTESIAN_POINT('Ctrl Pts',(56.1558553852743,19.3728042794595,26.8996661209773));
#40483=CARTESIAN_POINT('Ctrl Pts',(56.21145548081,19.4137560119269,26.9040702343608));
#40484=CARTESIAN_POINT('Ctrl Pts',(56.2648431341122,19.4575346329369,26.9084743477443));
#40485=CARTESIAN_POINT('Ctrl Pts',(56.3181807935537,19.5012722582831,26.912874336979));
#40486=CARTESIAN_POINT('Ctrl Pts',(56.3693097326684,19.5478312101843,26.9172743262136));
#40487=CARTESIAN_POINT('Ctrl Pts',(56.4179174630016,19.5969541594747,26.9216743154482));
#40488=CARTESIAN_POINT('Ctrl Pts',(56.4664969640683,19.6460485802819,26.9260717493595));
#40489=CARTESIAN_POINT('Ctrl Pts',(56.5125578089706,19.6977036912373,26.9304691832708));
#40490=CARTESIAN_POINT('Ctrl Pts',(56.5558227743796,19.7516238318432,26.9348666171821));
#40491=CARTESIAN_POINT('Ctrl Pts',(56.5990779999195,19.8055318338721,26.9392630611369));
#40492=CARTESIAN_POINT('Ctrl Pts',(56.6395382830616,19.8617034634036,26.9436595050918));
#40493=CARTESIAN_POINT('Ctrl Pts',(56.6769665367608,19.9198098329069,26.9480559490466));
#40494=CARTESIAN_POINT('Ctrl Pts',(56.7144248914634,19.9779629334183,26.9524559287629));
#40495=CARTESIAN_POINT('Ctrl Pts',(56.7488460713666,20.0380534629174,26.9568559084791));
#40496=CARTESIAN_POINT('Ctrl Pts',(56.7800368660057,20.0997243099135,26.9612558881954));
#40497=CARTESIAN_POINT('Ctrl Pts',(56.8112391841974,20.1614179414284,26.9656574935001));
#40498=CARTESIAN_POINT('Ctrl Pts',(56.8392085358469,20.2246925961809,26.9700590988049));
#40499=CARTESIAN_POINT('Ctrl Pts',(56.8637994165494,20.2891699940422,26.9744607041097));
#40500=CARTESIAN_POINT('Ctrl Pts',(56.8884337482449,20.3537613205989,26.9788700868553));
#40501=CARTESIAN_POINT('Ctrl Pts',(56.9096775275357,20.4195591594962,26.983279469601));
#40502=CARTESIAN_POINT('Ctrl Pts',(56.9274350256771,20.4861694984793,26.9876888523466));
#40503=CARTESIAN_POINT('Ctrl Pts',(56.9439566677346,20.5481440046422,26.9917913583887));
#40504=CARTESIAN_POINT('Ctrl Pts',(56.9574608765223,20.6108214008906,26.9958938644308));
#40505=CARTESIAN_POINT('Ctrl Pts',(56.9679107878093,20.6738793264392,26.9999963704729));
#40506=CARTESIAN_POINT('',(55.3268144232807,19.0322043055145,27.));
#40507=CARTESIAN_POINT('Origin',(55.,21.,27.));
#40508=CARTESIAN_POINT('',(53.0052507551611,21.0017357173056,26.7790451185624));
#40509=CARTESIAN_POINT('Ctrl Pts',(53.0052507551605,21.0017357166396,26.7790451186048));
#40510=CARTESIAN_POINT('Ctrl Pts',(53.0051914603514,20.9335919464819,26.7833890309428));
#40511=CARTESIAN_POINT('Ctrl Pts',(53.0086282717321,20.8653545643158,26.7877329432809));
#40512=CARTESIAN_POINT('Ctrl Pts',(53.015563321049,20.7974200658161,26.7920768556189));
#40513=CARTESIAN_POINT('Ctrl Pts',(53.022494410904,20.7295243534951,26.7964182878656));
#40514=CARTESIAN_POINT('Ctrl Pts',(53.0329197306783,20.6619316909371,26.8007597201123));
#40515=CARTESIAN_POINT('Ctrl Pts',(53.0467893877479,20.5950359686516,26.8051011523591));
#40516=CARTESIAN_POINT('Ctrl Pts',(53.0606562797094,20.5281535829544,26.8094417190812));
#40517=CARTESIAN_POINT('Ctrl Pts',(53.0779660429013,20.4619683635367,26.8137822858032));
#40518=CARTESIAN_POINT('Ctrl Pts',(53.0986176020176,20.3968644106482,26.8181228525253));
#40519=CARTESIAN_POINT('Ctrl Pts',(53.1192727174921,20.3317492463555,26.8224641667266));
#40520=CARTESIAN_POINT('Ctrl Pts',(53.1432706110484,20.2677162048407,26.8268054809278));
#40521=CARTESIAN_POINT('Ctrl Pts',(53.1704608818346,20.2051326037618,26.8311467951291));
#40522=CARTESIAN_POINT('Ctrl Pts',(53.1976845321881,20.1424721732336,26.8354934388539));
#40523=CARTESIAN_POINT('Ctrl Pts',(53.228108166454,20.0812652000635,26.8398400825788));
#40524=CARTESIAN_POINT('Ctrl Pts',(53.2615344726562,20.0218562617195,26.8441867263036));
#40525=CARTESIAN_POINT('Ctrl Pts',(53.294985710061,19.9624030128775,26.8485366119977));
#40526=CARTESIAN_POINT('Ctrl Pts',(53.3314437909819,19.904750892004,26.8528864976917));
#40527=CARTESIAN_POINT('Ctrl Pts',(53.3706686726283,19.8492146211629,26.8572363833858));
#40528=CARTESIAN_POINT('Ctrl Pts',(53.4099641060601,19.7935784600763,26.8615940929964));
#40529=CARTESIAN_POINT('Ctrl Pts',(53.4520359378455,19.7400661293411,26.865951802607));
#40530=CARTESIAN_POINT('Ctrl Pts',(53.4966054601351,19.6889575064078,26.8703095122176));
#40531=CARTESIAN_POINT('Ctrl Pts',(53.5056644870474,19.678569367455,26.8711952432421));
#40532=CARTESIAN_POINT('Ctrl Pts',(53.5148265887909,19.6682804025268,26.8720809742666));
#40533=CARTESIAN_POINT('Ctrl Pts',(53.5240892587333,19.6580927579323,26.8729667052911));
#40534=CARTESIAN_POINT('Ctrl Pts',(53.5719500758757,19.6054525366921,26.877543335017));
#40535=CARTESIAN_POINT('Ctrl Pts',(53.6227079385196,19.5552903614172,26.882119964743));
#40536=CARTESIAN_POINT('Ctrl Pts',(53.6760827272401,19.5079307598546,26.8866965944689));
#40537=CARTESIAN_POINT('Ctrl Pts',(53.731140940504,19.4590774509155,26.8914175696994));
#40538=CARTESIAN_POINT('Ctrl Pts',(53.7889836636027,19.4132068877389,26.8961385449298));
#40539=CARTESIAN_POINT('Ctrl Pts',(53.8492595652905,19.3706369298328,26.9008595201603));
#40540=CARTESIAN_POINT('Ctrl Pts',(53.9074978653635,19.3295060315267,26.9054209048001));
#40541=CARTESIAN_POINT('Ctrl Pts',(53.9680070691629,19.2914564589498,26.9099822894399));
#40542=CARTESIAN_POINT('Ctrl Pts',(54.0304355126644,19.2567351700336,26.9145436740797));
#40543=CARTESIAN_POINT('Ctrl Pts',(54.0928049320613,19.22204670899,26.9191007460756));
#40544=CARTESIAN_POINT('Ctrl Pts',(54.1570895870498,19.1906804991255,26.9236578180716));
#40545=CARTESIAN_POINT('Ctrl Pts',(54.2229100653257,19.1628394746436,26.9282148900675));
#40546=CARTESIAN_POINT('Ctrl Pts',(54.2886860851091,19.135017255403,26.9327688839857));
#40547=CARTESIAN_POINT('Ctrl Pts',(54.3559954457556,19.1107156654368,26.9373228779038));
#40548=CARTESIAN_POINT('Ctrl Pts',(54.424436672141,19.0900904686023,26.941876871822));
#40549=CARTESIAN_POINT('Ctrl Pts',(54.4928501330044,19.0694736390836,26.9464290182569));
#40550=CARTESIAN_POINT('Ctrl Pts',(54.5623941089844,19.0525303673778,26.9509811646918));
#40551=CARTESIAN_POINT('Ctrl Pts',(54.6326511025143,19.03936684971,26.9555333111268));
#40552=CARTESIAN_POINT('Ctrl Pts',(54.7029182418346,19.0262014311028,26.9600861149357));
#40553=CARTESIAN_POINT('Ctrl Pts',(54.7738981562464,19.016816947517,26.9646389187447));
#40554=CARTESIAN_POINT('Ctrl Pts',(54.8451632610788,19.0112684578405,26.9691917225537));
#40555=CARTESIAN_POINT('Ctrl Pts',(54.916433668482,19.0057195553215,26.9737448651198));
#40556=CARTESIAN_POINT('Ctrl Pts',(54.9879888521485,19.0040072420144,26.9782980076859));
#40557=CARTESIAN_POINT('Ctrl Pts',(55.0593980229147,19.0061345488289,26.9828511502521));
#40558=CARTESIAN_POINT('Ctrl Pts',(55.1308564692507,19.0082633235817,26.9874074346933));
#40559=CARTESIAN_POINT('Ctrl Pts',(55.2021682448793,19.0142369843338,26.9919637191345));
#40560=CARTESIAN_POINT('Ctrl Pts',(55.2729054141899,19.0240065290073,26.9965200035757));
#40561=CARTESIAN_POINT('Ctrl Pts',(55.2909146129457,19.0264937881596,26.9976800023838));
#40562=CARTESIAN_POINT('Ctrl Pts',(55.3088866054585,19.0292268269792,26.9988400011919));
#40563=CARTESIAN_POINT('Ctrl Pts',(55.3268144232807,19.0322043055145,27.));
#40564=CARTESIAN_POINT('Ctrl Pts',(55.1644483516311,22.987959834138,26.5685072087751));
#40565=CARTESIAN_POINT('Ctrl Pts',(55.0947777969994,22.993723133612,26.5729580929947));
#40566=CARTESIAN_POINT('Ctrl Pts',(55.0248300995882,22.9958174035433,26.5774089772144));
#40567=CARTESIAN_POINT('Ctrl Pts',(54.9550189243188,22.9942427799369,26.581859861434));
#40568=CARTESIAN_POINT('Ctrl Pts',(54.8851738235987,22.9926673911262,26.5863129086061));
#40569=CARTESIAN_POINT('Ctrl Pts',(54.8154658639627,22.9874195932691,26.5907659557782));
#40570=CARTESIAN_POINT('Ctrl Pts',(54.7463045870801,22.9785515408913,26.5952190029503));
#40571=CARTESIAN_POINT('Ctrl Pts',(54.6770210913026,22.9696678172649,26.5996799193598));
#40572=CARTESIAN_POINT('Ctrl Pts',(54.6082866887087,22.957151146555,26.6041408357693));
#40573=CARTESIAN_POINT('Ctrl Pts',(54.5405011077653,22.9411049251741,26.6086017521787));
#40574=CARTESIAN_POINT('Ctrl Pts',(54.4883383903836,22.9287569523561,26.6120345400769));
#40575=CARTESIAN_POINT('Ctrl Pts',(54.4367373486985,22.9143199493095,26.615467327975));
#40576=CARTESIAN_POINT('Ctrl Pts',(54.3858726940112,22.8978606941867,26.6189001158731));
#40577=CARTESIAN_POINT('Ctrl Pts',(54.3198027005323,22.8764811549897,26.6233590918642));
#40578=CARTESIAN_POINT('Ctrl Pts',(54.2547231915789,22.8516062006253,26.6278180678553));
#40579=CARTESIAN_POINT('Ctrl Pts',(54.1910294196137,22.8233469671375,26.6322770438463));
#40580=CARTESIAN_POINT('Ctrl Pts',(54.1274296624664,22.7951294455252,26.6367294381921));
#40581=CARTESIAN_POINT('Ctrl Pts',(54.0652120250352,22.7635377567045,26.6411818325378));
#40582=CARTESIAN_POINT('Ctrl Pts',(54.004755403991,22.7287324132482,26.6456342268836));
#40583=CARTESIAN_POINT('Ctrl Pts',(53.9443680865756,22.6939669684259,26.6500815172874));
#40584=CARTESIAN_POINT('Ctrl Pts',(53.885738197043,22.6559954285362,26.6545288076912));
#40585=CARTESIAN_POINT('Ctrl Pts',(53.829221865242,22.6150251148736,26.658976098095));
#40586=CARTESIAN_POINT('Ctrl Pts',(53.7727400807916,22.5740798455786,26.6634206699553));
#40587=CARTESIAN_POINT('Ctrl Pts',(53.7183696852096,22.530139725215,26.6678652418157));
#40588=CARTESIAN_POINT('Ctrl Pts',(53.6664382407234,22.4834556268035,26.6723098136761));
#40589=CARTESIAN_POINT('Ctrl Pts',(53.6145210174744,22.4367843126626,26.6767531684067));
#40590=CARTESIAN_POINT('Ctrl Pts',(53.5650417821479,22.3873708385779,26.6811965231372));
#40591=CARTESIAN_POINT('Ctrl Pts',(53.5182940102893,22.3355054932705,26.6856398778677));
#40592=CARTESIAN_POINT('Ctrl Pts',(53.4715432663981,22.2836368505759,26.6900835150886));
#40593=CARTESIAN_POINT('Ctrl Pts',(53.4275246558122,22.2293163913823,26.6945271523096));
#40594=CARTESIAN_POINT('Ctrl Pts',(53.3864926604128,22.1728689729028,26.6989707895305));
#40595=CARTESIAN_POINT('Ctrl Pts',(53.3454167996535,22.116361209166,26.7034191772331));
#40596=CARTESIAN_POINT('Ctrl Pts',(53.3073342142657,22.0577223434595,26.7078675649358));
#40597=CARTESIAN_POINT('Ctrl Pts',(53.2724565978743,21.9973070521518,26.7123159526384));
#40598=CARTESIAN_POINT('Ctrl Pts',(53.2375583093029,21.9368559523257,26.7167669769281));
#40599=CARTESIAN_POINT('Ctrl Pts',(53.2058689924398,21.8746267662481,26.7212180012178));
#40600=CARTESIAN_POINT('Ctrl Pts',(53.1775535288098,21.8109971776439,26.7256690255075));
#40601=CARTESIAN_POINT('Ctrl Pts',(53.1491888716133,21.7472570428577,26.7301277827364));
#40602=CARTESIAN_POINT('Ctrl Pts',(53.1242099429465,21.6821121046642,26.7345865399653));
#40603=CARTESIAN_POINT('Ctrl Pts',(53.1027325404657,21.6159575874134,26.7390452971942));
#40604=CARTESIAN_POINT('Ctrl Pts',(53.0916727483929,21.5818913074653,26.7413413349902));
#40605=CARTESIAN_POINT('Ctrl Pts',(53.0815406442462,21.5475575227488,26.7436373727861));
#40606=CARTESIAN_POINT('Ctrl Pts',(53.0723467389698,21.5130111770124,26.7459334105821));
#40607=CARTESIAN_POINT('Ctrl Pts',(53.0497110534813,21.4279569815042,26.751586328233));
#40608=CARTESIAN_POINT('Ctrl Pts',(53.0326903197989,21.3413349535193,26.757239245884));
#40609=CARTESIAN_POINT('Ctrl Pts',(53.0214612094316,21.2537948319336,26.762892163535));
#40610=CARTESIAN_POINT('Ctrl Pts',(53.0107656520835,21.1704141935701,26.7682764818774));
#40611=CARTESIAN_POINT('Ctrl Pts',(53.0053242516375,21.0862005322065,26.7736608002199));
#40612=CARTESIAN_POINT('Ctrl Pts',(53.0052507551611,21.0017357173056,26.7790451185623));
#40613=CARTESIAN_POINT('Origin',(55.,21.,27.));
#40614=CARTESIAN_POINT('',(52.6675979604224,21.7515656829407,27.));
#40615=CARTESIAN_POINT('',(52.5495,21.,27.));
#40616=CARTESIAN_POINT('Origin',(55.,21.,27.));
#40617=CARTESIAN_POINT('Ctrl Pts',(52.6675979604224,21.7515656829407,27.));
#40618=CARTESIAN_POINT('Ctrl Pts',(52.6581593165275,21.7103708819833,27.));
#40619=CARTESIAN_POINT('Ctrl Pts',(52.6498806799008,21.6689484082415,27.));
#40620=CARTESIAN_POINT('Ctrl Pts',(52.64279639573,21.6273284827364,27.));
#40621=CARTESIAN_POINT('Ctrl Pts',(52.6284952714311,21.5433098700432,27.));
#40622=CARTESIAN_POINT('Ctrl Pts',(52.6190581654961,21.4584860602675,27.));
#40623=CARTESIAN_POINT('Ctrl Pts',(52.6143486107364,21.3732318851031,27.));
#40624=CARTESIAN_POINT('Ctrl Pts',(52.611968832347,21.3301522196133,27.));
#40625=CARTESIAN_POINT('Ctrl Pts',(52.6107970049565,21.2869627536936,27.));
#40626=CARTESIAN_POINT('Ctrl Pts',(52.6108203452642,21.2437130426133,27.));
#40627=CARTESIAN_POINT('Ctrl Pts',(52.6108328628886,21.2205178196194,27.));
#40628=CARTESIAN_POINT('Ctrl Pts',(52.6111891968172,21.1973052874763,27.));
#40629=CARTESIAN_POINT('Ctrl Pts',(52.6118877304625,21.1740832515286,27.));
#40630=CARTESIAN_POINT('Ctrl Pts',(52.6123409031142,21.1590179906353,27.));
#40631=CARTESIAN_POINT('Ctrl Pts',(52.6129380504501,21.143952266255,27.));
#40632=CARTESIAN_POINT('Ctrl Pts',(52.6136780136879,21.128896584471,27.));
#40633=CARTESIAN_POINT('Ctrl Pts',(52.6178472913967,21.0440662641901,27.));
#40634=CARTESIAN_POINT('Ctrl Pts',(52.6265485898479,20.9594741460822,27.));
#40635=CARTESIAN_POINT('Ctrl Pts',(52.6396478697088,20.8754925672425,27.));
#40636=CARTESIAN_POINT('Ctrl Pts',(52.6498009700148,20.8103994168655,27.));
#40637=CARTESIAN_POINT('Ctrl Pts',(52.662597356556,20.7456730539443,27.));
#40638=CARTESIAN_POINT('Ctrl Pts',(52.6779943778682,20.6814954047314,27.));
#40639=CARTESIAN_POINT('Ctrl Pts',(52.6852626539292,20.6511998779559,27.));
#40640=CARTESIAN_POINT('Ctrl Pts',(52.6931106853611,20.6210267642035,27.));
#40641=CARTESIAN_POINT('Ctrl Pts',(52.701535187251,20.59099607487,27.));
#40642=CARTESIAN_POINT('Ctrl Pts',(52.7053028526838,20.5775655371831,27.));
#40643=CARTESIAN_POINT('Ctrl Pts',(52.7091858289863,20.5641634945839,27.));
#40644=CARTESIAN_POINT('Ctrl Pts',(52.7131838689533,20.5507917806399,27.));
#40645=CARTESIAN_POINT('Ctrl Pts',(52.7171931368534,20.5373825141172,27.));
#40646=CARTESIAN_POINT('Ctrl Pts',(52.7213152423352,20.524013371772,27.));
#40647=CARTESIAN_POINT('Ctrl Pts',(52.7255492350363,20.5106867826928,27.));
#40648=CARTESIAN_POINT('Ctrl Pts',(52.7506876133668,20.4315631606711,27.));
#40649=CARTESIAN_POINT('Ctrl Pts',(52.7797692419591,20.3539281551878,27.));
#40650=CARTESIAN_POINT('Ctrl Pts',(52.8126749747748,20.2781287589336,27.));
#40651=CARTESIAN_POINT('Ctrl Pts',(52.8452016800973,20.2032024644977,27.));
#40652=CARTESIAN_POINT('Ctrl Pts',(52.8814654159397,20.1300689107429,27.));
#40653=CARTESIAN_POINT('Ctrl Pts',(52.921392257506,20.0590922664586,27.));
#40654=CARTESIAN_POINT('Ctrl Pts',(52.9601079309623,19.9902686762288,27.));
#40655=CARTESIAN_POINT('Ctrl Pts',(53.0022683739052,19.9234725558841,27.));
#40656=CARTESIAN_POINT('Ctrl Pts',(53.0478373127237,19.8590733051686,27.));
#40657=CARTESIAN_POINT('Ctrl Pts',(53.0676678011867,19.8310483251832,27.));
#40658=CARTESIAN_POINT('Ctrl Pts',(53.0881441430014,19.8034777959598,27.));
#40659=CARTESIAN_POINT('Ctrl Pts',(53.1092649010727,19.7763948758004,27.));
#40660=CARTESIAN_POINT('Ctrl Pts',(53.117566242513,19.7657501552517,27.0000000000001));
#40661=CARTESIAN_POINT('Ctrl Pts',(53.1259678411942,19.7551800576066,27.));
#40662=CARTESIAN_POINT('Ctrl Pts',(53.1344588227666,19.7446996216994,27.));
#40663=CARTESIAN_POINT('Ctrl Pts',(53.1836538089366,19.6839781497331,27.));
#40664=CARTESIAN_POINT('Ctrl Pts',(53.235927021935,19.6261583160513,27.));
#40665=CARTESIAN_POINT('Ctrl Pts',(53.2912060581531,19.5715630117008,27.));
#40666=CARTESIAN_POINT('Ctrl Pts',(53.3132549044344,19.5497868818031,27.));
#40667=CARTESIAN_POINT('Ctrl Pts',(53.3357823343684,19.5285241787662,27.));
#40668=CARTESIAN_POINT('Ctrl Pts',(53.3587851728467,19.5077972530674,27.));
#40669=CARTESIAN_POINT('Ctrl Pts',(53.4176110563557,19.4547916330086,27.));
#40670=CARTESIAN_POINT('Ctrl Pts',(53.4795448432047,19.4052865427495,27.));
#40671=CARTESIAN_POINT('Ctrl Pts',(53.54422871254,19.3593757920684,27.));
#40672=CARTESIAN_POINT('Ctrl Pts',(53.6075401759656,19.3144391356428,27.));
#40673=CARTESIAN_POINT('Ctrl Pts',(53.6734872861446,19.2729459319649,27.));
#40674=CARTESIAN_POINT('Ctrl Pts',(53.7417440169708,19.2350307492206,27.));
#40675=CARTESIAN_POINT('Ctrl Pts',(53.7574393241756,19.2263123351727,27.));
#40676=CARTESIAN_POINT('Ctrl Pts',(53.7732620003945,19.2177807068876,27.));
#40677=CARTESIAN_POINT('Ctrl Pts',(53.789178685159,19.2094527983754,27.));
#40678=CARTESIAN_POINT('Ctrl Pts',(53.8580381744901,19.1734242198219,27.));
#40679=CARTESIAN_POINT('Ctrl Pts',(53.9287388139424,19.1411552595462,27.));
#40680=CARTESIAN_POINT('Ctrl Pts',(54.0009311833521,19.1127073066594,27.));
#40681=CARTESIAN_POINT('Ctrl Pts',(54.0728786828169,19.084355846639,27.));
#40682=CARTESIAN_POINT('Ctrl Pts',(54.1463088594656,19.0597994309732,27.));
#40683=CARTESIAN_POINT('Ctrl Pts',(54.2208852843057,19.0391489920333,27.));
#40684=CARTESIAN_POINT('Ctrl Pts',(54.294838653122,19.0186710792021,27.));
#40685=CARTESIAN_POINT('Ctrl Pts',(54.3699201671869,19.0020341080845,27.));
#40686=CARTESIAN_POINT('Ctrl Pts',(54.4457960554792,18.9893965582189,27.));
#40687=CARTESIAN_POINT('Ctrl Pts',(54.4747700166878,18.9845707843424,27.));
#40688=CARTESIAN_POINT('Ctrl Pts',(54.5038596760197,18.9803287228457,27.));
#40689=CARTESIAN_POINT('Ctrl Pts',(54.5330457778138,18.9766811777813,27.));
#40690=CARTESIAN_POINT('Ctrl Pts',(54.5453585497017,18.9751423840552,27.));
#40691=CARTESIAN_POINT('Ctrl Pts',(54.557688672971,18.9737094744325,27.));
#40692=CARTESIAN_POINT('Ctrl Pts',(54.5700200506845,18.9723846440183,27.));
#40693=CARTESIAN_POINT('Ctrl Pts',(54.6447271119773,18.9643584372752,27.));
#40694=CARTESIAN_POINT('Ctrl Pts',(54.7196133883747,18.9602774590628,27.));
#40695=CARTESIAN_POINT('Ctrl Pts',(54.7943672308826,18.9602361966031,27.));
#40696=CARTESIAN_POINT('Ctrl Pts',(54.8670339703188,18.9601960861779,27.));
#40697=CARTESIAN_POINT('Ctrl Pts',(54.9395763781891,18.9639734317702,27.));
#40698=CARTESIAN_POINT('Ctrl Pts',(55.0116978667239,18.9717019486186,27.));
#40699=CARTESIAN_POINT('Ctrl Pts',(55.0828084700766,18.9793221393173,27.));
#40700=CARTESIAN_POINT('Ctrl Pts',(55.1535105815583,18.9907835686913,27.));
#40701=CARTESIAN_POINT('Ctrl Pts',(55.2234985969135,19.0062592360608,27.));
#40702=CARTESIAN_POINT('Ctrl Pts',(55.2581256631984,19.0139159320977,27.));
#40703=CARTESIAN_POINT('Ctrl Pts',(55.2925775330345,19.0225559423173,27.));
#40704=CARTESIAN_POINT('Ctrl Pts',(55.3268144232807,19.0322043055145,27.));
#40705=CARTESIAN_POINT('Ctrl Pts',(56.9711550749276,20.6733990999081,27.));
#40706=CARTESIAN_POINT('Ctrl Pts',(56.9843403290936,20.7192200369488,27.));
#40707=CARTESIAN_POINT('Ctrl Pts',(56.9957486638496,20.7654588673864,27.));
#40708=CARTESIAN_POINT('Ctrl Pts',(57.0053244209566,20.8120332025565,27.));
#40709=CARTESIAN_POINT('Ctrl Pts',(57.0197547200195,20.8822189411518,27.));
#40710=CARTESIAN_POINT('Ctrl Pts',(57.0300261579609,20.9531657218038,27.));
#40711=CARTESIAN_POINT('Ctrl Pts',(57.0363241708791,21.0245726301505,27.));
#40712=CARTESIAN_POINT('Ctrl Pts',(57.0398083736352,21.0640765419541,27.));
#40713=CARTESIAN_POINT('Ctrl Pts',(57.0420756345699,21.1037217059478,27.));
#40714=CARTESIAN_POINT('Ctrl Pts',(57.04315111989,21.1434595266447,27.));
#40715=CARTESIAN_POINT('Ctrl Pts',(57.0435947853274,21.1598524027472,27.));
#40716=CARTESIAN_POINT('Ctrl Pts',(57.0438355858288,21.1762610615222,27.));
#40717=CARTESIAN_POINT('Ctrl Pts',(57.0438750725979,21.1926821425536,27.));
#40718=CARTESIAN_POINT('Ctrl Pts',(57.0439138408907,21.2088044359754,27.));
#40719=CARTESIAN_POINT('Ctrl Pts',(57.043758487098,21.2249300434683,27.));
#40720=CARTESIAN_POINT('Ctrl Pts',(57.0434112528463,21.2410498327371,27.));
#40721=CARTESIAN_POINT('Ctrl Pts',(57.041793511242,21.3161508736899,27.));
#40722=CARTESIAN_POINT('Ctrl Pts',(57.0360151353344,21.391163881607,27.));
#40723=CARTESIAN_POINT('Ctrl Pts',(57.0262731102432,21.4657603741072,27.));
#40724=CARTESIAN_POINT('Ctrl Pts',(57.0183309920558,21.5265746457048,27.));
#40725=CARTESIAN_POINT('Ctrl Pts',(57.0077535297998,21.5871127615298,27.));
#40726=CARTESIAN_POINT('Ctrl Pts',(56.994622590053,21.6472025604645,27.));
#40727=CARTESIAN_POINT('Ctrl Pts',(56.9891693654016,21.6721576039852,27.));
#40728=CARTESIAN_POINT('Ctrl Pts',(56.9832754808879,21.6970353561712,27.));
#40729=CARTESIAN_POINT('Ctrl Pts',(56.9769457075483,21.7218235275587,27.));
#40730=CARTESIAN_POINT('Ctrl Pts',(56.9732935075575,21.7361259921903,27.));
#40731=CARTESIAN_POINT('Ctrl Pts',(56.96949577252,21.7503997627616,27.));
#40732=CARTESIAN_POINT('Ctrl Pts',(56.9655583005791,21.7646255421325,27.));
#40733=CARTESIAN_POINT('Ctrl Pts',(56.9447075274203,21.8399577611619,27.));
#40734=CARTESIAN_POINT('Ctrl Pts',(56.9199157678371,21.9140520889315,27.));
#40735=CARTESIAN_POINT('Ctrl Pts',(56.8913863602786,21.9865684507146,27.));
#40736=CARTESIAN_POINT('Ctrl Pts',(56.8624995036878,22.0599933803778,27.));
#40737=CARTESIAN_POINT('Ctrl Pts',(56.8297806422816,22.1318015814284,27.));
#40738=CARTESIAN_POINT('Ctrl Pts',(56.7933873856968,22.2016439364836,27.));
#40739=CARTESIAN_POINT('Ctrl Pts',(56.7571899251842,22.2711105389935,27.));
#40740=CARTESIAN_POINT('Ctrl Pts',(56.7173572333979,22.3386334422686,27.));
#40741=CARTESIAN_POINT('Ctrl Pts',(56.6739948998583,22.4038573683784,27.));
#40742=CARTESIAN_POINT('Ctrl Pts',(56.6612704605766,22.4229969722639,27.));
#40743=CARTESIAN_POINT('Ctrl Pts',(56.6482417732324,22.4419384773733,27.));
#40744=CARTESIAN_POINT('Ctrl Pts',(56.6349107419457,22.4606725079749,27.));
#40745=CARTESIAN_POINT('Ctrl Pts',(56.6273072000305,22.4713577268342,27.));
#40746=CARTESIAN_POINT('Ctrl Pts',(56.6196039727324,22.4819772302926,27.));
#40747=CARTESIAN_POINT('Ctrl Pts',(56.611805607223,22.4925235206514,27.));
#40748=CARTESIAN_POINT('Ctrl Pts',(56.5635925023516,22.5577255687555,27.));
#40749=CARTESIAN_POINT('Ctrl Pts',(56.5119013821899,22.6199239206814,27.));
#40750=CARTESIAN_POINT('Ctrl Pts',(56.4569110326642,22.6787619007156,27.));
#40751=CARTESIAN_POINT('Ctrl Pts',(56.4321646798555,22.7052397359183,27.));
#40752=CARTESIAN_POINT('Ctrl Pts',(56.4067494980637,22.7310369552658,27.));
#40753=CARTESIAN_POINT('Ctrl Pts',(56.3806784609636,22.7561201322126,27.));
#40754=CARTESIAN_POINT('Ctrl Pts',(56.3241596085106,22.8104974234369,27.));
#40755=CARTESIAN_POINT('Ctrl Pts',(56.2645614152419,22.861521301469,27.));
#40756=CARTESIAN_POINT('Ctrl Pts',(56.2022367668188,22.9091785543743,27.));
#40757=CARTESIAN_POINT('Ctrl Pts',(56.1399121183956,22.9568358072795,27.));
#40758=CARTESIAN_POINT('Ctrl Pts',(56.0748602656315,23.0011267676018,27.));
#40759=CARTESIAN_POINT('Ctrl Pts',(56.0073956790906,23.0420027201548,27.));
#40760=CARTESIAN_POINT('Ctrl Pts',(55.995921828827,23.0489545830954,27.));
#40761=CARTESIAN_POINT('Ctrl Pts',(55.9843764396863,23.055808551695,27.));
#40762=CARTESIAN_POINT('Ctrl Pts',(55.9727662874617,23.0625611887514,27.));
#40763=CARTESIAN_POINT('Ctrl Pts',(55.9033022392179,23.1029625114202,27.));
#40764=CARTESIAN_POINT('Ctrl Pts',(55.8317582221578,23.1396040058116,27.));
#40765=CARTESIAN_POINT('Ctrl Pts',(55.7585161957843,23.1724925894664,27.));
#40766=CARTESIAN_POINT('Ctrl Pts',(55.6828327620042,23.206477462174,27.));
#40767=CARTESIAN_POINT('Ctrl Pts',(55.6053356039688,23.2364555943728,27.));
#40768=CARTESIAN_POINT('Ctrl Pts',(55.526403821075,23.2623966359773,27.));
#40769=CARTESIAN_POINT('Ctrl Pts',(55.4474720381812,23.2883376775817,27.));
#40770=CARTESIAN_POINT('Ctrl Pts',(55.3671047185148,23.3102419887007,27.));
#40771=CARTESIAN_POINT('Ctrl Pts',(55.2856513531316,23.3280353685059,27.));
#40772=CARTESIAN_POINT('Ctrl Pts',(55.2359251484301,23.3388979920741,27.));
#40773=CARTESIAN_POINT('Ctrl Pts',(55.1857936600202,23.3482276198764,27.));
#40774=CARTESIAN_POINT('Ctrl Pts',(55.1353332201589,23.355998440921,27.));
#40775=CARTESIAN_POINT('Ctrl Pts',(55.1216156589962,23.3581109217724,27.));
#40776=CARTESIAN_POINT('Ctrl Pts',(55.1078812076943,23.3601069820185,27.));
#40777=CARTESIAN_POINT('Ctrl Pts',(55.0941380647184,23.3619855976698,27.));
#40778=CARTESIAN_POINT('Ctrl Pts',(55.0090469708069,23.3736171044575,27.));
#40779=CARTESIAN_POINT('Ctrl Pts',(54.9235470750792,23.3807620486719,27.));
#40780=CARTESIAN_POINT('Ctrl Pts',(54.8380287552821,23.3833903704909,27.));
#40781=CARTESIAN_POINT('Ctrl Pts',(54.7524215968147,23.3860214226794,27.));
#40782=CARTESIAN_POINT('Ctrl Pts',(54.666795005057,23.3841268154452,27.));
#40783=CARTESIAN_POINT('Ctrl Pts',(54.5815186695155,23.377629130775,27.));
#40784=CARTESIAN_POINT('Ctrl Pts',(54.4980822478155,23.3712716395111,27.));
#40785=CARTESIAN_POINT('Ctrl Pts',(54.4149801838723,23.3605077155167,27.));
#40786=CARTESIAN_POINT('Ctrl Pts',(54.3325520387133,23.3452161635882,27.));
#40787=CARTESIAN_POINT('Ctrl Pts',(54.2891983220411,23.3371734542866,27.));
#40788=CARTESIAN_POINT('Ctrl Pts',(54.2460310044596,23.3278774277892,27.));
#40789=CARTESIAN_POINT('Ctrl Pts',(54.203100055607,23.3173046257725,27.));
#40790=CARTESIAN_POINT('Origin',(55.,21.,27.));
#40791=CARTESIAN_POINT('Ctrl Pts',(54.1264352462825,22.7892995080061,7.43479847215643));
#40792=CARTESIAN_POINT('Ctrl Pts',(53.5313636363274,22.4987759919214,7.47714290372609));
#40793=CARTESIAN_POINT('Ctrl Pts',(52.6642537907918,21.2821184890334,7.56183176686541));
#40794=CARTESIAN_POINT('Ctrl Pts',(53.4976472728867,19.1863830377497,7.68886506157439));
#40795=CARTESIAN_POINT('Ctrl Pts',(55.7087280813971,18.7562692203022,7.81589835628338));
#40796=CARTESIAN_POINT('Ctrl Pts',(57.2698128240574,20.3778916813317,7.94293165099235));
#40797=CARTESIAN_POINT('Ctrl Pts',(56.7533256858317,22.5703705433843,8.06996494570134));
#40798=CARTESIAN_POINT('Ctrl Pts',(54.6312789516365,23.3244325802832,8.19699824041032));
#40799=CARTESIAN_POINT('Ctrl Pts',(52.8469659787634,21.9506800446467,8.32403153511931));
#40800=CARTESIAN_POINT('Ctrl Pts',(53.0338008043911,19.706355415659,8.45106482982828));
#40801=CARTESIAN_POINT('Ctrl Pts',(55.0208406626359,18.6465226847945,8.57809812453727));
#40802=CARTESIAN_POINT('Ctrl Pts',(56.9887798196956,19.7413863016522,8.70513141924624));
#40803=CARTESIAN_POINT('Ctrl Pts',(57.1358892072027,21.9886045058084,8.83216471395522));
#40804=CARTESIAN_POINT('Ctrl Pts',(55.3274665165508,23.3306879153509,8.95919800866422));
#40805=CARTESIAN_POINT('Ctrl Pts',(53.2192324453698,22.5389012348763,9.08623130337319));
#40806=CARTESIAN_POINT('Ctrl Pts',(52.7413900137877,20.3381607386649,9.21326459808217));
#40807=CARTESIAN_POINT('Ctrl Pts',(54.3314329386002,18.7433729270463,9.34029789279115));
#40808=CARTESIAN_POINT('Ctrl Pts',(56.5335863102332,19.2146535088455,9.46733118750014));
#40809=CARTESIAN_POINT('Ctrl Pts',(57.3316552158584,21.3205197731518,9.59436448220912));
#40810=CARTESIAN_POINT('Ctrl Pts',(55.9949623455254,23.1329319227209,9.72139777691809));
#40811=CARTESIAN_POINT('Ctrl Pts',(53.7473254531283,22.9925248642322,9.84843107162709));
#40812=CARTESIAN_POINT('Ctrl Pts',(52.6465826422626,21.0278490069435,9.97546436633607));
#40813=CARTESIAN_POINT('Ctrl Pts',(53.7005259934764,19.0376758430876,10.102497661045));
#40814=CARTESIAN_POINT('Ctrl Pts',(55.9442109855123,18.8441209605304,10.229530955754));
#40815=CARTESIAN_POINT('Ctrl Pts',(57.32341763991,20.6243947780001,10.356564250463));
#40816=CARTESIAN_POINT('Ctrl Pts',(56.5754045744307,22.7485563288281,10.483597545172));
#40817=CARTESIAN_POINT('Ctrl Pts',(54.3850198856334,23.2718160732959,10.610630839881));
#40818=CARTESIAN_POINT('Ctrl Pts',(52.7576841304891,21.7151002393188,10.7376641345899));
#40819=CARTESIAN_POINT('Ctrl Pts',(53.183314854842,19.5036698579907,10.864697429299));
#40820=CARTESIAN_POINT('Ctrl Pts',(55.2722231561246,18.6622140037448,10.9917307240079));
#40821=CARTESIAN_POINT('Ctrl Pts',(57.1118958247853,19.9611329073913,11.1187640187169));
#40822=CARTESIAN_POINT('Ctrl Pts',(57.0180089111301,22.2111931495074,11.2457973134259));
#40823=CARTESIAN_POINT('Ctrl Pts',(55.0765211729318,23.3523378415888,11.3728306081349));
#40824=CARTESIAN_POINT('Ctrl Pts',(53.0649739907733,22.3397847418404,11.4998639028438));
#40825=CARTESIAN_POINT('Ctrl Pts',(52.8250521123875,20.1005832461981,11.6268971975528));
#40826=CARTESIAN_POINT('Ctrl Pts',(54.5764175312761,18.6848484492269,11.7539304922618));
#40827=CARTESIAN_POINT('Ctrl Pts',(56.7155965589988,19.3887653002727,11.8809637869708));
#40828=CARTESIAN_POINT('Ctrl Pts',(57.2840503042245,21.5678582733624,12.0079970816798));
#40829=CARTESIAN_POINT('Ctrl Pts',(55.7613273444601,23.2270450119906,12.1350303763887));
#40830=CARTESIAN_POINT('Ctrl Pts',(53.5415663183002,22.8472466015499,12.2620636710978));
#40831=CARTESIAN_POINT('Ctrl Pts',(52.6570834755071,20.7761898793339,12.3890969658067));
#40832=CARTESIAN_POINT('Ctrl Pts',(53.9176726780599,18.9100439289218,12.5161302605157));
#40833=CARTESIAN_POINT('Ctrl Pts',(56.1691935070438,18.957370480498,12.6431635552247));
#40834=CARTESIAN_POINT('Ctrl Pts',(57.3502518243073,20.8748394103778,12.7701968499337));
#40835=CARTESIAN_POINT('Ctrl Pts',(56.3795222160764,22.9068999098553,12.8972301446426));
#40836=CARTESIAN_POINT('Ctrl Pts',(54.1457623160259,23.1930861337697,13.0242634393516));
#40837=CARTESIAN_POINT('Ctrl Pts',(52.6941051314662,21.4713784743956,13.1512967340606));
#40838=CARTESIAN_POINT('Ctrl Pts',(53.3536245809391,19.3180972708369,13.2783300287696));
#40839=CARTESIAN_POINT('Ctrl Pts',(55.5204934603439,18.7046927507208,13.4053633234786));
#40840=CARTESIAN_POINT('Ctrl Pts',(57.2108212594767,20.1927713028513,13.5323966181875));
#40841=CARTESIAN_POINT('Ctrl Pts',(56.8770176687869,22.4199131952045,13.6594299128965));
#40842=CARTESIAN_POINT('Ctrl Pts',(54.8246986773802,23.3470445792831,13.7864632076055));
#40843=CARTESIAN_POINT('Ctrl Pts',(52.9328779208585,22.1253244513384,13.9134965023145));
#40844=CARTESIAN_POINT('Ctrl Pts',(52.9336238605588,19.8733064031411,14.0405297970235));
#40845=CARTESIAN_POINT('Ctrl Pts',(54.8262535466699,18.6528398050389,14.1675630917325));
#40846=CARTESIAN_POINT('Ctrl Pts',(56.8779578972515,19.5813305716253,14.2945963864414));
#40847=CARTESIAN_POINT('Ctrl Pts',(57.2102860149976,21.8086931078973,14.4216296811504));
#40848=CARTESIAN_POINT('Ctrl Pts',(55.5189727893898,23.2956515534217,14.5486629758594));
#40849=CARTESIAN_POINT('Ctrl Pts',(53.3525107434218,22.6808116968638,14.6756962705684));
#40850=CARTESIAN_POINT('Ctrl Pts',(52.6944179083708,20.5270940583868,14.8027295652774));
#40851=CARTESIAN_POINT('Ctrl Pts',(54.1472153424787,18.8063484463683,14.9297628599863));
#40852=CARTESIAN_POINT('Ctrl Pts',(56.3807851645167,19.0940143913699,15.0567961546953));
#40853=CARTESIAN_POINT('Ctrl Pts',(57.350168394301,21.1267175176638,15.1838294494043));
#40854=CARTESIAN_POINT('Ctrl Pts',(56.1678400834611,23.0434036190425,15.3108627441133));
#40855=CARTESIAN_POINT('Ctrl Pts',(53.9162883964239,23.0892386103863,15.4378960388223));
#40856=CARTESIAN_POINT('Ctrl Pts',(52.6569357236264,21.222257975417,15.5649293335312));
#40857=CARTESIAN_POINT('Ctrl Pts',(53.5427903713442,19.1517876450454,15.6919626282402));
#40858=CARTESIAN_POINT('Ctrl Pts',(55.762802512921,18.7734598280885,15.8189959229492));
#40859=CARTESIAN_POINT('Ctrl Pts',(57.2844259882859,20.4336549506721,15.9460292176582));
#40860=CARTESIAN_POINT('Ctrl Pts',(56.7145287987417,22.6123708658803,16.0730625123672));
#40861=CARTESIAN_POINT('Ctrl Pts',(54.5748839213591,23.3148704349348,16.2000958070762));
#40862=CARTESIAN_POINT('Ctrl Pts',(52.8244567590706,21.8979757333586,16.3271291017851));
#40863=CARTESIAN_POINT('Ctrl Pts',(53.0658619735541,19.6589336684897,16.4541623964941));
#40864=CARTESIAN_POINT('Ctrl Pts',(55.078079493554,18.647713367053,16.5811956912031));
#40865=CARTESIAN_POINT('Ctrl Pts',(57.0188108392977,19.7901439730331,16.7082289859121));
#40866=CARTESIAN_POINT('Ctrl Pts',(57.1112071500763,22.040265918081,16.8352622806211));
#40867=CARTESIAN_POINT('Ctrl Pts',(55.2706743990552,23.3379658210827,16.9622955753301));
#40868=CARTESIAN_POINT('Ctrl Pts',(53.1823239896862,22.4951263265638,17.089328870039));
#40869=CARTESIAN_POINT('Ctrl Pts',(52.7581583502224,20.2834144655543,17.216362164748));
#40870=CARTESIAN_POINT('Ctrl Pts',(54.3865250151568,18.727777023744,17.343395459457));
#40871=CARTESIAN_POINT('Ctrl Pts',(56.576562583322,19.2524877019822,17.470428754166));
#40872=CARTESIAN_POINT('Ctrl Pts',(57.3231683049537,21.3771443194757,17.597462048875));
#40873=CARTESIAN_POINT('Ctrl Pts',(55.9427825885663,23.1565040694491,17.7244953435839));
#40874=CARTESIAN_POINT('Ctrl Pts',(53.6992263091515,22.9614628765416,17.8515286382929));
#40875=CARTESIAN_POINT('Ctrl Pts',(52.6466016111188,20.970591938755,17.9785619330019));
#40876=CARTESIAN_POINT('Ctrl Pts',(53.7486456956814,19.0066457374772,18.1055952277109));
#40877=CARTESIAN_POINT('Ctrl Pts',(55.9963751296602,18.8677276412595,18.2326285224199));
#40878=CARTESIAN_POINT('Ctrl Pts',(57.3318670105856,20.6810249918929,18.3596618171288));
#40879=CARTESIAN_POINT('Ctrl Pts',(56.5324032985223,22.7863619290425,18.4866951118378));
#40880=CARTESIAN_POINT('Ctrl Pts',(54.3299380524767,23.2561839014885,18.6137284065468));
#40881=CARTESIAN_POINT('Ctrl Pts',(52.7409522613139,21.6603424302529,18.7407617012558));
#40882=CARTESIAN_POINT('Ctrl Pts',(53.2202519180959,19.4599202696571,18.8677949959648));
#40883=CARTESIAN_POINT('Ctrl Pts',(55.3290111899943,18.6695278487583,18.9948282906738));
#40884=CARTESIAN_POINT('Ctrl Pts',(57.1365421855609,20.0128139485519,19.1218615853827));
#40885=CARTESIAN_POINT('Ctrl Pts',(56.9879484673196,22.2599244827116,19.2488948800917));
#40886=CARTESIAN_POINT('Ctrl Pts',(55.019275954014,23.353503186412,19.3759281748007));
#40887=CARTESIAN_POINT('Ctrl Pts',(53.0329552190706,22.2923171594749,19.5029614695097));
#40888=CARTESIAN_POINT('Ctrl Pts',(52.84757477688,20.0479419819511,19.6299947642187));
#40889=CARTESIAN_POINT('Ctrl Pts',(54.6328608640107,18.6752295455939,19.7570280589276));
#40890=CARTESIAN_POINT('Ctrl Pts',(56.7542835096275,19.4309754053223,19.8840613536367));
#40891=CARTESIAN_POINT('Ctrl Pts',(57.2695607903648,21.6232516583953,20.0110946483456));
#40892=CARTESIAN_POINT('Ctrl Pts',(55.7069273321875,23.2449059129194,20.1381279430546));
#40893=CARTESIAN_POINT('Ctrl Pts',(53.4970620829863,22.8112223575412,20.2651612377636));
#40894=CARTESIAN_POINT('Ctrl Pts',(52.6632211513288,20.7192627148797,20.3921945324726));
#40895=CARTESIAN_POINT('Ctrl Pts',(53.9688328770913,18.884333869561,20.5192278271815));
#40896=CARTESIAN_POINT('Ctrl Pts',(56.2185361854212,18.9864165337207,20.6462611218906));
#40897=CARTESIAN_POINT('Ctrl Pts',(57.3526009806992,20.9320482784099,20.7732944165995));
#40898=CARTESIAN_POINT('Ctrl Pts',(56.3327270654876,22.9398936516653,20.9003277113085));
#40899=CARTESIAN_POINT('Ctrl Pts',(54.0926664546051,23.1716571203244,21.0273610060175));
#40900=CARTESIAN_POINT('Ctrl Pts',(52.6833208110228,21.4151461745151,21.1543943007264));
#40901=CARTESIAN_POINT('Ctrl Pts',(53.3950254542771,19.2785455224038,21.2814275954354));
#40902=CARTESIAN_POINT('Ctrl Pts',(55.5761746959756,18.7180334072183,21.4084608901444));
#40903=CARTESIAN_POINT('Ctrl Pts',(57.2298035498787,20.2467902418298,21.5354941848534));
#40904=CARTESIAN_POINT('Ctrl Pts',(56.8419216578993,22.4651530353571,21.6625274795624));
#40905=CARTESIAN_POINT('Ctrl Pts',(54.7676567399891,23.3420856987698,21.7895607742714));
#40906=CARTESIAN_POINT('Ctrl Pts',(52.9061151635912,22.0747069845831,21.9165940689803));
#40907=CARTESIAN_POINT('Ctrl Pts',(52.9616430951332,19.823373492039,22.0436273636893));
#40908=CARTESIAN_POINT('Ctrl Pts',(54.883401585621,18.6493078422263,22.1706606583983));
#40909=CARTESIAN_POINT('Ctrl Pts',(56.911912491998,19.6274332679986,22.2976939531073));
#40910=CARTESIAN_POINT('Ctrl Pts',(57.1899598215212,21.8622208481452,22.4247272478162));
#40911=CARTESIAN_POINT('Ctrl Pts',(55.4629755827127,23.3075966763422,22.5517605425253));
#40912=CARTESIAN_POINT('Ctrl Pts',(53.3121111203556,22.6402377696025,22.6787938372342));
#40913=CARTESIAN_POINT('Ctrl Pts',(52.7066039993849,20.4711487967183,22.8058271319432));
#40914=CARTESIAN_POINT('Ctrl Pts',(54.2008300948515,18.7862528885265,22.9328604266522));
#40915=CARTESIAN_POINT('Ctrl Pts',(56.4267412525533,19.1281671524571,23.0598937213612));
#40916=CARTESIAN_POINT('Ctrl Pts',(57.3463904308638,21.183849821225,23.1869270160701));
#40917=CARTESIAN_POINT('Ctrl Pts',(56.1177870069067,23.071207623113,23.3139603107791));
#40918=CARTESIAN_POINT('Ctrl Pts',(53.8657866175656,23.0622581831875,23.4409936054881));
#40919=CARTESIAN_POINT('Ctrl Pts',(52.6522224656966,21.1651952176771,23.5680269001971));
#40920=CARTESIAN_POINT('Ctrl Pts',(53.5881808872158,19.1168867257354,23.6950601949061));
#40921=CARTESIAN_POINT('Ctrl Pts',(55.8167392291167,18.7926745043891,23.822093489615));
#40922=CARTESIAN_POINT('Ctrl Pts',(57.2975268021679,20.4893931046865,23.9491267843241));
#40923=CARTESIAN_POINT('Ctrl Pts',(56.6747991790829,22.6536010770382,24.076160079033));
#40924=CARTESIAN_POINT('Ctrl Pts',(54.5186985692507,23.3038441246632,24.203193373742));
#40925=CARTESIAN_POINT('Ctrl Pts',(52.8032565359452,21.8447881057192,24.330226668451));
#40926=CARTESIAN_POINT('Ctrl Pts',(53.0990568643523,19.6122810003745,24.45725996316));
#40927=CARTESIAN_POINT('Ctrl Pts',(55.1352777323281,18.6503087883512,24.5842932578689));
#40928=CARTESIAN_POINT('Ctrl Pts',(57.0476441652364,19.8396112597284,24.711326552578));
#40929=CARTESIAN_POINT('Ctrl Pts',(57.0852771298678,22.0913149235079,24.8383598472869));
#40930=CARTESIAN_POINT('Ctrl Pts',(55.2137212298849,23.3438584215582,24.9653931419959));
#40931=CARTESIAN_POINT('Ctrl Pts',(53.1464918908666,22.45046728724,25.0924264367049));
#40932=CARTESIAN_POINT('Ctrl Pts',(52.7762528735532,20.2290920967572,25.2194597314139));
#40933=CARTESIAN_POINT('Ctrl Pts',(54.4419810779207,18.7135256448128,25.3464930261228));
#40934=CARTESIAN_POINT('Ctrl Pts',(56.6186041564239,19.2913569527159,25.4735263208318));
#40935=CARTESIAN_POINT('Ctrl Pts',(57.3133095927893,21.4335438873502,25.6005596155408));
#40936=CARTESIAN_POINT('Ctrl Pts',(55.8900387814265,23.1788034744911,25.7275929102498));
#40937=CARTESIAN_POINT('Ctrl Pts',(53.6519088779192,22.9292330426812,25.8546262049588));
#40938=CARTESIAN_POINT('Ctrl Pts',(52.6479901933195,20.9133659611559,25.9816594996677));
#40939=CARTESIAN_POINT('Ctrl Pts',(53.7975513738378,18.9767685882894,26.1086927943768));
#40940=CARTESIAN_POINT('Ctrl Pts',(56.0478608304085,18.8926486501099,26.2357260890857));
#40941=CARTESIAN_POINT('Ctrl Pts',(57.3391098950668,20.7377415341185,26.3627593837947));
#40942=CARTESIAN_POINT('Ctrl Pts',(56.4881554930549,22.823310792186,26.4897926785037));
#40943=CARTESIAN_POINT('Ctrl Pts',(54.2759180399637,23.2388230435375,26.6168259732127));
#40944=CARTESIAN_POINT('Ctrl Pts',(52.7242447265499,21.6059770109423,26.7438592679217));
#40945=CARTESIAN_POINT('Ctrl Pts',(53.261008001841,19.4150988751331,26.8709101685003));
#40946=CARTESIAN_POINT('Ctrl Pts',(54.6735570889175,18.9270516578725,26.9556166375094));
#40947=CARTESIAN_POINT('Ctrl Pts',(55.3270406347534,19.0358837922465,26.9979786749487));
#40948=CARTESIAN_POINT('Ctrl Pts',(54.0587940262274,22.9278472244179,7.52381308588823));
#40949=CARTESIAN_POINT('Ctrl Pts',(53.4176452713942,22.6148281062624,7.56615751745789));
#40950=CARTESIAN_POINT('Ctrl Pts',(52.4833940174808,21.3039632792647,7.65084638059721));
#40951=CARTESIAN_POINT('Ctrl Pts',(53.3813182074311,19.0459523902024,7.77787967530619));
#40952=CARTESIAN_POINT('Ctrl Pts',(55.7636057901289,18.5825343176886,7.90491297001517));
#40953=CARTESIAN_POINT('Ctrl Pts',(57.4455672922436,20.3297210500167,8.03194626472416));
#40954=CARTESIAN_POINT('Ctrl Pts',(56.8890879038456,22.6919663140939,8.15897955943315));
#40955=CARTESIAN_POINT('Ctrl Pts',(54.6027284160695,23.504416325045,8.28601285414212));
#40956=CARTESIAN_POINT('Ctrl Pts',(52.6802538404854,22.0242923988863,8.4130461488511));
#40957=CARTESIAN_POINT('Ctrl Pts',(52.8815555221769,19.6061868847859,8.54007944356008));
#40958=CARTESIAN_POINT('Ctrl Pts',(55.0224543814147,18.4642899695951,8.66711273826906));
#40959=CARTESIAN_POINT('Ctrl Pts',(57.1427735480971,19.6439302564397,8.79414603297805));
#40960=CARTESIAN_POINT('Ctrl Pts',(57.3012738009179,22.0651533988816,8.92117932768702));
#40961=CARTESIAN_POINT('Ctrl Pts',(55.3528226617163,23.5111560185922,9.04821262239602));
#40962=CARTESIAN_POINT('Ctrl Pts',(53.0813453688628,22.6580602973593,9.17524591710498));
#40963=CARTESIAN_POINT('Ctrl Pts',(52.5665029954577,20.2869136903762,9.30227921181398));
#40964=CARTESIAN_POINT('Ctrl Pts',(54.2796649482718,18.5686394481893,9.42931250652295));
#40965=CARTESIAN_POINT('Ctrl Pts',(56.6523338314015,19.0764118795115,9.55634580123193));
#40966=CARTESIAN_POINT('Ctrl Pts',(57.5121982183976,21.3453380232191,9.68337909594093));
#40967=CARTESIAN_POINT('Ctrl Pts',(56.0720035341421,23.298087530171,9.81041239064989));
#40968=CARTESIAN_POINT('Ctrl Pts',(53.6503292839014,23.1468085761529,9.93744568535889));
#40969=CARTESIAN_POINT('Ctrl Pts',(52.4643545696455,21.0300053906563,10.0644789800679));
#40970=CARTESIAN_POINT('Ctrl Pts',(53.5999060830955,18.8857306100042,10.1915122747768));
#40971=CARTESIAN_POINT('Ctrl Pts',(56.0173224323485,18.6771885289045,10.3185455694858));
#40972=CARTESIAN_POINT('Ctrl Pts',(57.5033227965594,20.5953111921903,10.4455788641948));
#40973=CARTESIAN_POINT('Ctrl Pts',(56.6973901365099,22.8839492495173,10.5726121589038));
#40974=CARTESIAN_POINT('Ctrl Pts',(54.3374012001631,23.4477256555959,10.6996454536128));
#40975=CARTESIAN_POINT('Ctrl Pts',(52.5840587861548,21.770471352271,10.8266787483217));
#40976=CARTESIAN_POINT('Ctrl Pts',(53.0426466340244,19.3878071288916,10.9537120430307));
#40977=CARTESIAN_POINT('Ctrl Pts',(55.2933017382551,18.4811962871516,11.0807453377397));
#40978=CARTESIAN_POINT('Ctrl Pts',(57.2754225806551,19.8806921188636,11.2077786324487));
#40979=CARTESIAN_POINT('Ctrl Pts',(57.174265884926,22.3049773618469,11.3348119271577));
#40980=CARTESIAN_POINT('Ctrl Pts',(55.082446303811,23.5344823259097,11.4618452218667));
#40981=CARTESIAN_POINT('Ctrl Pts',(52.9151424876759,22.4435259632707,11.5888785165756));
#40982=CARTESIAN_POINT('Ctrl Pts',(52.6566431558126,20.0309402731888,11.7159118112846));
#40983=CARTESIAN_POINT('Ctrl Pts',(54.5436190067747,18.5055833462792,11.8429451059936));
#40984=CARTESIAN_POINT('Ctrl Pts',(56.8484373631626,19.2640053664261,11.9699784007026));
#40985=CARTESIAN_POINT('Ctrl Pts',(57.460907198447,21.6118282552844,12.0970116954116));
#40986=CARTESIAN_POINT('Ctrl Pts',(55.8202778804352,23.3994879145773,12.2240449901205));
#40987=CARTESIAN_POINT('Ctrl Pts',(53.4286379598932,22.9902812344603,12.3510782848295));
#40988=CARTESIAN_POINT('Ctrl Pts',(52.4756684956452,20.7588599795662,12.4781115795385));
#40989=CARTESIAN_POINT('Ctrl Pts',(53.8338667091912,18.7482159958377,12.6051448742475));
#40990=CARTESIAN_POINT('Ctrl Pts',(56.2597256341247,18.7992071019601,12.7321781689565));
#40991=CARTESIAN_POINT('Ctrl Pts',(57.5322347856805,20.8651480681519,12.8592114636654));
#40992=CARTESIAN_POINT('Ctrl Pts',(56.4863403602281,23.0545535736237,12.9862447583744));
#40993=CARTESIAN_POINT('Ctrl Pts',(54.079617615344,23.3628995576089,13.1132780530834));
#40994=CARTESIAN_POINT('Ctrl Pts',(52.5155567850928,21.5078779038655,13.2403113477924));
#40995=CARTESIAN_POINT('Ctrl Pts',(53.2261436568976,19.1878654223903,13.3673446425014));
#40996=CARTESIAN_POINT('Ctrl Pts',(55.5607959250878,18.5269642170526,13.4943779372104));
#40997=CARTESIAN_POINT('Ctrl Pts',(57.3820079364554,20.1302665672765,13.6214112319193));
#40998=CARTESIAN_POINT('Ctrl Pts',(57.0223575129614,22.529858863785,13.7484445266283));
#40999=CARTESIAN_POINT('Ctrl Pts',(54.8111248749932,23.5287791996311,13.8754778213373));
#41000=CARTESIAN_POINT('Ctrl Pts',(52.7728180525535,22.2124597421367,14.0025111160463));
#41001=CARTESIAN_POINT('Ctrl Pts',(52.7736217513052,19.7860650976794,14.1295444107553));
#41002=CARTESIAN_POINT('Ctrl Pts',(54.8128001397719,18.4710962324233,14.2565777054643));
#41003=CARTESIAN_POINT('Ctrl Pts',(57.0233705445013,19.4714812094783,14.3836110001732));
#41004=CARTESIAN_POINT('Ctrl Pts',(57.3814312473215,21.8713112346423,14.5106442948822));
#41005=CARTESIAN_POINT('Ctrl Pts',(55.5591575066651,23.4734067469936,14.6376775895912));
#41006=CARTESIAN_POINT('Ctrl Pts',(53.2249435735374,22.8109590653041,14.7647108843002));
#41007=CARTESIAN_POINT('Ctrl Pts',(52.5158937807075,20.4904763552047,14.8917441790092));
#41008=CARTESIAN_POINT('Ctrl Pts',(54.0811831514666,18.6364912413565,15.0187774737181));
#41009=CARTESIAN_POINT('Ctrl Pts',(56.4877011003582,18.9464315230977,15.1458107684271));
#41010=CARTESIAN_POINT('Ctrl Pts',(57.5321448955836,21.1365294147907,15.2728440631361));
#41011=CARTESIAN_POINT('Ctrl Pts',(56.2582674132478,23.2016269370836,15.3998773578451));
#41012=CARTESIAN_POINT('Ctrl Pts',(53.832375240883,23.2510109895845,15.5269106525541));
#41013=CARTESIAN_POINT('Ctrl Pts',(52.4755093031501,21.2394676906214,15.653943947263));
#41014=CARTESIAN_POINT('Ctrl Pts',(53.4299567929073,19.0086782326316,15.780977241972));
#41015=CARTESIAN_POINT('Ctrl Pts',(55.8218672730494,18.6010560159054,15.908010536681));
#41016=CARTESIAN_POINT('Ctrl Pts',(57.461311972199,20.3898021395946,16.03504383139));
#41017=CARTESIAN_POINT('Ctrl Pts',(56.8472869248829,22.7372187745043,16.162077126099));
#41018=CARTESIAN_POINT('Ctrl Pts',(54.5419666475085,23.4941137707287,16.289110420808));
#41019=CARTESIAN_POINT('Ctrl Pts',(52.6560017035378,21.9675071263385,16.4161437155169));
#41020=CARTESIAN_POINT('Ctrl Pts',(52.9160992280829,19.5550932119557,16.5431770102259));
#41021=CARTESIAN_POINT('Ctrl Pts',(55.0841252871632,18.4655728478819,16.6702103049349));
#41022=CARTESIAN_POINT('Ctrl Pts',(57.1751299074027,19.6964632957773,16.7972435996439));
#41023=CARTESIAN_POINT('Ctrl Pts',(57.2746805809953,22.1208150194284,16.9242768943529));
#41024=CARTESIAN_POINT('Ctrl Pts',(55.2916330589735,23.5189974617389,17.0513101890619));
#41025=CARTESIAN_POINT('Ctrl Pts',(53.0415790449306,22.6108958427156,17.1783434837708));
#41026=CARTESIAN_POINT('Ctrl Pts',(52.58456972532,20.2279283443282,17.3053767784798));
#41027=CARTESIAN_POINT('Ctrl Pts',(54.3390228737627,18.5518359344349,17.4324100731888));
#41028=CARTESIAN_POINT('Ctrl Pts',(56.6986378114894,19.1171756219148,17.5594433678978));
#41029=CARTESIAN_POINT('Ctrl Pts',(57.5030541552832,21.4063470795431,17.6864766626068));
#41030=CARTESIAN_POINT('Ctrl Pts',(56.0157834328264,23.3234848979343,17.8135099573157));
#41031=CARTESIAN_POINT('Ctrl Pts',(53.5985057625751,23.1133414196002,17.9405432520247));
#41032=CARTESIAN_POINT('Ctrl Pts',(52.4643750072844,20.9683148355023,18.0675765467337));
#41033=CARTESIAN_POINT('Ctrl Pts',(53.6517517544994,18.8522978042014,18.1946098414427));
#41034=CARTESIAN_POINT('Ctrl Pts',(56.0735257119335,18.7026231046798,18.3216431361517));
#41035=CARTESIAN_POINT('Ctrl Pts',(57.5124264126573,20.6563263549304,18.4486764308606));
#41036=CARTESIAN_POINT('Ctrl Pts',(56.6510592176025,22.9246821850121,18.5757097255696));
#41037=CARTESIAN_POINT('Ctrl Pts',(54.2780543112314,23.4308830650201,18.7027430202786));
#41038=CARTESIAN_POINT('Ctrl Pts',(52.5660313472582,21.711473577024,18.8297763149876));
#41039=CARTESIAN_POINT('Ctrl Pts',(53.0824437806473,19.3406699547845,18.9568096096966));
#41040=CARTESIAN_POINT('Ctrl Pts',(55.3544869411717,18.4890764524041,19.0838429044055));
#41041=CARTESIAN_POINT('Ctrl Pts',(57.3019773402135,19.9363748881879,19.2108761991145));
#41042=CARTESIAN_POINT('Ctrl Pts',(57.1418778230586,22.3574820236096,19.3379094938235));
#41043=CARTESIAN_POINT('Ctrl Pts',(55.0207685154315,23.5357379048514,19.4649427885325));
#41044=CARTESIAN_POINT('Ctrl Pts',(52.8806444621192,22.3923829061673,19.5919760832415));
#41045=CARTESIAN_POINT('Ctrl Pts',(52.6809097786076,19.9742229294939,19.7190093779505));
#41046=CARTESIAN_POINT('Ctrl Pts',(54.6044328179128,18.4952196388129,19.8460426726595));
#41047=CARTESIAN_POINT('Ctrl Pts',(56.8901198931453,19.3094838531177,19.9730759673684));
#41048=CARTESIAN_POINT('Ctrl Pts',(57.4452957432646,21.6715108199466,20.1001092620774));
#41049=CARTESIAN_POINT('Ctrl Pts',(55.7616656066381,23.4187318075798,20.2271425567864));
#41050=CARTESIAN_POINT('Ctrl Pts',(53.3806877055391,22.9514675878275,20.3541758514954));
#41051=CARTESIAN_POINT('Ctrl Pts',(52.4822814194424,20.6975248730086,20.4812091462044));
#41052=CARTESIAN_POINT('Ctrl Pts',(53.8889883069237,18.7205151741717,20.6082424409133));
#41053=CARTESIAN_POINT('Ctrl Pts',(56.312888978288,18.8305022276979,20.7352757356224));
#41054=CARTESIAN_POINT('Ctrl Pts',(57.5347658402131,20.9267866909505,20.8623090303313));
#41055=CARTESIAN_POINT('Ctrl Pts',(56.4359218021414,23.0901020624526,20.9893423250403));
#41056=CARTESIAN_POINT('Ctrl Pts',(54.0224104744431,23.33981126864,21.1163756197492));
#41057=CARTESIAN_POINT('Ctrl Pts',(52.5039374211234,21.4472914661216,21.2434089144583));
#41058=CARTESIAN_POINT('Ctrl Pts',(53.2707502520462,19.1452511322188,21.3704422091672));
#41059=CARTESIAN_POINT('Ctrl Pts',(55.620788628984,18.5413378573993,21.4974755038762));
#41060=CARTESIAN_POINT('Ctrl Pts',(57.4024600495314,20.1884682607939,21.6245087985852));
#41061=CARTESIAN_POINT('Ctrl Pts',(56.9845439737103,22.5786016817879,21.7515420932942));
#41062=CARTESIAN_POINT('Ctrl Pts',(54.7496661084856,23.5234363467488,21.8785753880032));
#41063=CARTESIAN_POINT('Ctrl Pts',(52.7439830212551,22.1579229011245,22.0056086827121));
#41064=CARTESIAN_POINT('Ctrl Pts',(52.8038105505325,19.7322658183275,22.1326419774211));
#41065=CARTESIAN_POINT('Ctrl Pts',(54.8743732234172,18.4672907852779,22.2596752721301));
#41066=CARTESIAN_POINT('Ctrl Pts',(57.0599542863205,19.5211536957466,22.3867085668391));
#41067=CARTESIAN_POINT('Ctrl Pts',(57.3595311710622,21.9289836952922,22.5137418615481));
#41068=CARTESIAN_POINT('Ctrl Pts',(55.4988243656874,23.4862767958393,22.640775156257));
#41069=CARTESIAN_POINT('Ctrl Pts',(53.1814157567314,22.7672434477095,22.767808450966));
#41070=CARTESIAN_POINT('Ctrl Pts',(52.5290234561101,20.430199181403,22.894841745675));
#41071=CARTESIAN_POINT('Ctrl Pts',(54.1389493616999,18.6148396591396,23.021875040384));
#41072=CARTESIAN_POINT('Ctrl Pts',(56.5372156262214,18.9832287755273,23.148908335093));
#41073=CARTESIAN_POINT('Ctrl Pts',(57.5280743996752,21.1980855446349,23.275941629802));
#41074=CARTESIAN_POINT('Ctrl Pts',(56.2043386638812,23.2315838402376,23.4029749245109));
#41075=CARTESIAN_POINT('Ctrl Pts',(53.7779630456277,23.2219414338976,23.5300082192199));
#41076=CARTESIAN_POINT('Ctrl Pts',(52.4704310917174,21.1779864916192,23.6570415139289));
#41077=CARTESIAN_POINT('Ctrl Pts',(53.4788619536403,18.971074891145,23.7840748086379));
#41078=CARTESIAN_POINT('Ctrl Pts',(55.8799803771704,18.6217585088131,23.9111081033468));
#41079=CARTESIAN_POINT('Ctrl Pts',(57.4754271986143,20.4498561691353,24.0381413980558));
#41080=CARTESIAN_POINT('Ctrl Pts',(56.8044809906924,22.7816414928851,24.1651746927648));
#41081=CARTESIAN_POINT('Ctrl Pts',(54.4814307927619,23.4822336793536,24.2922079874738));
#41082=CARTESIAN_POINT('Ctrl Pts',(52.6331599204118,21.9102011136452,24.4192412821828));
#41083=CARTESIAN_POINT('Ctrl Pts',(52.9518644411195,19.5048281689401,24.5462745768917));
#41084=CARTESIAN_POINT('Ctrl Pts',(55.1457524576671,18.4683692359229,24.6733078716008));
#41085=CARTESIAN_POINT('Ctrl Pts',(57.2061958341146,19.7497608968377,24.8003411663097));
#41086=CARTESIAN_POINT('Ctrl Pts',(57.2467427666359,22.1758168136955,24.9273744610187));
#41087=CARTESIAN_POINT('Ctrl Pts',(55.2302699341218,23.5253463336973,25.0544077557277));
#41088=CARTESIAN_POINT('Ctrl Pts',(53.0029724215312,22.5627787976819,25.1814410504367));
#41089=CARTESIAN_POINT('Ctrl Pts',(52.6040653304014,20.1693997260389,25.3084743451457));
#41090=CARTESIAN_POINT('Ctrl Pts',(54.3987729693717,18.5364810532685,25.4355076398546));
#41091=CARTESIAN_POINT('Ctrl Pts',(56.7439347165923,19.1590545677295,25.5625409345636));
#41092=CARTESIAN_POINT('Ctrl Pts',(57.4924320706083,21.4671137370528,25.6895742292726));
#41093=CARTESIAN_POINT('Ctrl Pts',(55.9589556062135,23.3475109740183,25.8166075239816));
#41094=CARTESIAN_POINT('Ctrl Pts',(53.547524482996,23.0786159890765,25.9436408186906));
#41095=CARTESIAN_POINT('Ctrl Pts',(52.4658711091553,20.9066577783214,26.0706741133995));
#41096=CARTESIAN_POINT('Ctrl Pts',(53.7044442609637,18.8201072296902,26.1977074081085));
#41097=CARTESIAN_POINT('Ctrl Pts',(56.1289980153912,18.7294737786598,26.3247407028175));
#41098=CARTESIAN_POINT('Ctrl Pts',(57.5202301228141,20.7174345305146,26.4517739975265));
#41099=CARTESIAN_POINT('Ctrl Pts',(56.6033852487809,22.964492045205,26.5788072922355));
#41100=CARTESIAN_POINT('Ctrl Pts',(54.2198514610545,23.4121779339536,26.7058405869444));
#41101=CARTESIAN_POINT('Ctrl Pts',(52.5480301270164,21.6528985747657,26.8328738816534));
#41102=CARTESIAN_POINT('Ctrl Pts',(53.126355659332,19.2923779831827,26.9599247822321));
#41103=CARTESIAN_POINT('Ctrl Pts',(54.6482802028138,18.7665406546803,27.0446312512411));
#41104=CARTESIAN_POINT('Ctrl Pts',(55.3523638033544,18.8837997984075,27.0869932886805));
#41105=CARTESIAN_POINT('Ctrl Pts',(53.9911528061724,23.0663949408297,7.61282769962002));
#41106=CARTESIAN_POINT('Ctrl Pts',(53.3039269064612,22.7308802206034,7.65517213118968));
#41107=CARTESIAN_POINT('Ctrl Pts',(52.3025342441699,21.3258080694959,7.739860994329));
#41108=CARTESIAN_POINT('Ctrl Pts',(53.2649891419755,18.905521742655,7.86689428903798));
#41109=CARTESIAN_POINT('Ctrl Pts',(55.8184834988608,18.408799415075,7.99392758374697));
#41110=CARTESIAN_POINT('Ctrl Pts',(57.6213217604298,20.2815504187016,8.12096087845594));
#41111=CARTESIAN_POINT('Ctrl Pts',(57.0248501218595,22.8135620848035,8.24799417316493));
#41112=CARTESIAN_POINT('Ctrl Pts',(54.5741778805022,23.6844000698069,8.37502746787391));
#41113=CARTESIAN_POINT('Ctrl Pts',(52.5135417022076,22.0979047531258,8.50206076258288));
#41114=CARTESIAN_POINT('Ctrl Pts',(52.7293102399626,19.5060183539129,8.62909405729188));
#41115=CARTESIAN_POINT('Ctrl Pts',(55.0240681001933,18.2820572543959,8.75612735200084));
#41116=CARTESIAN_POINT('Ctrl Pts',(57.2967672764985,19.5464742112274,8.88316064670985));
#41117=CARTESIAN_POINT('Ctrl Pts',(57.4666583946333,22.1417022919548,9.01019394141881));
#41118=CARTESIAN_POINT('Ctrl Pts',(55.3781788068818,23.6916241218337,9.13722723612782));
#41119=CARTESIAN_POINT('Ctrl Pts',(52.9434582923559,22.7772193598424,9.26426053083678));
#41120=CARTESIAN_POINT('Ctrl Pts',(52.3916159771276,20.2356666420876,9.39129382554576));
#41121=CARTESIAN_POINT('Ctrl Pts',(54.2278969579434,18.3939059693325,9.51832712025476));
#41122=CARTESIAN_POINT('Ctrl Pts',(56.7710813525697,18.9381702501774,9.64536041496372));
#41123=CARTESIAN_POINT('Ctrl Pts',(57.6927412209364,21.3701562732864,9.77239370967272));
#41124=CARTESIAN_POINT('Ctrl Pts',(56.149044722759,23.4632431376211,9.89942700438167));
#41125=CARTESIAN_POINT('Ctrl Pts',(53.5533331146744,23.3010922880737,10.0264602990907));
#41126=CARTESIAN_POINT('Ctrl Pts',(52.2821264970286,21.0321617743691,10.1534935937996));
#41127=CARTESIAN_POINT('Ctrl Pts',(53.4992861727145,18.7337853769208,10.2805268885086));
#41128=CARTESIAN_POINT('Ctrl Pts',(56.0904338791848,18.5102560972785,10.4075601832176));
#41129=CARTESIAN_POINT('Ctrl Pts',(57.6832279532088,20.5662276063806,10.5345934779266));
#41130=CARTESIAN_POINT('Ctrl Pts',(56.8193756985891,23.0193421702064,10.6616267726356));
#41131=CARTESIAN_POINT('Ctrl Pts',(54.2897825146926,23.6236352378958,10.7886600673446));
#41132=CARTESIAN_POINT('Ctrl Pts',(52.4104334418206,21.8258424652233,10.9156933620535));
#41133=CARTESIAN_POINT('Ctrl Pts',(52.9019784132069,19.2719443997923,11.0427266567625));
#41134=CARTESIAN_POINT('Ctrl Pts',(55.3143803203856,18.3001785705584,11.1697599514715));
#41135=CARTESIAN_POINT('Ctrl Pts',(57.438949336525,19.8002513303359,11.2967932461805));
#41136=CARTESIAN_POINT('Ctrl Pts',(57.3305228587221,22.3987615741865,11.4238265408895));
#41137=CARTESIAN_POINT('Ctrl Pts',(55.0883714346901,23.7166268102304,11.5508598355984));
#41138=CARTESIAN_POINT('Ctrl Pts',(52.7653109845788,22.5472671847012,11.6778931303074));
#41139=CARTESIAN_POINT('Ctrl Pts',(52.4882341992375,19.9612973001794,11.8049264250164));
#41140=CARTESIAN_POINT('Ctrl Pts',(54.5108204822733,18.3263182433315,11.9319597197254));
#41141=CARTESIAN_POINT('Ctrl Pts',(56.9812781673263,19.1392454325794,12.0589930144344));
#41142=CARTESIAN_POINT('Ctrl Pts',(57.6377640926697,21.6557982372063,12.1860263091434));
#41143=CARTESIAN_POINT('Ctrl Pts',(55.8792284164104,23.5719308171641,12.3130596038523));
#41144=CARTESIAN_POINT('Ctrl Pts',(53.3157096014861,23.1333158673706,12.4400928985613));
#41145=CARTESIAN_POINT('Ctrl Pts',(52.2942535157833,20.7415300797984,12.5671261932703));
#41146=CARTESIAN_POINT('Ctrl Pts',(53.7500607403224,18.5863880627537,12.6941594879793));
#41147=CARTESIAN_POINT('Ctrl Pts',(56.3502577612055,18.6410437234223,12.8211927826883));
#41148=CARTESIAN_POINT('Ctrl Pts',(57.7142177470537,20.8554567259259,12.9482260773972));
#41149=CARTESIAN_POINT('Ctrl Pts',(56.5931585043799,23.2022072373923,13.0752593721062));
#41150=CARTESIAN_POINT('Ctrl Pts',(54.013472914662,23.5327129814481,13.2022926668152));
#41151=CARTESIAN_POINT('Ctrl Pts',(52.3370084387196,21.5443773333356,13.3293259615242));
#41152=CARTESIAN_POINT('Ctrl Pts',(53.0986627328562,19.0576335739436,13.4563592562332));
#41153=CARTESIAN_POINT('Ctrl Pts',(55.6010983898319,18.3492356833845,13.5833925509422));
#41154=CARTESIAN_POINT('Ctrl Pts',(57.5531946134341,20.0677618317017,13.7104258456511));
#41155=CARTESIAN_POINT('Ctrl Pts',(57.1676973571359,22.6398045323657,13.8374591403601));
#41156=CARTESIAN_POINT('Ctrl Pts',(54.7975510726062,23.7105138199792,13.9644924350691));
#41157=CARTESIAN_POINT('Ctrl Pts',(52.6127581842486,22.2995950329349,14.0915257297781));
#41158=CARTESIAN_POINT('Ctrl Pts',(52.6136196420517,19.6988237922175,14.2185590244871));
#41159=CARTESIAN_POINT('Ctrl Pts',(54.7993467328741,18.2893526598075,14.345592319196));
#41160=CARTESIAN_POINT('Ctrl Pts',(57.168783191751,19.3616318473313,14.472625613905));
#41161=CARTESIAN_POINT('Ctrl Pts',(57.5525764796455,21.9339293613873,14.599658908614));
#41162=CARTESIAN_POINT('Ctrl Pts',(55.5993422239403,23.6511619405656,14.726692203323));
#41163=CARTESIAN_POINT('Ctrl Pts',(53.097376403653,22.9411064337446,14.853725498032));
#41164=CARTESIAN_POINT('Ctrl Pts',(52.3373696530442,20.4538586520226,14.9807587927409));
#41165=CARTESIAN_POINT('Ctrl Pts',(54.0151509604544,18.4666340363447,15.1077920874499));
#41166=CARTESIAN_POINT('Ctrl Pts',(56.5946170361996,18.7988486548256,15.2348253821589));
#41167=CARTESIAN_POINT('Ctrl Pts',(57.7141213968662,21.1463413119175,15.3618586768679));
#41168=CARTESIAN_POINT('Ctrl Pts',(56.3486947430345,23.3598502551246,15.4888919715769));
#41169=CARTESIAN_POINT('Ctrl Pts',(53.7484620853422,23.4127833687828,15.6159252662859));
#41170=CARTESIAN_POINT('Ctrl Pts',(52.2940828826737,21.2566774058259,15.7429585609948));
#41171=CARTESIAN_POINT('Ctrl Pts',(53.3171232144706,18.8655688202178,15.8699918557038));
#41172=CARTESIAN_POINT('Ctrl Pts',(55.8809320331778,18.4286522037224,15.9970251504128));
#41173=CARTESIAN_POINT('Ctrl Pts',(57.6381979561121,20.3459493285172,16.1240584451218));
#41174=CARTESIAN_POINT('Ctrl Pts',(56.9800450510238,22.8620666831285,16.2510917398307));
#41175=CARTESIAN_POINT('Ctrl Pts',(54.5090493736581,23.6733571065227,16.3781250345398));
#41176=CARTESIAN_POINT('Ctrl Pts',(52.4875466480051,22.0370385193185,16.5051583292487));
#41177=CARTESIAN_POINT('Ctrl Pts',(52.7663364826117,19.4512527554216,16.6321916239577));
#41178=CARTESIAN_POINT('Ctrl Pts',(55.0901710807725,18.2834323287108,16.7592249186667));
#41179=CARTESIAN_POINT('Ctrl Pts',(57.3314489755076,19.6027826185216,16.8862582133757));
#41180=CARTESIAN_POINT('Ctrl Pts',(57.4381540119143,22.2013641207758,17.0132915080847));
#41181=CARTESIAN_POINT('Ctrl Pts',(55.3125917188917,23.7000291023953,17.1403248027936));
#41182=CARTESIAN_POINT('Ctrl Pts',(52.900834100175,22.7266653588675,17.2673580975026));
#41183=CARTESIAN_POINT('Ctrl Pts',(52.4109811004174,20.1724422231019,17.3943913922116));
#41184=CARTESIAN_POINT('Ctrl Pts',(54.2915207323686,18.3758948451258,17.5214246869206));
#41185=CARTESIAN_POINT('Ctrl Pts',(56.8207130396567,18.9818635418474,17.6484579816296));
#41186=CARTESIAN_POINT('Ctrl Pts',(57.6829400056126,21.4355498396105,17.7754912763385));
#41187=CARTESIAN_POINT('Ctrl Pts',(56.0887842770866,23.4904657264195,17.9025245710475));
#41188=CARTESIAN_POINT('Ctrl Pts',(53.4977852159983,23.2652199626587,18.0295578657565));
#41189=CARTESIAN_POINT('Ctrl Pts',(52.2821484034498,20.9660377322496,18.1565911604655));
#41190=CARTESIAN_POINT('Ctrl Pts',(53.5548578133176,18.6979498709256,18.2836244551745));
#41191=CARTESIAN_POINT('Ctrl Pts',(56.1506762942069,18.5375185681002,18.4106577498834));
#41192=CARTESIAN_POINT('Ctrl Pts',(57.6929858147289,20.6316277179677,18.5376910445924));
#41193=CARTESIAN_POINT('Ctrl Pts',(56.7697151366827,23.0630024409818,18.6647243393014));
#41194=CARTESIAN_POINT('Ctrl Pts',(54.226170569986,23.6055822285518,18.7917576340104));
#41195=CARTESIAN_POINT('Ctrl Pts',(52.3911104332023,21.7626047237951,18.9187909287194));
#41196=CARTESIAN_POINT('Ctrl Pts',(52.9446356431986,19.2214196399119,19.0458242234284));
#41197=CARTESIAN_POINT('Ctrl Pts',(55.3799626923489,18.3086250560496,19.1728575181373));
#41198=CARTESIAN_POINT('Ctrl Pts',(57.4674124948662,19.859935827824,19.2998908128463));
#41199=CARTESIAN_POINT('Ctrl Pts',(57.2958071787975,22.4550395645076,19.4269241075553));
#41200=CARTESIAN_POINT('Ctrl Pts',(55.0222610768493,23.7179726232908,19.5539574022643));
#41201=CARTESIAN_POINT('Ctrl Pts',(52.7283337051675,22.4924486528597,19.6809906969732));
#41202=CARTESIAN_POINT('Ctrl Pts',(52.5142447803355,19.9005038770367,19.8080239916823));
#41203=CARTESIAN_POINT('Ctrl Pts',(54.5760047718148,18.3152097320318,19.9350572863912));
#41204=CARTESIAN_POINT('Ctrl Pts',(57.0259562766631,19.1879923009132,20.0620905811002));
#41205=CARTESIAN_POINT('Ctrl Pts',(57.6210306961643,21.7197699814979,20.1891238758092));
#41206=CARTESIAN_POINT('Ctrl Pts',(55.8164038810887,23.5925577022401,20.3161571705182));
#41207=CARTESIAN_POINT('Ctrl Pts',(53.2643133280918,23.0917128181136,20.4431904652271));
#41208=CARTESIAN_POINT('Ctrl Pts',(52.3013416875561,20.6757870311375,20.5702237599362));
#41209=CARTESIAN_POINT('Ctrl Pts',(53.8091437367561,18.5566964787825,20.6972570546451));
#41210=CARTESIAN_POINT('Ctrl Pts',(56.4072417711545,18.6745879216752,20.8242903493541));
#41211=CARTESIAN_POINT('Ctrl Pts',(57.716930699727,20.9215251034911,20.9513236440631));
#41212=CARTESIAN_POINT('Ctrl Pts',(56.5391165387953,23.2403104732399,21.0783569387721));
#41213=CARTESIAN_POINT('Ctrl Pts',(53.9521544942811,23.5079654169557,21.205390233481));
#41214=CARTESIAN_POINT('Ctrl Pts',(52.324554031224,21.479436757728,21.33242352819));
#41215=CARTESIAN_POINT('Ctrl Pts',(53.1464750498154,19.011956742034,21.459456822899));
#41216=CARTESIAN_POINT('Ctrl Pts',(55.665402561992,18.3646423075804,21.586490117608));
#41217=CARTESIAN_POINT('Ctrl Pts',(57.5751165491841,20.130146279758,21.713523412317));
#41218=CARTESIAN_POINT('Ctrl Pts',(57.1271662895212,22.6920503282187,21.840556707026));
#41219=CARTESIAN_POINT('Ctrl Pts',(54.7316754769819,23.7047869947277,21.9675900017349));
#41220=CARTESIAN_POINT('Ctrl Pts',(52.5818508789192,22.2411388176659,22.0946232964439));
#41221=CARTESIAN_POINT('Ctrl Pts',(52.6459780059317,19.641158144616,22.2216565911529));
#41222=CARTESIAN_POINT('Ctrl Pts',(54.8653448612133,18.2852737283293,22.3486898858619));
#41223=CARTESIAN_POINT('Ctrl Pts',(57.207996080643,19.4148741234946,22.4757231805709));
#41224=CARTESIAN_POINT('Ctrl Pts',(57.529102520603,21.9957465424392,22.6027564752798));
#41225=CARTESIAN_POINT('Ctrl Pts',(55.5346731486622,23.6649569153365,22.7297897699888));
#41226=CARTESIAN_POINT('Ctrl Pts',(53.050720393107,22.8942491258165,22.8568230646978));
#41227=CARTESIAN_POINT('Ctrl Pts',(52.3514429128353,20.389249566088,22.9838563594068));
#41228=CARTESIAN_POINT('Ctrl Pts',(54.0770686285482,18.4434264297526,23.1108896541158));
#41229=CARTESIAN_POINT('Ctrl Pts',(56.6476899998897,18.8382903985975,23.2379229488247));
#41230=CARTESIAN_POINT('Ctrl Pts',(57.7097583684865,21.2123212680449,23.3649562435337));
#41231=CARTESIAN_POINT('Ctrl Pts',(56.2908903208558,23.3919600573624,23.4919895382427));
#41232=CARTESIAN_POINT('Ctrl Pts',(53.6901394736897,23.3816246846075,23.6190228329517));
#41233=CARTESIAN_POINT('Ctrl Pts',(52.2886397177381,21.1907777655613,23.7460561276607));
#41234=CARTESIAN_POINT('Ctrl Pts',(53.3695430200646,18.8252630565545,23.8730894223697));
#41235=CARTESIAN_POINT('Ctrl Pts',(55.943221525224,18.4508425132372,24.0001227170786));
#41236=CARTESIAN_POINT('Ctrl Pts',(57.6533275950606,20.4103192335841,24.1271560117877));
#41237=CARTESIAN_POINT('Ctrl Pts',(56.934162802302,22.9096819087321,24.2541893064966));
#41238=CARTESIAN_POINT('Ctrl Pts',(54.444163016273,23.6606232340439,24.3812226012056));
#41239=CARTESIAN_POINT('Ctrl Pts',(52.4630633048785,21.9756141215713,24.5082558959146));
#41240=CARTESIAN_POINT('Ctrl Pts',(52.8046720178866,19.3973753375057,24.6352891906235));
#41241=CARTESIAN_POINT('Ctrl Pts',(55.1562271830061,18.2864296834945,24.7623224853325));
#41242=CARTESIAN_POINT('Ctrl Pts',(57.3647475029929,19.6599105339469,24.8893557800415));
#41243=CARTESIAN_POINT('Ctrl Pts',(57.408208403404,22.2603187038831,25.0163890747505));
#41244=CARTESIAN_POINT('Ctrl Pts',(55.2468186383588,23.7068342458364,25.1434223694595));
#41245=CARTESIAN_POINT('Ctrl Pts',(52.8594529521957,22.6750903081238,25.2704556641685));
#41246=CARTESIAN_POINT('Ctrl Pts',(52.4318777872494,20.1097073553205,25.3974889588775));
#41247=CARTESIAN_POINT('Ctrl Pts',(54.3555648608227,18.3594364617242,25.5245222535864));
#41248=CARTESIAN_POINT('Ctrl Pts',(56.8692652767605,19.0267521827433,25.6515555482954));
#41249=CARTESIAN_POINT('Ctrl Pts',(57.6715545484274,21.5006835867554,25.7785888430044));
#41250=CARTESIAN_POINT('Ctrl Pts',(56.0278724310004,23.5162184735454,25.9056221377133));
#41251=CARTESIAN_POINT('Ctrl Pts',(53.4431400880731,23.2279989354718,26.0326554324224));
#41252=CARTESIAN_POINT('Ctrl Pts',(52.2837520249908,20.899949595487,26.1596887271313));
#41253=CARTESIAN_POINT('Ctrl Pts',(53.6113371480899,18.663445871091,26.2867220218403));
#41254=CARTESIAN_POINT('Ctrl Pts',(56.2101352003739,18.5662989072097,26.4137553165493));
#41255=CARTESIAN_POINT('Ctrl Pts',(57.7013503505611,20.6971275269108,26.5407886112583));
#41256=CARTESIAN_POINT('Ctrl Pts',(56.7186150045072,23.1056732982239,26.6678219059673));
#41257=CARTESIAN_POINT('Ctrl Pts',(54.1637848821451,23.5855328243699,26.7948552006763));
#41258=CARTESIAN_POINT('Ctrl Pts',(52.3718155274831,21.6998201385892,26.9218884953852));
#41259=CARTESIAN_POINT('Ctrl Pts',(52.9917033168228,19.1696570912324,27.0489393959639));
#41260=CARTESIAN_POINT('Ctrl Pts',(54.6230033167101,18.606029651488,27.1336458649729));
#41261=CARTESIAN_POINT('Ctrl Pts',(55.3776869719554,18.7317158045685,27.1760079024124));
#41262=CARTESIAN_POINT('Ctrl Pts',(53.9235115861173,23.2049426572415,7.70184231335182));
#41263=CARTESIAN_POINT('Ctrl Pts',(53.190208541528,22.8469323349445,7.74418674492148));
#41264=CARTESIAN_POINT('Ctrl Pts',(52.121674470859,21.347652859727,7.8288756080608));
#41265=CARTESIAN_POINT('Ctrl Pts',(53.1486600765197,18.7650910951076,7.95590890276978));
#41266=CARTESIAN_POINT('Ctrl Pts',(55.8733612075929,18.2350645124613,8.08294219747876));
#41267=CARTESIAN_POINT('Ctrl Pts',(57.7970762286159,20.2333797873867,8.20997549218775));
#41268=CARTESIAN_POINT('Ctrl Pts',(57.1606123398736,22.935157855513,8.33700878689672));
#41269=CARTESIAN_POINT('Ctrl Pts',(54.5456273449349,23.8643838145687,8.46404208160572));
#41270=CARTESIAN_POINT('Ctrl Pts',(52.3468295639297,22.1715171073655,8.59107537631469));
#41271=CARTESIAN_POINT('Ctrl Pts',(52.5770649577483,19.4058498230397,8.71810867102368));
#41272=CARTESIAN_POINT('Ctrl Pts',(55.025681818972,18.0998245391965,8.84514196573266));
#41273=CARTESIAN_POINT('Ctrl Pts',(57.4507610049,19.449018166015,8.97217526044164));
#41274=CARTESIAN_POINT('Ctrl Pts',(57.6320429883485,22.218251185028,9.09920855515061));
#41275=CARTESIAN_POINT('Ctrl Pts',(55.4035349520473,23.872092225075,9.22624184985961));
#41276=CARTESIAN_POINT('Ctrl Pts',(52.8055712158489,22.8963784223254,9.35327514456858));
#41277=CARTESIAN_POINT('Ctrl Pts',(52.2167289587976,20.1844195937989,9.48030843927757));
#41278=CARTESIAN_POINT('Ctrl Pts',(54.1761289676149,18.2191724904756,9.60734173398655));
#41279=CARTESIAN_POINT('Ctrl Pts',(56.889828873738,18.7999286208435,9.73437502869553));
#41280=CARTESIAN_POINT('Ctrl Pts',(57.8732842234754,21.3949745233537,9.86140832340451));
#41281=CARTESIAN_POINT('Ctrl Pts',(56.2260859113758,23.6283987450711,9.98844161811349));
#41282=CARTESIAN_POINT('Ctrl Pts',(53.4563369454474,23.4553759999944,10.1154749128224));
#41283=CARTESIAN_POINT('Ctrl Pts',(52.0998984244116,21.0343181580819,10.2425082075314));
#41284=CARTESIAN_POINT('Ctrl Pts',(53.3986662623335,18.5818401438375,10.3695415022404));
#41285=CARTESIAN_POINT('Ctrl Pts',(56.1635453260211,18.3433236656525,10.4965747969494));
#41286=CARTESIAN_POINT('Ctrl Pts',(57.8631331098581,20.5371440205708,10.6236080916584));
#41287=CARTESIAN_POINT('Ctrl Pts',(56.9413612606683,23.1547350908955,10.7506413863674));
#41288=CARTESIAN_POINT('Ctrl Pts',(54.2421638292222,23.7995448201956,10.8776746810763));
#41289=CARTESIAN_POINT('Ctrl Pts',(52.2368080974863,21.8812135781755,11.0047079757853));
#41290=CARTESIAN_POINT('Ctrl Pts',(52.7613101923895,19.156081670693,11.1317412704943));
#41291=CARTESIAN_POINT('Ctrl Pts',(55.335458902516,18.1191608539651,11.2587745652033));
#41292=CARTESIAN_POINT('Ctrl Pts',(57.6024760923949,19.7198105418082,11.3858078599123));
#41293=CARTESIAN_POINT('Ctrl Pts',(57.4867798325181,22.492545786526,11.5128411546213));
#41294=CARTESIAN_POINT('Ctrl Pts',(55.0942965655693,23.8987712945513,11.6398744493302));
#41295=CARTESIAN_POINT('Ctrl Pts',(52.6154794814812,22.6510084061315,11.7669077440392));
#41296=CARTESIAN_POINT('Ctrl Pts',(52.3198252426627,19.89165432717,11.8939410387482));
#41297=CARTESIAN_POINT('Ctrl Pts',(54.4780219577718,18.1470531403838,12.0209743334572));
#41298=CARTESIAN_POINT('Ctrl Pts',(57.1141189714901,19.0144854987329,12.1480076281661));
#41299=CARTESIAN_POINT('Ctrl Pts',(57.8146209868923,21.6997682191282,12.2750409228752));
#41300=CARTESIAN_POINT('Ctrl Pts',(55.9381789523853,23.7443737197508,12.4020742175841));
#41301=CARTESIAN_POINT('Ctrl Pts',(53.2027812430792,23.2763505002808,12.5291075122931));
#41302=CARTESIAN_POINT('Ctrl Pts',(52.1128385359212,20.7242001800308,12.6561408070021));
#41303=CARTESIAN_POINT('Ctrl Pts',(53.6662547714537,18.4245601296697,12.7831741017111));
#41304=CARTESIAN_POINT('Ctrl Pts',(56.4407898882863,18.4828803448845,12.9102073964201));
#41305=CARTESIAN_POINT('Ctrl Pts',(57.8962007084268,20.8457653836999,13.037240691129));
#41306=CARTESIAN_POINT('Ctrl Pts',(56.6999766485317,23.3498609011608,13.164273985838));
#41307=CARTESIAN_POINT('Ctrl Pts',(53.94732821398,23.7025264052872,13.291307280547));
#41308=CARTESIAN_POINT('Ctrl Pts',(52.1584600923461,21.5808767628056,13.418340575256));
#41309=CARTESIAN_POINT('Ctrl Pts',(52.9711818088149,18.9274017254969,13.545373869965));
#41310=CARTESIAN_POINT('Ctrl Pts',(55.641400854576,18.1715071497163,13.6724071646739));
#41311=CARTESIAN_POINT('Ctrl Pts',(57.7243812904128,20.0052570961269,13.7994404593829));
#41312=CARTESIAN_POINT('Ctrl Pts',(57.3130372013104,22.7497502009462,13.9264737540919));
#41313=CARTESIAN_POINT('Ctrl Pts',(54.783977270219,23.8922484403271,14.0535070488009));
#41314=CARTESIAN_POINT('Ctrl Pts',(52.4526983159437,22.3867303237331,14.1805403435099));
#41315=CARTESIAN_POINT('Ctrl Pts',(52.453617532798,19.6115824867557,14.3075736382189));
#41316=CARTESIAN_POINT('Ctrl Pts',(54.7858933259761,18.1076090871918,14.4346069329278));
#41317=CARTESIAN_POINT('Ctrl Pts',(57.3141958390006,19.2517824851842,14.5616402276368));
#41318=CARTESIAN_POINT('Ctrl Pts',(57.7237217119695,21.9965474881324,14.6886735223458));
#41319=CARTESIAN_POINT('Ctrl Pts',(55.6395269412154,23.8289171341376,14.8157068170548));
#41320=CARTESIAN_POINT('Ctrl Pts',(52.9698092337686,23.0712538021851,14.9427401117638));
#41321=CARTESIAN_POINT('Ctrl Pts',(52.1588455253809,20.4172409488405,15.0697734064727));
#41322=CARTESIAN_POINT('Ctrl Pts',(53.9491187694424,18.2967768313329,15.1968067011817));
#41323=CARTESIAN_POINT('Ctrl Pts',(56.701532972041,18.6512657865535,15.3238399958907));
#41324=CARTESIAN_POINT('Ctrl Pts',(57.8960978981489,21.1561532090444,15.4508732905997));
#41325=CARTESIAN_POINT('Ctrl Pts',(56.4391220728212,23.5180735731657,15.5779065853087));
#41326=CARTESIAN_POINT('Ctrl Pts',(53.6645489298014,23.574555747981,15.7049398800177));
#41327=CARTESIAN_POINT('Ctrl Pts',(52.1126564621973,21.2738871210305,15.8319731747266));
#41328=CARTESIAN_POINT('Ctrl Pts',(53.2042896360337,18.7224594078039,15.9590064694356));
#41329=CARTESIAN_POINT('Ctrl Pts',(55.9399967933065,18.2562483915393,16.0860397641446));
#41330=CARTESIAN_POINT('Ctrl Pts',(57.8150839400251,20.3020965174398,16.2130730588536));
#41331=CARTESIAN_POINT('Ctrl Pts',(57.1128031771649,22.9869145917525,16.3401063535625));
#41332=CARTESIAN_POINT('Ctrl Pts',(54.4761320998075,23.8526004423166,16.4671396482715));
#41333=CARTESIAN_POINT('Ctrl Pts',(52.3190915924723,22.1065699122985,16.5941729429805));
#41334=CARTESIAN_POINT('Ctrl Pts',(52.6165737371404,19.3474122988875,16.7212062376895));
#41335=CARTESIAN_POINT('Ctrl Pts',(55.0962168743818,18.1012918095397,16.8482395323985));
#41336=CARTESIAN_POINT('Ctrl Pts',(57.4877680436125,19.5091019412658,16.9752728271075));
#41337=CARTESIAN_POINT('Ctrl Pts',(57.6016274428333,22.2819132221231,17.1023061218164));
#41338=CARTESIAN_POINT('Ctrl Pts',(55.3335503788099,23.8810607430516,17.2293394165254));
#41339=CARTESIAN_POINT('Ctrl Pts',(52.7600891554195,22.8424348750194,17.3563727112344));
#41340=CARTESIAN_POINT('Ctrl Pts',(52.2373924755148,20.1169561018757,17.4834060059434));
#41341=CARTESIAN_POINT('Ctrl Pts',(54.2440185909744,18.1999537558167,17.6104393006524));
#41342=CARTESIAN_POINT('Ctrl Pts',(56.9427882678241,18.84655146178,17.7374725953614));
#41343=CARTESIAN_POINT('Ctrl Pts',(57.862825855942,21.4647525996779,17.8645058900703));
#41344=CARTESIAN_POINT('Ctrl Pts',(56.1617851213467,23.6574465549046,17.9915391847793));
#41345=CARTESIAN_POINT('Ctrl Pts',(53.3970646694217,23.4170985057174,18.1185724794883));
#41346=CARTESIAN_POINT('Ctrl Pts',(52.0999217996153,20.963760628997,18.2456057741973));
#41347=CARTESIAN_POINT('Ctrl Pts',(53.4579638721358,18.5436019376496,18.3726390689062));
#41348=CARTESIAN_POINT('Ctrl Pts',(56.2278268764801,18.3724140315205,18.4996723636153));
#41349=CARTESIAN_POINT('Ctrl Pts',(57.8735452168006,20.6069290810051,18.6267056583242));
#41350=CARTESIAN_POINT('Ctrl Pts',(56.8883710557629,23.2013226969515,18.7537389530332));
#41351=CARTESIAN_POINT('Ctrl Pts',(54.1742868287406,23.7802813920835,18.8807722477422));
#41352=CARTESIAN_POINT('Ctrl Pts',(52.2161895191464,21.8137358705663,19.0078055424512));
#41353=CARTESIAN_POINT('Ctrl Pts',(52.8068275057499,19.1021693250393,19.1348388371601));
#41354=CARTESIAN_POINT('Ctrl Pts',(55.4054384435264,18.1281736596952,19.2618721318691));
#41355=CARTESIAN_POINT('Ctrl Pts',(57.6328476495188,19.7834967674601,19.3889054265781));
#41356=CARTESIAN_POINT('Ctrl Pts',(57.4497365345366,22.5525971054056,19.5159387212871));
#41357=CARTESIAN_POINT('Ctrl Pts',(55.0237536382671,23.9002073417302,19.6429720159961));
#41358=CARTESIAN_POINT('Ctrl Pts',(52.5760229482159,22.5925143995522,19.770005310705));
#41359=CARTESIAN_POINT('Ctrl Pts',(52.3475797820632,19.8267848245796,19.897038605414));
#41360=CARTESIAN_POINT('Ctrl Pts',(54.5475767257167,18.1351998252507,20.024071900123));
#41361=CARTESIAN_POINT('Ctrl Pts',(57.1617926601811,19.0665007487085,20.151105194832));
#41362=CARTESIAN_POINT('Ctrl Pts',(57.7967656490639,21.7680291430493,20.278138489541));
#41363=CARTESIAN_POINT('Ctrl Pts',(55.8711421555395,23.7663835969004,20.40517178425));
#41364=CARTESIAN_POINT('Ctrl Pts',(53.1479389506444,23.2319580483999,20.5322050789589));
#41365=CARTESIAN_POINT('Ctrl Pts',(52.1204019556699,20.6540491892665,20.6592383736679));
#41366=CARTESIAN_POINT('Ctrl Pts',(53.7292991665885,18.3928777833932,20.7862716683769));
#41367=CARTESIAN_POINT('Ctrl Pts',(56.5015945640211,18.5186736156525,20.9133049630859));
#41368=CARTESIAN_POINT('Ctrl Pts',(57.8990955592407,20.9162635160316,21.0403382577949));
#41369=CARTESIAN_POINT('Ctrl Pts',(56.6423112754491,23.390518884027,21.1673715525038));
#41370=CARTESIAN_POINT('Ctrl Pts',(53.8818985141192,23.6761195652714,21.2944048472128));
#41371=CARTESIAN_POINT('Ctrl Pts',(52.1451706413245,21.5115820493345,21.4214381419218));
#41372=CARTESIAN_POINT('Ctrl Pts',(53.0221998475846,18.878662351849,21.5484714366308));
#41373=CARTESIAN_POINT('Ctrl Pts',(55.7100164950001,18.1879467577614,21.6755047313398));
#41374=CARTESIAN_POINT('Ctrl Pts',(57.7477730488369,20.071824298722,21.8025380260487));
#41375=CARTESIAN_POINT('Ctrl Pts',(57.2697886053323,22.8054989746496,21.9295713207578));
#41376=CARTESIAN_POINT('Ctrl Pts',(54.7136848454783,23.8861376427066,22.0566046154667));
#41377=CARTESIAN_POINT('Ctrl Pts',(52.4197187365831,22.3243547342073,22.1836379101757));
#41378=CARTESIAN_POINT('Ctrl Pts',(52.488145461331,19.5500504709044,22.3106712048847));
#41379=CARTESIAN_POINT('Ctrl Pts',(54.8563164990095,18.1032566713808,22.4377044995937));
#41380=CARTESIAN_POINT('Ctrl Pts',(57.3560378749654,19.3085945512426,22.5647377943026));
#41381=CARTESIAN_POINT('Ctrl Pts',(57.6986738701439,22.0625093895861,22.6917710890117));
#41382=CARTESIAN_POINT('Ctrl Pts',(55.5705219316369,23.8436370348337,22.8188043837206));
#41383=CARTESIAN_POINT('Ctrl Pts',(52.9200250294827,23.0212548039235,22.9458376784296));
#41384=CARTESIAN_POINT('Ctrl Pts',(52.1738623695604,20.3482999507729,23.0728709731386));
#41385=CARTESIAN_POINT('Ctrl Pts',(54.0151878953965,18.2720132003655,23.1999042678476));
#41386=CARTESIAN_POINT('Ctrl Pts',(56.7581643735579,18.6933520216677,23.3269375625566));
#41387=CARTESIAN_POINT('Ctrl Pts',(57.8914423372978,21.2265569914547,23.4539708572655));
#41388=CARTESIAN_POINT('Ctrl Pts',(56.3774419778305,23.552336274487,23.5810041519745));
#41389=CARTESIAN_POINT('Ctrl Pts',(53.6023159017516,23.5413079353176,23.7080374466835));
#41390=CARTESIAN_POINT('Ctrl Pts',(52.1068483437591,21.2035690395033,23.8350707413925));
#41391=CARTESIAN_POINT('Ctrl Pts',(53.2602240864888,18.679451221964,23.9621040361015));
#41392=CARTESIAN_POINT('Ctrl Pts',(56.0064626732777,18.2799265176612,24.0891373308104));
#41393=CARTESIAN_POINT('Ctrl Pts',(57.8312279915067,20.3707822980329,24.2161706255194));
#41394=CARTESIAN_POINT('Ctrl Pts',(57.0638446139116,23.0377223245789,24.3432039202284));
#41395=CARTESIAN_POINT('Ctrl Pts',(54.4068952397841,23.8390127887343,24.4702372149373));
#41396=CARTESIAN_POINT('Ctrl Pts',(52.2929666893451,22.0410271294973,24.5972705096464));
#41397=CARTESIAN_POINT('Ctrl Pts',(52.6574795946538,19.2899225060713,24.7243038043553));
#41398=CARTESIAN_POINT('Ctrl Pts',(55.1667019083449,18.1044901310662,24.8513370990643));
#41399=CARTESIAN_POINT('Ctrl Pts',(57.5232991718713,19.5700601710561,24.9783703937733));
#41400=CARTESIAN_POINT('Ctrl Pts',(57.569674040172,22.3448205940707,25.1054036884823));
#41401=CARTESIAN_POINT('Ctrl Pts',(55.2633673425956,23.8883221579753,25.2324369831912));
#41402=CARTESIAN_POINT('Ctrl Pts',(52.7159334828604,22.7874018185658,25.3594702779003));
#41403=CARTESIAN_POINT('Ctrl Pts',(52.2596902440975,20.0500149846021,25.4865035726092));
#41404=CARTESIAN_POINT('Ctrl Pts',(54.3123567522736,18.1823918701799,25.6135368673182));
#41405=CARTESIAN_POINT('Ctrl Pts',(56.9945958369287,18.8944497977569,25.7405701620272));
#41406=CARTESIAN_POINT('Ctrl Pts',(57.8506770262465,21.534253436458,25.8676034567362));
#41407=CARTESIAN_POINT('Ctrl Pts',(56.0967892557872,23.6849259730726,25.9946367514452));
#41408=CARTESIAN_POINT('Ctrl Pts',(53.33875569315,23.3773818818673,26.1216700461541));
#41409=CARTESIAN_POINT('Ctrl Pts',(52.1016329408265,20.8932414126525,26.2487033408631));
#41410=CARTESIAN_POINT('Ctrl Pts',(53.5182300352158,18.5067845124918,26.3757366355721));
#41411=CARTESIAN_POINT('Ctrl Pts',(56.2912723853565,18.4031240357596,26.5027699302811));
#41412=CARTESIAN_POINT('Ctrl Pts',(57.8824705783081,20.6768205233068,26.62980322499));
#41413=CARTESIAN_POINT('Ctrl Pts',(56.8338447602333,23.2468545512428,26.7568365196991));
#41414=CARTESIAN_POINT('Ctrl Pts',(54.1077183032358,23.7588877147861,26.883869814408));
#41415=CARTESIAN_POINT('Ctrl Pts',(52.1956009279497,21.7467417024125,27.010903109117));
#41416=CARTESIAN_POINT('Ctrl Pts',(52.8570509743138,19.046936199282,27.1379540096957));
#41417=CARTESIAN_POINT('Ctrl Pts',(54.5977264306064,18.4455186482959,27.2226604787048));
#41418=CARTESIAN_POINT('Ctrl Pts',(55.4030101405564,18.5796318107295,27.2650225161442));
#41419=CARTESIAN_POINT('Ctrl Pts',(52.682543123578,21.7964570772642,27.));
#41420=CARTESIAN_POINT('Ctrl Pts',(52.6775614025261,21.7814932791564,27.));
#41421=CARTESIAN_POINT('Ctrl Pts',(52.6725796814742,21.7665294810485,27.));
#41422=CARTESIAN_POINT('Ctrl Pts',(52.6675979604224,21.7515656829407,27.));
#41423=CARTESIAN_POINT('',(53.8384922642054,19.3763282842596,7.69906393853165));
#41424=CARTESIAN_POINT('Ctrl Pts',(53.8371246242104,19.3752411305972,7.7));
#41425=CARTESIAN_POINT('Ctrl Pts',(53.7954009457829,19.3983180443861,7.69999999999996));
#41426=CARTESIAN_POINT('Ctrl Pts',(53.7546382435995,19.4229469258337,7.7));
#41427=CARTESIAN_POINT('Ctrl Pts',(53.714934131533,19.4491088737553,7.7));
#41428=CARTESIAN_POINT('Ctrl Pts',(53.6548222073576,19.4887179960324,7.69999999999998));
#41429=CARTESIAN_POINT('Ctrl Pts',(53.5971353757259,19.5318385392025,7.69999999999999));
#41430=CARTESIAN_POINT('Ctrl Pts',(53.5419564862638,19.5781218769382,7.69999999999999));
#41431=CARTESIAN_POINT('Ctrl Pts',(53.5118285687018,19.6033927839351,7.7));
#41432=CARTESIAN_POINT('Ctrl Pts',(53.4824486254372,19.6296074937631,7.7));
#41433=CARTESIAN_POINT('Ctrl Pts',(53.4538328165778,19.6567151749008,7.7));
#41434=CARTESIAN_POINT('Ctrl Pts',(53.441927541973,19.6679930104997,7.7));
#41435=CARTESIAN_POINT('Ctrl Pts',(53.4301545553945,19.679425454428,7.70000000000001));
#41436=CARTESIAN_POINT('Ctrl Pts',(53.4185151361639,19.6910090336056,7.7));
#41437=CARTESIAN_POINT('Ctrl Pts',(53.4070875682394,19.7023817778327,7.7));
#41438=CARTESIAN_POINT('Ctrl Pts',(53.3957949213602,19.7138941297562,7.69999999999996));
#41439=CARTESIAN_POINT('Ctrl Pts',(53.3846420678092,19.7255380469733,7.69999999999997));
#41440=CARTESIAN_POINT('Ctrl Pts',(53.3326376402129,19.77983224595,7.69999999999998));
#41441=CARTESIAN_POINT('Ctrl Pts',(53.2836425471235,19.8370110695029,7.69999999999998));
#41442=CARTESIAN_POINT('Ctrl Pts',(53.2377500175545,19.8967020336691,7.69999999999999));
#41443=CARTESIAN_POINT('Ctrl Pts',(53.1912145152524,19.9572292921675,7.7));
#41444=CARTESIAN_POINT('Ctrl Pts',(53.1478684980368,20.02034026621,7.7));
#41445=CARTESIAN_POINT('Ctrl Pts',(53.1078385251695,20.0856923523535,7.7));
#41446=CARTESIAN_POINT('Ctrl Pts',(53.1023914173776,20.0945851852022,7.7));
#41447=CARTESIAN_POINT('Ctrl Pts',(53.0970057638649,20.1035195747242,7.7));
#41448=CARTESIAN_POINT('Ctrl Pts',(53.0916819349052,20.1124947106681,7.69999999999999));
#41449=CARTESIAN_POINT('Ctrl Pts',(53.0841510691443,20.1251905625617,7.69999999999999));
#41450=CARTESIAN_POINT('Ctrl Pts',(53.0767434016693,20.1379690332957,7.69999999999999));
#41451=CARTESIAN_POINT('Ctrl Pts',(53.0694684776847,20.1508123778746,7.69999999999999));
#41452=CARTESIAN_POINT('Ctrl Pts',(53.0310782388569,20.2185875280722,7.69999999999999));
#41453=CARTESIAN_POINT('Ctrl Pts',(52.9963246122019,20.2882608100817,7.69999999999999));
#41454=CARTESIAN_POINT('Ctrl Pts',(52.9653032278674,20.3594518913737,7.7));
#41455=CARTESIAN_POINT('Ctrl Pts',(52.9337377497509,20.431891615352,7.70000000000001));
#41456=CARTESIAN_POINT('Ctrl Pts',(52.9060359082978,20.5059036185587,7.70000000000002));
#41457=CARTESIAN_POINT('Ctrl Pts',(52.8823336043208,20.5811279320593,7.7));
#41458=CARTESIAN_POINT('Ctrl Pts',(52.8649251749872,20.6363772929238,7.69999999999999));
#41459=CARTESIAN_POINT('Ctrl Pts',(52.8496749210952,20.6922815309851,7.7));
#41460=CARTESIAN_POINT('Ctrl Pts',(52.8366516865568,20.7487078095979,7.70000000000001));
#41461=CARTESIAN_POINT('Ctrl Pts',(52.8268614045027,20.7911265482954,7.70000000000001));
#41462=CARTESIAN_POINT('Ctrl Pts',(52.8183299413487,20.8338404939063,7.70000000000001));
#41463=CARTESIAN_POINT('Ctrl Pts',(52.8110920343712,20.8767951347477,7.70000000000003));
#41464=CARTESIAN_POINT('Ctrl Pts',(52.8089129591374,20.8897272426518,7.70000000000003));
#41465=CARTESIAN_POINT('Ctrl Pts',(52.8068508399361,20.9026833709167,7.69999999999999));
#41466=CARTESIAN_POINT('Ctrl Pts',(52.8049077631042,20.9156550025417,7.69999999999999));
#41467=CARTESIAN_POINT('Ctrl Pts',(52.7928947628234,20.9958516328525,7.69999999999999));
#41468=CARTESIAN_POINT('Ctrl Pts',(52.7854650253443,21.0763836557487,7.69999999999999));
#41469=CARTESIAN_POINT('Ctrl Pts',(52.782744337916,21.1568724422313,7.69999999999999));
#41470=CARTESIAN_POINT('Ctrl Pts',(52.7815199940722,21.1930934168272,7.69999999999998));
#41471=CARTESIAN_POINT('Ctrl Pts',(52.7812498521346,21.2293060564157,7.69999999999999));
#41472=CARTESIAN_POINT('Ctrl Pts',(52.7819483744862,21.2654775510389,7.7));
#41473=CARTESIAN_POINT('Ctrl Pts',(52.7834470595638,21.3430837709493,7.70000000000002));
#41474=CARTESIAN_POINT('Ctrl Pts',(52.7894010863567,21.4205001805428,7.7));
#41475=CARTESIAN_POINT('Ctrl Pts',(52.7995773579842,21.4974758085045,7.7));
#41476=CARTESIAN_POINT('Ctrl Pts',(52.8099658437043,21.5760566720218,7.70000000000001));
#41477=CARTESIAN_POINT('Ctrl Pts',(52.8247546273921,21.6541789515393,7.70000000000002));
#41478=CARTESIAN_POINT('Ctrl Pts',(52.8437496449139,21.731577817109,7.70000000000001));
#41479=CARTESIAN_POINT('Ctrl Pts',(52.8469471737087,21.7446067654141,7.70000000000001));
#41480=CARTESIAN_POINT('Ctrl Pts',(52.8502645099437,21.7576170775422,7.70000000000002));
#41481=CARTESIAN_POINT('Ctrl Pts',(52.8536992928806,21.7706015318293,7.70000000000002));
#41482=CARTESIAN_POINT('Ctrl Pts',(52.8742497443937,21.8482880707327,7.69999999999999));
#41483=CARTESIAN_POINT('Ctrl Pts',(52.8989295562313,21.9247867684672,7.69999999999999));
#41484=CARTESIAN_POINT('Ctrl Pts',(52.9274637506463,21.9998324308231,7.7));
#41485=CARTESIAN_POINT('Ctrl Pts',(52.9569490877993,22.0773796229483,7.70000000000001));
#41486=CARTESIAN_POINT('Ctrl Pts',(52.9905501152123,22.1533761176763,7.70000000000002));
#41487=CARTESIAN_POINT('Ctrl Pts',(53.0280202297069,22.2275323910215,7.70000000000002));
#41488=CARTESIAN_POINT('Ctrl Pts',(53.0654903442015,22.3016886643666,7.70000000000002));
#41489=CARTESIAN_POINT('Ctrl Pts',(53.106829935963,22.3740056157837,7.70000000000001));
#41490=CARTESIAN_POINT('Ctrl Pts',(53.1518443452297,22.4441836503775,7.7));
#41491=CARTESIAN_POINT('Ctrl Pts',(53.1793250417929,22.4870264046308,7.69999999999999));
#41492=CARTESIAN_POINT('Ctrl Pts',(53.2081763082173,22.5290717465152,7.70000000000003));
#41493=CARTESIAN_POINT('Ctrl Pts',(53.238362420557,22.5702474500133,7.70000000000002));
#41494=CARTESIAN_POINT('Ctrl Pts',(53.2465684646758,22.5814409960959,7.70000000000001));
#41495=CARTESIAN_POINT('Ctrl Pts',(53.2548687740561,22.5925641633568,7.70000000000003));
#41496=CARTESIAN_POINT('Ctrl Pts',(53.2632582755064,22.6036104304445,7.70000000000003));
#41497=CARTESIAN_POINT('Ctrl Pts',(53.3152020503275,22.6720036256326,7.70000000000003));
#41498=CARTESIAN_POINT('Ctrl Pts',(53.3706073701717,22.7375134092656,7.70000000000001));
#41499=CARTESIAN_POINT('Ctrl Pts',(53.4292194516112,22.7998424876121,7.70000000000002));
#41500=CARTESIAN_POINT('Ctrl Pts',(53.487892423166,22.8622363175366,7.70000000000003));
#41501=CARTESIAN_POINT('Ctrl Pts',(53.5497792603426,22.9214437654044,7.69999999999998));
#41502=CARTESIAN_POINT('Ctrl Pts',(53.6146732957803,22.9771486789419,7.70000000000001));
#41503=CARTESIAN_POINT('Ctrl Pts',(53.6781671893094,23.0316517133942,7.70000000000003));
#41504=CARTESIAN_POINT('Ctrl Pts',(53.7445404747154,23.0828025035925,7.7));
#41505=CARTESIAN_POINT('Ctrl Pts',(53.8136387438114,23.1302752460601,7.7));
#41506=CARTESIAN_POINT('Ctrl Pts',(53.8499814999668,23.155243893265,7.7));
#41507=CARTESIAN_POINT('Ctrl Pts',(53.8870786806954,23.1791945082043,7.7));
#41508=CARTESIAN_POINT('Ctrl Pts',(53.9249115396487,23.2020751695661,7.7));
#41509=CARTESIAN_POINT('Ctrl Pts',(53.8394226943829,19.3776289326463,7.69906393853165));
#41510=CARTESIAN_POINT('Ctrl Pts',(53.8468827378282,19.3722923254447,7.6993759590211));
#41511=CARTESIAN_POINT('Ctrl Pts',(53.8543795903139,19.3670071736118,7.69968797951055));
#41512=CARTESIAN_POINT('Ctrl Pts',(53.8619125385576,19.3617739799992,7.7));
#41513=CARTESIAN_POINT('Origin',(55.,21.,7.7));
#41514=CARTESIAN_POINT('',(56.1178200348344,23.1806945269163,7.7));
#41515=CARTESIAN_POINT('',(57.4505,21.,7.7));
#41516=CARTESIAN_POINT('Origin',(55.,21.,7.7));
#41517=CARTESIAN_POINT('Ctrl Pts',(56.1178200348344,23.1806945269163,7.70000000000001));
#41518=CARTESIAN_POINT('Ctrl Pts',(56.1536233275691,23.1582395113502,7.7));
#41519=CARTESIAN_POINT('Ctrl Pts',(56.188767358605,23.1348032560045,7.69999999999999));
#41520=CARTESIAN_POINT('Ctrl Pts',(56.2232064725664,23.1103828446799,7.7));
#41521=CARTESIAN_POINT('Ctrl Pts',(56.2929518967896,23.0609271023095,7.7));
#41522=CARTESIAN_POINT('Ctrl Pts',(56.3598088918619,23.0074368937122,7.70000000000002));
#41523=CARTESIAN_POINT('Ctrl Pts',(56.4236072141696,22.9502772007722,7.70000000000002));
#41524=CARTESIAN_POINT('Ctrl Pts',(56.4555381659656,22.9216688716826,7.70000000000002));
#41525=CARTESIAN_POINT('Ctrl Pts',(56.4867022725918,22.8921408163768,7.70000000000001));
#41526=CARTESIAN_POINT('Ctrl Pts',(56.5170740148072,22.861736276879,7.70000000000001));
#41527=CARTESIAN_POINT('Ctrl Pts',(56.5334666656307,22.845325924259,7.70000000000001));
#41528=CARTESIAN_POINT('Ctrl Pts',(56.5496284408635,22.8286602173332,7.7));
#41529=CARTESIAN_POINT('Ctrl Pts',(56.5655549643951,22.8117458184104,7.7));
#41530=CARTESIAN_POINT('Ctrl Pts',(56.5758872739768,22.800772626068,7.69999999999999));
#41531=CARTESIAN_POINT('Ctrl Pts',(56.5861181057108,22.7896973004763,7.70000000000001));
#41532=CARTESIAN_POINT('Ctrl Pts',(56.5962408500655,22.7785280899325,7.70000000000001));
#41533=CARTESIAN_POINT('Ctrl Pts',(56.6532768133754,22.7155958790167,7.70000000000001));
#41534=CARTESIAN_POINT('Ctrl Pts',(56.70693971914,22.6496274807739,7.7));
#41535=CARTESIAN_POINT('Ctrl Pts',(56.7570610656381,22.5809809569958,7.69999999999999));
#41536=CARTESIAN_POINT('Ctrl Pts',(56.7959095405622,22.5277738318097,7.69999999999999));
#41537=CARTESIAN_POINT('Ctrl Pts',(56.8326295718789,22.4729569792761,7.70000000000001));
#41538=CARTESIAN_POINT('Ctrl Pts',(56.8671226775623,22.4166891996158,7.70000000000001));
#41539=CARTESIAN_POINT('Ctrl Pts',(56.8834054025986,22.39012757907,7.70000000000001));
#41540=CARTESIAN_POINT('Ctrl Pts',(56.899191619411,22.3632425685576,7.70000000000001));
#41541=CARTESIAN_POINT('Ctrl Pts',(56.9144695005957,22.3360506410446,7.7));
#41542=CARTESIAN_POINT('Ctrl Pts',(56.9213021800373,22.3238896795965,7.7));
#41543=CARTESIAN_POINT('Ctrl Pts',(56.9280331733587,22.3116673301508,7.70000000000001));
#41544=CARTESIAN_POINT('Ctrl Pts',(56.9346613588346,22.299385064033,7.70000000000001));
#41545=CARTESIAN_POINT('Ctrl Pts',(56.9413081562691,22.2870683092863,7.7));
#41546=CARTESIAN_POINT('Ctrl Pts',(56.9478467935192,22.2747001384903,7.7));
#41547=CARTESIAN_POINT('Ctrl Pts',(56.9542762249967,22.2622829412227,7.7));
#41548=CARTESIAN_POINT('Ctrl Pts',(56.9924776523494,22.1885043091617,7.70000000000001));
#41549=CARTESIAN_POINT('Ctrl Pts',(57.0268325187052,22.1129874340337,7.70000000000002));
#41550=CARTESIAN_POINT('Ctrl Pts',(57.0571793379516,22.0360626483818,7.70000000000002));
#41551=CARTESIAN_POINT('Ctrl Pts',(57.0868760352299,21.9607858276332,7.70000000000002));
#41552=CARTESIAN_POINT('Ctrl Pts',(57.1127347053609,21.8841598409799,7.70000000000001));
#41553=CARTESIAN_POINT('Ctrl Pts',(57.1345559806643,21.8064859127151,7.7));
#41554=CARTESIAN_POINT('Ctrl Pts',(57.1559121045188,21.730467714456,7.69999999999999));
#41555=CARTESIAN_POINT('Ctrl Pts',(57.1734012228511,21.6534450032609,7.70000000000001));
#41556=CARTESIAN_POINT('Ctrl Pts',(57.1867882744522,21.5757044772605,7.70000000000002));
#41557=CARTESIAN_POINT('Ctrl Pts',(57.1927334778934,21.5411798293788,7.70000000000003));
#41558=CARTESIAN_POINT('Ctrl Pts',(57.1978689951837,21.5065137364553,7.7));
#41559=CARTESIAN_POINT('Ctrl Pts',(57.2021710133261,21.4717321844435,7.7));
#41560=CARTESIAN_POINT('Ctrl Pts',(57.2038280264685,21.4583353351305,7.7));
#41561=CARTESIAN_POINT('Ctrl Pts',(57.20536138141,21.4449203597091,7.7));
#41562=CARTESIAN_POINT('Ctrl Pts',(57.2067681334423,21.4315055814218,7.7));
#41563=CARTESIAN_POINT('Ctrl Pts',(57.2149185872068,21.3537829070064,7.69999999999999));
#41564=CARTESIAN_POINT('Ctrl Pts',(57.2188406380943,21.2759353641072,7.7));
#41565=CARTESIAN_POINT('Ctrl Pts',(57.218357164912,21.1982424679639,7.69999999999999));
#41566=CARTESIAN_POINT('Ctrl Pts',(57.2181643246661,21.1672535367307,7.69999999999999));
#41567=CARTESIAN_POINT('Ctrl Pts',(57.2172700275202,21.1362892430631,7.69999999999999));
#41568=CARTESIAN_POINT('Ctrl Pts',(57.2156607144632,21.1053676362415,7.7));
#41569=CARTESIAN_POINT('Ctrl Pts',(57.2115281138556,21.0259631657548,7.70000000000001));
#41570=CARTESIAN_POINT('Ctrl Pts',(57.2026838747762,20.9468386113069,7.70000000000001));
#41571=CARTESIAN_POINT('Ctrl Pts',(57.1893169135748,20.8683173591924,7.70000000000001));
#41572=CARTESIAN_POINT('Ctrl Pts',(57.1763427050985,20.7921032459471,7.70000000000002));
#41573=CARTESIAN_POINT('Ctrl Pts',(57.1591068601941,20.7164568346722,7.70000000000001));
#41574=CARTESIAN_POINT('Ctrl Pts',(57.1377429730716,20.64169976062,7.7));
#41575=CARTESIAN_POINT('Ctrl Pts',(57.1328095664832,20.6244366549156,7.7));
#41576=CARTESIAN_POINT('Ctrl Pts',(57.1276540190574,20.6072155631192,7.70000000000002));
#41577=CARTESIAN_POINT('Ctrl Pts',(57.1222879460442,20.59007204879,7.70000000000002));
#41578=CARTESIAN_POINT('Ctrl Pts',(57.0990729898313,20.5159049747478,7.7));
#41579=CARTESIAN_POINT('Ctrl Pts',(57.0718976926733,20.4430944616305,7.70000000000001));
#41580=CARTESIAN_POINT('Ctrl Pts',(57.0409657230395,20.3719309959309,7.70000000000001));
#41581=CARTESIAN_POINT('Ctrl Pts',(57.0101386747369,20.3010089169146,7.70000000000001));
#41582=CARTESIAN_POINT('Ctrl Pts',(56.9755797145763,20.2317219276503,7.69999999999998));
#41583=CARTESIAN_POINT('Ctrl Pts',(56.9374482924625,20.1643863607663,7.69999999999998));
#41584=CARTESIAN_POINT('Ctrl Pts',(56.8996354441195,20.0976133573605,7.69999999999998));
#41585=CARTESIAN_POINT('Ctrl Pts',(56.8583089214272,20.0327585902461,7.69999999999998));
#41586=CARTESIAN_POINT('Ctrl Pts',(56.813592673895,19.9701701334681,7.70000000000001));
#41587=CARTESIAN_POINT('Ctrl Pts',(56.7965173240937,19.9462701004379,7.70000000000002));
#41588=CARTESIAN_POINT('Ctrl Pts',(56.7789474160572,19.9227010037022,7.70000000000001));
#41589=CARTESIAN_POINT('Ctrl Pts',(56.7608889259661,19.8994840987326,7.7));
#41590=CARTESIAN_POINT('Ctrl Pts',(56.7532705735319,19.8896895608949,7.7));
#41591=CARTESIAN_POINT('Ctrl Pts',(56.7455650804365,19.8799576251608,7.69999999999999));
#41592=CARTESIAN_POINT('Ctrl Pts',(56.7377822767593,19.8703012259636,7.69999999999999));
#41593=CARTESIAN_POINT('Ctrl Pts',(56.6906318007196,19.8117999662811,7.7));
#41594=CARTESIAN_POINT('Ctrl Pts',(56.6405649027111,19.755961680436,7.69999999999998));
#41595=CARTESIAN_POINT('Ctrl Pts',(56.5877351390234,19.7030735504476,7.69999999999999));
#41596=CARTESIAN_POINT('Ctrl Pts',(56.5363803686456,19.6516620433412,7.7));
#41597=CARTESIAN_POINT('Ctrl Pts',(56.482414165105,19.6030378011168,7.7));
#41598=CARTESIAN_POINT('Ctrl Pts',(56.4259516963983,19.5575050942091,7.7));
#41599=CARTESIAN_POINT('Ctrl Pts',(56.3702806307515,19.5126105939615,7.7));
#41600=CARTESIAN_POINT('Ctrl Pts',(56.3121822465846,19.470721107261,7.69999999999999));
#41601=CARTESIAN_POINT('Ctrl Pts',(56.2517503094704,19.4321750581638,7.69999999999998));
#41602=CARTESIAN_POINT('Ctrl Pts',(56.2218511525908,19.4131041095217,7.69999999999997));
#41603=CARTESIAN_POINT('Ctrl Pts',(56.1913805690498,19.394852353254,7.69999999999999));
#41604=CARTESIAN_POINT('Ctrl Pts',(56.1603489846691,19.3774656255483,7.7));
#41605=CARTESIAN_POINT('Origin',(55.,21.,7.7));
#41606=CARTESIAN_POINT('Ctrl Pts',(56.4264070134832,19.0036827380914,7.43505745955369));
#41607=CARTESIAN_POINT('Ctrl Pts',(57.0906234180576,19.4782451892435,7.47741949721597));
#41608=CARTESIAN_POINT('Ctrl Pts',(57.8961547049334,21.13426194966,7.56212596644791));
#41609=CARTESIAN_POINT('Ctrl Pts',(56.4549014799736,23.5108937710809,7.68917686724951));
#41610=CARTESIAN_POINT('Ctrl Pts',(53.6801846690842,23.5816210589062,7.8162101619585));
#41611=CARTESIAN_POINT('Ctrl Pts',(52.1146727379514,21.2920254590205,7.94324345666747));
#41612=CARTESIAN_POINT('Ctrl Pts',(53.190410041307,18.7333910992113,8.07027675137646));
#41613=CARTESIAN_POINT('Ctrl Pts',(55.923149040188,18.2508190898123,8.19731004608543));
#41614=CARTESIAN_POINT('Ctrl Pts',(57.8105805181925,20.2848403969102,8.32434334079443));
#41615=CARTESIAN_POINT('Ctrl Pts',(57.1248247841991,22.9738538538107,8.45137663550339));
#41616=CARTESIAN_POINT('Ctrl Pts',(54.4936428464113,23.8555787817053,8.57840993021239));
#41617=CARTESIAN_POINT('Ctrl Pts',(52.3260744517511,22.122918854144,8.70544322492136));
#41618=CARTESIAN_POINT('Ctrl Pts',(52.6066278141553,19.3621336254897,8.83247651963035));
#41619=CARTESIAN_POINT('Ctrl Pts',(55.0784521557293,18.1009225745723,8.95950981433934));
#41620=CARTESIAN_POINT('Ctrl Pts',(57.478447118452,19.4939723991015,9.0865431090483));
#41621=CARTESIAN_POINT('Ctrl Pts',(57.6092851715724,22.2658793094417,9.2135764037573));
#41622=CARTESIAN_POINT('Ctrl Pts',(55.3511751536352,23.878800370662,9.34060969846627));
#41623=CARTESIAN_POINT('Ctrl Pts',(52.7715447710963,22.8560185838881,9.46764299317526));
#41624=CARTESIAN_POINT('Ctrl Pts',(52.2321905331791,20.1339467082752,9.59467628788425));
#41625=CARTESIAN_POINT('Ctrl Pts',(54.2269218321233,18.2047956751683,9.72170958259321));
#41626=CARTESIAN_POINT('Ctrl Pts',(56.9294497022423,18.8348115048152,9.84874287730221));
#41627=CARTESIAN_POINT('Ctrl Pts',(57.8654577101017,21.4471794295255,9.97577617201117));
#41628=CARTESIAN_POINT('Ctrl Pts',(56.1779777751286,23.6501293622297,10.1028094667202));
#41629=CARTESIAN_POINT('Ctrl Pts',(53.4119928410238,23.4267366111919,10.2298427614291));
#41630=CARTESIAN_POINT('Ctrl Pts',(52.0999179046356,20.9815297946576,10.3568760561381));
#41631=CARTESIAN_POINT('Ctrl Pts',(53.4430314779032,18.5532334963378,10.4839093508471));
#41632=CARTESIAN_POINT('Ctrl Pts',(56.211637430355,18.3650897462597,10.6109426455561));
#41633=CARTESIAN_POINT('Ctrl Pts',(57.8709210689259,20.5893547487726,10.737975940265));
#41634=CARTESIAN_POINT('Ctrl Pts',(56.9017147611579,23.1895886081475,10.865009234974));
#41635=CARTESIAN_POINT('Ctrl Pts',(54.1913814736041,23.7851307662754,10.992042529683));
#41636=CARTESIAN_POINT('Ctrl Pts',(52.2213839931885,21.8307288323652,11.119075824392));
#41637=CARTESIAN_POINT('Ctrl Pts',(52.7953659754236,19.1157478608594,11.246109119101));
#41638=CARTESIAN_POINT('Ctrl Pts',(55.3878145854162,18.1259058551238,11.37314241381));
#41639=CARTESIAN_POINT('Ctrl Pts',(57.6251970984125,19.7674589253413,11.5001757085189));
#41640=CARTESIAN_POINT('Ctrl Pts',(57.4590638008941,22.5374727735356,11.6272090032279));
#41641=CARTESIAN_POINT('Ctrl Pts',(55.0415190843716,23.8998436978354,11.7542422979369));
#41642=CARTESIAN_POINT('Ctrl Pts',(52.5859613075013,22.6072443800978,11.8812755926459));
#41643=CARTESIAN_POINT('Ctrl Pts',(52.3405919268156,19.8431223026964,12.0083088873549));
#41644=CARTESIAN_POINT('Ctrl Pts',(54.5300604310133,18.1381869194969,12.1353421820638));
#41645=CARTESIAN_POINT('Ctrl Pts',(57.149785080446,19.0534026060509,12.2623754767728));
#41646=CARTESIAN_POINT('Ctrl Pts',(57.801260399884,21.750837850857,12.3894087714818));
#41647=CARTESIAN_POINT('Ctrl Pts',(55.8880240393673,23.7608387514926,12.5164420661908));
#41648=CARTESIAN_POINT('Ctrl Pts',(53.1617516519464,23.2431362680666,12.6434753608998));
#41649=CARTESIAN_POINT('Ctrl Pts',(52.1184991683894,20.671716184278,12.7705086556088));
#41650=CARTESIAN_POINT('Ctrl Pts',(53.7134229996573,18.400858424705,12.8975419503177));
#41651=CARTESIAN_POINT('Ctrl Pts',(56.4862805425061,18.5096611766257,13.0245752450267));
#41652=CARTESIAN_POINT('Ctrl Pts',(57.8983645324169,20.8985093922302,13.1516085397357));
#41653=CARTESIAN_POINT('Ctrl Pts',(56.6568325395494,23.3802779758105,13.2786418344447));
#41654=CARTESIAN_POINT('Ctrl Pts',(53.8983770339348,23.6827680009414,13.4056751291537));
#41655=CARTESIAN_POINT('Ctrl Pts',(52.1485194037946,21.5290328115554,13.5327084238626));
#41656=CARTESIAN_POINT('Ctrl Pts',(53.0093528720454,18.8909382848755,13.6597417185716));
#41657=CARTESIAN_POINT('Ctrl Pts',(55.6927359111768,18.1838085534531,13.7867750132806));
#41658=CARTESIAN_POINT('Ctrl Pts',(57.7418802045661,20.0550607162118,13.9138083079896));
#41659=CARTESIAN_POINT('Ctrl Pts',(57.2806787314646,22.7914580179515,14.0408416026986));
#41660=CARTESIAN_POINT('Ctrl Pts',(54.7313874181419,23.887674598549,14.1678748974076));
#41661=CARTESIAN_POINT('Ctrl Pts',(52.4280260533891,22.3400624329458,14.2949081921165));
#41662=CARTESIAN_POINT('Ctrl Pts',(52.4794517058251,19.5655476295917,14.4219414868255));
#41663=CARTESIAN_POINT('Ctrl Pts',(54.8385812940423,18.1043547683453,14.5489747815345));
#41664=CARTESIAN_POINT('Ctrl Pts',(57.3454987996377,19.2942882168619,14.6760080762435));
#41665=CARTESIAN_POINT('Ctrl Pts',(57.7049800415428,22.0458968788046,14.8030413709524));
#41666=CARTESIAN_POINT('Ctrl Pts',(55.5878996946444,23.8399280369887,14.9300746656615));
#41667=CARTESIAN_POINT('Ctrl Pts',(52.9325640632467,23.0338451154545,15.0571079603704));
#41668=CARTESIAN_POINT('Ctrl Pts',(52.1700824823932,20.3656624323127,15.1841412550794));
#41669=CARTESIAN_POINT('Ctrl Pts',(53.9985497869111,18.2782515221016,15.3111745497884));
#41670=CARTESIAN_POINT('Ctrl Pts',(56.7439011692209,18.682754648677,15.4382078444974));
#41671=CARTESIAN_POINT('Ctrl Pts',(57.8926128040896,21.2088264156062,15.5652411392064));
#41672=CARTESIAN_POINT('Ctrl Pts',(56.3929744874356,23.5437058366862,15.6922744339153));
#41673=CARTESIAN_POINT('Ctrl Pts',(53.6179895668198,23.5496792874436,15.8193077286243));
#41674=CARTESIAN_POINT('Ctrl Pts',(52.1083130409334,21.2212777372493,15.9463410233333));
#41675=CARTESIAN_POINT('Ctrl Pts',(53.246138803302,18.6902839549081,16.0733743180423));
#41676=CARTESIAN_POINT('Ctrl Pts',(55.9897232792757,18.2739653089702,16.2004076127513));
#41677=CARTESIAN_POINT('Ctrl Pts',(57.8271603458951,20.353484969366,16.3274409074602));
#41678=CARTESIAN_POINT('Ctrl Pts',(57.0761728731458,23.0249255559283,16.4544742021693));
#41679=CARTESIAN_POINT('Ctrl Pts',(54.424332192468,23.8424327400326,16.5815074968782));
#41680=CARTESIAN_POINT('Ctrl Pts',(52.2995478146647,22.057532647702,16.7085407915872));
#41681=CARTESIAN_POINT('Ctrl Pts',(52.6471795182707,19.3044018497907,16.8355740862962));
#41682=CARTESIAN_POINT('Ctrl Pts',(55.1489508979232,18.1036866646984,16.9626073810052));
#41683=CARTESIAN_POINT('Ctrl Pts',(57.514349340715,19.5547094758896,17.0896406757141));
#41684=CARTESIAN_POINT('Ctrl Pts',(57.5777193387807,22.3289771693728,17.2166739704231));
#41685=CARTESIAN_POINT('Ctrl Pts',(55.2810420895108,23.8864914082951,17.3437072651321));
#41686=CARTESIAN_POINT('Ctrl Pts',(52.7270549773104,22.8012601783385,17.4707405598411));
#41687=CARTESIAN_POINT('Ctrl Pts',(52.2540770593384,20.0668737972888,17.59777385455));
#41688=CARTESIAN_POINT('Ctrl Pts',(54.2951462604641,18.1868170141102,17.7248071492591));
#41689=CARTESIAN_POINT('Ctrl Pts',(56.9815487617436,18.8823877099265,17.851840443968));
#41690=CARTESIAN_POINT('Ctrl Pts',(57.8537317588834,21.5167517339861,17.978873738677));
#41691=CARTESIAN_POINT('Ctrl Pts',(56.1131625914016,23.6780004390108,18.105907033386));
#41692=CARTESIAN_POINT('Ctrl Pts',(53.3534303714686,23.3873889010037,18.232940328095));
#41693=CARTESIAN_POINT('Ctrl Pts',(52.1012253911768,20.9109883520029,18.3599736228039));
#41694=CARTESIAN_POINT('Ctrl Pts',(53.5030118417111,18.5160829804156,18.487006917513));
#41695=CARTESIAN_POINT('Ctrl Pts',(56.2753752705501,18.3953435494279,18.6140402122219));
#41696=CARTESIAN_POINT('Ctrl Pts',(57.8800608023822,20.659313808881,18.7410735069309));
#41697=CARTESIAN_POINT('Ctrl Pts',(56.8478884472591,23.2352014658021,18.8681068016399));
#41698=CARTESIAN_POINT('Ctrl Pts',(54.123870134461,23.7646362807697,18.9951400963489));
#41699=CARTESIAN_POINT('Ctrl Pts',(52.2019980624758,21.7628908597228,19.1221733910578));
#41700=CARTESIAN_POINT('Ctrl Pts',(52.8418543646187,19.0626758859906,19.2492066857668));
#41701=CARTESIAN_POINT('Ctrl Pts',(55.4576145557163,18.1361902603989,19.3762399804758));
#41702=CARTESIAN_POINT('Ctrl Pts',(57.6544028454472,19.8316837584284,19.5032732751848));
#41703=CARTESIAN_POINT('Ctrl Pts',(57.4209358182124,22.5968365822257,19.6303065698938));
#41704=CARTESIAN_POINT('Ctrl Pts',(54.9709656877149,23.8999955715394,19.7573398646027));
#41705=CARTESIAN_POINT('Ctrl Pts',(52.5475781055017,22.5480452698882,19.8843731593118));
#41706=CARTESIAN_POINT('Ctrl Pts',(52.3695209028766,19.7787723284191,20.0114064540207));
#41707=CARTESIAN_POINT('Ctrl Pts',(54.5998154780972,18.1276021071817,20.1384397487297));
#41708=CARTESIAN_POINT('Ctrl Pts',(57.1965015239227,19.1062739475724,20.2654730434386));
#41709=CARTESIAN_POINT('Ctrl Pts',(57.7821667043993,21.81875865502,20.3925063381477));
#41710=CARTESIAN_POINT('Ctrl Pts',(55.8206015586093,23.7816236963769,20.5195396328566));
#41711=CARTESIAN_POINT('Ctrl Pts',(53.1077294646894,23.1977555658974,20.6465729275656));
#41712=CARTESIAN_POINT('Ctrl Pts',(52.1273376299221,20.6017184240057,20.7736062222746));
#41713=CARTESIAN_POINT('Ctrl Pts',(53.7770300006112,18.3703304985544,20.9006395169836));
#41714=CARTESIAN_POINT('Ctrl Pts',(56.5464202907784,18.5465531205044,21.0276728116926));
#41715=CARTESIAN_POINT('Ctrl Pts',(57.8999757010312,20.9690445535407,21.1547061064016));
#41716=CARTESIAN_POINT('Ctrl Pts',(56.5984400128888,23.4198774414078,21.2817394011105));
#41717=CARTESIAN_POINT('Ctrl Pts',(53.8334424591756,23.6551762295908,21.4087726958195));
#41718=CARTESIAN_POINT('Ctrl Pts',(52.1364940416356,21.4595116240631,21.5358059905285));
#41719=CARTESIAN_POINT('Ctrl Pts',(53.0612466188837,18.8431382442427,21.6628392852375));
#41720=CARTESIAN_POINT('Ctrl Pts',(55.7610371188136,18.2014932892656,21.7898725799465));
#41721=CARTESIAN_POINT('Ctrl Pts',(57.7640552702745,20.1220388567222,21.9169058746554));
#41722=CARTESIAN_POINT('Ctrl Pts',(57.2364251335552,22.8464073029103,22.0439391693644));
#41723=CARTESIAN_POINT('Ctrl Pts',(54.6612218181301,23.8802858625016,22.1709724640734));
#41724=CARTESIAN_POINT('Ctrl Pts',(52.3961890102348,22.2771004799217,22.2980057587824));
#41725=CARTESIAN_POINT('Ctrl Pts',(52.5150918257906,19.5046576739809,22.4250390534914));
#41726=CARTESIAN_POINT('Ctrl Pts',(54.9090680398321,18.1012849941988,22.5520723482003));
#41727=CARTESIAN_POINT('Ctrl Pts',(57.3862975852447,19.3518491753185,22.6791056429093));
#41728=CARTESIAN_POINT('Ctrl Pts',(57.6787372807074,22.1113882702183,22.8061389376183));
#41729=CARTESIAN_POINT('Ctrl Pts',(55.5186421130676,23.8533888036486,22.9331722323273));
#41730=CARTESIAN_POINT('Ctrl Pts',(52.883700877855,22.9829511672962,23.0602055270362));
#41731=CARTESIAN_POINT('Ctrl Pts',(52.1863506917035,20.2970100455204,23.1872388217453));
#41732=CARTESIAN_POINT('Ctrl Pts',(54.0650549289335,18.2546958237164,23.3142721164542));
#41733=CARTESIAN_POINT('Ctrl Pts',(56.7997540405474,18.725862207337,23.4413054111632));
#41734=CARTESIAN_POINT('Ctrl Pts',(57.8866769548865,21.2791298333439,23.5683387058722));
#41735=CARTESIAN_POINT('Ctrl Pts',(56.330684522312,23.5768383745275,23.6953720005812));
#41736=CARTESIAN_POINT('Ctrl Pts',(53.5563754567649,23.5153062410116,23.8224052952901));
#41737=CARTESIAN_POINT('Ctrl Pts',(52.1037859754078,21.1508695661785,23.9494385899992));
#41738=CARTESIAN_POINT('Ctrl Pts',(53.3028435633851,18.6483033065475,24.0764718847081));
#41739=CARTESIAN_POINT('Ctrl Pts',(56.0557434678534,18.298847829695,24.2035051794171));
#41740=CARTESIAN_POINT('Ctrl Pts',(57.8420507524862,20.4224493134434,24.3305384741261));
#41741=CARTESIAN_POINT('Ctrl Pts',(57.0263005097603,23.0748309749754,24.4575717688351));
#41742=CARTESIAN_POINT('Ctrl Pts',(54.3553579817675,23.8275880254189,24.5846050635441));
#41743=CARTESIAN_POINT('Ctrl Pts',(52.2746216002963,21.9915289454338,24.711638358253));
#41744=CARTESIAN_POINT('Ctrl Pts',(52.6891225191036,19.2476693185881,24.838671652962));
#41745=CARTESIAN_POINT('Ctrl Pts',(55.2193621970339,18.1081670315388,24.965704947671));
#41746=CARTESIAN_POINT('Ctrl Pts',(57.5487629137497,19.616300909826,25.09273824238));
#41747=CARTESIAN_POINT('Ctrl Pts',(57.5446286265918,22.3912888576387,25.2197715370889));
#41748=CARTESIAN_POINT('Ctrl Pts',(55.2107415367077,23.8924742450603,25.346804831798));
#41749=CARTESIAN_POINT('Ctrl Pts',(52.6839125453877,22.7454350638024,25.4738381265069));
#41750=CARTESIAN_POINT('Ctrl Pts',(52.2775845533845,20.0003546545124,25.6008714212159));
#41751=CARTESIAN_POINT('Ctrl Pts',(54.3637959560076,18.1705002200075,25.7279047159249));
#41752=CARTESIAN_POINT('Ctrl Pts',(57.0324592249323,18.9312232492356,25.8549380106339));
#41753=CARTESIAN_POINT('Ctrl Pts',(57.8403478634403,21.5860063262462,25.9819713053429));
#41754=CARTESIAN_POINT('Ctrl Pts',(56.0476279930325,23.704309837158,26.1090046000518));
#41755=CARTESIAN_POINT('Ctrl Pts',(53.2959609336026,23.3465827680974,26.2360378947608));
#41756=CARTESIAN_POINT('Ctrl Pts',(52.1040166225385,20.8405885662721,26.3630711894698));
#41757=CARTESIAN_POINT('Ctrl Pts',(53.5643317699236,18.480228381185,26.4901044841788));
#41758=CARTESIAN_POINT('Ctrl Pts',(56.337469579789,18.4274808217143,26.6171377788878));
#41759=CARTESIAN_POINT('Ctrl Pts',(57.8892510608654,20.7287913102977,26.7441710735968));
#41760=CARTESIAN_POINT('Ctrl Pts',(56.7893549764862,23.2809819920617,26.8712043683057));
#41761=CARTESIAN_POINT('Ctrl Pts',(54.9737389170402,23.5855482158792,26.9558932314451));
#41762=CARTESIAN_POINT('Ctrl Pts',(54.202107399834,23.3201911685949,26.9982376630147));
#41763=CARTESIAN_POINT('Ctrl Pts',(56.3368004103323,19.1290909890044,7.52404542325027));
#41764=CARTESIAN_POINT('Ctrl Pts',(56.9592908732868,19.5738415219392,7.56640746091254));
#41765=CARTESIAN_POINT('Ctrl Pts',(57.7142188459145,21.1258276408493,7.65111393014448));
#41766=CARTESIAN_POINT('Ctrl Pts',(56.3635048601399,23.3531599268327,7.77816483094608));
#41767=CARTESIAN_POINT('Ctrl Pts',(53.7630952040661,23.41944414059,7.90519812565507));
#41768=CARTESIAN_POINT('Ctrl Pts',(52.295928419175,21.2736804781216,8.03223142036406));
#41769=CARTESIAN_POINT('Ctrl Pts',(53.3040881203977,18.8757790167912,8.15926471507303));
#41770=CARTESIAN_POINT('Ctrl Pts',(55.8651570022134,18.4235220844559,8.28629800978201));
#41771=CARTESIAN_POINT('Ctrl Pts',(57.6340204124606,20.3297665800668,8.41333130449099));
#41772=CARTESIAN_POINT('Ctrl Pts',(56.9913437164512,22.8498567496991,8.54036459919998));
#41773=CARTESIAN_POINT('Ctrl Pts',(54.5254521014734,23.676191894064,8.66739789390895));
#41774=CARTESIAN_POINT('Ctrl Pts',(52.4940499196169,22.0523773164323,8.79443118861795));
#41775=CARTESIAN_POINT('Ctrl Pts',(52.7569789759361,19.4650240633855,8.92146448332691));
#41776=CARTESIAN_POINT('Ctrl Pts',(55.0735238070052,18.2830420383076,9.04849777803592));
#41777=CARTESIAN_POINT('Ctrl Pts',(57.3227515664291,19.588580751621,9.17553107274487));
#41778=CARTESIAN_POINT('Ctrl Pts',(57.4453703992343,22.1863570245358,9.30256436745386));
#41779=CARTESIAN_POINT('Ctrl Pts',(55.329114400757,23.6979547074494,9.42959766216286));
#41780=CARTESIAN_POINT('Ctrl Pts',(52.9115358826433,22.7394238678533,9.55663095687182));
#41781=CARTESIAN_POINT('Ctrl Pts',(52.4060637700227,20.1883520027568,9.68366425158081));
#41782=CARTESIAN_POINT('Ctrl Pts',(54.2754864479299,18.3803898515102,9.81069754628979));
#41783=CARTESIAN_POINT('Ctrl Pts',(56.8082420580466,18.9708282128101,9.93773084099876));
#41784=CARTESIAN_POINT('Ctrl Pts',(57.6854502301555,21.4190877072471,10.0647641357078));
#41785=CARTESIAN_POINT('Ctrl Pts',(56.1039774470183,23.4836487660078,10.1917974304167));
#41786=CARTESIAN_POINT('Ctrl Pts',(53.511751132977,23.2742895028874,10.3188307251257));
#41787=CARTESIAN_POINT('Ctrl Pts',(52.2821004815354,20.9826900892612,10.4458640198347));
#41788=CARTESIAN_POINT('Ctrl Pts',(53.5408399288986,18.7069388784791,10.5728973145437));
#41789=CARTESIAN_POINT('Ctrl Pts',(56.1355226094391,18.5306142811318,10.6999306092526));
#41790=CARTESIAN_POINT('Ctrl Pts',(57.6905703818716,20.6151514012811,10.8269639039617));
#41791=CARTESIAN_POINT('Ctrl Pts',(56.7822494204112,23.052039089939,10.9539971986706));
#41792=CARTESIAN_POINT('Ctrl Pts',(54.2421787276209,23.6101694088663,11.0810304933796));
#41793=CARTESIAN_POINT('Ctrl Pts',(52.3959360947117,21.7785426133519,11.2080637880886));
#41794=CARTESIAN_POINT('Ctrl Pts',(52.9338606436813,19.2341162031854,11.3350970827976));
#41795=CARTESIAN_POINT('Ctrl Pts',(55.3634521507654,18.3064558741743,11.4621303775066));
#41796=CARTESIAN_POINT('Ctrl Pts',(57.4602827420143,19.8448869090094,11.5891636722155));
#41797=CARTESIAN_POINT('Ctrl Pts',(57.3045859050014,22.4408890415635,11.7161969669245));
#41798=CARTESIAN_POINT('Ctrl Pts',(55.0389108637997,23.7176760970207,11.8432302616335));
#41799=CARTESIAN_POINT('Ctrl Pts',(52.7376107350945,22.5062776097633,11.9702635563425));
#41800=CARTESIAN_POINT('Ctrl Pts',(52.5076554098029,19.9157971281401,12.0972968510515));
#41801=CARTESIAN_POINT('Ctrl Pts',(54.5595819406981,18.3179654445409,12.2243301457604));
#41802=CARTESIAN_POINT('Ctrl Pts',(57.0147360118826,19.1756874648082,12.3513634404694));
#41803=CARTESIAN_POINT('Ctrl Pts',(57.6252857821193,21.7036703673151,12.4783967351784));
#41804=CARTESIAN_POINT('Ctrl Pts',(55.8322385469154,23.5874034135911,12.6054300298874));
#41805=CARTESIAN_POINT('Ctrl Pts',(53.2772300453221,23.1022228965773,12.7324633245964));
#41806=CARTESIAN_POINT('Ctrl Pts',(52.2995144740184,20.6923389078893,12.8594966193053));
#41807=CARTESIAN_POINT('Ctrl Pts',(53.7942455093638,18.5641359783547,12.9865299140143));
#41808=CARTESIAN_POINT('Ctrl Pts',(56.3929126962432,18.6661037631722,13.1135632087233));
#41809=CARTESIAN_POINT('Ctrl Pts',(57.7162898524779,20.9048850119012,13.2405965034323));
#41810=CARTESIAN_POINT('Ctrl Pts',(56.5527506509611,23.2307493896838,13.3676297981413));
#41811=CARTESIAN_POINT('Ctrl Pts',(53.9675807682189,23.5142370519669,13.4946630928503));
#41812=CARTESIAN_POINT('Ctrl Pts',(52.3276488442428,21.4957990761975,13.6216963875592));
#41813=CARTESIAN_POINT('Ctrl Pts',(53.1344049262782,19.0234291197785,13.7487296822682));
#41814=CARTESIAN_POINT('Ctrl Pts',(55.649218379859,18.3607211365814,13.8757629769772));
#41815=CARTESIAN_POINT('Ctrl Pts',(57.5696358387888,20.114421612929,14.0027962716862));
#41816=CARTESIAN_POINT('Ctrl Pts',(57.1374069499372,22.6789189837497,14.1298295663952));
#41817=CARTESIAN_POINT('Ctrl Pts',(54.7482616067825,23.7062714581164,14.2568628611041));
#41818=CARTESIAN_POINT('Ctrl Pts',(52.5895969420414,22.255879979066,14.3838961558131));
#41819=CARTESIAN_POINT('Ctrl Pts',(52.6377920452821,19.6556596404547,14.5109294505221));
#41820=CARTESIAN_POINT('Ctrl Pts',(54.8487215848493,18.2862586223546,14.6379627452311));
#41821=CARTESIAN_POINT('Ctrl Pts',(57.1981550343987,19.4014406897513,14.7649960399401));
#41822=CARTESIAN_POINT('Ctrl Pts',(57.5350537366225,21.9801938461708,14.8920293346491));
#41823=CARTESIAN_POINT('Ctrl Pts',(55.5509679534706,23.6615243259989,15.019062629358));
#41824=CARTESIAN_POINT('Ctrl Pts',(53.062439975082,22.9060793722914,15.146095924067));
#41825=CARTESIAN_POINT('Ctrl Pts',(52.3478573345588,20.4055113913785,15.273129218776));
#41826=CARTESIAN_POINT('Ctrl Pts',(54.0614606888986,18.4492312168382,15.400162513485));
#41827=CARTESIAN_POINT('Ctrl Pts',(56.6343496467399,18.8283235379467,15.527195808194));
#41828=CARTESIAN_POINT('Ctrl Pts',(57.7108994465729,21.1957079819658,15.654229102903));
#41829=CARTESIAN_POINT('Ctrl Pts',(56.305468108881,23.3839107450426,15.7812623976119));
#41830=CARTESIAN_POINT('Ctrl Pts',(53.7048071856801,23.3895089448189,15.9082956923209));
#41831=CARTESIAN_POINT('Ctrl Pts',(52.2899682370509,21.2073771140749,16.0353289870299));
#41832=CARTESIAN_POINT('Ctrl Pts',(53.3563160127161,18.835379854667,16.1623622817389));
#41833=CARTESIAN_POINT('Ctrl Pts',(55.9275490609236,18.4452142627581,16.2893955764478));
#41834=CARTESIAN_POINT('Ctrl Pts',(57.6495586987047,20.3940989142172,16.4164288711569));
#41835=CARTESIAN_POINT('Ctrl Pts',(56.9457481087146,22.8977201377096,16.5434621658658));
#41836=CARTESIAN_POINT('Ctrl Pts',(54.4604955289412,23.6638716840987,16.6704954605748));
#41837=CARTESIAN_POINT('Ctrl Pts',(52.4691896805641,21.9910986583945,16.7975287552838));
#41838=CARTESIAN_POINT('Ctrl Pts',(52.7949832301137,19.4109189862833,16.9245620499928));
#41839=CARTESIAN_POINT('Ctrl Pts',(55.1395938323219,18.2856324888452,17.0515953447017));
#41840=CARTESIAN_POINT('Ctrl Pts',(57.3563984182741,19.6455023373993,17.1786286394107));
#41841=CARTESIAN_POINT('Ctrl Pts',(57.4157875257419,22.2454910895324,17.3056619341197));
#41842=CARTESIAN_POINT('Ctrl Pts',(55.2633870816867,23.7051625956373,17.4326952288287));
#41843=CARTESIAN_POINT('Ctrl Pts',(52.8698409288001,22.6881053743827,17.5597285235377));
#41844=CARTESIAN_POINT('Ctrl Pts',(52.4265753889884,20.1254925986166,17.6867618182466));
#41845=CARTESIAN_POINT('Ctrl Pts',(54.3394250313344,18.363540606342,17.8137951129556));
#41846=CARTESIAN_POINT('Ctrl Pts',(56.8570682650556,19.0154156902367,17.9408284076646));
#41847=CARTESIAN_POINT('Ctrl Pts',(57.6744609008463,21.4842894934635,18.0678617023736));
#41848=CARTESIAN_POINT('Ctrl Pts',(56.043233940163,23.5097689873227,18.1948949970826));
#41849=CARTESIAN_POINT('Ctrl Pts',(53.4568675460404,23.2374136079795,18.3219282917916));
#41850=CARTESIAN_POINT('Ctrl Pts',(52.2833258320335,20.9165800459181,18.4489615865005));
#41851=CARTESIAN_POINT('Ctrl Pts',(53.5970523382548,18.6721221505331,18.5759948812095));
#41852=CARTESIAN_POINT('Ctrl Pts',(56.1952564512676,18.558967546439,18.7030281759185));
#41853=CARTESIAN_POINT('Ctrl Pts',(57.6991359591011,20.6807156472329,18.8300614706275));
#41854=CARTESIAN_POINT('Ctrl Pts',(56.7318044647805,23.0947865570032,18.9570947653365));
#41855=CARTESIAN_POINT('Ctrl Pts',(54.178908437293,23.590962382839,19.0841280600455));
#41856=CARTESIAN_POINT('Ctrl Pts',(52.3777679842871,21.7149662085759,19.2111613547544));
#41857=CARTESIAN_POINT('Ctrl Pts',(52.9774286415701,19.1843781991577,19.3381946494634));
#41858=CARTESIAN_POINT('Ctrl Pts',(55.4288673008988,18.316094215168,19.4652279441724));
#41859=CARTESIAN_POINT('Ctrl Pts',(57.4876537898647,19.905077150934,19.5922612388814));
#41860=CARTESIAN_POINT('Ctrl Pts',(57.268853114562,22.4965236276708,19.7192945335903));
#41861=CARTESIAN_POINT('Ctrl Pts',(54.9727896174025,23.7178184300489,19.8463278282993));
#41862=CARTESIAN_POINT('Ctrl Pts',(52.7016387581638,22.4507973758109,19.9733611230083));
#41863=CARTESIAN_POINT('Ctrl Pts',(52.5347670733767,19.8554896063698,20.1003944177173));
#41864=CARTESIAN_POINT('Ctrl Pts',(54.6249549896826,18.3080455680173,20.2274277124263));
#41865=CARTESIAN_POINT('Ctrl Pts',(57.0585177377285,19.2252374392353,20.3544610071353));
#41866=CARTESIAN_POINT('Ctrl Pts',(57.6073915487639,21.7673244001521,20.4814943018443));
#41867=CARTESIAN_POINT('Ctrl Pts',(55.7690515329069,23.6068826523971,20.6085275965532));
#41868=CARTESIAN_POINT('Ctrl Pts',(53.2266015210582,23.0596930010373,20.7355608912622));
#41869=CARTESIAN_POINT('Ctrl Pts',(52.3077977051663,20.6267383929101,20.8625941859712));
#41870=CARTESIAN_POINT('Ctrl Pts',(53.8538567312461,18.5355258104161,20.9896274806802));
#41871=CARTESIAN_POINT('Ctrl Pts',(56.4492744775635,18.7006781625187,21.1166607753892));
#41872=CARTESIAN_POINT('Ctrl Pts',(57.7177998078022,20.9709891684928,21.2436940700982));
#41873=CARTESIAN_POINT('Ctrl Pts',(56.4980263311406,23.2678612247765,21.3707273648071));
#41874=CARTESIAN_POINT('Ctrl Pts',(53.9067253704522,23.4883785901712,21.4977606595161));
#41875=CARTESIAN_POINT('Ctrl Pts',(52.3163789129282,21.4306451957916,21.6247939542251));
#41876=CARTESIAN_POINT('Ctrl Pts',(53.1830387183245,18.9786318681331,21.7518272489341));
#41877=CARTESIAN_POINT('Ctrl Pts',(55.7132289192997,18.377294920829,21.8788605436431));
#41878=CARTESIAN_POINT('Ctrl Pts',(57.5904178713067,20.1771922000554,22.005893838352));
#41879=CARTESIAN_POINT('Ctrl Pts',(57.0959333541929,22.7304163656232,22.132927133061));
#41880=CARTESIAN_POINT('Ctrl Pts',(54.6825037957228,23.6993468809889,22.25996042777));
#41881=CARTESIAN_POINT('Ctrl Pts',(52.5597598955672,22.1968732833317,22.386993722479));
#41882=CARTESIAN_POINT('Ctrl Pts',(52.6711932600432,19.5985947796707,22.514027017188));
#41883=CARTESIAN_POINT('Ctrl Pts',(54.9147803673736,18.2833816908058,22.6410603118969));
#41884=CARTESIAN_POINT('Ctrl Pts',(57.236390848458,19.455385680316,22.7680936066059));
#41885=CARTESIAN_POINT('Ctrl Pts',(57.5104595407713,22.0415710814815,22.8951269013149));
#41886=CARTESIAN_POINT('Ctrl Pts',(55.4860611193094,23.6741394899906,23.0221601960239));
#41887=CARTESIAN_POINT('Ctrl Pts',(53.0166463652187,22.858382571772,23.1491934907328));
#41888=CARTESIAN_POINT('Ctrl Pts',(52.3631035782157,20.3411717337866,23.2762267854419));
#41889=CARTESIAN_POINT('Ctrl Pts',(54.1237879912074,18.4271552827118,23.4032600801508));
#41890=CARTESIAN_POINT('Ctrl Pts',(56.6866938518662,18.8687230883979,23.5302933748598));
#41891=CARTESIAN_POINT('Ctrl Pts',(57.7053364862291,21.2615949530694,23.6573266695688));
#41892=CARTESIAN_POINT('Ctrl Pts',(56.2470911869016,23.4149619034869,23.7843599642777));
#41893=CARTESIAN_POINT('Ctrl Pts',(53.6470636616895,23.3572952062854,23.9113932589868));
#41894=CARTESIAN_POINT('Ctrl Pts',(52.2857255608756,21.1413919702215,24.0384265536957));
#41895=CARTESIAN_POINT('Ctrl Pts',(53.4094585911178,18.7960364222356,24.1654598484047));
#41896=CARTESIAN_POINT('Ctrl Pts',(55.9894218744662,18.4685336685102,24.2924931431137));
#41897=CARTESIAN_POINT('Ctrl Pts',(57.6635136929334,20.458730932,24.4195264378227));
#41898=CARTESIAN_POINT('Ctrl Pts',(56.8990087172171,22.9444905083188,24.5465597325316));
#41899=CARTESIAN_POINT('Ctrl Pts',(54.3958542643545,23.6499595114864,24.6735930272407));
#41900=CARTESIAN_POINT('Ctrl Pts',(52.4458293259943,21.9292412954949,24.8006263219496));
#41901=CARTESIAN_POINT('Ctrl Pts',(52.8342913800274,19.3577503813382,24.9276596166586));
#41902=CARTESIAN_POINT('Ctrl Pts',(55.2055819077125,18.2898313999373,25.0546929113676));
#41903=CARTESIAN_POINT('Ctrl Pts',(57.388650137537,19.7032246097807,25.1817262060766));
#41904=CARTESIAN_POINT('Ctrl Pts',(57.384775565471,22.3038883700105,25.3087595007855));
#41905=CARTESIAN_POINT('Ctrl Pts',(55.1975027955429,23.7107695917942,25.4357927954946));
#41906=CARTESIAN_POINT('Ctrl Pts',(52.8294086958177,22.6357871823707,25.5628260902035));
#41907=CARTESIAN_POINT('Ctrl Pts',(52.4486061469625,20.0631521750783,25.6898593849125));
#41908=CARTESIAN_POINT('Ctrl Pts',(54.4037621667412,18.3482488299797,25.8168926796215));
#41909=CARTESIAN_POINT('Ctrl Pts',(56.9047805431344,19.0611833907388,25.9439259743305));
#41910=CARTESIAN_POINT('Ctrl Pts',(57.6619177790366,21.5491935260962,26.0709592690394));
#41911=CARTESIAN_POINT('Ctrl Pts',(55.9818162121494,23.5344256343431,26.1979925637484));
#41912=CARTESIAN_POINT('Ctrl Pts',(53.403008326761,23.1991709081766,26.3250258584574));
#41913=CARTESIAN_POINT('Ctrl Pts',(52.2859417187998,20.8506027606393,26.4520591531664));
#41914=CARTESIAN_POINT('Ctrl Pts',(53.6545201608476,18.6385199300512,26.5790924478753));
#41915=CARTESIAN_POINT('Ctrl Pts',(56.2534500084256,18.5890859617113,26.7061257425844));
#41916=CARTESIAN_POINT('Ctrl Pts',(57.7077488873855,20.7458285859136,26.8331590372933));
#41917=CARTESIAN_POINT('Ctrl Pts',(56.6769480549284,23.1376911597642,26.9601923320024));
#41918=CARTESIAN_POINT('Ctrl Pts',(54.9753886330167,23.4231245943478,27.0448811951416));
#41919=CARTESIAN_POINT('Ctrl Pts',(54.2522308533113,23.1744372236737,27.0872256267113));
#41920=CARTESIAN_POINT('Ctrl Pts',(56.2471938071815,19.2544992399175,7.61303338694684));
#41921=CARTESIAN_POINT('Ctrl Pts',(56.8279583285158,19.6694378546349,7.65539542460912));
#41922=CARTESIAN_POINT('Ctrl Pts',(57.5322829868957,21.1173933320387,7.74010189384106));
#41923=CARTESIAN_POINT('Ctrl Pts',(56.2721082403061,23.1954260825845,7.86715279464267));
#41924=CARTESIAN_POINT('Ctrl Pts',(53.846005739048,23.2572672222738,7.99418608935165));
#41925=CARTESIAN_POINT('Ctrl Pts',(52.4771841003984,21.2553354972227,8.12121938406063));
#41926=CARTESIAN_POINT('Ctrl Pts',(53.4177661994886,19.0181669343711,8.2482526787696));
#41927=CARTESIAN_POINT('Ctrl Pts',(55.8071649642388,18.5962250790995,8.37528597347859));
#41928=CARTESIAN_POINT('Ctrl Pts',(57.4574603067288,20.3746927632235,8.50231926818757));
#41929=CARTESIAN_POINT('Ctrl Pts',(56.8578626487033,22.7258596455877,8.62935256289655));
#41930=CARTESIAN_POINT('Ctrl Pts',(54.5572613565354,23.4968050064229,8.75638585760554));
#41931=CARTESIAN_POINT('Ctrl Pts',(52.6620253874827,21.9818357787205,8.88341915231452));
#41932=CARTESIAN_POINT('Ctrl Pts',(52.9073301377167,19.5679145012814,9.01045244702349));
#41933=CARTESIAN_POINT('Ctrl Pts',(55.0685954582813,18.465161502043,9.13748574173249));
#41934=CARTESIAN_POINT('Ctrl Pts',(57.1670560144063,19.6831891041406,9.26451903644145));
#41935=CARTESIAN_POINT('Ctrl Pts',(57.2814556268961,22.1068347396299,9.39155233115045));
#41936=CARTESIAN_POINT('Ctrl Pts',(55.3070536478788,23.5171090442367,9.51858562585943));
#41937=CARTESIAN_POINT('Ctrl Pts',(53.0515269941901,22.6228291518185,9.6456189205684));
#41938=CARTESIAN_POINT('Ctrl Pts',(52.5799370068662,20.2427572972383,9.7726522152774));
#41939=CARTESIAN_POINT('Ctrl Pts',(54.3240510637364,18.5559840278521,9.89968550998636));
#41940=CARTESIAN_POINT('Ctrl Pts',(56.687034413851,19.106844920805,10.0267188046954));
#41941=CARTESIAN_POINT('Ctrl Pts',(57.5054427502093,21.3909959849688,10.1537520994043));
#41942=CARTESIAN_POINT('Ctrl Pts',(56.029977118908,23.3171681697859,10.2807853941133));
#41943=CARTESIAN_POINT('Ctrl Pts',(53.6115094249302,23.1218423945828,10.4078186888223));
#41944=CARTESIAN_POINT('Ctrl Pts',(52.464283058435,20.9838503838648,10.5348519835313));
#41945=CARTESIAN_POINT('Ctrl Pts',(53.6386483798942,18.8606442606204,10.6618852782403));
#41946=CARTESIAN_POINT('Ctrl Pts',(56.059407788523,18.6961388160039,10.7889185729493));
#41947=CARTESIAN_POINT('Ctrl Pts',(57.5102196948175,20.6409480537896,10.9159518676582));
#41948=CARTESIAN_POINT('Ctrl Pts',(56.6627840796645,22.9144895717303,11.0429851623672));
#41949=CARTESIAN_POINT('Ctrl Pts',(54.2929759816377,23.4352080514572,11.1700184570762));
#41950=CARTESIAN_POINT('Ctrl Pts',(52.570488196235,21.7263563943386,11.2970517517852));
#41951=CARTESIAN_POINT('Ctrl Pts',(53.0723553119393,19.3524845455114,11.4240850464941));
#41952=CARTESIAN_POINT('Ctrl Pts',(55.3390897161145,18.4870058932248,11.5511183412032));
#41953=CARTESIAN_POINT('Ctrl Pts',(57.2953683856162,19.9223148926776,11.6781516359121));
#41954=CARTESIAN_POINT('Ctrl Pts',(57.1501080091089,22.3443053095913,11.8051849306211));
#41955=CARTESIAN_POINT('Ctrl Pts',(55.0363026432278,23.535508496206,11.9322182253301));
#41956=CARTESIAN_POINT('Ctrl Pts',(52.8892601626876,22.4053108394288,12.0592515200391));
#41957=CARTESIAN_POINT('Ctrl Pts',(52.6747188927902,19.9884719535837,12.1862848147481));
#41958=CARTESIAN_POINT('Ctrl Pts',(54.589103450383,18.4977439695851,12.313318109457));
#41959=CARTESIAN_POINT('Ctrl Pts',(56.8796869433191,19.2979723235654,12.440351404166));
#41960=CARTESIAN_POINT('Ctrl Pts',(57.4493111643545,21.6565028837733,12.567384698875));
#41961=CARTESIAN_POINT('Ctrl Pts',(55.7764530544634,23.4139680756897,12.694417993584));
#41962=CARTESIAN_POINT('Ctrl Pts',(53.3927084386978,22.9613095250879,12.821451288293));
#41963=CARTESIAN_POINT('Ctrl Pts',(52.4805297796474,20.7129616315005,12.9484845830019));
#41964=CARTESIAN_POINT('Ctrl Pts',(53.8750680190704,18.7274135320046,13.0755178777109));
#41965=CARTESIAN_POINT('Ctrl Pts',(56.2995448499803,18.8225463497186,13.2025511724199));
#41966=CARTESIAN_POINT('Ctrl Pts',(57.5342151725387,20.9112606315721,13.3295844671289));
#41967=CARTESIAN_POINT('Ctrl Pts',(56.4486687623729,23.0812208035572,13.4566177618379));
#41968=CARTESIAN_POINT('Ctrl Pts',(54.036784502503,23.3457061029925,13.5836510565469));
#41969=CARTESIAN_POINT('Ctrl Pts',(52.506778284691,21.4625653408395,13.7106843512558));
#41970=CARTESIAN_POINT('Ctrl Pts',(53.2594569805109,19.1559199546814,13.8377176459648));
#41971=CARTESIAN_POINT('Ctrl Pts',(55.6057008485412,18.5376337197097,13.9647509406738));
#41972=CARTESIAN_POINT('Ctrl Pts',(57.3973914730114,20.1737825096463,14.0917842353828));
#41973=CARTESIAN_POINT('Ctrl Pts',(56.9941351684097,22.5663799495479,14.2188175300918));
#41974=CARTESIAN_POINT('Ctrl Pts',(54.7651357954234,23.5248683176836,14.3458508248007));
#41975=CARTESIAN_POINT('Ctrl Pts',(52.7511678306937,22.1716975251863,14.4728841195097));
#41976=CARTESIAN_POINT('Ctrl Pts',(52.7961323847391,19.7457716513177,14.5999174142187));
#41977=CARTESIAN_POINT('Ctrl Pts',(54.8588618756563,18.468162476364,14.7269507089277));
#41978=CARTESIAN_POINT('Ctrl Pts',(57.0508112691597,19.5085931626406,14.8539840036367));
#41979=CARTESIAN_POINT('Ctrl Pts',(57.3651274317021,21.9144908135372,14.9810172983457));
#41980=CARTESIAN_POINT('Ctrl Pts',(55.5140362122968,23.4831206150089,15.1080505930546));
#41981=CARTESIAN_POINT('Ctrl Pts',(53.1923158869174,22.7783136291282,15.2350838877636));
#41982=CARTESIAN_POINT('Ctrl Pts',(52.5256321867243,20.4453603504442,15.3621171824726));
#41983=CARTESIAN_POINT('Ctrl Pts',(54.1243715908862,18.6202109115749,15.4891504771816));
#41984=CARTESIAN_POINT('Ctrl Pts',(56.5247981242588,18.9738924272164,15.6161837718905));
#41985=CARTESIAN_POINT('Ctrl Pts',(57.5291860890565,21.1825895483253,15.7432170665996));
#41986=CARTESIAN_POINT('Ctrl Pts',(56.2179617303263,23.2241156533991,15.8702503613085));
#41987=CARTESIAN_POINT('Ctrl Pts',(53.7916248045405,23.2293386021941,15.9972836560175));
#41988=CARTESIAN_POINT('Ctrl Pts',(52.4716234331684,21.1934764909004,16.1243169507265));
#41989=CARTESIAN_POINT('Ctrl Pts',(53.4664932221301,18.980475754426,16.2513502454355));
#41990=CARTESIAN_POINT('Ctrl Pts',(55.8653748425715,18.6164632165459,16.3783835401444));
#41991=CARTESIAN_POINT('Ctrl Pts',(57.4719570515144,20.4347128590685,16.5054168348534));
#41992=CARTESIAN_POINT('Ctrl Pts',(56.8153233442833,22.770514719491,16.6324501295624));
#41993=CARTESIAN_POINT('Ctrl Pts',(54.4966588654143,23.4853106281647,16.7594834242714));
#41994=CARTESIAN_POINT('Ctrl Pts',(52.6388315464635,21.9246646690871,16.8865167189804));
#41995=CARTESIAN_POINT('Ctrl Pts',(52.9427869419565,19.5174361227759,17.0135500136893));
#41996=CARTESIAN_POINT('Ctrl Pts',(55.1302367667208,18.467578312992,17.1405833083984));
#41997=CARTESIAN_POINT('Ctrl Pts',(57.1984474958328,19.736295198909,17.2676166031073));
#41998=CARTESIAN_POINT('Ctrl Pts',(57.2538557127032,22.1620050096919,17.3946498978163));
#41999=CARTESIAN_POINT('Ctrl Pts',(55.2457320738625,23.5238337829797,17.5216831925253));
#42000=CARTESIAN_POINT('Ctrl Pts',(53.0126268802899,22.5749505704269,17.6487164872343));
#42001=CARTESIAN_POINT('Ctrl Pts',(52.5990737186382,20.1841113999444,17.7757497819432));
#42002=CARTESIAN_POINT('Ctrl Pts',(54.383703802205,18.5402641985739,17.9027830766522));
#42003=CARTESIAN_POINT('Ctrl Pts',(56.7325877683674,19.148443670547,18.0298163713612));
#42004=CARTESIAN_POINT('Ctrl Pts',(57.4951900428093,21.4518272529408,18.1568496660702));
#42005=CARTESIAN_POINT('Ctrl Pts',(55.9733052889244,23.3415375356346,18.2838829607792));
#42006=CARTESIAN_POINT('Ctrl Pts',(53.5603047206123,23.0874383149551,18.4109162554881));
#42007=CARTESIAN_POINT('Ctrl Pts',(52.4654262728904,20.9221717398333,18.5379495501971));
#42008=CARTESIAN_POINT('Ctrl Pts',(53.6910928347986,18.8281613206505,18.6649828449061));
#42009=CARTESIAN_POINT('Ctrl Pts',(56.115137631985,18.7225915434501,18.7920161396151));
#42010=CARTESIAN_POINT('Ctrl Pts',(57.5182111158202,20.7021174855848,18.9190494343241));
#42011=CARTESIAN_POINT('Ctrl Pts',(56.6157204823017,22.9543716482043,19.0460827290331));
#42012=CARTESIAN_POINT('Ctrl Pts',(54.2339467401253,23.4172884849082,19.173116023742));
#42013=CARTESIAN_POINT('Ctrl Pts',(52.5535379060985,21.667041557429,19.300149318451));
#42014=CARTESIAN_POINT('Ctrl Pts',(53.1130029185214,19.3060805123247,19.42718261316));
#42015=CARTESIAN_POINT('Ctrl Pts',(55.4001200460813,18.4959981699371,19.554215907869));
#42016=CARTESIAN_POINT('Ctrl Pts',(57.3209047342821,19.9784705434396,19.681249202578));
#42017=CARTESIAN_POINT('Ctrl Pts',(57.1167704109117,22.3962106731159,19.808282497287));
#42018=CARTESIAN_POINT('Ctrl Pts',(54.9746135470903,23.5356412885585,19.9353157919959));
#42019=CARTESIAN_POINT('Ctrl Pts',(52.8556994108257,22.3535494817334,20.0623490867049));
#42020=CARTESIAN_POINT('Ctrl Pts',(52.7000132438769,19.9322068843205,20.1893823814139));
#42021=CARTESIAN_POINT('Ctrl Pts',(54.6500945012683,18.488489028853,20.3164156761229));
#42022=CARTESIAN_POINT('Ctrl Pts',(56.9205339515342,19.3442009308982,20.4434489708319));
#42023=CARTESIAN_POINT('Ctrl Pts',(57.4326163931288,21.7158901452844,20.5704822655408));
#42024=CARTESIAN_POINT('Ctrl Pts',(55.7175015072043,23.4321416084171,20.6975155602498));
#42025=CARTESIAN_POINT('Ctrl Pts',(53.345473577427,22.9216304361771,20.8245488549588));
#42026=CARTESIAN_POINT('Ctrl Pts',(52.4882577804106,20.6517583618146,20.9515821496678));
#42027=CARTESIAN_POINT('Ctrl Pts',(53.930683461881,18.7007211222778,21.0786154443768));
#42028=CARTESIAN_POINT('Ctrl Pts',(56.3521286643486,18.8548032045331,21.2056487390858));
#42029=CARTESIAN_POINT('Ctrl Pts',(57.5356239145732,20.9729337834449,21.3326820337947));
#42030=CARTESIAN_POINT('Ctrl Pts',(56.3976126493923,23.1158450081452,21.4597153285037));
#42031=CARTESIAN_POINT('Ctrl Pts',(53.9800082817287,23.3215809507515,21.5867486232127));
#42032=CARTESIAN_POINT('Ctrl Pts',(52.4962637842209,21.4017787675202,21.7137819179217));
#42033=CARTESIAN_POINT('Ctrl Pts',(53.3048308177651,19.1141254920234,21.8408152126307));
#42034=CARTESIAN_POINT('Ctrl Pts',(55.6654207197859,18.5530965523924,21.9678485073396));
#42035=CARTESIAN_POINT('Ctrl Pts',(57.416780472339,20.2323455433887,22.0948818020486));
#42036=CARTESIAN_POINT('Ctrl Pts',(56.9554415748307,22.6144254283362,22.2219150967576));
#42037=CARTESIAN_POINT('Ctrl Pts',(54.7037857733155,23.5184078994761,22.3489483914666));
#42038=CARTESIAN_POINT('Ctrl Pts',(52.7233307808997,22.1166460867416,22.4759816861756));
#42039=CARTESIAN_POINT('Ctrl Pts',(52.8272946942958,19.6925318853606,22.6030149808846));
#42040=CARTESIAN_POINT('Ctrl Pts',(54.9204926949152,18.4654783874128,22.7300482755935));
#42041=CARTESIAN_POINT('Ctrl Pts',(57.0864841116712,19.5589221853135,22.8570815703025));
#42042=CARTESIAN_POINT('Ctrl Pts',(57.3421818008354,21.9717538927445,22.9841148650115));
#42043=CARTESIAN_POINT('Ctrl Pts',(55.4534801255511,23.4948901763327,23.1111481597205));
#42044=CARTESIAN_POINT('Ctrl Pts',(53.1495918525825,22.7338139762478,23.2381814544295));
#42045=CARTESIAN_POINT('Ctrl Pts',(52.5398564647277,20.3853334220528,23.3652147491384));
#42046=CARTESIAN_POINT('Ctrl Pts',(54.1825210534815,18.5996147417073,23.4922480438474));
#42047=CARTESIAN_POINT('Ctrl Pts',(56.5736336631851,19.0115839694587,23.6192813385564));
#42048=CARTESIAN_POINT('Ctrl Pts',(57.5239960175717,21.244060072795,23.7463146332654));
#42049=CARTESIAN_POINT('Ctrl Pts',(56.1634978514913,23.2530854324462,23.8733479279744));
#42050=CARTESIAN_POINT('Ctrl Pts',(53.7377518666139,23.1992841715592,24.0003812226833));
#42051=CARTESIAN_POINT('Ctrl Pts',(52.4676651463435,21.1319143742643,24.1274145173924));
#42052=CARTESIAN_POINT('Ctrl Pts',(53.5160736188505,18.943769537924,24.2544478121013));
#42053=CARTESIAN_POINT('Ctrl Pts',(55.9231002810787,18.6382195073252,24.3814811068103));
#42054=CARTESIAN_POINT('Ctrl Pts',(57.4849766333806,20.4950125505569,24.5085144015193));
#42055=CARTESIAN_POINT('Ctrl Pts',(56.7717169246738,22.814150041662,24.6355476962283));
#42056=CARTESIAN_POINT('Ctrl Pts',(54.4363505469416,23.4723309975539,24.7625809909372));
#42057=CARTESIAN_POINT('Ctrl Pts',(52.6170370516924,21.8669536455561,24.8896142856462));
#42058=CARTESIAN_POINT('Ctrl Pts',(52.9794602409511,19.4678314440883,25.0166475803552));
#42059=CARTESIAN_POINT('Ctrl Pts',(55.191801618391,18.4714957683358,25.1436808750642));
#42060=CARTESIAN_POINT('Ctrl Pts',(57.2285373613243,19.7901483097356,25.2707141697732));
#42061=CARTESIAN_POINT('Ctrl Pts',(57.2249225043503,22.2164878823824,25.3977474644821));
#42062=CARTESIAN_POINT('Ctrl Pts',(55.184264054378,23.5290649385282,25.5247807591912));
#42063=CARTESIAN_POINT('Ctrl Pts',(52.9749048462477,22.526139300939,25.6518140539001));
#42064=CARTESIAN_POINT('Ctrl Pts',(52.6196277405404,20.1259496956444,25.7788473486091));
#42065=CARTESIAN_POINT('Ctrl Pts',(54.4437283774751,18.5259974399519,25.9058806433181));
#42066=CARTESIAN_POINT('Ctrl Pts',(56.7771018613365,19.191143532242,26.032913938027));
#42067=CARTESIAN_POINT('Ctrl Pts',(57.483487694633,21.5123807259463,26.159947232736));
#42068=CARTESIAN_POINT('Ctrl Pts',(55.9160044312663,23.3645414315281,26.286980527445));
#42069=CARTESIAN_POINT('Ctrl Pts',(53.5100557199194,23.0517590482558,26.414013822154));
#42070=CARTESIAN_POINT('Ctrl Pts',(52.4678668150611,20.8606169550065,26.541047116863));
#42071=CARTESIAN_POINT('Ctrl Pts',(53.7447085517716,18.7968114789175,26.668080411572));
#42072=CARTESIAN_POINT('Ctrl Pts',(56.1694304370623,18.7506911017083,26.7951137062809));
#42073=CARTESIAN_POINT('Ctrl Pts',(57.5262467139057,20.7628658615296,26.9221470009899));
#42074=CARTESIAN_POINT('Ctrl Pts',(56.5645411333706,22.9944003274668,27.0491802956989));
#42075=CARTESIAN_POINT('Ctrl Pts',(54.9770383489932,23.2607009728164,27.1338691588382));
#42076=CARTESIAN_POINT('Ctrl Pts',(54.3023543067887,23.0286832787525,27.1762135904079));
#42077=CARTESIAN_POINT('Ctrl Pts',(56.1575872040306,19.3799074908306,7.70202135064341));
#42078=CARTESIAN_POINT('Ctrl Pts',(56.6966257837449,19.7650341873306,7.74438338830569));
#42079=CARTESIAN_POINT('Ctrl Pts',(57.3503471278769,21.1089590232279,7.82908985753763));
#42080=CARTESIAN_POINT('Ctrl Pts',(56.1807116204721,23.0376922383364,7.95614075833924));
#42081=CARTESIAN_POINT('Ctrl Pts',(53.9289162740299,23.0950903039575,8.08317405304821));
#42082=CARTESIAN_POINT('Ctrl Pts',(52.6584397816218,21.2369905163238,8.2102073477572));
#42083=CARTESIAN_POINT('Ctrl Pts',(53.5314442785794,19.160554851951,8.33724064246617));
#42084=CARTESIAN_POINT('Ctrl Pts',(55.7491729262641,18.768928073743,8.46427393717517));
#42085=CARTESIAN_POINT('Ctrl Pts',(57.2809002009969,20.41961894638,8.59130723188414));
#42086=CARTESIAN_POINT('Ctrl Pts',(56.7243815809553,22.6018625414762,8.71834052659312));
#42087=CARTESIAN_POINT('Ctrl Pts',(54.5890706115975,23.3174181187817,8.84537382130211));
#42088=CARTESIAN_POINT('Ctrl Pts',(52.8300008553486,21.9112942410088,8.97240711601109));
#42089=CARTESIAN_POINT('Ctrl Pts',(53.0576812994974,19.6708049391771,9.09944041072007));
#42090=CARTESIAN_POINT('Ctrl Pts',(55.0636671095574,18.6472809657784,9.22647370542905));
#42091=CARTESIAN_POINT('Ctrl Pts',(57.0113604623833,19.7777974566601,9.35350700013803));
#42092=CARTESIAN_POINT('Ctrl Pts',(57.1175408545581,22.0273124547239,9.48054029484702));
#42093=CARTESIAN_POINT('Ctrl Pts',(55.2849928950004,23.3362633810241,9.607573589556));
#42094=CARTESIAN_POINT('Ctrl Pts',(53.1915181057372,22.5062344357837,9.73460688426498));
#42095=CARTESIAN_POINT('Ctrl Pts',(52.7538102437097,20.2971625917199,9.86164017897397));
#42096=CARTESIAN_POINT('Ctrl Pts',(54.3726156795429,18.7315782041938,9.98867347368293));
#42097=CARTESIAN_POINT('Ctrl Pts',(56.5658267696552,19.2428616288,10.115706768392));
#42098=CARTESIAN_POINT('Ctrl Pts',(57.3254352702633,21.3629042626903,10.2427400631009));
#42099=CARTESIAN_POINT('Ctrl Pts',(55.9559767907978,23.1506875735641,10.3697733578099));
#42100=CARTESIAN_POINT('Ctrl Pts',(53.7112677168834,22.9693952862784,10.4968066525189));
#42101=CARTESIAN_POINT('Ctrl Pts',(52.6464656353348,20.9850106784683,10.6238399472279));
#42102=CARTESIAN_POINT('Ctrl Pts',(53.7364568308897,19.0143496427617,10.7508732419369));
#42103=CARTESIAN_POINT('Ctrl Pts',(55.9832929676071,18.861663350876,10.8779065366458));
#42104=CARTESIAN_POINT('Ctrl Pts',(57.3298690077631,20.6667447062981,11.0049398313548));
#42105=CARTESIAN_POINT('Ctrl Pts',(56.5433187389178,22.7769400535218,11.1319731260638));
#42106=CARTESIAN_POINT('Ctrl Pts',(54.3437732356544,23.2602466940481,11.2590064207728));
#42107=CARTESIAN_POINT('Ctrl Pts',(52.7450402977582,21.6741701753253,11.3860397154818));
#42108=CARTESIAN_POINT('Ctrl Pts',(53.2108499801973,19.4708528878373,11.5130730101907));
#42109=CARTESIAN_POINT('Ctrl Pts',(55.3147272814636,18.6675559122754,11.6401063048997));
#42110=CARTESIAN_POINT('Ctrl Pts',(57.1304540292182,19.9997428763457,11.7671395996087));
#42111=CARTESIAN_POINT('Ctrl Pts',(56.9956301132161,22.2477215776191,11.8941728943177));
#42112=CARTESIAN_POINT('Ctrl Pts',(55.033694422656,23.3533408953913,12.0212061890267));
#42113=CARTESIAN_POINT('Ctrl Pts',(53.0409095902807,22.3043440690943,12.1482394837357));
#42114=CARTESIAN_POINT('Ctrl Pts',(52.8417823757775,20.0611467790271,12.2752727784447));
#42115=CARTESIAN_POINT('Ctrl Pts',(54.6186249600678,18.6775224946293,12.4023060731536));
#42116=CARTESIAN_POINT('Ctrl Pts',(56.7446378747558,19.4202571823225,12.5293393678626));
#42117=CARTESIAN_POINT('Ctrl Pts',(57.2733365465898,21.6093354002316,12.6563726625716));
#42118=CARTESIAN_POINT('Ctrl Pts',(55.7206675620115,23.2405327377881,12.7834059572806));
#42119=CARTESIAN_POINT('Ctrl Pts',(53.5081868320733,22.8203961535986,12.9104392519896));
#42120=CARTESIAN_POINT('Ctrl Pts',(52.6615450852764,20.7335843551119,13.0374725466985));
#42121=CARTESIAN_POINT('Ctrl Pts',(53.955890528777,18.8906910856543,13.1645058414075));
#42122=CARTESIAN_POINT('Ctrl Pts',(56.2061770037176,18.9789889362651,13.2915391361165));
#42123=CARTESIAN_POINT('Ctrl Pts',(57.3521404925994,20.9176362512431,13.4185724308254));
#42124=CARTESIAN_POINT('Ctrl Pts',(56.3445868737848,22.9316922174306,13.5456057255345));
#42125=CARTESIAN_POINT('Ctrl Pts',(54.1059882367871,23.1771751540179,13.6726390202434));
#42126=CARTESIAN_POINT('Ctrl Pts',(52.6859077251393,21.4293316054816,13.7996723149524));
#42127=CARTESIAN_POINT('Ctrl Pts',(53.3845090347436,19.2884107895844,13.9267056096614));
#42128=CARTESIAN_POINT('Ctrl Pts',(55.5621833172234,18.714546302838,14.0537389043704));
#42129=CARTESIAN_POINT('Ctrl Pts',(57.225147107234,20.2331434063634,14.1807721990794));
#42130=CARTESIAN_POINT('Ctrl Pts',(56.8508633868822,22.4538409153462,14.3078054937884));
#42131=CARTESIAN_POINT('Ctrl Pts',(54.7820099840639,23.343465177251,14.4348387884973));
#42132=CARTESIAN_POINT('Ctrl Pts',(52.912738719346,22.0875150713064,14.5618720832063));
#42133=CARTESIAN_POINT('Ctrl Pts',(52.954472724196,19.8358836621806,14.6889053779153));
#42134=CARTESIAN_POINT('Ctrl Pts',(54.8690021664633,18.6500663303734,14.8159386726243));
#42135=CARTESIAN_POINT('Ctrl Pts',(56.9034675039205,19.61574563553,14.9429719673333));
#42136=CARTESIAN_POINT('Ctrl Pts',(57.1952011267819,21.8487877809036,15.0700052620422));
#42137=CARTESIAN_POINT('Ctrl Pts',(55.4771044711229,23.3047169040189,15.1970385567512));
#42138=CARTESIAN_POINT('Ctrl Pts',(53.3221917987528,22.650547885965,15.3240718514602));
#42139=CARTESIAN_POINT('Ctrl Pts',(52.7034070388898,20.4852093095101,15.4511051461692));
#42140=CARTESIAN_POINT('Ctrl Pts',(54.1872824928738,18.7911906063115,15.5781384408781));
#42141=CARTESIAN_POINT('Ctrl Pts',(56.4152466017777,19.119461316486,15.7051717355872));
#42142=CARTESIAN_POINT('Ctrl Pts',(57.3474727315399,21.1694711146848,15.8322050302961));
#42143=CARTESIAN_POINT('Ctrl Pts',(56.1304553517716,23.0643205617556,15.9592383250051));
#42144=CARTESIAN_POINT('Ctrl Pts',(53.8784424234009,23.0691682595693,16.0862716197141));
#42145=CARTESIAN_POINT('Ctrl Pts',(52.6532786292859,21.179575867726,16.213304914423));
#42146=CARTESIAN_POINT('Ctrl Pts',(53.5766704315442,19.1255716541848,16.3403382091321));
#42147=CARTESIAN_POINT('Ctrl Pts',(55.8032006242194,18.7877121703337,16.467371503841));
#42148=CARTESIAN_POINT('Ctrl Pts',(57.294355404324,20.4753268039198,16.59440479855));
#42149=CARTESIAN_POINT('Ctrl Pts',(56.6848985798521,22.6433093012723,16.721438093259));
#42150=CARTESIAN_POINT('Ctrl Pts',(54.5328222018875,23.3067495722308,16.848471387968));
#42151=CARTESIAN_POINT('Ctrl Pts',(52.8084734123629,21.8582306797798,16.975504682677));
#42152=CARTESIAN_POINT('Ctrl Pts',(53.0905906537993,19.6239532592685,17.1025379773859));
#42153=CARTESIAN_POINT('Ctrl Pts',(55.1208797011197,18.6495241371388,17.2295712720949));
#42154=CARTESIAN_POINT('Ctrl Pts',(57.0404965733917,19.8270880604187,17.3566045668039));
#42155=CARTESIAN_POINT('Ctrl Pts',(57.0919238996646,22.0785189298516,17.4836378615129));
#42156=CARTESIAN_POINT('Ctrl Pts',(55.2280770660383,23.342504970322,17.6106711562219));
#42157=CARTESIAN_POINT('Ctrl Pts',(53.1554128317797,22.4617957664712,17.7377044509309));
#42158=CARTESIAN_POINT('Ctrl Pts',(52.7715720482881,20.2427302012723,17.8647377456398));
#42159=CARTESIAN_POINT('Ctrl Pts',(54.4279825730753,18.7169877908057,17.9917710403488));
#42160=CARTESIAN_POINT('Ctrl Pts',(56.6081072716794,19.2814716508572,18.1188043350578));
#42161=CARTESIAN_POINT('Ctrl Pts',(57.3159191847721,21.4193650124183,18.2458376297668));
#42162=CARTESIAN_POINT('Ctrl Pts',(55.9033766376859,23.1733060839466,18.3728709244757));
#42163=CARTESIAN_POINT('Ctrl Pts',(53.6637418951841,22.9374630219308,18.4999042191848));
#42164=CARTESIAN_POINT('Ctrl Pts',(52.6475267137473,20.9277634337484,18.6269375138937));
#42165=CARTESIAN_POINT('Ctrl Pts',(53.7851333313421,18.984200490768,18.7539708086027));
#42166=CARTESIAN_POINT('Ctrl Pts',(56.0350188127026,18.8862155404612,18.8810041033117));
#42167=CARTESIAN_POINT('Ctrl Pts',(57.337286272539,20.7235193239367,19.0080373980207));
#42168=CARTESIAN_POINT('Ctrl Pts',(56.4996364998232,22.8139567394053,19.1350706927297));
#42169=CARTESIAN_POINT('Ctrl Pts',(54.2889850429573,23.2436145869774,19.2621039874386));
#42170=CARTESIAN_POINT('Ctrl Pts',(52.7293078279099,21.6191169062822,19.3891372821476));
#42171=CARTESIAN_POINT('Ctrl Pts',(53.2485771954729,19.4277828254919,19.5161705768566));
#42172=CARTESIAN_POINT('Ctrl Pts',(55.3713727912637,18.6759021247062,19.6432038715656));
#42173=CARTESIAN_POINT('Ctrl Pts',(57.1541556786998,20.0518639359451,19.7702371662746));
#42174=CARTESIAN_POINT('Ctrl Pts',(56.9646877072614,22.295897718561,19.8972704609836));
#42175=CARTESIAN_POINT('Ctrl Pts',(54.976437476778,23.3534641470682,20.0243037556925));
#42176=CARTESIAN_POINT('Ctrl Pts',(53.0097600634877,22.256301587656,20.1513370504015));
#42177=CARTESIAN_POINT('Ctrl Pts',(52.8652594143769,20.0089241622712,20.2783703451105));
#42178=CARTESIAN_POINT('Ctrl Pts',(54.6752340128539,18.6689324896887,20.4054036398195));
#42179=CARTESIAN_POINT('Ctrl Pts',(56.78255016534,19.4631644225609,20.5324369345285));
#42180=CARTESIAN_POINT('Ctrl Pts',(57.2578412374936,21.6644558904165,20.6594702292374));
#42181=CARTESIAN_POINT('Ctrl Pts',(55.6659514815017,23.2574005644372,20.7865035239464));
#42182=CARTESIAN_POINT('Ctrl Pts',(53.4643456337959,22.783567871317,20.9135368186554));
#42183=CARTESIAN_POINT('Ctrl Pts',(52.6687178556547,20.6767783307191,21.0405701133644));
#42184=CARTESIAN_POINT('Ctrl Pts',(54.0075101925159,18.8659164341394,21.1676034080733));
#42185=CARTESIAN_POINT('Ctrl Pts',(56.2549828511337,19.0089282465475,21.2946367027823));
#42186=CARTESIAN_POINT('Ctrl Pts',(57.3534480213442,20.9748783983971,21.4216699974913));
#42187=CARTESIAN_POINT('Ctrl Pts',(56.297198967644,22.963828791514,21.5487032922003));
#42188=CARTESIAN_POINT('Ctrl Pts',(54.0532911930052,23.1547833113319,21.6757365869093));
#42189=CARTESIAN_POINT('Ctrl Pts',(52.6761486555135,21.3729123392486,21.8027698816183));
#42190=CARTESIAN_POINT('Ctrl Pts',(53.4266229172058,19.2496191159138,21.9298031763272));
#42191=CARTESIAN_POINT('Ctrl Pts',(55.6176125202719,18.7288981839558,22.0568364710362));
#42192=CARTESIAN_POINT('Ctrl Pts',(57.2431430733712,20.287498886722,22.1838697657452));
#42193=CARTESIAN_POINT('Ctrl Pts',(56.8149497954683,22.4984344910491,22.3109030604542));
#42194=CARTESIAN_POINT('Ctrl Pts',(54.7250677509081,23.3374689179634,22.4379363551632));
#42195=CARTESIAN_POINT('Ctrl Pts',(52.8869016662319,22.0364188901516,22.5649696498721));
#42196=CARTESIAN_POINT('Ctrl Pts',(52.9833961285485,19.7864689910505,22.6920029445812));
#42197=CARTESIAN_POINT('Ctrl Pts',(54.9262050224566,18.6475750840197,22.8190362392901));
#42198=CARTESIAN_POINT('Ctrl Pts',(56.9365773748846,19.6624586903111,22.9460695339992));
#42199=CARTESIAN_POINT('Ctrl Pts',(57.1739040608994,21.9019367040076,23.073102828708));
#42200=CARTESIAN_POINT('Ctrl Pts',(55.420899131793,23.3156408626749,23.2001361234171));
#42201=CARTESIAN_POINT('Ctrl Pts',(53.2825373399461,22.6092453807235,23.327169418126));
#42202=CARTESIAN_POINT('Ctrl Pts',(52.7166093512399,20.4294951103189,23.454202712835));
#42203=CARTESIAN_POINT('Ctrl Pts',(54.2412541157553,18.7720742007028,23.581236007544));
#42204=CARTESIAN_POINT('Ctrl Pts',(56.460573474504,19.1544448505195,23.708269302253));
#42205=CARTESIAN_POINT('Ctrl Pts',(57.3426555489142,21.2265251925206,23.835302596962));
#42206=CARTESIAN_POINT('Ctrl Pts',(56.0799045160809,23.0912089614057,23.9623358916709));
#42207=CARTESIAN_POINT('Ctrl Pts',(53.8284400715384,23.0412731368329,24.0893691863799));
#42208=CARTESIAN_POINT('Ctrl Pts',(52.6496047318115,21.1224367783073,24.216402481089));
#42209=CARTESIAN_POINT('Ctrl Pts',(53.6226886465833,19.0915026536122,24.3434357757979));
#42210=CARTESIAN_POINT('Ctrl Pts',(55.8567786876913,18.8079053461403,24.4704690705069));
#42211=CARTESIAN_POINT('Ctrl Pts',(57.306439573828,20.5312941691135,24.5975023652159));
#42212=CARTESIAN_POINT('Ctrl Pts',(56.6444251321306,22.6838095750054,24.7245356599248));
#42213=CARTESIAN_POINT('Ctrl Pts',(54.4768468295286,23.2947024836215,24.8515689546338));
#42214=CARTESIAN_POINT('Ctrl Pts',(52.7882447773904,21.8046659956174,24.9786022493428));
#42215=CARTESIAN_POINT('Ctrl Pts',(53.1246291018748,19.5779125068384,25.1056355440518));
#42216=CARTESIAN_POINT('Ctrl Pts',(55.1780213290696,18.6531601367342,25.2326688387608));
#42217=CARTESIAN_POINT('Ctrl Pts',(57.0684245851116,19.8770720096903,25.3597021334698));
#42218=CARTESIAN_POINT('Ctrl Pts',(57.0650694432295,22.1290873947541,25.4867354281787));
#42219=CARTESIAN_POINT('Ctrl Pts',(55.1710253132133,23.3473602852621,25.6137687228878));
#42220=CARTESIAN_POINT('Ctrl Pts',(53.1204009966777,22.4164914195073,25.7408020175967));
#42221=CARTESIAN_POINT('Ctrl Pts',(52.7906493341184,20.1887472162105,25.8678353123057));
#42222=CARTESIAN_POINT('Ctrl Pts',(54.4836945882088,18.7037460499241,25.9948686070146));
#42223=CARTESIAN_POINT('Ctrl Pts',(56.6494231795385,19.3211036737453,26.1219019017237));
#42224=CARTESIAN_POINT('Ctrl Pts',(57.3050576102293,21.4755679257963,26.2489351964326));
#42225=CARTESIAN_POINT('Ctrl Pts',(55.8501926503833,23.1946572287132,26.3759684911416));
#42226=CARTESIAN_POINT('Ctrl Pts',(53.6171031130779,22.9043471883351,26.5030017858506));
#42227=CARTESIAN_POINT('Ctrl Pts',(52.6497919113224,20.8706311493737,26.6300350805596));
#42228=CARTESIAN_POINT('Ctrl Pts',(53.8348969426956,18.9551030277838,26.7570683752686));
#42229=CARTESIAN_POINT('Ctrl Pts',(56.085410865699,18.9122962417053,26.8841016699775));
#42230=CARTESIAN_POINT('Ctrl Pts',(57.3447445404256,20.7799031371454,27.0111349646865));
#42231=CARTESIAN_POINT('Ctrl Pts',(56.452134211813,22.8511094951693,27.1381682593955));
#42232=CARTESIAN_POINT('Ctrl Pts',(54.9786880649696,23.098277351285,27.2228571225348));
#42233=CARTESIAN_POINT('Ctrl Pts',(54.352477760266,22.8829293338312,27.2652015541045));
#42234=CARTESIAN_POINT('Ctrl Pts',(56.0772665381941,23.205491718641,7.7));
#42235=CARTESIAN_POINT('Ctrl Pts',(56.0907843704075,23.1972259880661,7.7));
#42236=CARTESIAN_POINT('Ctrl Pts',(56.104302202621,23.1889602574912,7.7));
#42237=CARTESIAN_POINT('Ctrl Pts',(56.1178200348344,23.1806945269163,7.7));
#42238=CARTESIAN_POINT('Origin',(55.,21.,7.7));
#42239=CARTESIAN_POINT('',(57.6505,21.,7.5));
#42240=CARTESIAN_POINT('Origin',(55.,21.,7.5));
#42241=CARTESIAN_POINT('Origin',(57.6505,21.,7.7));
#42242=CARTESIAN_POINT('Origin',(55.,21.,7.5));
#42243=CARTESIAN_POINT('',(50.95,21.,7.5));
#42244=CARTESIAN_POINT('Origin',(55.,21.,7.5));
#42245=CARTESIAN_POINT('Origin',(55.,21.,27.25));
#42246=CARTESIAN_POINT('',(53.0495,21.,27.5));
#42247=CARTESIAN_POINT('',(52.7995,21.,27.25));
#42248=CARTESIAN_POINT('Origin',(55.,21.,27.5));
#42249=CARTESIAN_POINT('Origin',(55.,21.,27.5));
#42250=CARTESIAN_POINT('Origin',(59.2592935317778,20.2489716315905,6.9));
#42251=CARTESIAN_POINT('',(59.1721341053809,20.1901870544887,6.9));
#42252=CARTESIAN_POINT('',(59.1974959714464,20.3340213444176,6.9));
#42253=CARTESIAN_POINT('Origin',(55.,21.,6.9));
#42254=CARTESIAN_POINT('',(59.0377117873501,20.2880424715656,6.9));
#42255=CARTESIAN_POINT('',(59.0377117873501,20.2880424715656,6.9));
#42256=CARTESIAN_POINT('',(59.5190778752923,20.4265584972782,6.9));
#42257=CARTESIAN_POINT('Origin',(59.5190778752923,20.4265584972782,2.5));
#42258=CARTESIAN_POINT('',(59.1974959714464,20.3340213444176,2.9));
#42259=CARTESIAN_POINT('',(59.1974959714464,20.3340213444176,7.5));
#42260=CARTESIAN_POINT('',(59.0377117873501,20.2880424715656,2.75000000000001));
#42261=CARTESIAN_POINT('',(59.0377117873501,20.2880424715656,2.5));
#42262=CARTESIAN_POINT('Ctrl Pts',(59.1974959714464,20.3340213444176,2.90000000000003));
#42263=CARTESIAN_POINT('Ctrl Pts',(59.1161686921159,20.3106189241037,2.82334460824933));
#42264=CARTESIAN_POINT('Ctrl Pts',(59.0377117873501,20.2880424715656,2.75000000000001));
#42265=CARTESIAN_POINT('Origin',(59.0377117873501,20.2880424715656,2.5));
#42266=CARTESIAN_POINT('',(59.1721341053809,20.1901870544887,2.9));
#42267=CARTESIAN_POINT('',(59.1721341053809,20.1901870544887,7.5));
#42268=CARTESIAN_POINT('Ctrl Pts',(59.0377117873501,20.2880424715656,2.75000000000001));
#42269=CARTESIAN_POINT('Ctrl Pts',(59.1037155602747,20.2399937038996,2.82334460824863));
#42270=CARTESIAN_POINT('Ctrl Pts',(59.1721341053809,20.1901870544887,2.90000000000003));
#42271=CARTESIAN_POINT('Origin',(55.,21.,7.5));
#42272=CARTESIAN_POINT('',(50.7506274441751,21.0730265828477,6.9));
#42273=CARTESIAN_POINT('',(50.75,21.,6.9));
#42274=CARTESIAN_POINT('Origin',(55.,21.,6.9));
#42275=CARTESIAN_POINT('',(50.75,21.,7.3));
#42276=CARTESIAN_POINT('',(50.75,21.,7.5));
#42277=CARTESIAN_POINT('Origin',(55.,21.,7.3));
#42278=CARTESIAN_POINT('',(50.7506274441751,20.9269734171523,6.9));
#42279=CARTESIAN_POINT('Origin',(55.,21.,6.9));
#42280=CARTESIAN_POINT('',(50.7506274441751,20.9269734171523,2.9));
#42281=CARTESIAN_POINT('',(50.7506274441751,20.9269734171523,7.5));
#42282=CARTESIAN_POINT('',(50.8025040285536,20.3340213444176,2.9));
#42283=CARTESIAN_POINT('Origin',(55.,21.,2.9));
#42284=CARTESIAN_POINT('',(50.8025040285536,20.3340213444176,6.9));
#42285=CARTESIAN_POINT('',(50.8025040285536,20.3340213444176,7.5));
#42286=CARTESIAN_POINT('',(50.8278658946191,20.1901870544887,6.9));
#42287=CARTESIAN_POINT('Origin',(55.,21.,6.9));
#42288=CARTESIAN_POINT('',(50.8278658946191,20.1901870544887,2.9));
#42289=CARTESIAN_POINT('',(50.8278658946191,20.1901870544887,7.5));
#42290=CARTESIAN_POINT('',(50.9819194039891,19.6152515304358,2.9));
#42291=CARTESIAN_POINT('Origin',(55.,21.,2.9));
#42292=CARTESIAN_POINT('',(50.9819194039891,19.6152515304358,6.9));
#42293=CARTESIAN_POINT('',(50.9819194039891,19.6152515304358,7.5));
#42294=CARTESIAN_POINT('',(51.0318725286534,19.4780064483894,6.9));
#42295=CARTESIAN_POINT('Origin',(55.,21.,6.9));
#42296=CARTESIAN_POINT('',(51.0318725286534,19.4780064483894,2.9));
#42297=CARTESIAN_POINT('',(51.0318725286534,19.4780064483894,7.5));
#42298=CARTESIAN_POINT('',(51.2834221250874,18.9385565979853,2.9));
#42299=CARTESIAN_POINT('Origin',(55.,21.,2.9));
#42300=CARTESIAN_POINT('',(51.2834221250874,18.9385565979853,6.9));
#42301=CARTESIAN_POINT('',(51.2834221250874,18.9385565979853,7.5));
#42302=CARTESIAN_POINT('',(51.3564487079351,18.8120708461899,6.9));
#42303=CARTESIAN_POINT('Origin',(55.,21.,6.9));
#42304=CARTESIAN_POINT('',(51.3564487079351,18.8120708461899,2.9));
#42305=CARTESIAN_POINT('',(51.3564487079351,18.8120708461899,7.5));
#42306=CARTESIAN_POINT('',(51.6978511842358,18.3244975801642,2.9));
#42307=CARTESIAN_POINT('Origin',(55.,21.,2.9));
#42308=CARTESIAN_POINT('',(51.6978511842358,18.3244975801642,6.9));
#42309=CARTESIAN_POINT('',(51.6978511842358,18.3244975801642,7.5));
#42310=CARTESIAN_POINT('',(51.7917323495003,18.2126143641833,6.9));
#42311=CARTESIAN_POINT('Origin',(55.,21.,6.9));
#42312=CARTESIAN_POINT('',(51.7917323495003,18.2126143641833,2.9));
#42313=CARTESIAN_POINT('',(51.7917323495003,18.2126143641833,7.5));
#42314=CARTESIAN_POINT('',(52.2126143641833,17.7917323495003,2.9));
#42315=CARTESIAN_POINT('Origin',(55.,21.,2.9));
#42316=CARTESIAN_POINT('',(52.2126143641833,17.7917323495003,6.9));
#42317=CARTESIAN_POINT('',(52.2126143641833,17.7917323495003,7.5));
#42318=CARTESIAN_POINT('',(52.3244975801642,17.6978511842358,6.9));
#42319=CARTESIAN_POINT('Origin',(55.,21.,6.9));
#42320=CARTESIAN_POINT('',(52.3244975801642,17.6978511842358,2.9));
#42321=CARTESIAN_POINT('',(52.3244975801642,17.6978511842358,7.5));
#42322=CARTESIAN_POINT('',(52.8120708461899,17.3564487079351,2.9));
#42323=CARTESIAN_POINT('Origin',(55.,21.,2.9));
#42324=CARTESIAN_POINT('',(52.8120708461899,17.3564487079351,6.9));
#42325=CARTESIAN_POINT('',(52.8120708461899,17.3564487079351,7.5));
#42326=CARTESIAN_POINT('',(52.9385565979852,17.2834221250874,6.9));
#42327=CARTESIAN_POINT('Origin',(55.,21.,6.9));
#42328=CARTESIAN_POINT('',(52.9385565979852,17.2834221250874,2.9));
#42329=CARTESIAN_POINT('',(52.9385565979852,17.2834221250874,7.5));
#42330=CARTESIAN_POINT('',(53.4780064483894,17.0318725286534,2.9));
#42331=CARTESIAN_POINT('Origin',(55.,21.,2.9));
#42332=CARTESIAN_POINT('',(53.4780064483894,17.0318725286534,6.9));
#42333=CARTESIAN_POINT('',(53.4780064483894,17.0318725286534,7.5));
#42334=CARTESIAN_POINT('',(53.6152515304358,16.9819194039891,6.9));
#42335=CARTESIAN_POINT('Origin',(55.,21.,6.9));
#42336=CARTESIAN_POINT('',(53.6152515304358,16.9819194039891,2.9));
#42337=CARTESIAN_POINT('',(53.6152515304358,16.9819194039891,7.5));
#42338=CARTESIAN_POINT('',(54.1901870544887,16.8278658946191,2.9));
#42339=CARTESIAN_POINT('Origin',(55.,21.,2.9));
#42340=CARTESIAN_POINT('',(54.1901870544887,16.8278658946191,6.9));
#42341=CARTESIAN_POINT('',(54.1901870544887,16.8278658946191,7.5));
#42342=CARTESIAN_POINT('',(54.3340213444176,16.8025040285536,6.9));
#42343=CARTESIAN_POINT('Origin',(55.,21.,6.9));
#42344=CARTESIAN_POINT('',(54.3340213444176,16.8025040285536,2.9));
#42345=CARTESIAN_POINT('',(54.3340213444176,16.8025040285536,7.5));
#42346=CARTESIAN_POINT('',(54.9269734171523,16.7506274441751,2.9));
#42347=CARTESIAN_POINT('Origin',(55.,21.,2.9));
#42348=CARTESIAN_POINT('',(54.9269734171523,16.7506274441751,6.9));
#42349=CARTESIAN_POINT('',(54.9269734171523,16.7506274441751,7.5));
#42350=CARTESIAN_POINT('',(55.0730265828477,16.7506274441751,6.9));
#42351=CARTESIAN_POINT('Origin',(55.,21.,6.9));
#42352=CARTESIAN_POINT('',(55.0730265828477,16.7506274441751,2.9));
#42353=CARTESIAN_POINT('',(55.0730265828477,16.7506274441751,7.5));
#42354=CARTESIAN_POINT('',(55.6659786555824,16.8025040285536,2.9));
#42355=CARTESIAN_POINT('Origin',(55.,21.,2.9));
#42356=CARTESIAN_POINT('',(55.6659786555824,16.8025040285536,6.9));
#42357=CARTESIAN_POINT('',(55.6659786555824,16.8025040285536,7.5));
#42358=CARTESIAN_POINT('',(55.8098129455113,16.8278658946191,6.9));
#42359=CARTESIAN_POINT('Origin',(55.,21.,6.9));
#42360=CARTESIAN_POINT('',(55.8098129455113,16.8278658946191,2.9));
#42361=CARTESIAN_POINT('',(55.8098129455113,16.8278658946191,7.5));
#42362=CARTESIAN_POINT('',(56.3847484695642,16.9819194039891,2.9));
#42363=CARTESIAN_POINT('Origin',(55.,21.,2.9));
#42364=CARTESIAN_POINT('',(56.3847484695642,16.9819194039891,6.9));
#42365=CARTESIAN_POINT('',(56.3847484695642,16.9819194039891,7.5));
#42366=CARTESIAN_POINT('',(56.5219935516106,17.0318725286534,6.9));
#42367=CARTESIAN_POINT('Origin',(55.,21.,6.9));
#42368=CARTESIAN_POINT('',(56.5219935516106,17.0318725286534,2.9));
#42369=CARTESIAN_POINT('',(56.5219935516106,17.0318725286534,7.5));
#42370=CARTESIAN_POINT('',(57.0614434020148,17.2834221250874,2.9));
#42371=CARTESIAN_POINT('Origin',(55.,21.,2.9));
#42372=CARTESIAN_POINT('',(57.0614434020148,17.2834221250874,6.9));
#42373=CARTESIAN_POINT('',(57.0614434020148,17.2834221250874,7.5));
#42374=CARTESIAN_POINT('',(57.1879291538101,17.3564487079351,6.9));
#42375=CARTESIAN_POINT('Origin',(55.,21.,6.9));
#42376=CARTESIAN_POINT('',(57.1879291538101,17.3564487079351,2.9));
#42377=CARTESIAN_POINT('',(57.1879291538101,17.3564487079351,7.5));
#42378=CARTESIAN_POINT('',(57.6755024198358,17.6978511842358,2.9));
#42379=CARTESIAN_POINT('Origin',(55.,21.,2.9));
#42380=CARTESIAN_POINT('',(57.6755024198358,17.6978511842358,6.9));
#42381=CARTESIAN_POINT('',(57.6755024198358,17.6978511842358,7.5));
#42382=CARTESIAN_POINT('',(57.7873856358167,17.7917323495003,6.9));
#42383=CARTESIAN_POINT('Origin',(55.,21.,6.9));
#42384=CARTESIAN_POINT('',(57.7873856358167,17.7917323495003,2.9));
#42385=CARTESIAN_POINT('',(57.7873856358167,17.7917323495003,7.5));
#42386=CARTESIAN_POINT('',(58.2082676504997,18.2126143641833,2.9));
#42387=CARTESIAN_POINT('Origin',(55.,21.,2.9));
#42388=CARTESIAN_POINT('',(58.2082676504997,18.2126143641833,6.9));
#42389=CARTESIAN_POINT('',(58.2082676504997,18.2126143641833,7.5));
#42390=CARTESIAN_POINT('',(58.3021488157642,18.3244975801642,6.9));
#42391=CARTESIAN_POINT('Origin',(55.,21.,6.9));
#42392=CARTESIAN_POINT('',(58.3021488157642,18.3244975801642,2.9));
#42393=CARTESIAN_POINT('',(58.3021488157642,18.3244975801642,7.5));
#42394=CARTESIAN_POINT('',(58.6435512920649,18.8120708461899,2.9));
#42395=CARTESIAN_POINT('Origin',(55.,21.,2.9));
#42396=CARTESIAN_POINT('',(58.6435512920649,18.8120708461899,6.9));
#42397=CARTESIAN_POINT('',(58.6435512920649,18.8120708461899,7.5));
#42398=CARTESIAN_POINT('',(58.7165778749126,18.9385565979853,6.9));
#42399=CARTESIAN_POINT('Origin',(55.,21.,6.9));
#42400=CARTESIAN_POINT('',(58.7165778749126,18.9385565979853,2.9));
#42401=CARTESIAN_POINT('',(58.7165778749126,18.9385565979853,7.5));
#42402=CARTESIAN_POINT('',(58.9681274713466,19.4780064483894,2.9));
#42403=CARTESIAN_POINT('Origin',(55.,21.,2.9));
#42404=CARTESIAN_POINT('',(58.9681274713466,19.4780064483894,6.9));
#42405=CARTESIAN_POINT('',(58.9681274713466,19.4780064483894,7.5));
#42406=CARTESIAN_POINT('',(59.0180805960109,19.6152515304358,6.9));
#42407=CARTESIAN_POINT('Origin',(55.,21.,6.9));
#42408=CARTESIAN_POINT('',(59.0180805960109,19.6152515304358,2.9));
#42409=CARTESIAN_POINT('',(59.0180805960109,19.6152515304358,7.5));
#42410=CARTESIAN_POINT('Origin',(55.,21.,2.9));
#42411=CARTESIAN_POINT('',(59.2493725558249,20.9269734171523,2.9));
#42412=CARTESIAN_POINT('Origin',(55.,21.,2.9));
#42413=CARTESIAN_POINT('',(59.2493725558249,20.9269734171523,6.9));
#42414=CARTESIAN_POINT('',(59.2493725558249,20.9269734171523,7.5));
#42415=CARTESIAN_POINT('',(59.2493725558249,21.0730265828477,6.9));
#42416=CARTESIAN_POINT('Origin',(55.,21.,6.9));
#42417=CARTESIAN_POINT('',(59.2493725558249,21.0730265828477,2.9));
#42418=CARTESIAN_POINT('',(59.2493725558249,21.0730265828477,7.5));
#42419=CARTESIAN_POINT('',(59.1974959714464,21.6659786555824,2.9));
#42420=CARTESIAN_POINT('Origin',(55.,21.,2.9));
#42421=CARTESIAN_POINT('',(59.1974959714464,21.6659786555824,6.9));
#42422=CARTESIAN_POINT('',(59.1974959714464,21.6659786555824,7.5));
#42423=CARTESIAN_POINT('',(59.1721341053809,21.8098129455113,6.9));
#42424=CARTESIAN_POINT('Origin',(55.,21.,6.9));
#42425=CARTESIAN_POINT('',(59.1721341053809,21.8098129455113,2.9));
#42426=CARTESIAN_POINT('',(59.1721341053809,21.8098129455113,7.5));
#42427=CARTESIAN_POINT('',(59.0180805960109,22.3847484695642,2.9));
#42428=CARTESIAN_POINT('Origin',(55.,21.,2.9));
#42429=CARTESIAN_POINT('',(59.0180805960109,22.3847484695642,6.9));
#42430=CARTESIAN_POINT('',(59.0180805960109,22.3847484695642,7.5));
#42431=CARTESIAN_POINT('',(58.9681274713466,22.5219935516106,6.9));
#42432=CARTESIAN_POINT('Origin',(55.,21.,6.9));
#42433=CARTESIAN_POINT('',(58.9681274713466,22.5219935516106,2.9));
#42434=CARTESIAN_POINT('',(58.9681274713466,22.5219935516106,7.5));
#42435=CARTESIAN_POINT('',(58.7165778749126,23.0614434020147,2.9));
#42436=CARTESIAN_POINT('Origin',(55.,21.,2.9));
#42437=CARTESIAN_POINT('',(58.7165778749126,23.0614434020147,6.9));
#42438=CARTESIAN_POINT('',(58.7165778749126,23.0614434020147,7.5));
#42439=CARTESIAN_POINT('',(58.6435512920649,23.1879291538101,6.9));
#42440=CARTESIAN_POINT('Origin',(55.,21.,6.9));
#42441=CARTESIAN_POINT('',(58.6435512920649,23.1879291538101,2.9));
#42442=CARTESIAN_POINT('',(58.6435512920649,23.1879291538101,7.5));
#42443=CARTESIAN_POINT('',(58.3021488157642,23.6755024198358,2.9));
#42444=CARTESIAN_POINT('Origin',(55.,21.,2.9));
#42445=CARTESIAN_POINT('',(58.3021488157642,23.6755024198358,6.9));
#42446=CARTESIAN_POINT('',(58.3021488157642,23.6755024198358,7.5));
#42447=CARTESIAN_POINT('',(58.2082676504997,23.7873856358167,6.9));
#42448=CARTESIAN_POINT('Origin',(55.,21.,6.9));
#42449=CARTESIAN_POINT('',(58.2082676504997,23.7873856358167,2.9));
#42450=CARTESIAN_POINT('',(58.2082676504997,23.7873856358167,7.5));
#42451=CARTESIAN_POINT('',(57.7873856358167,24.2082676504997,2.9));
#42452=CARTESIAN_POINT('Origin',(55.,21.,2.9));
#42453=CARTESIAN_POINT('',(57.7873856358167,24.2082676504997,6.9));
#42454=CARTESIAN_POINT('',(57.7873856358167,24.2082676504997,7.5));
#42455=CARTESIAN_POINT('',(57.6755024198358,24.3021488157642,6.9));
#42456=CARTESIAN_POINT('Origin',(55.,21.,6.9));
#42457=CARTESIAN_POINT('',(57.6755024198358,24.3021488157642,2.9));
#42458=CARTESIAN_POINT('',(57.6755024198358,24.3021488157642,7.5));
#42459=CARTESIAN_POINT('',(57.1879291538101,24.6435512920649,2.9));
#42460=CARTESIAN_POINT('Origin',(55.,21.,2.9));
#42461=CARTESIAN_POINT('',(57.1879291538101,24.6435512920649,6.9));
#42462=CARTESIAN_POINT('',(57.1879291538101,24.6435512920649,7.5));
#42463=CARTESIAN_POINT('',(57.0614434020147,24.7165778749126,6.9));
#42464=CARTESIAN_POINT('Origin',(55.,21.,6.9));
#42465=CARTESIAN_POINT('',(57.0614434020147,24.7165778749126,2.9));
#42466=CARTESIAN_POINT('',(57.0614434020147,24.7165778749126,7.5));
#42467=CARTESIAN_POINT('',(56.5219935516106,24.9681274713466,2.9));
#42468=CARTESIAN_POINT('Origin',(55.,21.,2.9));
#42469=CARTESIAN_POINT('',(56.5219935516106,24.9681274713466,6.9));
#42470=CARTESIAN_POINT('',(56.5219935516106,24.9681274713466,7.5));
#42471=CARTESIAN_POINT('',(56.3847484695642,25.0180805960109,6.9));
#42472=CARTESIAN_POINT('Origin',(55.,21.,6.9));
#42473=CARTESIAN_POINT('',(56.3847484695642,25.0180805960109,2.9));
#42474=CARTESIAN_POINT('',(56.3847484695642,25.0180805960109,7.5));
#42475=CARTESIAN_POINT('',(55.8098129455113,25.1721341053809,2.9));
#42476=CARTESIAN_POINT('Origin',(55.,21.,2.9));
#42477=CARTESIAN_POINT('',(55.8098129455113,25.1721341053809,6.9));
#42478=CARTESIAN_POINT('',(55.8098129455113,25.1721341053809,7.5));
#42479=CARTESIAN_POINT('',(55.6659786555824,25.1974959714464,6.9));
#42480=CARTESIAN_POINT('Origin',(55.,21.,6.9));
#42481=CARTESIAN_POINT('',(55.6659786555824,25.1974959714464,2.9));
#42482=CARTESIAN_POINT('',(55.6659786555824,25.1974959714464,7.5));
#42483=CARTESIAN_POINT('',(55.0730265828477,25.2493725558249,2.9));
#42484=CARTESIAN_POINT('Origin',(55.,21.,2.9));
#42485=CARTESIAN_POINT('',(55.0730265828477,25.2493725558249,6.9));
#42486=CARTESIAN_POINT('',(55.0730265828477,25.2493725558249,7.5));
#42487=CARTESIAN_POINT('',(54.9269734171523,25.2493725558249,6.9));
#42488=CARTESIAN_POINT('Origin',(55.,21.,6.9));
#42489=CARTESIAN_POINT('',(54.9269734171523,25.2493725558249,2.9));
#42490=CARTESIAN_POINT('',(54.9269734171523,25.2493725558249,7.5));
#42491=CARTESIAN_POINT('',(54.3340213444176,25.1974959714464,2.9));
#42492=CARTESIAN_POINT('Origin',(55.,21.,2.9));
#42493=CARTESIAN_POINT('',(54.3340213444176,25.1974959714464,6.9));
#42494=CARTESIAN_POINT('',(54.3340213444176,25.1974959714464,7.5));
#42495=CARTESIAN_POINT('',(54.1901870544887,25.1721341053809,6.9));
#42496=CARTESIAN_POINT('Origin',(55.,21.,6.9));
#42497=CARTESIAN_POINT('',(54.1901870544887,25.1721341053809,2.9));
#42498=CARTESIAN_POINT('',(54.1901870544887,25.1721341053809,7.5));
#42499=CARTESIAN_POINT('',(53.6152515304358,25.0180805960109,2.9));
#42500=CARTESIAN_POINT('Origin',(55.,21.,2.9));
#42501=CARTESIAN_POINT('',(53.6152515304358,25.0180805960109,6.9));
#42502=CARTESIAN_POINT('',(53.6152515304358,25.0180805960109,7.5));
#42503=CARTESIAN_POINT('',(53.4780064483894,24.9681274713466,6.9));
#42504=CARTESIAN_POINT('Origin',(55.,21.,6.9));
#42505=CARTESIAN_POINT('',(53.4780064483894,24.9681274713466,2.9));
#42506=CARTESIAN_POINT('',(53.4780064483894,24.9681274713466,7.5));
#42507=CARTESIAN_POINT('',(52.9385565979853,24.7165778749126,2.9));
#42508=CARTESIAN_POINT('Origin',(55.,21.,2.9));
#42509=CARTESIAN_POINT('',(52.9385565979853,24.7165778749126,6.9));
#42510=CARTESIAN_POINT('',(52.9385565979853,24.7165778749126,7.5));
#42511=CARTESIAN_POINT('',(52.8120708461899,24.6435512920649,6.9));
#42512=CARTESIAN_POINT('Origin',(55.,21.,6.9));
#42513=CARTESIAN_POINT('',(52.8120708461899,24.6435512920649,2.9));
#42514=CARTESIAN_POINT('',(52.8120708461899,24.6435512920649,7.5));
#42515=CARTESIAN_POINT('',(52.3244975801642,24.3021488157642,2.9));
#42516=CARTESIAN_POINT('Origin',(55.,21.,2.9));
#42517=CARTESIAN_POINT('',(52.3244975801642,24.3021488157642,6.9));
#42518=CARTESIAN_POINT('',(52.3244975801642,24.3021488157642,7.5));
#42519=CARTESIAN_POINT('',(52.2126143641833,24.2082676504997,6.9));
#42520=CARTESIAN_POINT('Origin',(55.,21.,6.9));
#42521=CARTESIAN_POINT('',(52.2126143641833,24.2082676504997,2.9));
#42522=CARTESIAN_POINT('',(52.2126143641833,24.2082676504997,7.5));
#42523=CARTESIAN_POINT('',(51.7917323495003,23.7873856358167,2.9));
#42524=CARTESIAN_POINT('Origin',(55.,21.,2.9));
#42525=CARTESIAN_POINT('',(51.7917323495003,23.7873856358167,6.9));
#42526=CARTESIAN_POINT('',(51.7917323495003,23.7873856358167,7.5));
#42527=CARTESIAN_POINT('',(51.6978511842358,23.6755024198358,6.9));
#42528=CARTESIAN_POINT('Origin',(55.,21.,6.9));
#42529=CARTESIAN_POINT('',(51.6978511842358,23.6755024198358,2.9));
#42530=CARTESIAN_POINT('',(51.6978511842358,23.6755024198358,7.5));
#42531=CARTESIAN_POINT('',(51.3564487079351,23.1879291538101,2.9));
#42532=CARTESIAN_POINT('Origin',(55.,21.,2.9));
#42533=CARTESIAN_POINT('',(51.3564487079351,23.1879291538101,6.9));
#42534=CARTESIAN_POINT('',(51.3564487079351,23.1879291538101,7.5));
#42535=CARTESIAN_POINT('',(51.2834221250874,23.0614434020147,6.9));
#42536=CARTESIAN_POINT('Origin',(55.,21.,6.9));
#42537=CARTESIAN_POINT('',(51.2834221250874,23.0614434020147,2.9));
#42538=CARTESIAN_POINT('',(51.2834221250874,23.0614434020147,7.5));
#42539=CARTESIAN_POINT('',(51.0318725286534,22.5219935516106,2.9));
#42540=CARTESIAN_POINT('Origin',(55.,21.,2.9));
#42541=CARTESIAN_POINT('',(51.0318725286534,22.5219935516106,6.9));
#42542=CARTESIAN_POINT('',(51.0318725286534,22.5219935516106,7.5));
#42543=CARTESIAN_POINT('',(50.9819194039891,22.3847484695642,6.9));
#42544=CARTESIAN_POINT('Origin',(55.,21.,6.9));
#42545=CARTESIAN_POINT('',(50.9819194039891,22.3847484695642,2.9));
#42546=CARTESIAN_POINT('',(50.9819194039891,22.3847484695642,7.5));
#42547=CARTESIAN_POINT('',(50.8278658946191,21.8098129455113,2.9));
#42548=CARTESIAN_POINT('Origin',(55.,21.,2.9));
#42549=CARTESIAN_POINT('',(50.8278658946191,21.8098129455113,6.9));
#42550=CARTESIAN_POINT('',(50.8278658946191,21.8098129455113,7.5));
#42551=CARTESIAN_POINT('',(50.8025040285536,21.6659786555824,6.9));
#42552=CARTESIAN_POINT('Origin',(55.,21.,6.9));
#42553=CARTESIAN_POINT('',(50.8025040285536,21.6659786555824,2.9));
#42554=CARTESIAN_POINT('',(50.8025040285536,21.6659786555824,7.5));
#42555=CARTESIAN_POINT('',(50.7506274441751,21.0730265828477,2.9));
#42556=CARTESIAN_POINT('Origin',(55.,21.,2.9));
#42557=CARTESIAN_POINT('',(50.7506274441751,21.0730265828477,7.5));
#42558=CARTESIAN_POINT('Origin',(59.3508458561075,19.6505407244411,2.5));
#42559=CARTESIAN_POINT('',(58.8527397452222,19.5977174123648,6.9));
#42560=CARTESIAN_POINT('',(59.3508458561075,19.6505407244411,6.9));
#42561=CARTESIAN_POINT('',(58.8527397452222,19.5977174123648,2.75));
#42562=CARTESIAN_POINT('',(58.8527397452222,19.5977174123648,2.5));
#42563=CARTESIAN_POINT('Ctrl Pts',(59.018080596011,19.6152515304358,2.90000000000003));
#42564=CARTESIAN_POINT('Ctrl Pts',(58.9339250731542,19.6063269793218,2.82334460824915));
#42565=CARTESIAN_POINT('Ctrl Pts',(58.8527397452222,19.5977174123648,2.75));
#42566=CARTESIAN_POINT('Origin',(58.8527397452222,19.5977174123648,2.5));
#42567=CARTESIAN_POINT('Ctrl Pts',(58.8527397452222,19.5977174123648,2.75));
#42568=CARTESIAN_POINT('Ctrl Pts',(58.9093971915826,19.5389371785566,2.82334460824922));
#42569=CARTESIAN_POINT('Ctrl Pts',(58.9681274713466,19.4780064483894,2.90000000000003));
#42570=CARTESIAN_POINT('',(58.8527397452222,19.5977174123648,6.9));
#42571=CARTESIAN_POINT('Origin',(59.0641705848991,19.5207628801165,6.9));
#42572=CARTESIAN_POINT('Origin',(55.,21.,2.7));
#42573=CARTESIAN_POINT('',(50.9,21.,2.75000000000001));
#42574=CARTESIAN_POINT('Ctrl Pts',(50.9,21.,2.75000000000001));
#42575=CARTESIAN_POINT('Ctrl Pts',(50.826655391751,21.0358573640328,2.82334460824898));
#42576=CARTESIAN_POINT('Ctrl Pts',(50.7506274441751,21.0730265828477,2.90000000000001));
#42577=CARTESIAN_POINT('',(50.9622882126499,21.7119575284344,2.75));
#42578=CARTESIAN_POINT('Ctrl Pts',(50.8025040285536,21.6659786555824,2.90000000000001));
#42579=CARTESIAN_POINT('Ctrl Pts',(50.8838313078845,21.6893810758964,2.82334460824893));
#42580=CARTESIAN_POINT('Ctrl Pts',(50.9622882126499,21.7119575284344,2.75));
#42581=CARTESIAN_POINT('Ctrl Pts',(50.96228821265,21.7119575284344,2.75));
#42582=CARTESIAN_POINT('Ctrl Pts',(50.8962844397247,21.7600062961009,2.82334460824929));
#42583=CARTESIAN_POINT('Ctrl Pts',(50.8278658946191,21.8098129455113,2.90000000000001));
#42584=CARTESIAN_POINT('',(51.1472602547778,22.4022825876352,2.75000000000001));
#42585=CARTESIAN_POINT('Ctrl Pts',(50.9819194039891,22.3847484695642,2.90000000000001));
#42586=CARTESIAN_POINT('Ctrl Pts',(51.0660749268463,22.3936730206783,2.8233446082487));
#42587=CARTESIAN_POINT('Ctrl Pts',(51.1472602547778,22.4022825876352,2.75000000000001));
#42588=CARTESIAN_POINT('Ctrl Pts',(51.1472602547778,22.4022825876352,2.75000000000001));
#42589=CARTESIAN_POINT('Ctrl Pts',(51.0906028084177,22.4610628214431,2.82334460824887));
#42590=CARTESIAN_POINT('Ctrl Pts',(51.0318725286534,22.5219935516106,2.90000000000001));
#42591=CARTESIAN_POINT('',(51.4492958444838,23.05,2.75000000000001));
#42592=CARTESIAN_POINT('Ctrl Pts',(51.2834221250874,23.0614434020147,2.90000000000001));
#42593=CARTESIAN_POINT('Ctrl Pts',(51.3678488684927,23.0556189159593,2.82334460824942));
#42594=CARTESIAN_POINT('Ctrl Pts',(51.4492958444838,23.05,2.75000000000001));
#42595=CARTESIAN_POINT('Ctrl Pts',(51.4492958444838,23.05,2.75000000000001));
#42596=CARTESIAN_POINT('Ctrl Pts',(51.4037062325258,23.1177256922899,2.82334460824926));
#42597=CARTESIAN_POINT('Ctrl Pts',(51.3564487079351,23.1879291538101,2.90000000000001));
#42598=CARTESIAN_POINT('',(51.8592177832122,23.6354291997148,2.75000000000001));
#42599=CARTESIAN_POINT('Ctrl Pts',(51.6978511842358,23.6755024198358,2.90000000000001));
#42600=CARTESIAN_POINT('Ctrl Pts',(51.7799838843138,23.6551058706724,2.82334460824921));
#42601=CARTESIAN_POINT('Ctrl Pts',(51.8592177832122,23.6354291997148,2.75000000000001));
#42602=CARTESIAN_POINT('Ctrl Pts',(51.8592177832122,23.6354291997148,2.75000000000001));
#42603=CARTESIAN_POINT('Ctrl Pts',(51.8260812229464,23.7100425395973,2.8233446082495));
#42604=CARTESIAN_POINT('Ctrl Pts',(51.7917323495003,23.7873856358167,2.90000000000001));
#42605=CARTESIAN_POINT('',(52.3645708002852,24.1407822167878,2.75));
#42606=CARTESIAN_POINT('Ctrl Pts',(52.2126143641833,24.2082676504997,2.90000000000001));
#42607=CARTESIAN_POINT('Ctrl Pts',(52.2899574604024,24.1739187770537,2.82334460824978));
#42608=CARTESIAN_POINT('Ctrl Pts',(52.3645708002852,24.1407822167878,2.75));
#42609=CARTESIAN_POINT('Ctrl Pts',(52.3645708002852,24.1407822167878,2.75));
#42610=CARTESIAN_POINT('Ctrl Pts',(52.3448941293277,24.220016115686,2.82334460824898));
#42611=CARTESIAN_POINT('Ctrl Pts',(52.3244975801642,24.3021488157642,2.90000000000001));
#42612=CARTESIAN_POINT('',(52.95,24.5507041555162,2.75));
#42613=CARTESIAN_POINT('Ctrl Pts',(52.8120708461899,24.6435512920649,2.90000000000001));
#42614=CARTESIAN_POINT('Ctrl Pts',(52.8822743077101,24.5962937674742,2.82334460824929));
#42615=CARTESIAN_POINT('Ctrl Pts',(52.95,24.5507041555162,2.75));
#42616=CARTESIAN_POINT('Ctrl Pts',(52.95,24.5507041555162,2.75));
#42617=CARTESIAN_POINT('Ctrl Pts',(52.9443810840407,24.6321511315072,2.8233446082493));
#42618=CARTESIAN_POINT('Ctrl Pts',(52.9385565979853,24.7165778749126,2.9));
#42619=CARTESIAN_POINT('',(53.5977174123648,24.8527397452222,2.75));
#42620=CARTESIAN_POINT('Ctrl Pts',(53.4780064483894,24.9681274713466,2.90000000000001));
#42621=CARTESIAN_POINT('Ctrl Pts',(53.5389371785568,24.9093971915825,2.82334460824902));
#42622=CARTESIAN_POINT('Ctrl Pts',(53.5977174123648,24.8527397452222,2.75));
#42623=CARTESIAN_POINT('Ctrl Pts',(53.5977174123648,24.8527397452222,2.75));
#42624=CARTESIAN_POINT('Ctrl Pts',(53.6063269793218,24.9339250731547,2.82334460824958));
#42625=CARTESIAN_POINT('Ctrl Pts',(53.6152515304358,25.018080596011,2.90000000000001));
#42626=CARTESIAN_POINT('',(54.2880424715656,25.0377117873501,2.75000000000001));
#42627=CARTESIAN_POINT('Ctrl Pts',(54.1901870544887,25.1721341053809,2.9));
#42628=CARTESIAN_POINT('Ctrl Pts',(54.2399937038992,25.1037155602753,2.82334460824924));
#42629=CARTESIAN_POINT('Ctrl Pts',(54.2880424715656,25.0377117873501,2.75000000000001));
#42630=CARTESIAN_POINT('Ctrl Pts',(54.2880424715656,25.0377117873501,2.75000000000001));
#42631=CARTESIAN_POINT('Ctrl Pts',(54.3106189241037,25.1161686921158,2.82334460824925));
#42632=CARTESIAN_POINT('Ctrl Pts',(54.3340213444176,25.1974959714464,2.90000000000001));
#42633=CARTESIAN_POINT('',(55.,25.1,2.75));
#42634=CARTESIAN_POINT('Ctrl Pts',(54.9269734171523,25.2493725558249,2.9));
#42635=CARTESIAN_POINT('Ctrl Pts',(54.9641426359669,25.1733446082495,2.82334460824949));
#42636=CARTESIAN_POINT('Ctrl Pts',(55.,25.1,2.75));
#42637=CARTESIAN_POINT('Ctrl Pts',(55.,25.1,2.75));
#42638=CARTESIAN_POINT('Ctrl Pts',(55.0358573640329,25.173344608249,2.82334460824903));
#42639=CARTESIAN_POINT('Ctrl Pts',(55.0730265828477,25.2493725558249,2.90000000000001));
#42640=CARTESIAN_POINT('',(55.7119575284344,25.0377117873501,2.75000000000001));
#42641=CARTESIAN_POINT('Ctrl Pts',(55.6659786555824,25.1974959714464,2.90000000000001));
#42642=CARTESIAN_POINT('Ctrl Pts',(55.6893810758964,25.1161686921158,2.82334460824919));
#42643=CARTESIAN_POINT('Ctrl Pts',(55.7119575284344,25.0377117873501,2.75000000000001));
#42644=CARTESIAN_POINT('Ctrl Pts',(55.7119575284344,25.0377117873501,2.75000000000001));
#42645=CARTESIAN_POINT('Ctrl Pts',(55.7600062961009,25.1037155602753,2.82334460824931));
#42646=CARTESIAN_POINT('Ctrl Pts',(55.8098129455113,25.1721341053809,2.9));
#42647=CARTESIAN_POINT('',(56.4022825876352,24.8527397452222,2.75000000000001));
#42648=CARTESIAN_POINT('Ctrl Pts',(56.3847484695642,25.0180805960109,2.9));
#42649=CARTESIAN_POINT('Ctrl Pts',(56.3936730206782,24.9339250731545,2.82334460824946));
#42650=CARTESIAN_POINT('Ctrl Pts',(56.4022825876352,24.8527397452222,2.75000000000001));
#42651=CARTESIAN_POINT('Ctrl Pts',(56.4022825876352,24.8527397452222,2.75000000000001));
#42652=CARTESIAN_POINT('Ctrl Pts',(56.4610628214436,24.9093971915828,2.82334460824951));
#42653=CARTESIAN_POINT('Ctrl Pts',(56.5219935516106,24.9681274713466,2.90000000000001));
#42654=CARTESIAN_POINT('',(57.05,24.5507041555162,2.75000000000001));
#42655=CARTESIAN_POINT('Ctrl Pts',(57.0614434020147,24.7165778749126,2.9));
#42656=CARTESIAN_POINT('Ctrl Pts',(57.0556189159594,24.6321511315074,2.82334460824945));
#42657=CARTESIAN_POINT('Ctrl Pts',(57.05,24.5507041555162,2.75000000000001));
#42658=CARTESIAN_POINT('Ctrl Pts',(57.05,24.5507041555162,2.75000000000001));
#42659=CARTESIAN_POINT('Ctrl Pts',(57.1177256922902,24.5962937674744,2.82334460824958));
#42660=CARTESIAN_POINT('Ctrl Pts',(57.1879291538101,24.6435512920649,2.9));
#42661=CARTESIAN_POINT('',(57.6354291997148,24.1407822167878,2.75000000000001));
#42662=CARTESIAN_POINT('Ctrl Pts',(57.6755024198358,24.3021488157642,2.9));
#42663=CARTESIAN_POINT('Ctrl Pts',(57.6551058706725,24.2200161156869,2.82334460824982));
#42664=CARTESIAN_POINT('Ctrl Pts',(57.6354291997148,24.1407822167878,2.75000000000001));
#42665=CARTESIAN_POINT('Ctrl Pts',(57.6354291997148,24.1407822167878,2.75000000000001));
#42666=CARTESIAN_POINT('Ctrl Pts',(57.7100425395966,24.1739187770533,2.82334460824876));
#42667=CARTESIAN_POINT('Ctrl Pts',(57.7873856358167,24.2082676504997,2.9));
#42668=CARTESIAN_POINT('',(58.1407822167878,23.6354291997148,2.75000000000001));
#42669=CARTESIAN_POINT('Ctrl Pts',(58.2082676504997,23.7873856358167,2.9));
#42670=CARTESIAN_POINT('Ctrl Pts',(58.1739187770533,23.7100425395967,2.82334460824884));
#42671=CARTESIAN_POINT('Ctrl Pts',(58.1407822167878,23.6354291997148,2.75000000000001));
#42672=CARTESIAN_POINT('Ctrl Pts',(58.1407822167878,23.6354291997148,2.75000000000001));
#42673=CARTESIAN_POINT('Ctrl Pts',(58.220016115686,23.6551058706723,2.82334460824898));
#42674=CARTESIAN_POINT('Ctrl Pts',(58.3021488157642,23.6755024198358,2.9));
#42675=CARTESIAN_POINT('',(58.5507041555162,23.05,2.75));
#42676=CARTESIAN_POINT('Ctrl Pts',(58.6435512920649,23.1879291538101,2.9));
#42677=CARTESIAN_POINT('Ctrl Pts',(58.5962937674744,23.1177256922902,2.82334460824956));
#42678=CARTESIAN_POINT('Ctrl Pts',(58.5507041555162,23.05,2.75));
#42679=CARTESIAN_POINT('Ctrl Pts',(58.5507041555162,23.05,2.75));
#42680=CARTESIAN_POINT('Ctrl Pts',(58.632151131507,23.0556189159593,2.82334460824912));
#42681=CARTESIAN_POINT('Ctrl Pts',(58.7165778749126,23.0614434020147,2.9));
#42682=CARTESIAN_POINT('',(58.8527397452222,22.4022825876352,2.75));
#42683=CARTESIAN_POINT('Ctrl Pts',(58.9681274713466,22.5219935516106,2.9));
#42684=CARTESIAN_POINT('Ctrl Pts',(58.9093971915824,22.4610628214431,2.82334460824888));
#42685=CARTESIAN_POINT('Ctrl Pts',(58.8527397452222,22.4022825876352,2.75));
#42686=CARTESIAN_POINT('Ctrl Pts',(58.8527397452222,22.4022825876352,2.75));
#42687=CARTESIAN_POINT('Ctrl Pts',(58.933925073154,22.3936730206782,2.82334460824898));
#42688=CARTESIAN_POINT('Ctrl Pts',(59.0180805960109,22.3847484695642,2.9));
#42689=CARTESIAN_POINT('',(59.0377117873501,21.7119575284344,2.75000000000001));
#42690=CARTESIAN_POINT('Ctrl Pts',(59.1721341053809,21.8098129455113,2.9));
#42691=CARTESIAN_POINT('Ctrl Pts',(59.1037155602755,21.760006296101,2.82334460824946));
#42692=CARTESIAN_POINT('Ctrl Pts',(59.0377117873501,21.7119575284344,2.75000000000001));
#42693=CARTESIAN_POINT('Ctrl Pts',(59.0377117873501,21.7119575284344,2.75000000000001));
#42694=CARTESIAN_POINT('Ctrl Pts',(59.116168692116,21.6893810758963,2.82334460824939));
#42695=CARTESIAN_POINT('Ctrl Pts',(59.1974959714464,21.6659786555824,2.9));
#42696=CARTESIAN_POINT('',(59.1,21.,2.75000000000001));
#42697=CARTESIAN_POINT('Ctrl Pts',(59.2493725558249,21.0730265828477,2.9));
#42698=CARTESIAN_POINT('Ctrl Pts',(59.1733446082494,21.035857364033,2.82334460824937));
#42699=CARTESIAN_POINT('Ctrl Pts',(59.1,21.,2.75000000000001));
#42700=CARTESIAN_POINT('Ctrl Pts',(59.1,21.,2.75000000000001));
#42701=CARTESIAN_POINT('Ctrl Pts',(59.1733446082493,20.964142635967,2.82334460824927));
#42702=CARTESIAN_POINT('Ctrl Pts',(59.2493725558249,20.9269734171523,2.9));
#42703=CARTESIAN_POINT('',(58.5507041555162,18.95,2.75));
#42704=CARTESIAN_POINT('Ctrl Pts',(58.7165778749126,18.9385565979853,2.90000000000002));
#42705=CARTESIAN_POINT('Ctrl Pts',(58.6321511315069,18.9443810840407,2.82334460824905));
#42706=CARTESIAN_POINT('Ctrl Pts',(58.5507041555162,18.95,2.75));
#42707=CARTESIAN_POINT('Ctrl Pts',(58.5507041555162,18.95,2.75));
#42708=CARTESIAN_POINT('Ctrl Pts',(58.596293767474,18.8822743077104,2.8233446082489));
#42709=CARTESIAN_POINT('Ctrl Pts',(58.6435512920649,18.8120708461898,2.90000000000003));
#42710=CARTESIAN_POINT('',(58.1407822167878,18.3645708002852,2.74999999999999));
#42711=CARTESIAN_POINT('Ctrl Pts',(58.3021488157642,18.3244975801642,2.90000000000002));
#42712=CARTESIAN_POINT('Ctrl Pts',(58.2200161156863,18.3448941293276,2.82334460824921));
#42713=CARTESIAN_POINT('Ctrl Pts',(58.1407822167878,18.3645708002852,2.74999999999999));
#42714=CARTESIAN_POINT('Ctrl Pts',(58.1407822167878,18.3645708002852,2.74999999999999));
#42715=CARTESIAN_POINT('Ctrl Pts',(58.1739187770535,18.2899574604028,2.82334460824939));
#42716=CARTESIAN_POINT('Ctrl Pts',(58.2082676504997,18.2126143641833,2.90000000000002));
#42717=CARTESIAN_POINT('',(57.6354291997148,17.8592177832122,2.75000000000001));
#42718=CARTESIAN_POINT('Ctrl Pts',(57.7873856358167,17.7917323495003,2.90000000000002));
#42719=CARTESIAN_POINT('Ctrl Pts',(57.7100425395974,17.8260812229464,2.82334460824953));
#42720=CARTESIAN_POINT('Ctrl Pts',(57.6354291997148,17.8592177832122,2.75000000000001));
#42721=CARTESIAN_POINT('Ctrl Pts',(57.6354291997148,17.8592177832122,2.75000000000001));
#42722=CARTESIAN_POINT('Ctrl Pts',(57.6551058706724,17.7799838843136,2.82334460824937));
#42723=CARTESIAN_POINT('Ctrl Pts',(57.6755024198358,17.6978511842358,2.90000000000002));
#42724=CARTESIAN_POINT('',(57.05,17.4492958444838,2.75));
#42725=CARTESIAN_POINT('Ctrl Pts',(57.1879291538101,17.3564487079351,2.90000000000002));
#42726=CARTESIAN_POINT('Ctrl Pts',(57.1177256922899,17.4037062325258,2.82334460824927));
#42727=CARTESIAN_POINT('Ctrl Pts',(57.05,17.4492958444838,2.75));
#42728=CARTESIAN_POINT('Ctrl Pts',(57.05,17.4492958444838,2.75));
#42729=CARTESIAN_POINT('Ctrl Pts',(57.0556189159594,17.3678488684924,2.82334460824966));
#42730=CARTESIAN_POINT('Ctrl Pts',(57.0614434020148,17.2834221250874,2.90000000000002));
#42731=CARTESIAN_POINT('',(56.4022825876352,17.1472602547778,2.75000000000001));
#42732=CARTESIAN_POINT('Ctrl Pts',(56.5219935516106,17.0318725286534,2.90000000000002));
#42733=CARTESIAN_POINT('Ctrl Pts',(56.4610628214436,17.0906028084172,2.82334460824948));
#42734=CARTESIAN_POINT('Ctrl Pts',(56.4022825876352,17.1472602547778,2.75000000000001));
#42735=CARTESIAN_POINT('Ctrl Pts',(56.4022825876352,17.1472602547778,2.75000000000001));
#42736=CARTESIAN_POINT('Ctrl Pts',(56.3936730206782,17.0660749268454,2.82334460824955));
#42737=CARTESIAN_POINT('Ctrl Pts',(56.3847484695642,16.981919403989,2.90000000000002));
#42738=CARTESIAN_POINT('',(55.7119575284344,16.9622882126499,2.75000000000001));
#42739=CARTESIAN_POINT('Ctrl Pts',(55.8098129455113,16.8278658946191,2.90000000000002));
#42740=CARTESIAN_POINT('Ctrl Pts',(55.760006296101,16.8962844397245,2.82334460824944));
#42741=CARTESIAN_POINT('Ctrl Pts',(55.7119575284344,16.9622882126499,2.75000000000001));
#42742=CARTESIAN_POINT('Ctrl Pts',(55.7119575284344,16.9622882126499,2.75000000000001));
#42743=CARTESIAN_POINT('Ctrl Pts',(55.6893810758963,16.8838313078841,2.82334460824935));
#42744=CARTESIAN_POINT('Ctrl Pts',(55.6659786555824,16.8025040285536,2.90000000000002));
#42745=CARTESIAN_POINT('',(55.,16.9,2.75000000000001));
#42746=CARTESIAN_POINT('Ctrl Pts',(55.0730265828477,16.7506274441751,2.90000000000002));
#42747=CARTESIAN_POINT('Ctrl Pts',(55.035857364033,16.8266553917508,2.82334460824925));
#42748=CARTESIAN_POINT('Ctrl Pts',(55.,16.9,2.75000000000001));
#42749=CARTESIAN_POINT('Ctrl Pts',(55.,16.9,2.75000000000001));
#42750=CARTESIAN_POINT('Ctrl Pts',(54.964142635967,16.8266553917506,2.82334460824936));
#42751=CARTESIAN_POINT('Ctrl Pts',(54.9269734171523,16.7506274441751,2.90000000000002));
#42752=CARTESIAN_POINT('',(54.2880424715656,16.9622882126499,2.75000000000002));
#42753=CARTESIAN_POINT('Ctrl Pts',(54.3340213444176,16.8025040285536,2.90000000000002));
#42754=CARTESIAN_POINT('Ctrl Pts',(54.3106189241037,16.8838313078841,2.82334460824935));
#42755=CARTESIAN_POINT('Ctrl Pts',(54.2880424715656,16.9622882126499,2.75000000000002));
#42756=CARTESIAN_POINT('Ctrl Pts',(54.2880424715656,16.9622882126499,2.75000000000002));
#42757=CARTESIAN_POINT('Ctrl Pts',(54.2399937038991,16.8962844397246,2.82334460824941));
#42758=CARTESIAN_POINT('Ctrl Pts',(54.1901870544887,16.8278658946191,2.90000000000002));
#42759=CARTESIAN_POINT('',(53.5977174123648,17.1472602547778,2.75));
#42760=CARTESIAN_POINT('Ctrl Pts',(53.6152515304358,16.981919403989,2.90000000000002));
#42761=CARTESIAN_POINT('Ctrl Pts',(53.6063269793218,17.0660749268453,2.82334460824959));
#42762=CARTESIAN_POINT('Ctrl Pts',(53.5977174123648,17.1472602547778,2.75));
#42763=CARTESIAN_POINT('Ctrl Pts',(53.5977174123648,17.1472602547778,2.75));
#42764=CARTESIAN_POINT('Ctrl Pts',(53.5389371785566,17.0906028084174,2.82334460824923));
#42765=CARTESIAN_POINT('Ctrl Pts',(53.4780064483894,17.0318725286534,2.90000000000002));
#42766=CARTESIAN_POINT('',(52.95,17.4492958444838,2.75));
#42767=CARTESIAN_POINT('Ctrl Pts',(52.9385565979853,17.2834221250874,2.90000000000002));
#42768=CARTESIAN_POINT('Ctrl Pts',(52.9443810840407,17.3678488684929,2.8233446082492));
#42769=CARTESIAN_POINT('Ctrl Pts',(52.95,17.4492958444838,2.75));
#42770=CARTESIAN_POINT('Ctrl Pts',(52.95,17.4492958444838,2.75));
#42771=CARTESIAN_POINT('Ctrl Pts',(52.88227430771,17.4037062325258,2.82334460824929));
#42772=CARTESIAN_POINT('Ctrl Pts',(52.8120708461899,17.3564487079351,2.90000000000002));
#42773=CARTESIAN_POINT('',(52.3645708002852,17.8592177832122,2.75000000000001));
#42774=CARTESIAN_POINT('Ctrl Pts',(52.3244975801642,17.6978511842358,2.90000000000002));
#42775=CARTESIAN_POINT('Ctrl Pts',(52.3448941293275,17.7799838843134,2.82334460824955));
#42776=CARTESIAN_POINT('Ctrl Pts',(52.3645708002852,17.8592177832122,2.75000000000001));
#42777=CARTESIAN_POINT('Ctrl Pts',(52.3645708002852,17.8592177832122,2.75000000000001));
#42778=CARTESIAN_POINT('Ctrl Pts',(52.2899574604026,17.8260812229464,2.82334460824958));
#42779=CARTESIAN_POINT('Ctrl Pts',(52.2126143641833,17.7917323495003,2.90000000000002));
#42780=CARTESIAN_POINT('',(51.8592177832122,18.3645708002852,2.75));
#42781=CARTESIAN_POINT('Ctrl Pts',(51.7917323495003,18.2126143641833,2.90000000000002));
#42782=CARTESIAN_POINT('Ctrl Pts',(51.8260812229464,18.2899574604027,2.82334460824945));
#42783=CARTESIAN_POINT('Ctrl Pts',(51.8592177832122,18.3645708002852,2.75));
#42784=CARTESIAN_POINT('Ctrl Pts',(51.8592177832122,18.3645708002852,2.75));
#42785=CARTESIAN_POINT('Ctrl Pts',(51.7799838843133,18.3448941293275,2.82334460824967));
#42786=CARTESIAN_POINT('Ctrl Pts',(51.6978511842358,18.3244975801642,2.90000000000001));
#42787=CARTESIAN_POINT('',(51.4492958444838,18.95,2.75));
#42788=CARTESIAN_POINT('Ctrl Pts',(51.3564487079351,18.8120708461899,2.90000000000001));
#42789=CARTESIAN_POINT('Ctrl Pts',(51.403706232526,18.8822743077104,2.82334460824892));
#42790=CARTESIAN_POINT('Ctrl Pts',(51.4492958444838,18.95,2.75));
#42791=CARTESIAN_POINT('Ctrl Pts',(51.4492958444838,18.95,2.75));
#42792=CARTESIAN_POINT('Ctrl Pts',(51.3678488684935,18.9443810840407,2.8233446082487));
#42793=CARTESIAN_POINT('Ctrl Pts',(51.2834221250874,18.9385565979853,2.90000000000001));
#42794=CARTESIAN_POINT('',(51.1472602547778,19.5977174123648,2.75000000000001));
#42795=CARTESIAN_POINT('Ctrl Pts',(51.0318725286534,19.4780064483894,2.90000000000001));
#42796=CARTESIAN_POINT('Ctrl Pts',(51.090602808417,19.5389371785562,2.82334460824971));
#42797=CARTESIAN_POINT('Ctrl Pts',(51.1472602547778,19.5977174123648,2.75000000000001));
#42798=CARTESIAN_POINT('Ctrl Pts',(51.1472602547778,19.5977174123648,2.75000000000001));
#42799=CARTESIAN_POINT('Ctrl Pts',(51.0660749268459,19.6063269793218,2.82334460824904));
#42800=CARTESIAN_POINT('Ctrl Pts',(50.981919403989,19.6152515304358,2.90000000000001));
#42801=CARTESIAN_POINT('',(50.9622882126499,20.2880424715656,2.75000000000002));
#42802=CARTESIAN_POINT('Ctrl Pts',(50.8278658946191,20.1901870544887,2.90000000000001));
#42803=CARTESIAN_POINT('Ctrl Pts',(50.8962844397244,20.2399937038989,2.8233446082496));
#42804=CARTESIAN_POINT('Ctrl Pts',(50.9622882126499,20.2880424715656,2.75000000000002));
#42805=CARTESIAN_POINT('Ctrl Pts',(50.9622882126499,20.2880424715656,2.75000000000002));
#42806=CARTESIAN_POINT('Ctrl Pts',(50.8838313078844,20.3106189241036,2.82334460824907));
#42807=CARTESIAN_POINT('Ctrl Pts',(50.8025040285536,20.3340213444176,2.90000000000001));
#42808=CARTESIAN_POINT('Ctrl Pts',(50.7506274441751,20.9269734171523,2.90000000000001));
#42809=CARTESIAN_POINT('Ctrl Pts',(50.8266553917513,20.9641426359673,2.8233446082487));
#42810=CARTESIAN_POINT('Ctrl Pts',(50.9,21.,2.75000000000001));
#42811=CARTESIAN_POINT('',(51.15,21.,2.5));
#42812=CARTESIAN_POINT('',(50.95,21.,2.7));
#42813=CARTESIAN_POINT('Origin',(55.,21.,2.5));
#42814=CARTESIAN_POINT('Origin',(58.7455598713677,18.8375,6.9));
#42815=CARTESIAN_POINT('',(58.5507041555162,18.95,6.9));
#42816=CARTESIAN_POINT('',(58.5507041555162,18.95,6.9));
#42817=CARTESIAN_POINT('',(59.0504155872192,18.9155255888326,6.9));
#42818=CARTESIAN_POINT('Origin',(59.0504155872192,18.9155255888326,2.5));
#42819=CARTESIAN_POINT('',(58.5507041555162,18.95,2.5));
#42820=CARTESIAN_POINT('Origin',(58.5507041555162,18.95,2.5));
#42821=CARTESIAN_POINT('Origin',(58.6269154903224,18.2438461534124,2.5));
#42822=CARTESIAN_POINT('',(58.1407822167878,18.3645708002852,6.9));
#42823=CARTESIAN_POINT('',(58.6269154903224,18.2438461534124,6.9));
#42824=CARTESIAN_POINT('',(58.1407822167878,18.3645708002852,2.5));
#42825=CARTESIAN_POINT('Origin',(58.1407822167878,18.3645708002852,2.5));
#42826=CARTESIAN_POINT('',(58.1407822167878,18.3645708002852,6.9));
#42827=CARTESIAN_POINT('Origin',(58.3131422164896,18.2199435881057,6.9));
#42828=CARTESIAN_POINT('Origin',(57.7800564118943,17.6868577835104,6.9));
#42829=CARTESIAN_POINT('',(57.6354291997148,17.8592177832122,6.9));
#42830=CARTESIAN_POINT('',(57.6354291997148,17.8592177832122,6.9));
#42831=CARTESIAN_POINT('',(58.0932134015599,17.6559110579397,6.9));
#42832=CARTESIAN_POINT('Origin',(58.0932134015599,17.6559110579397,2.5));
#42833=CARTESIAN_POINT('',(57.6354291997148,17.8592177832122,2.5));
#42834=CARTESIAN_POINT('Origin',(57.6354291997148,17.8592177832122,2.5));
#42835=CARTESIAN_POINT('Origin',(57.4655255888326,17.1695844127808,2.5));
#42836=CARTESIAN_POINT('',(57.05,17.4492958444838,6.9));
#42837=CARTESIAN_POINT('',(57.4655255888326,17.1695844127808,6.9));
#42838=CARTESIAN_POINT('',(57.05,17.4492958444838,2.5));
#42839=CARTESIAN_POINT('Origin',(57.05,17.4492958444838,2.5));
#42840=CARTESIAN_POINT('',(57.05,17.4492958444838,6.9));
#42841=CARTESIAN_POINT('Origin',(57.1625,17.2544401286323,6.9));
#42842=CARTESIAN_POINT('Origin',(56.4792371198835,16.9358294151009,6.9));
#42843=CARTESIAN_POINT('',(56.4022825876352,17.1472602547778,6.9));
#42844=CARTESIAN_POINT('',(56.4022825876352,17.1472602547778,6.9));
#42845=CARTESIAN_POINT('',(56.7629240287047,16.7996430069558,6.9));
#42846=CARTESIAN_POINT('Origin',(56.7629240287047,16.7996430069558,2.5));
#42847=CARTESIAN_POINT('',(56.4022825876352,17.1472602547778,2.5));
#42848=CARTESIAN_POINT('Origin',(56.4022825876352,17.1472602547778,2.5));
#42849=CARTESIAN_POINT('Origin',(56.0067569140472,16.5573273228812,2.5));
#42850=CARTESIAN_POINT('',(55.7119575284344,16.9622882126499,6.9));
#42851=CARTESIAN_POINT('',(56.0067569140472,16.5573273228812,6.9));
#42852=CARTESIAN_POINT('',(55.7119575284344,16.9622882126499,2.5));
#42853=CARTESIAN_POINT('Origin',(55.7119575284344,16.9622882126499,2.5));
#42854=CARTESIAN_POINT('',(55.7119575284344,16.9622882126499,6.9));
#42855=CARTESIAN_POINT('Origin',(55.7510283684095,16.7407064682222,6.9));
#42856=CARTESIAN_POINT('Origin',(55.,16.675,6.9));
#42857=CARTESIAN_POINT('',(55.,16.9,6.9));
#42858=CARTESIAN_POINT('',(55.,16.9,6.9));
#42859=CARTESIAN_POINT('',(55.22,16.45,6.9));
#42860=CARTESIAN_POINT('Origin',(55.22,16.45,2.5));
#42861=CARTESIAN_POINT('',(55.,16.9,2.5));
#42862=CARTESIAN_POINT('Origin',(55.,16.9,2.5));
#42863=CARTESIAN_POINT('Origin',(54.4265584972782,16.4809221247077,2.5));
#42864=CARTESIAN_POINT('',(54.2880424715656,16.9622882126499,6.9));
#42865=CARTESIAN_POINT('',(54.4265584972782,16.4809221247077,6.9));
#42866=CARTESIAN_POINT('',(54.2880424715656,16.9622882126499,2.5));
#42867=CARTESIAN_POINT('Origin',(54.2880424715656,16.9622882126499,2.5));
#42868=CARTESIAN_POINT('',(54.2880424715656,16.9622882126499,6.9));
#42869=CARTESIAN_POINT('Origin',(54.2489716315905,16.7407064682222,6.9));
#42870=CARTESIAN_POINT('Origin',(53.5207628801165,16.9358294151009,6.9));
#42871=CARTESIAN_POINT('',(53.5977174123648,17.1472602547778,6.9));
#42872=CARTESIAN_POINT('',(53.5977174123648,17.1472602547778,6.9));
#42873=CARTESIAN_POINT('',(53.6505407244411,16.6491541438925,6.9));
#42874=CARTESIAN_POINT('Origin',(53.6505407244411,16.6491541438925,2.5));
#42875=CARTESIAN_POINT('',(53.5977174123648,17.1472602547778,2.5));
#42876=CARTESIAN_POINT('Origin',(53.5977174123648,17.1472602547778,2.5));
#42877=CARTESIAN_POINT('Origin',(52.9155255888326,16.9495844127808,2.5));
#42878=CARTESIAN_POINT('',(52.95,17.4492958444838,6.9));
#42879=CARTESIAN_POINT('',(52.9155255888326,16.9495844127808,6.9));
#42880=CARTESIAN_POINT('',(52.95,17.4492958444838,2.5));
#42881=CARTESIAN_POINT('Origin',(52.95,17.4492958444838,2.5));
#42882=CARTESIAN_POINT('',(52.95,17.4492958444838,6.9));
#42883=CARTESIAN_POINT('Origin',(52.8375,17.2544401286323,6.9));
#42884=CARTESIAN_POINT('Origin',(52.2199435881057,17.6868577835104,6.9));
#42885=CARTESIAN_POINT('',(52.3645708002852,17.8592177832122,6.9));
#42886=CARTESIAN_POINT('',(52.3645708002852,17.8592177832122,6.9));
#42887=CARTESIAN_POINT('',(52.2438461534124,17.3730845096776,6.9));
#42888=CARTESIAN_POINT('Origin',(52.2438461534124,17.3730845096776,2.5));
#42889=CARTESIAN_POINT('',(52.3645708002852,17.8592177832122,2.5));
#42890=CARTESIAN_POINT('Origin',(52.3645708002852,17.8592177832122,2.5));
#42891=CARTESIAN_POINT('Origin',(51.6559110579397,17.9067865984401,2.5));
#42892=CARTESIAN_POINT('',(51.8592177832122,18.3645708002852,6.9));
#42893=CARTESIAN_POINT('',(51.6559110579397,17.9067865984401,6.9));
#42894=CARTESIAN_POINT('',(51.8592177832122,18.3645708002852,2.5));
#42895=CARTESIAN_POINT('Origin',(51.8592177832122,18.3645708002852,2.5));
#42896=CARTESIAN_POINT('',(51.8592177832122,18.3645708002852,6.9));
#42897=CARTESIAN_POINT('Origin',(51.6868577835104,18.2199435881057,6.9));
#42898=CARTESIAN_POINT('Origin',(51.2544401286323,18.8375,6.9));
#42899=CARTESIAN_POINT('',(51.4492958444838,18.95,6.9));
#42900=CARTESIAN_POINT('',(51.4492958444838,18.95,6.9));
#42901=CARTESIAN_POINT('',(51.1695844127808,18.5344744111674,6.9));
#42902=CARTESIAN_POINT('Origin',(51.1695844127808,18.5344744111674,2.5));
#42903=CARTESIAN_POINT('',(51.4492958444838,18.95,2.5));
#42904=CARTESIAN_POINT('Origin',(51.4492958444838,18.95,2.5));
#42905=CARTESIAN_POINT('Origin',(50.7996430069557,19.2370759712953,2.5));
#42906=CARTESIAN_POINT('',(51.1472602547778,19.5977174123648,6.9));
#42907=CARTESIAN_POINT('',(50.7996430069557,19.2370759712953,6.9));
#42908=CARTESIAN_POINT('',(51.1472602547778,19.5977174123648,2.5));
#42909=CARTESIAN_POINT('Origin',(51.1472602547778,19.5977174123648,2.5));
#42910=CARTESIAN_POINT('',(51.1472602547778,19.5977174123648,6.9));
#42911=CARTESIAN_POINT('Origin',(50.9358294151009,19.5207628801165,6.9));
#42912=CARTESIAN_POINT('Origin',(50.7407064682222,20.2489716315905,6.9));
#42913=CARTESIAN_POINT('',(50.9622882126499,20.2880424715656,6.9));
#42914=CARTESIAN_POINT('',(50.9622882126499,20.2880424715656,6.9));
#42915=CARTESIAN_POINT('',(50.5573273228812,19.9932430859528,6.9));
#42916=CARTESIAN_POINT('Origin',(50.5573273228812,19.9932430859528,2.5));
#42917=CARTESIAN_POINT('',(50.9622882126499,20.2880424715656,2.5));
#42918=CARTESIAN_POINT('Origin',(50.9622882126499,20.2880424715656,2.5));
#42919=CARTESIAN_POINT('Origin',(50.45,20.78,2.5));
#42920=CARTESIAN_POINT('',(50.9,21.,6.9));
#42921=CARTESIAN_POINT('',(50.45,20.78,6.9));
#42922=CARTESIAN_POINT('',(50.9,21.,2.5));
#42923=CARTESIAN_POINT('Origin',(50.9,21.,2.5));
#42924=CARTESIAN_POINT('',(50.9,21.,6.9));
#42925=CARTESIAN_POINT('Origin',(50.675,21.,6.9));
#42926=CARTESIAN_POINT('Origin',(50.7407064682222,21.7510283684095,6.9));
#42927=CARTESIAN_POINT('',(50.9622882126499,21.7119575284344,6.9));
#42928=CARTESIAN_POINT('',(50.9622882126499,21.7119575284344,6.9));
#42929=CARTESIAN_POINT('',(50.4809221247077,21.5734415027218,6.9));
#42930=CARTESIAN_POINT('Origin',(50.4809221247077,21.5734415027218,2.5));
#42931=CARTESIAN_POINT('',(50.9622882126499,21.7119575284344,2.5));
#42932=CARTESIAN_POINT('Origin',(50.9622882126499,21.7119575284344,2.5));
#42933=CARTESIAN_POINT('Origin',(50.6491541438925,22.3494592755589,2.5));
#42934=CARTESIAN_POINT('',(51.1472602547778,22.4022825876352,6.9));
#42935=CARTESIAN_POINT('',(50.6491541438925,22.3494592755589,6.9));
#42936=CARTESIAN_POINT('',(51.1472602547778,22.4022825876352,2.5));
#42937=CARTESIAN_POINT('Origin',(51.1472602547778,22.4022825876352,2.5));
#42938=CARTESIAN_POINT('',(51.1472602547778,22.4022825876352,6.9));
#42939=CARTESIAN_POINT('Origin',(50.9358294151009,22.4792371198835,6.9));
#42940=CARTESIAN_POINT('Origin',(51.2544401286323,23.1625,6.9));
#42941=CARTESIAN_POINT('',(51.4492958444838,23.05,6.9));
#42942=CARTESIAN_POINT('',(51.4492958444838,23.05,6.9));
#42943=CARTESIAN_POINT('',(50.9495844127808,23.0844744111674,6.9));
#42944=CARTESIAN_POINT('Origin',(50.9495844127808,23.0844744111674,2.5));
#42945=CARTESIAN_POINT('',(51.4492958444838,23.05,2.5));
#42946=CARTESIAN_POINT('Origin',(51.4492958444838,23.05,2.5));
#42947=CARTESIAN_POINT('Origin',(51.3730845096776,23.7561538465876,2.5));
#42948=CARTESIAN_POINT('',(51.8592177832122,23.6354291997148,6.9));
#42949=CARTESIAN_POINT('',(51.3730845096776,23.7561538465876,6.9));
#42950=CARTESIAN_POINT('',(51.8592177832122,23.6354291997148,2.5));
#42951=CARTESIAN_POINT('Origin',(51.8592177832122,23.6354291997148,2.5));
#42952=CARTESIAN_POINT('',(51.8592177832122,23.6354291997148,6.9));
#42953=CARTESIAN_POINT('Origin',(51.6868577835104,23.7800564118943,6.9));
#42954=CARTESIAN_POINT('Origin',(52.2199435881057,24.3131422164896,6.9));
#42955=CARTESIAN_POINT('',(52.3645708002852,24.1407822167878,6.9));
#42956=CARTESIAN_POINT('',(52.3645708002852,24.1407822167878,6.9));
#42957=CARTESIAN_POINT('',(51.9067865984401,24.3440889420603,6.9));
#42958=CARTESIAN_POINT('Origin',(51.9067865984401,24.3440889420603,2.5));
#42959=CARTESIAN_POINT('',(52.3645708002852,24.1407822167878,2.5));
#42960=CARTESIAN_POINT('Origin',(52.3645708002852,24.1407822167878,2.5));
#42961=CARTESIAN_POINT('Origin',(52.5344744111674,24.8304155872192,2.5));
#42962=CARTESIAN_POINT('',(52.95,24.5507041555162,6.9));
#42963=CARTESIAN_POINT('',(52.5344744111674,24.8304155872192,6.9));
#42964=CARTESIAN_POINT('',(52.95,24.5507041555162,2.5));
#42965=CARTESIAN_POINT('Origin',(52.95,24.5507041555162,2.5));
#42966=CARTESIAN_POINT('',(52.95,24.5507041555162,6.9));
#42967=CARTESIAN_POINT('Origin',(52.8375,24.7455598713677,6.9));
#42968=CARTESIAN_POINT('Origin',(53.5207628801165,25.0641705848991,6.9));
#42969=CARTESIAN_POINT('',(53.5977174123648,24.8527397452222,6.9));
#42970=CARTESIAN_POINT('',(53.5977174123648,24.8527397452222,6.9));
#42971=CARTESIAN_POINT('',(53.2370759712953,25.2003569930442,6.9));
#42972=CARTESIAN_POINT('Origin',(53.2370759712953,25.2003569930442,2.5));
#42973=CARTESIAN_POINT('',(53.5977174123648,24.8527397452222,2.5));
#42974=CARTESIAN_POINT('Origin',(53.5977174123648,24.8527397452222,2.5));
#42975=CARTESIAN_POINT('Origin',(53.9932430859528,25.4426726771188,2.5));
#42976=CARTESIAN_POINT('',(54.2880424715656,25.0377117873501,6.9));
#42977=CARTESIAN_POINT('',(53.9932430859528,25.4426726771188,6.9));
#42978=CARTESIAN_POINT('',(54.2880424715656,25.0377117873501,2.5));
#42979=CARTESIAN_POINT('Origin',(54.2880424715656,25.0377117873501,2.5));
#42980=CARTESIAN_POINT('',(54.2880424715656,25.0377117873501,6.9));
#42981=CARTESIAN_POINT('Origin',(54.2489716315905,25.2592935317778,6.9));
#42982=CARTESIAN_POINT('Origin',(55.,25.325,6.9));
#42983=CARTESIAN_POINT('',(55.,25.1,6.9));
#42984=CARTESIAN_POINT('',(55.,25.1,6.9));
#42985=CARTESIAN_POINT('',(54.78,25.55,6.9));
#42986=CARTESIAN_POINT('Origin',(54.78,25.55,2.5));
#42987=CARTESIAN_POINT('',(55.,25.1,2.5));
#42988=CARTESIAN_POINT('Origin',(55.,25.1,2.5));
#42989=CARTESIAN_POINT('Origin',(55.5734415027219,25.5190778752923,2.5));
#42990=CARTESIAN_POINT('',(55.7119575284344,25.0377117873501,6.9));
#42991=CARTESIAN_POINT('',(55.5734415027219,25.5190778752923,6.9));
#42992=CARTESIAN_POINT('',(55.7119575284344,25.0377117873501,2.5));
#42993=CARTESIAN_POINT('Origin',(55.7119575284344,25.0377117873501,2.5));
#42994=CARTESIAN_POINT('',(55.7119575284344,25.0377117873501,6.9));
#42995=CARTESIAN_POINT('Origin',(55.7510283684095,25.2592935317778,6.9));
#42996=CARTESIAN_POINT('Origin',(56.4792371198835,25.0641705848991,6.9));
#42997=CARTESIAN_POINT('',(56.4022825876352,24.8527397452222,6.9));
#42998=CARTESIAN_POINT('',(56.4022825876352,24.8527397452222,6.9));
#42999=CARTESIAN_POINT('',(56.3494592755589,25.3508458561075,6.9));
#43000=CARTESIAN_POINT('Origin',(56.3494592755589,25.3508458561075,2.5));
#43001=CARTESIAN_POINT('',(56.4022825876352,24.8527397452222,2.5));
#43002=CARTESIAN_POINT('Origin',(56.4022825876352,24.8527397452222,2.5));
#43003=CARTESIAN_POINT('Origin',(57.0844744111674,25.0504155872192,2.5));
#43004=CARTESIAN_POINT('',(57.05,24.5507041555162,6.9));
#43005=CARTESIAN_POINT('',(57.0844744111674,25.0504155872192,6.9));
#43006=CARTESIAN_POINT('',(57.05,24.5507041555162,2.5));
#43007=CARTESIAN_POINT('Origin',(57.05,24.5507041555162,2.5));
#43008=CARTESIAN_POINT('',(57.05,24.5507041555162,6.9));
#43009=CARTESIAN_POINT('Origin',(57.1625,24.7455598713677,6.9));
#43010=CARTESIAN_POINT('Origin',(57.7800564118943,24.3131422164896,6.9));
#43011=CARTESIAN_POINT('',(57.6354291997148,24.1407822167878,6.9));
#43012=CARTESIAN_POINT('',(57.6354291997148,24.1407822167878,6.9));
#43013=CARTESIAN_POINT('',(57.7561538465876,24.6269154903224,6.9));
#43014=CARTESIAN_POINT('Origin',(57.7561538465876,24.6269154903224,2.5));
#43015=CARTESIAN_POINT('',(57.6354291997148,24.1407822167878,2.5));
#43016=CARTESIAN_POINT('Origin',(57.6354291997148,24.1407822167878,2.5));
#43017=CARTESIAN_POINT('Origin',(58.3440889420603,24.0932134015599,2.5));
#43018=CARTESIAN_POINT('',(58.1407822167878,23.6354291997148,6.9));
#43019=CARTESIAN_POINT('',(58.3440889420603,24.0932134015599,6.9));
#43020=CARTESIAN_POINT('',(58.1407822167878,23.6354291997148,2.5));
#43021=CARTESIAN_POINT('Origin',(58.1407822167878,23.6354291997148,2.5));
#43022=CARTESIAN_POINT('',(58.1407822167878,23.6354291997148,6.9));
#43023=CARTESIAN_POINT('Origin',(58.3131422164896,23.7800564118943,6.9));
#43024=CARTESIAN_POINT('Origin',(58.7455598713677,23.1625,6.9));
#43025=CARTESIAN_POINT('',(58.5507041555162,23.05,6.9));
#43026=CARTESIAN_POINT('',(58.5507041555162,23.05,6.9));
#43027=CARTESIAN_POINT('',(58.8304155872192,23.4655255888326,6.9));
#43028=CARTESIAN_POINT('Origin',(58.8304155872192,23.4655255888326,2.5));
#43029=CARTESIAN_POINT('',(58.5507041555162,23.05,2.5));
#43030=CARTESIAN_POINT('Origin',(58.5507041555162,23.05,2.5));
#43031=CARTESIAN_POINT('Origin',(59.2003569930442,22.7629240287047,2.5));
#43032=CARTESIAN_POINT('',(58.8527397452222,22.4022825876352,6.9));
#43033=CARTESIAN_POINT('',(59.2003569930442,22.7629240287047,6.9));
#43034=CARTESIAN_POINT('',(58.8527397452222,22.4022825876352,2.5));
#43035=CARTESIAN_POINT('Origin',(58.8527397452222,22.4022825876352,2.5));
#43036=CARTESIAN_POINT('',(58.8527397452222,22.4022825876352,6.9));
#43037=CARTESIAN_POINT('Origin',(59.0641705848991,22.4792371198835,6.9));
#43038=CARTESIAN_POINT('Origin',(59.2592935317778,21.7510283684095,6.9));
#43039=CARTESIAN_POINT('',(59.0377117873501,21.7119575284344,6.9));
#43040=CARTESIAN_POINT('',(59.0377117873501,21.7119575284344,6.9));
#43041=CARTESIAN_POINT('',(59.4426726771188,22.0067569140472,6.9));
#43042=CARTESIAN_POINT('Origin',(59.4426726771188,22.0067569140472,2.5));
#43043=CARTESIAN_POINT('',(59.0377117873501,21.7119575284344,2.5));
#43044=CARTESIAN_POINT('Origin',(59.0377117873501,21.7119575284344,2.5));
#43045=CARTESIAN_POINT('Origin',(59.55,21.22,2.5));
#43046=CARTESIAN_POINT('',(59.1,21.,6.9));
#43047=CARTESIAN_POINT('',(59.55,21.22,6.9));
#43048=CARTESIAN_POINT('',(59.1,21.,2.5));
#43049=CARTESIAN_POINT('Origin',(59.1,21.,2.5));
#43050=CARTESIAN_POINT('',(59.1,21.,6.9));
#43051=CARTESIAN_POINT('Origin',(59.325,21.,6.9));
#43052=CARTESIAN_POINT('Origin',(55.,21.,7.3));
#43053=CARTESIAN_POINT('Origin',(50.95,21.,7.3));
#43054=CARTESIAN_POINT('Origin',(55.,21.,2.5));
#43055=CARTESIAN_POINT('',(52.4405989232415,21.,2.5));
#43056=CARTESIAN_POINT('Origin',(55.,21.,2.5));
#43057=CARTESIAN_POINT('Origin',(55.,21.,2.65));
#43058=CARTESIAN_POINT('',(52.7423796856917,20.9103130885817,2.8));
#43059=CARTESIAN_POINT('',(52.6905989232415,21.,2.75));
#43060=CARTESIAN_POINT('Ctrl Pts',(52.7423796856916,20.9103130885817,2.8));
#43061=CARTESIAN_POINT('Ctrl Pts',(52.7167726432976,20.9546657870398,2.77617372005609));
#43062=CARTESIAN_POINT('Ctrl Pts',(52.6905989232415,21.,2.75));
#43063=CARTESIAN_POINT('',(53.7935186991706,19.0896869114183,2.8));
#43064=CARTESIAN_POINT('Origin',(55.,21.,2.8));
#43065=CARTESIAN_POINT('',(53.8452994616207,19.,2.75));
#43066=CARTESIAN_POINT('Ctrl Pts',(53.8452994616207,19.,2.75));
#43067=CARTESIAN_POINT('Ctrl Pts',(53.8191257415647,19.0453342129602,2.77617372005608));
#43068=CARTESIAN_POINT('Ctrl Pts',(53.7935186991706,19.0896869114183,2.8));
#43069=CARTESIAN_POINT('',(53.9488609865211,19.,2.8));
#43070=CARTESIAN_POINT('Ctrl Pts',(53.9488609865211,19.,2.8));
#43071=CARTESIAN_POINT('Ctrl Pts',(53.8976469017329,19.,2.77617372005608));
#43072=CARTESIAN_POINT('Ctrl Pts',(53.8452994616207,19.,2.75));
#43073=CARTESIAN_POINT('',(56.0511390134789,19.,2.8));
#43074=CARTESIAN_POINT('Origin',(55.,21.,2.8));
#43075=CARTESIAN_POINT('',(56.1547005383793,19.,2.75));
#43076=CARTESIAN_POINT('Ctrl Pts',(56.1547005383793,19.,2.75));
#43077=CARTESIAN_POINT('Ctrl Pts',(56.1023530982671,19.,2.77617372005608));
#43078=CARTESIAN_POINT('Ctrl Pts',(56.0511390134789,19.,2.8));
#43079=CARTESIAN_POINT('',(56.2064813008294,19.0896869114183,2.8));
#43080=CARTESIAN_POINT('Ctrl Pts',(56.2064813008294,19.0896869114183,2.8));
#43081=CARTESIAN_POINT('Ctrl Pts',(56.1808742584353,19.0453342129602,2.77617372005607));
#43082=CARTESIAN_POINT('Ctrl Pts',(56.1547005383793,19.,2.75));
#43083=CARTESIAN_POINT('',(57.2576203143083,20.9103130885817,2.8));
#43084=CARTESIAN_POINT('Origin',(55.,21.,2.8));
#43085=CARTESIAN_POINT('',(57.3094010767585,21.,2.75));
#43086=CARTESIAN_POINT('Ctrl Pts',(57.3094010767585,21.,2.75));
#43087=CARTESIAN_POINT('Ctrl Pts',(57.2832273567024,20.9546657870398,2.77617372005609));
#43088=CARTESIAN_POINT('Ctrl Pts',(57.2576203143084,20.9103130885817,2.8));
#43089=CARTESIAN_POINT('',(57.2576203143084,21.0896869114183,2.8));
#43090=CARTESIAN_POINT('Ctrl Pts',(57.2576203143084,21.0896869114183,2.8));
#43091=CARTESIAN_POINT('Ctrl Pts',(57.2832273567024,21.0453342129602,2.77617372005609));
#43092=CARTESIAN_POINT('Ctrl Pts',(57.3094010767585,21.,2.75));
#43093=CARTESIAN_POINT('',(56.2064813008294,22.9103130885817,2.8));
#43094=CARTESIAN_POINT('Origin',(55.,21.,2.8));
#43095=CARTESIAN_POINT('',(56.1547005383793,23.,2.75));
#43096=CARTESIAN_POINT('Ctrl Pts',(56.1547005383793,23.,2.75));
#43097=CARTESIAN_POINT('Ctrl Pts',(56.1808742584353,22.9546657870398,2.7761737200561));
#43098=CARTESIAN_POINT('Ctrl Pts',(56.2064813008294,22.9103130885817,2.8));
#43099=CARTESIAN_POINT('',(56.0511390134789,23.,2.8));
#43100=CARTESIAN_POINT('Ctrl Pts',(56.051139013479,23.,2.8));
#43101=CARTESIAN_POINT('Ctrl Pts',(56.1023530982671,23.,2.77617372005609));
#43102=CARTESIAN_POINT('Ctrl Pts',(56.1547005383793,23.,2.75));
#43103=CARTESIAN_POINT('',(53.9488609865211,23.,2.8));
#43104=CARTESIAN_POINT('Origin',(55.,21.,2.8));
#43105=CARTESIAN_POINT('',(53.8452994616207,23.,2.75));
#43106=CARTESIAN_POINT('Ctrl Pts',(53.8452994616207,23.,2.75));
#43107=CARTESIAN_POINT('Ctrl Pts',(53.8976469017329,23.,2.77617372005609));
#43108=CARTESIAN_POINT('Ctrl Pts',(53.948860986521,23.,2.8));
#43109=CARTESIAN_POINT('',(53.7935186991706,22.9103130885817,2.8));
#43110=CARTESIAN_POINT('Ctrl Pts',(53.7935186991706,22.9103130885817,2.8));
#43111=CARTESIAN_POINT('Ctrl Pts',(53.8191257415647,22.9546657870398,2.77617372005606));
#43112=CARTESIAN_POINT('Ctrl Pts',(53.8452994616207,23.,2.75));
#43113=CARTESIAN_POINT('',(52.7423796856917,21.0896869114183,2.8));
#43114=CARTESIAN_POINT('Origin',(55.,21.,2.8));
#43115=CARTESIAN_POINT('Ctrl Pts',(52.6905989232415,21.,2.75));
#43116=CARTESIAN_POINT('Ctrl Pts',(52.7167726432976,21.0453342129602,2.77617372005609));
#43117=CARTESIAN_POINT('Ctrl Pts',(52.7423796856916,21.0896869114183,2.8));
#43118=CARTESIAN_POINT('',(52.5905989232415,21.,2.65));
#43119=CARTESIAN_POINT('Origin',(55.,21.,2.65));
#43120=CARTESIAN_POINT('',(57.2576203143083,20.9103130885817,2.5));
#43121=CARTESIAN_POINT('',(57.2576203143083,20.9103130885817,2.65));
#43122=CARTESIAN_POINT('',(56.2064813008294,19.0896869114183,2.5));
#43123=CARTESIAN_POINT('',(56.2064813008294,19.0896869114183,2.65));
#43124=CARTESIAN_POINT('Origin',(55.,21.,2.5));
#43125=CARTESIAN_POINT('Origin',(55.,21.,2.65));
#43126=CARTESIAN_POINT('',(56.2064813008294,22.9103130885817,2.5));
#43127=CARTESIAN_POINT('',(56.2064813008294,22.9103130885817,2.65));
#43128=CARTESIAN_POINT('',(57.2576203143084,21.0896869114183,2.5));
#43129=CARTESIAN_POINT('',(57.2576203143084,21.0896869114183,2.65));
#43130=CARTESIAN_POINT('Origin',(55.,21.,2.5));
#43131=CARTESIAN_POINT('Origin',(55.,21.,2.65));
#43132=CARTESIAN_POINT('',(53.9488609865211,19.,2.5));
#43133=CARTESIAN_POINT('',(53.9488609865211,19.,2.65));
#43134=CARTESIAN_POINT('',(56.0511390134789,19.,2.5));
#43135=CARTESIAN_POINT('Origin',(55.,21.,2.5));
#43136=CARTESIAN_POINT('',(56.0511390134789,19.,2.65));
#43137=CARTESIAN_POINT('Origin',(55.,21.,2.65));
#43138=CARTESIAN_POINT('',(53.9488609865211,23.,2.5));
#43139=CARTESIAN_POINT('',(53.9488609865211,23.,2.65));
#43140=CARTESIAN_POINT('',(56.0511390134789,23.,2.5));
#43141=CARTESIAN_POINT('',(56.0511390134789,23.,2.65));
#43142=CARTESIAN_POINT('Origin',(55.,21.,2.5));
#43143=CARTESIAN_POINT('Origin',(55.,21.,2.65));
#43144=CARTESIAN_POINT('',(52.7423796856917,20.9103130885817,2.5));
#43145=CARTESIAN_POINT('',(52.7423796856917,20.9103130885817,2.65));
#43146=CARTESIAN_POINT('',(53.7935186991706,19.0896869114183,2.5));
#43147=CARTESIAN_POINT('Origin',(55.,21.,2.5));
#43148=CARTESIAN_POINT('',(53.7935186991706,19.0896869114183,2.65));
#43149=CARTESIAN_POINT('Origin',(55.,21.,2.65));
#43150=CARTESIAN_POINT('',(53.7935186991706,22.9103130885817,2.5));
#43151=CARTESIAN_POINT('',(53.7935186991706,22.9103130885817,2.65));
#43152=CARTESIAN_POINT('',(52.7423796856917,21.0896869114183,2.5));
#43153=CARTESIAN_POINT('Origin',(55.,21.,2.5));
#43154=CARTESIAN_POINT('',(52.7423796856917,21.0896869114183,2.65));
#43155=CARTESIAN_POINT('Origin',(56.1547005383793,23.,2.5));
#43156=CARTESIAN_POINT('',(55.5773502691896,23.,2.5));
#43157=CARTESIAN_POINT('',(56.1547005383793,23.,5.));
#43158=CARTESIAN_POINT('',(56.1547005383793,23.,2.5));
#43159=CARTESIAN_POINT('',(53.8452994616207,23.,5.));
#43160=CARTESIAN_POINT('',(56.1547005383793,23.,5.));
#43161=CARTESIAN_POINT('',(53.8452994616207,23.,2.5));
#43162=CARTESIAN_POINT('Origin',(57.3094010767585,21.,2.5));
#43163=CARTESIAN_POINT('',(57.0207259421637,21.5,2.5));
#43164=CARTESIAN_POINT('',(57.3094010767585,21.,5.));
#43165=CARTESIAN_POINT('',(57.3094010767585,21.,2.5));
#43166=CARTESIAN_POINT('',(57.3094010767585,21.,5.));
#43167=CARTESIAN_POINT('Origin',(56.1547005383793,19.,2.5));
#43168=CARTESIAN_POINT('',(56.4433756729741,19.5,2.5));
#43169=CARTESIAN_POINT('',(56.1547005383793,19.,5.));
#43170=CARTESIAN_POINT('',(56.1547005383793,19.,2.5));
#43171=CARTESIAN_POINT('',(56.1547005383793,19.,5.));
#43172=CARTESIAN_POINT('Origin',(55.,21.,2.5));
#43173=CARTESIAN_POINT('Origin',(55.,21.,2.5));
#43174=CARTESIAN_POINT('Origin',(55.,21.,2.5));
#43175=CARTESIAN_POINT('',(54.4226497308104,19.,2.5));
#43176=CARTESIAN_POINT('Origin',(55.,21.,2.5));
#43177=CARTESIAN_POINT('Origin',(55.,21.,2.5));
#43178=CARTESIAN_POINT('',(52.9792740578363,20.5,2.5));
#43179=CARTESIAN_POINT('Origin',(55.,21.,2.5));
#43180=CARTESIAN_POINT('',(53.5566243270259,22.5,2.5));
#43181=CARTESIAN_POINT('Origin',(57.3094010767585,21.,5.));
#43182=CARTESIAN_POINT('',(53.8452994616207,19.,5.));
#43183=CARTESIAN_POINT('',(53.8452994616207,19.,5.));
#43184=CARTESIAN_POINT('Origin',(55.,21.,5.));
#43185=CARTESIAN_POINT('Origin',(57.3094010767585,21.,5.));
#43186=CARTESIAN_POINT('Origin',(55.,21.,5.));
#43187=CARTESIAN_POINT('Origin',(57.3094010767585,21.,5.));
#43188=CARTESIAN_POINT('Origin',(55.,21.,5.));
#43189=CARTESIAN_POINT('Origin',(57.3094010767585,21.,5.));
#43190=CARTESIAN_POINT('Origin',(55.,21.,5.));
#43191=CARTESIAN_POINT('Origin',(57.3094010767585,21.,5.));
#43192=CARTESIAN_POINT('',(52.6905989232415,21.,5.));
#43193=CARTESIAN_POINT('',(53.8452994616207,23.,5.));
#43194=CARTESIAN_POINT('Origin',(55.,21.,5.));
#43195=CARTESIAN_POINT('Origin',(57.3094010767585,21.,5.));
#43196=CARTESIAN_POINT('',(52.6905989232415,21.,5.));
#43197=CARTESIAN_POINT('Origin',(55.,21.,5.));
#43198=CARTESIAN_POINT('Origin',(55.,21.,5.));
#43199=CARTESIAN_POINT('',(55.,21.,6.38762816056403));
#43200=CARTESIAN_POINT('',(52.6905989232415,21.,5.));
#43201=CARTESIAN_POINT('Origin',(53.8452994616207,19.,2.5));
#43202=CARTESIAN_POINT('',(53.8452994616207,19.,2.5));
#43203=CARTESIAN_POINT('Origin',(52.6905989232415,21.,2.5));
#43204=CARTESIAN_POINT('',(52.6905989232415,21.,2.5));
#43205=CARTESIAN_POINT('Origin',(53.8452994616207,23.,2.5));
#81024=UNCERTAINTY_MEASURE_WITH_UNIT(LENGTH_MEASURE(0.01),#81041,
'DISTANCE_ACCURACY_VALUE',
'Maximum model space distance between geometric entities at asserted c
onnectivities');
#81028=UNCERTAINTY_MEASURE_WITH_UNIT(LENGTH_MEASURE(0.01),#81041,
'DISTANCE_ACCURACY_VALUE',
'Maximum model space distance between geometric entities at asserted c
onnectivities');
#81036=(
GEOMETRIC_REPRESENTATION_CONTEXT(3)
GLOBAL_UNCERTAINTY_ASSIGNED_CONTEXT((#81024))
GLOBAL_UNIT_ASSIGNED_CONTEXT((#81041,#81043,#81044))
REPRESENTATION_CONTEXT('','3D')
);
#81040=(
GEOMETRIC_REPRESENTATION_CONTEXT(3)
GLOBAL_UNCERTAINTY_ASSIGNED_CONTEXT((#81028))
GLOBAL_UNIT_ASSIGNED_CONTEXT((#81041,#81043,#81044))
REPRESENTATION_CONTEXT('','3D')
);
#81041=(
LENGTH_UNIT()
NAMED_UNIT(*)
SI_UNIT(.MILLI.,.METRE.)
);
#81043=(
NAMED_UNIT(*)
PLANE_ANGLE_UNIT()
SI_UNIT($,.RADIAN.)
);
#81044=(
NAMED_UNIT(*)
SI_UNIT($,.STERADIAN.)
SOLID_ANGLE_UNIT()
);
#81052=SHAPE_DEFINITION_REPRESENTATION(#81063,#81136);
#81063=PRODUCT_DEFINITION_SHAPE('',$,#81148);
#81136=SHAPE_REPRESENTATION('',(#16085),#81036);
#81140=PRODUCT_DEFINITION_CONTEXT('part definition',#81175,'design');
#81148=PRODUCT_DEFINITION('ISO 4762 - M5 x 20 - 12.9',
'ISO 4762 - M5 x 20 - 12.9',#81159,#81140);
#81159=PRODUCT_DEFINITION_FORMATION('',$,#81184);
#81175=APPLICATION_CONTEXT(
'Core Data for Automotive Mechanical Design Process');
#81176=PRODUCT_CONTEXT('part definition',#81175,'mechanical');
#81184=PRODUCT('ISO 4762 - M5 x 20 - 12.9','ISO 4762 - M5 x 20 - 12.9',
$,(#81176));
#81195=PRESENTATION_STYLE_ASSIGNMENT((#81206));
#81206=SURFACE_STYLE_USAGE(.BOTH.,#81217);
#81217=SURFACE_SIDE_STYLE('',(#81228));
#81228=SURFACE_STYLE_FILL_AREA(#81239);
#81239=FILL_AREA_STYLE('Opaque(199,204,210)',(#81250));
#81250=FILL_AREA_STYLE_COLOUR('Opaque(199,204,210)',#81261);
#81261=COLOUR_RGB('Opaque(199,204,210)', 0.09019608, 0.27058824, 0.51372549);
ENDSEC;
END-ISO-10303-21;
